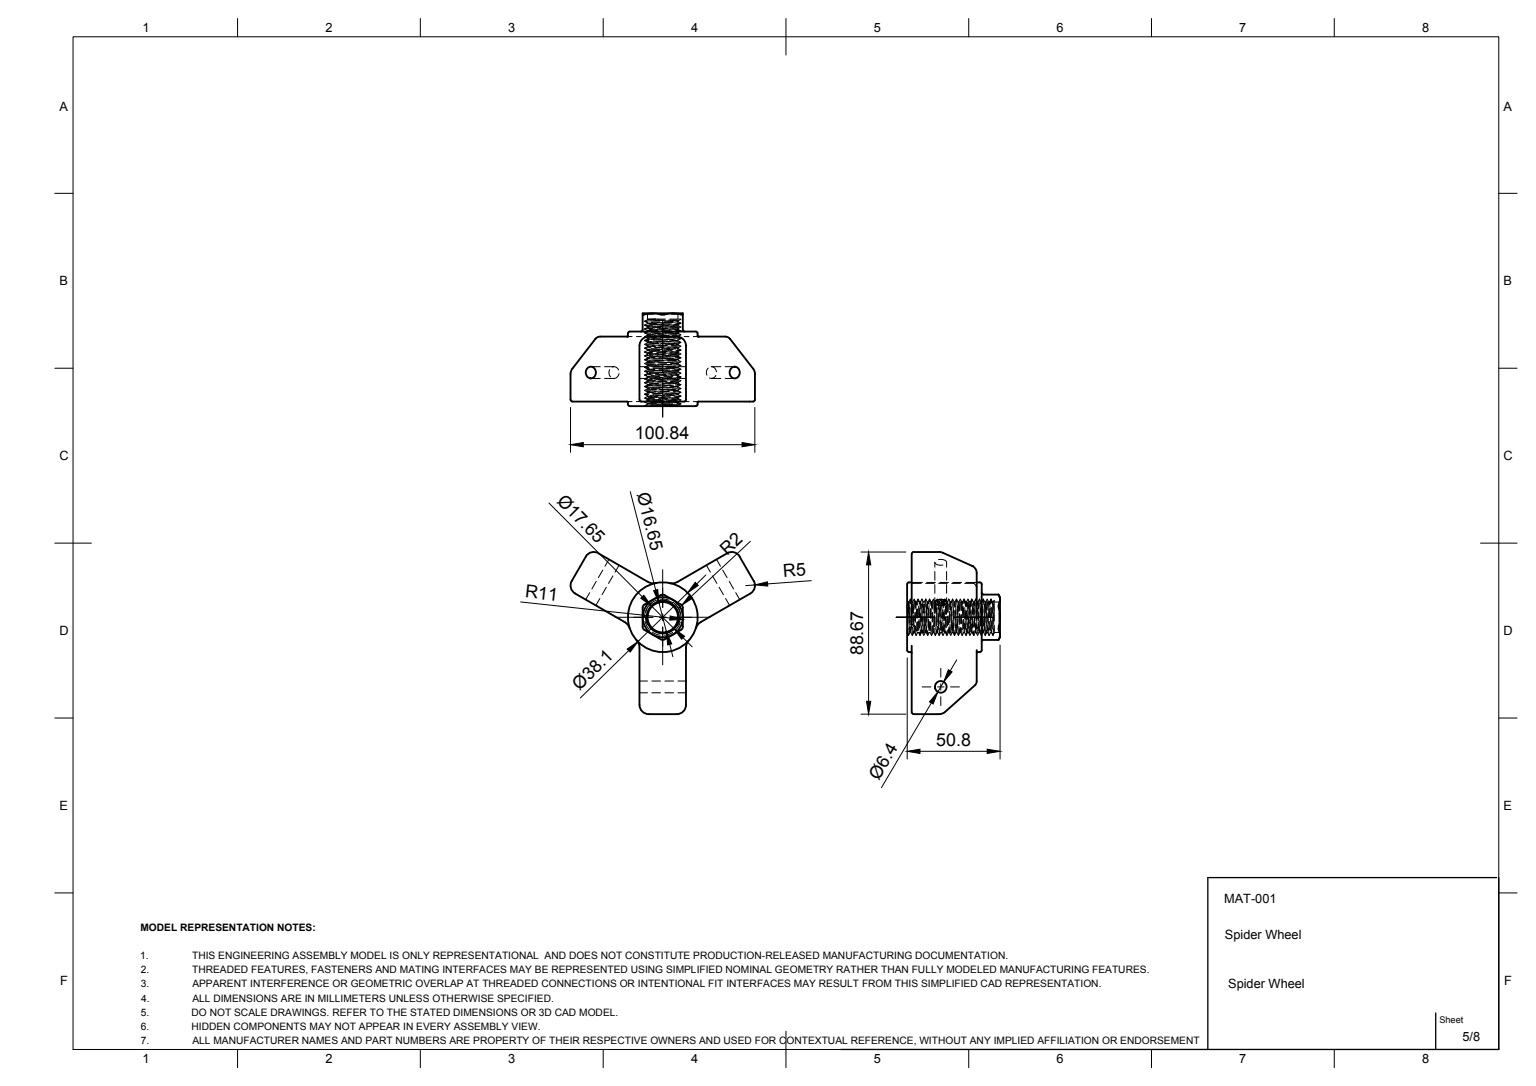
ISO-10303-21;
HEADER;
/* Generated by software containing ST-Developer
 * from STEP Tools, Inc. (www.steptools.com) 
 */

FILE_DESCRIPTION(
/* description */ ('STEP AP214'),
/* implementation_level */ '2;1');

FILE_NAME(
/* name */ 'Spider Wheel.step',
/* time_stamp */ '2026-11-14T04:30:00-08:00',
/* author */ (''),
/* organization */ (''),
/* preprocessor_version */ 'ST-DEVELOPER v20.2',
/* originating_system */ 'Autodesk Translation Framework v15.17.0.0',
/* authorisation */ '');

FILE_SCHEMA (('AUTOMOTIVE_DESIGN { 1 0 10303 214 3 1 1 }'));
ENDSEC;

DATA;
#10=MECHANICAL_DESIGN_GEOMETRIC_PRESENTATION_REPRESENTATION('',(#123),#40809);
#107=SHAPE_REPRESENTATION_RELATIONSHIP('SRR','None',#40857,#115);
#115=ADVANCED_BREP_SHAPE_REPRESENTATION('',(#131),#40801);
#123=STYLED_ITEM('',(#40906),#131);
#131=MANIFOLD_SOLID_BREP('Body1',#6298);
#139=SPHERICAL_SURFACE('',#6615,5.);
#140=SPHERICAL_SURFACE('',#6624,5.);
#141=SPHERICAL_SURFACE('',#6633,5.);
#142=SPHERICAL_SURFACE('',#6642,5.);
#143=SPHERICAL_SURFACE('',#6643,5.);
#144=SPHERICAL_SURFACE('',#6652,5.);
#148=(
BOUNDED_SURFACE()
B_SPLINE_SURFACE(1,2,((#13053,#13054,#13055,#13056,#13057,#13058,#13059,
#13060,#13061,#13062,#13063,#13064,#13065,#13066,#13067,#13068,#13069,#13070,
#13071,#13072,#13073,#13074,#13075,#13076,#13077,#13078,#13079,#13080,#13081,
#13082,#13083,#13084,#13085,#13086,#13087,#13088,#13089,#13090,#13091,#13092,
#13093,#13094,#13095,#13096,#13097,#13098,#13099,#13100,#13101,#13102,#13103,
#13104,#13105,#13106,#13107,#13108,#13109,#13110,#13111,#13112,#13113,#13114,
#13115,#13116,#13117,#13118,#13119,#13120,#13121,#13122,#13123,#13124,#13125,
#13126,#13127,#13128,#13129,#13130,#13131,#13132,#13133,#13134,#13135,#13136,
#13137,#13138,#13139,#13140,#13141,#13142,#13143,#13144,#13145,#13146,#13147,
#13148,#13149,#13150,#13151,#13152,#13153,#13154,#13155,#13156,#13157,#13158,
#13159,#13160,#13161,#13162,#13163,#13164,#13165,#13166,#13167,#13168,#13169,
#13170,#13171,#13172,#13173,#13174,#13175,#13176,#13177,#13178,#13179,#13180,
#13181,#13182,#13183,#13184,#13185,#13186,#13187,#13188,#13189,#13190,#13191,
#13192,#13193,#13194,#13195,#13196,#13197,#13198,#13199,#13200,#13201,#13202,
#13203,#13204,#13205,#13206,#13207,#13208,#13209,#13210,#13211,#13212,#13213,
#13214,#13215,#13216,#13217,#13218,#13219,#13220,#13221,#13222,#13223,#13224,
#13225,#13226,#13227,#13228,#13229,#13230,#13231,#13232,#13233,#13234,#13235,
#13236,#13237,#13238,#13239,#13240,#13241,#13242,#13243,#13244,#13245,#13246,
#13247,#13248,#13249,#13250,#13251,#13252,#13253,#13254,#13255,#13256,#13257,
#13258,#13259,#13260,#13261,#13262,#13263,#13264,#13265,#13266,#13267,#13268,
#13269,#13270,#13271,#13272,#13273,#13274,#13275,#13276,#13277,#13278,#13279,
#13280,#13281,#13282,#13283,#13284,#13285,#13286,#13287,#13288,#13289,#13290,
#13291,#13292,#13293,#13294,#13295,#13296,#13297,#13298,#13299,#13300,#13301,
#13302,#13303,#13304,#13305,#13306,#13307,#13308,#13309,#13310,#13311,#13312,
#13313,#13314,#13315,#13316,#13317,#13318,#13319,#13320,#13321,#13322,#13323,
#13324,#13325,#13326,#13327,#13328,#13329,#13330,#13331,#13332,#13333,#13334,
#13335,#13336,#13337,#13338,#13339,#13340,#13341,#13342,#13343,#13344,#13345,
#13346,#13347,#13348,#13349,#13350,#13351,#13352,#13353,#13354,#13355,#13356,
#13357,#13358,#13359,#13360,#13361,#13362,#13363,#13364,#13365,#13366,#13367,
#13368,#13369,#13370,#13371,#13372,#13373,#13374,#13375,#13376,#13377,#13378,
#13379,#13380,#13381,#13382,#13383,#13384,#13385,#13386,#13387,#13388,#13389,
#13390,#13391,#13392,#13393,#13394,#13395,#13396,#13397,#13398,#13399,#13400,
#13401,#13402,#13403,#13404,#13405,#13406,#13407,#13408,#13409,#13410,#13411,
#13412,#13413,#13414,#13415,#13416,#13417,#13418,#13419,#13420,#13421,#13422,
#13423,#13424,#13425,#13426,#13427,#13428,#13429,#13430,#13431,#13432,#13433,
#13434,#13435,#13436,#13437,#13438,#13439,#13440,#13441,#13442,#13443,#13444,
#13445,#13446,#13447,#13448,#13449,#13450,#13451,#13452,#13453,#13454,#13455,
#13456,#13457,#13458,#13459,#13460,#13461,#13462,#13463,#13464,#13465,#13466,
#13467,#13468,#13469,#13470,#13471,#13472,#13473,#13474,#13475,#13476,#13477,
#13478,#13479,#13480,#13481,#13482,#13483,#13484,#13485,#13486,#13487,#13488,
#13489,#13490,#13491,#13492,#13493,#13494,#13495,#13496,#13497,#13498,#13499,
#13500,#13501,#13502,#13503,#13504,#13505,#13506,#13507,#13508,#13509,#13510,
#13511,#13512,#13513,#13514,#13515,#13516,#13517,#13518,#13519,#13520,#13521,
#13522,#13523,#13524,#13525,#13526,#13527,#13528,#13529,#13530,#13531,#13532,
#13533,#13534,#13535,#13536,#13537,#13538,#13539,#13540,#13541,#13542,#13543,
#13544,#13545,#13546,#13547,#13548,#13549,#13550,#13551,#13552,#13553,#13554,
#13555,#13556,#13557,#13558,#13559,#13560,#13561,#13562,#13563,#13564,#13565,
#13566,#13567,#13568,#13569,#13570,#13571,#13572,#13573,#13574,#13575,#13576,
#13577,#13578,#13579,#13580,#13581,#13582,#13583,#13584,#13585,#13586,#13587,
#13588,#13589,#13590,#13591,#13592,#13593,#13594,#13595,#13596,#13597,#13598,
#13599,#13600,#13601,#13602,#13603,#13604,#13605,#13606,#13607,#13608,#13609,
#13610,#13611,#13612,#13613,#13614,#13615,#13616,#13617,#13618,#13619,#13620,
#13621,#13622,#13623,#13624,#13625,#13626,#13627,#13628,#13629,#13630,#13631,
#13632,#13633,#13634,#13635,#13636,#13637,#13638,#13639,#13640,#13641,#13642,
#13643,#13644,#13645,#13646,#13647,#13648,#13649,#13650,#13651,#13652,#13653,
#13654,#13655,#13656,#13657,#13658,#13659,#13660,#13661,#13662,#13663,#13664,
#13665,#13666,#13667,#13668,#13669,#13670,#13671,#13672,#13673,#13674,#13675,
#13676,#13677,#13678,#13679,#13680,#13681,#13682,#13683,#13684,#13685,#13686,
#13687,#13688,#13689,#13690,#13691,#13692,#13693,#13694,#13695,#13696,#13697,
#13698,#13699,#13700,#13701,#13702,#13703,#13704,#13705,#13706,#13707,#13708,
#13709,#13710,#13711,#13712,#13713,#13714,#13715,#13716,#13717,#13718,#13719,
#13720,#13721,#13722,#13723,#13724,#13725,#13726,#13727,#13728,#13729,#13730,
#13731,#13732,#13733,#13734,#13735,#13736,#13737,#13738,#13739,#13740,#13741,
#13742,#13743,#13744,#13745,#13746,#13747,#13748,#13749,#13750,#13751,#13752,
#13753,#13754,#13755,#13756,#13757,#13758,#13759,#13760,#13761,#13762,#13763,
#13764,#13765,#13766,#13767,#13768,#13769,#13770,#13771,#13772,#13773,#13774,
#13775,#13776,#13777,#13778,#13779,#13780,#13781,#13782,#13783,#13784,#13785,
#13786,#13787,#13788,#13789,#13790,#13791,#13792,#13793,#13794,#13795,#13796,
#13797,#13798,#13799,#13800,#13801,#13802,#13803,#13804,#13805,#13806,#13807,
#13808,#13809,#13810,#13811,#13812,#13813,#13814,#13815,#13816,#13817,#13818,
#13819,#13820,#13821,#13822,#13823,#13824,#13825,#13826,#13827,#13828,#13829,
#13830,#13831,#13832,#13833,#13834,#13835,#13836,#13837,#13838,#13839,#13840,
#13841,#13842,#13843,#13844,#13845,#13846,#13847,#13848,#13849,#13850,#13851,
#13852,#13853,#13854,#13855,#13856,#13857,#13858,#13859,#13860,#13861,#13862,
#13863,#13864,#13865,#13866,#13867,#13868,#13869,#13870,#13871,#13872,#13873,
#13874,#13875,#13876,#13877,#13878,#13879,#13880,#13881,#13882,#13883,#13884,
#13885,#13886,#13887,#13888,#13889,#13890,#13891,#13892,#13893,#13894,#13895,
#13896,#13897,#13898,#13899,#13900,#13901,#13902,#13903,#13904,#13905,#13906,
#13907,#13908,#13909,#13910,#13911,#13912,#13913,#13914,#13915,#13916,#13917,
#13918,#13919,#13920,#13921,#13922,#13923,#13924,#13925,#13926,#13927,#13928,
#13929,#13930,#13931,#13932,#13933,#13934,#13935,#13936,#13937,#13938,#13939,
#13940,#13941,#13942,#13943,#13944,#13945,#13946,#13947,#13948,#13949,#13950,
#13951,#13952,#13953,#13954,#13955,#13956,#13957,#13958,#13959,#13960,#13961,
#13962,#13963,#13964,#13965,#13966,#13967,#13968,#13969,#13970,#13971,#13972,
#13973,#13974,#13975,#13976,#13977,#13978,#13979,#13980,#13981,#13982,#13983,
#13984,#13985,#13986,#13987,#13988,#13989,#13990,#13991,#13992,#13993,#13994,
#13995,#13996,#13997,#13998,#13999,#14000,#14001,#14002,#14003,#14004,#14005,
#14006,#14007,#14008,#14009,#14010,#14011,#14012,#14013,#14014,#14015,#14016,
#14017,#14018,#14019,#14020,#14021,#14022,#14023,#14024,#14025),(#14026,
#14027,#14028,#14029,#14030,#14031,#14032,#14033,#14034,#14035,#14036,#14037,
#14038,#14039,#14040,#14041,#14042,#14043,#14044,#14045,#14046,#14047,#14048,
#14049,#14050,#14051,#14052,#14053,#14054,#14055,#14056,#14057,#14058,#14059,
#14060,#14061,#14062,#14063,#14064,#14065,#14066,#14067,#14068,#14069,#14070,
#14071,#14072,#14073,#14074,#14075,#14076,#14077,#14078,#14079,#14080,#14081,
#14082,#14083,#14084,#14085,#14086,#14087,#14088,#14089,#14090,#14091,#14092,
#14093,#14094,#14095,#14096,#14097,#14098,#14099,#14100,#14101,#14102,#14103,
#14104,#14105,#14106,#14107,#14108,#14109,#14110,#14111,#14112,#14113,#14114,
#14115,#14116,#14117,#14118,#14119,#14120,#14121,#14122,#14123,#14124,#14125,
#14126,#14127,#14128,#14129,#14130,#14131,#14132,#14133,#14134,#14135,#14136,
#14137,#14138,#14139,#14140,#14141,#14142,#14143,#14144,#14145,#14146,#14147,
#14148,#14149,#14150,#14151,#14152,#14153,#14154,#14155,#14156,#14157,#14158,
#14159,#14160,#14161,#14162,#14163,#14164,#14165,#14166,#14167,#14168,#14169,
#14170,#14171,#14172,#14173,#14174,#14175,#14176,#14177,#14178,#14179,#14180,
#14181,#14182,#14183,#14184,#14185,#14186,#14187,#14188,#14189,#14190,#14191,
#14192,#14193,#14194,#14195,#14196,#14197,#14198,#14199,#14200,#14201,#14202,
#14203,#14204,#14205,#14206,#14207,#14208,#14209,#14210,#14211,#14212,#14213,
#14214,#14215,#14216,#14217,#14218,#14219,#14220,#14221,#14222,#14223,#14224,
#14225,#14226,#14227,#14228,#14229,#14230,#14231,#14232,#14233,#14234,#14235,
#14236,#14237,#14238,#14239,#14240,#14241,#14242,#14243,#14244,#14245,#14246,
#14247,#14248,#14249,#14250,#14251,#14252,#14253,#14254,#14255,#14256,#14257,
#14258,#14259,#14260,#14261,#14262,#14263,#14264,#14265,#14266,#14267,#14268,
#14269,#14270,#14271,#14272,#14273,#14274,#14275,#14276,#14277,#14278,#14279,
#14280,#14281,#14282,#14283,#14284,#14285,#14286,#14287,#14288,#14289,#14290,
#14291,#14292,#14293,#14294,#14295,#14296,#14297,#14298,#14299,#14300,#14301,
#14302,#14303,#14304,#14305,#14306,#14307,#14308,#14309,#14310,#14311,#14312,
#14313,#14314,#14315,#14316,#14317,#14318,#14319,#14320,#14321,#14322,#14323,
#14324,#14325,#14326,#14327,#14328,#14329,#14330,#14331,#14332,#14333,#14334,
#14335,#14336,#14337,#14338,#14339,#14340,#14341,#14342,#14343,#14344,#14345,
#14346,#14347,#14348,#14349,#14350,#14351,#14352,#14353,#14354,#14355,#14356,
#14357,#14358,#14359,#14360,#14361,#14362,#14363,#14364,#14365,#14366,#14367,
#14368,#14369,#14370,#14371,#14372,#14373,#14374,#14375,#14376,#14377,#14378,
#14379,#14380,#14381,#14382,#14383,#14384,#14385,#14386,#14387,#14388,#14389,
#14390,#14391,#14392,#14393,#14394,#14395,#14396,#14397,#14398,#14399,#14400,
#14401,#14402,#14403,#14404,#14405,#14406,#14407,#14408,#14409,#14410,#14411,
#14412,#14413,#14414,#14415,#14416,#14417,#14418,#14419,#14420,#14421,#14422,
#14423,#14424,#14425,#14426,#14427,#14428,#14429,#14430,#14431,#14432,#14433,
#14434,#14435,#14436,#14437,#14438,#14439,#14440,#14441,#14442,#14443,#14444,
#14445,#14446,#14447,#14448,#14449,#14450,#14451,#14452,#14453,#14454,#14455,
#14456,#14457,#14458,#14459,#14460,#14461,#14462,#14463,#14464,#14465,#14466,
#14467,#14468,#14469,#14470,#14471,#14472,#14473,#14474,#14475,#14476,#14477,
#14478,#14479,#14480,#14481,#14482,#14483,#14484,#14485,#14486,#14487,#14488,
#14489,#14490,#14491,#14492,#14493,#14494,#14495,#14496,#14497,#14498,#14499,
#14500,#14501,#14502,#14503,#14504,#14505,#14506,#14507,#14508,#14509,#14510,
#14511,#14512,#14513,#14514,#14515,#14516,#14517,#14518,#14519,#14520,#14521,
#14522,#14523,#14524,#14525,#14526,#14527,#14528,#14529,#14530,#14531,#14532,
#14533,#14534,#14535,#14536,#14537,#14538,#14539,#14540,#14541,#14542,#14543,
#14544,#14545,#14546,#14547,#14548,#14549,#14550,#14551,#14552,#14553,#14554,
#14555,#14556,#14557,#14558,#14559,#14560,#14561,#14562,#14563,#14564,#14565,
#14566,#14567,#14568,#14569,#14570,#14571,#14572,#14573,#14574,#14575,#14576,
#14577,#14578,#14579,#14580,#14581,#14582,#14583,#14584,#14585,#14586,#14587,
#14588,#14589,#14590,#14591,#14592,#14593,#14594,#14595,#14596,#14597,#14598,
#14599,#14600,#14601,#14602,#14603,#14604,#14605,#14606,#14607,#14608,#14609,
#14610,#14611,#14612,#14613,#14614,#14615,#14616,#14617,#14618,#14619,#14620,
#14621,#14622,#14623,#14624,#14625,#14626,#14627,#14628,#14629,#14630,#14631,
#14632,#14633,#14634,#14635,#14636,#14637,#14638,#14639,#14640,#14641,#14642,
#14643,#14644,#14645,#14646,#14647,#14648,#14649,#14650,#14651,#14652,#14653,
#14654,#14655,#14656,#14657,#14658,#14659,#14660,#14661,#14662,#14663,#14664,
#14665,#14666,#14667,#14668,#14669,#14670,#14671,#14672,#14673,#14674,#14675,
#14676,#14677,#14678,#14679,#14680,#14681,#14682,#14683,#14684,#14685,#14686,
#14687,#14688,#14689,#14690,#14691,#14692,#14693,#14694,#14695,#14696,#14697,
#14698,#14699,#14700,#14701,#14702,#14703,#14704,#14705,#14706,#14707,#14708,
#14709,#14710,#14711,#14712,#14713,#14714,#14715,#14716,#14717,#14718,#14719,
#14720,#14721,#14722,#14723,#14724,#14725,#14726,#14727,#14728,#14729,#14730,
#14731,#14732,#14733,#14734,#14735,#14736,#14737,#14738,#14739,#14740,#14741,
#14742,#14743,#14744,#14745,#14746,#14747,#14748,#14749,#14750,#14751,#14752,
#14753,#14754,#14755,#14756,#14757,#14758,#14759,#14760,#14761,#14762,#14763,
#14764,#14765,#14766,#14767,#14768,#14769,#14770,#14771,#14772,#14773,#14774,
#14775,#14776,#14777,#14778,#14779,#14780,#14781,#14782,#14783,#14784,#14785,
#14786,#14787,#14788,#14789,#14790,#14791,#14792,#14793,#14794,#14795,#14796,
#14797,#14798,#14799,#14800,#14801,#14802,#14803,#14804,#14805,#14806,#14807,
#14808,#14809,#14810,#14811,#14812,#14813,#14814,#14815,#14816,#14817,#14818,
#14819,#14820,#14821,#14822,#14823,#14824,#14825,#14826,#14827,#14828,#14829,
#14830,#14831,#14832,#14833,#14834,#14835,#14836,#14837,#14838,#14839,#14840,
#14841,#14842,#14843,#14844,#14845,#14846,#14847,#14848,#14849,#14850,#14851,
#14852,#14853,#14854,#14855,#14856,#14857,#14858,#14859,#14860,#14861,#14862,
#14863,#14864,#14865,#14866,#14867,#14868,#14869,#14870,#14871,#14872,#14873,
#14874,#14875,#14876,#14877,#14878,#14879,#14880,#14881,#14882,#14883,#14884,
#14885,#14886,#14887,#14888,#14889,#14890,#14891,#14892,#14893,#14894,#14895,
#14896,#14897,#14898,#14899,#14900,#14901,#14902,#14903,#14904,#14905,#14906,
#14907,#14908,#14909,#14910,#14911,#14912,#14913,#14914,#14915,#14916,#14917,
#14918,#14919,#14920,#14921,#14922,#14923,#14924,#14925,#14926,#14927,#14928,
#14929,#14930,#14931,#14932,#14933,#14934,#14935,#14936,#14937,#14938,#14939,
#14940,#14941,#14942,#14943,#14944,#14945,#14946,#14947,#14948,#14949,#14950,
#14951,#14952,#14953,#14954,#14955,#14956,#14957,#14958,#14959,#14960,#14961,
#14962,#14963,#14964,#14965,#14966,#14967,#14968,#14969,#14970,#14971,#14972,
#14973,#14974,#14975,#14976,#14977,#14978,#14979,#14980,#14981,#14982,#14983,
#14984,#14985,#14986,#14987,#14988,#14989,#14990,#14991,#14992,#14993,#14994,
#14995,#14996,#14997,#14998)),.UNSPECIFIED.,.F.,.F.,.F.)
B_SPLINE_SURFACE_WITH_KNOTS((2,2),(3,2,2,2,2,2,2,2,2,2,2,2,2,2,2,2,2,2,
2,2,2,2,2,2,2,2,2,2,2,2,2,2,2,2,2,2,2,2,2,2,2,2,2,2,2,2,2,2,2,2,2,2,2,2,
2,2,2,2,2,2,2,2,2,2,2,2,2,2,2,2,2,2,2,2,2,2,2,2,2,2,2,2,2,2,2,2,2,2,2,2,
2,2,2,2,2,2,2,2,2,2,2,2,2,2,2,2,2,2,2,2,2,2,2,2,2,2,2,2,2,2,2,2,2,2,2,2,
2,2,2,2,2,2,2,2,2,2,2,2,2,2,2,2,2,2,2,2,2,2,2,2,2,2,2,2,2,2,2,2,2,2,2,2,
2,2,2,2,2,2,2,2,2,2,2,2,2,2,2,2,2,2,2,2,2,2,2,2,2,2,2,2,2,2,2,2,2,2,2,2,
2,2,2,2,2,2,2,2,2,2,2,2,2,2,2,2,2,2,2,2,2,2,2,2,2,2,2,2,2,2,2,2,2,2,2,2,
2,2,2,2,2,2,2,2,2,2,2,2,2,2,2,2,2,2,2,2,2,2,2,2,2,2,2,2,2,2,2,2,2,2,2,2,
2,2,2,2,2,2,2,2,2,2,2,2,2,2,2,2,2,2,2,2,2,2,2,2,2,2,2,2,2,2,2,2,2,2,2,2,
2,2,2,2,2,2,2,2,2,2,2,2,2,2,2,2,2,2,2,2,2,2,2,2,2,2,2,2,2,2,2,2,2,2,2,2,
2,2,2,2,2,2,2,2,2,2,2,2,2,2,2,2,2,2,2,2,2,2,2,2,2,2,2,2,2,2,2,2,2,2,2,2,
2,2,2,2,2,2,2,2,2,2,2,2,2,2,2,2,2,2,2,2,2,2,2,2,2,2,2,2,2,2,2,2,2,2,2,2,
2,2,2,2,2,2,2,2,2,2,2,2,2,2,2,2,2,2,2,2,2,2,2,2,2,2,2,2,2,2,2,2,2,2,2,2,
2,2,2,2,2,2,2,2,2,2,2,2,2,2,2,2,2,2,2,2,2,2,2,2,2,2,2,2,2,2,2,2,2,2,2,2,
3),(0.,1.00000404874212),(0.,0.00205761316872428,0.00411522633744856,0.00617283950617284,
0.00823045267489712,0.0102880658436214,0.0123456790123457,0.01440329218107,
0.0164609053497942,0.0185185185185185,0.0205761316872428,0.0226337448559671,
0.0246913580246914,0.0267489711934156,0.0288065843621399,0.0308641975308642,
0.0329218106995885,0.0349794238683128,0.037037037037037,0.0390946502057613,
0.0411522633744856,0.0432098765432099,0.0452674897119342,0.0473251028806584,
0.0493827160493827,0.051440329218107,0.0534979423868313,0.0555555555555556,
0.0576131687242798,0.0596707818930041,0.0617283950617284,0.0637860082304527,
0.065843621399177,0.0679012345679012,0.0699588477366255,0.0720164609053498,
0.0740740740740741,0.0761316872427984,0.0781893004115226,0.0802469135802469,
0.0823045267489712,0.0843621399176955,0.0864197530864197,0.088477366255144,
0.0905349794238683,0.0925925925925926,0.0946502057613169,0.0967078189300412,
0.0987654320987654,0.10082304526749,0.102880658436214,0.104938271604938,
0.106995884773663,0.109053497942387,0.111111111111111,0.113168724279835,
0.11522633744856,0.117283950617284,0.119341563786008,0.121399176954733,
0.123456790123457,0.125514403292181,0.127572016460905,0.12962962962963,
0.131687242798354,0.133744855967078,0.135802469135802,0.137860082304527,
0.139917695473251,0.141975308641975,0.1440329218107,0.146090534979424,0.148148148148148,
0.150205761316872,0.152263374485597,0.154320987654321,0.156378600823045,
0.15843621399177,0.160493827160494,0.162551440329218,0.164609053497942,
0.166666666666667,0.168724279835391,0.170781893004115,0.172839506172839,
0.174897119341564,0.176954732510288,0.179012345679012,0.181069958847737,
0.183127572016461,0.185185185185185,0.187242798353909,0.189300411522634,
0.191358024691358,0.193415637860082,0.195473251028807,0.197530864197531,
0.199588477366255,0.201646090534979,0.203703703703704,0.205761316872428,
0.207818930041152,0.209876543209877,0.211934156378601,0.213991769547325,
0.216049382716049,0.218106995884774,0.220164609053498,0.222222222222222,
0.224279835390947,0.226337448559671,0.228395061728395,0.230452674897119,
0.232510288065844,0.234567901234568,0.236625514403292,0.238683127572016,
0.240740740740741,0.242798353909465,0.244855967078189,0.246913580246914,
0.248971193415638,0.251028806584362,0.253086419753086,0.255144032921811,
0.257201646090535,0.259259259259259,0.261316872427984,0.263374485596708,
0.265432098765432,0.267489711934156,0.269547325102881,0.271604938271605,
0.273662551440329,0.275720164609054,0.277777777777778,0.279835390946502,
0.281893004115226,0.283950617283951,0.286008230452675,0.288065843621399,
0.290123456790123,0.292181069958848,0.294238683127572,0.296296296296296,
0.298353909465021,0.300411522633745,0.302469135802469,0.304526748971193,
0.306584362139918,0.308641975308642,0.310699588477366,0.312757201646091,
0.314814814814815,0.316872427983539,0.318930041152263,0.320987654320988,
0.323045267489712,0.325102880658436,0.327160493827161,0.329218106995885,
0.331275720164609,0.333333333333333,0.335390946502058,0.337448559670782,
0.339506172839506,0.34156378600823,0.343621399176955,0.345679012345679,
0.347736625514403,0.349794238683128,0.351851851851852,0.353909465020576,
0.3559670781893,0.358024691358025,0.360082304526749,0.362139917695473,0.364197530864198,
0.366255144032922,0.368312757201646,0.37037037037037,0.372427983539095,
0.374485596707819,0.376543209876543,0.378600823045267,0.380658436213992,
0.382716049382716,0.38477366255144,0.386831275720165,0.388888888888889,
0.390946502057613,0.393004115226337,0.395061728395062,0.397119341563786,
0.39917695473251,0.401234567901235,0.403292181069959,0.405349794238683,
0.407407407407407,0.409465020576132,0.411522633744856,0.41358024691358,
0.415637860082305,0.417695473251029,0.419753086419753,0.421810699588477,
0.423868312757202,0.425925925925926,0.42798353909465,0.430041152263374,
0.432098765432099,0.434156378600823,0.436213991769547,0.438271604938272,
0.440329218106996,0.44238683127572,0.444444444444444,0.446502057613169,
0.448559670781893,0.450617283950617,0.452674897119342,0.454732510288066,
0.45679012345679,0.458847736625514,0.460905349794239,0.462962962962963,
0.465020576131687,0.467078189300412,0.469135802469136,0.47119341563786,
0.473251028806584,0.475308641975309,0.477366255144033,0.479423868312757,
0.481481481481481,0.483539094650206,0.48559670781893,0.487654320987654,
0.489711934156379,0.491769547325103,0.493827160493827,0.495884773662551,
0.497942386831276,0.5,0.502057613168724,0.504115226337449,0.506172839506173,
0.508230452674897,0.510288065843621,0.512345679012346,0.51440329218107,
0.516460905349794,0.518518518518518,0.520576131687243,0.522633744855967,
0.524691358024691,0.526748971193416,0.52880658436214,0.530864197530864,
0.532921810699588,0.534979423868313,0.537037037037037,0.539094650205761,
0.541152263374486,0.54320987654321,0.545267489711934,0.547325102880658,
0.549382716049383,0.551440329218107,0.553497942386831,0.555555555555556,
0.55761316872428,0.559670781893004,0.561728395061728,0.563786008230453,
0.565843621399177,0.567901234567901,0.569958847736626,0.57201646090535,
0.574074074074074,0.576131687242798,0.578189300411523,0.580246913580247,
0.582304526748971,0.584362139917695,0.58641975308642,0.588477366255144,
0.590534979423868,0.592592592592593,0.594650205761317,0.596707818930041,
0.598765432098765,0.60082304526749,0.602880658436214,0.604938271604938,
0.606995884773663,0.609053497942387,0.611111111111111,0.613168724279835,
0.61522633744856,0.617283950617284,0.619341563786008,0.621399176954732,
0.623456790123457,0.625514403292181,0.627572016460905,0.62962962962963,
0.631687242798354,0.633744855967078,0.635802469135803,0.637860082304527,
0.639917695473251,0.641975308641975,0.6440329218107,0.646090534979424,0.648148148148148,
0.650205761316872,0.652263374485597,0.654320987654321,0.656378600823045,
0.65843621399177,0.660493827160494,0.662551440329218,0.664609053497942,
0.666666666666667,0.668724279835391,0.670781893004115,0.672839506172839,
0.674897119341564,0.676954732510288,0.679012345679012,0.681069958847737,
0.683127572016461,0.685185185185185,0.687242798353909,0.689300411522634,
0.691358024691358,0.693415637860082,0.695473251028807,0.697530864197531,
0.699588477366255,0.701646090534979,0.703703703703704,0.705761316872428,
0.707818930041152,0.709876543209877,0.711934156378601,0.713991769547325,
0.716049382716049,0.718106995884774,0.720164609053498,0.722222222222222,
0.724279835390947,0.726337448559671,0.728395061728395,0.730452674897119,
0.732510288065844,0.734567901234568,0.736625514403292,0.738683127572016,
0.740740740740741,0.742798353909465,0.744855967078189,0.746913580246914,
0.748971193415638,0.751028806584362,0.753086419753086,0.755144032921811,
0.757201646090535,0.759259259259259,0.761316872427984,0.763374485596708,
0.765432098765432,0.767489711934156,0.769547325102881,0.771604938271605,
0.773662551440329,0.775720164609053,0.777777777777778,0.779835390946502,
0.781893004115226,0.783950617283951,0.786008230452675,0.788065843621399,
0.790123456790123,0.792181069958848,0.794238683127572,0.796296296296296,
0.798353909465021,0.800411522633745,0.802469135802469,0.804526748971193,
0.806584362139918,0.808641975308642,0.810699588477366,0.812757201646091,
0.814814814814815,0.816872427983539,0.818930041152263,0.820987654320988,
0.823045267489712,0.825102880658436,0.827160493827161,0.829218106995885,
0.831275720164609,0.833333333333333,0.835390946502058,0.837448559670782,
0.839506172839506,0.84156378600823,0.843621399176955,0.845679012345679,
0.847736625514403,0.849794238683128,0.851851851851852,0.853909465020576,
0.8559670781893,0.858024691358025,0.860082304526749,0.862139917695473,0.864197530864197,
0.866255144032922,0.868312757201646,0.87037037037037,0.872427983539095,
0.874485596707819,0.876543209876543,0.878600823045268,0.880658436213992,
0.882716049382716,0.88477366255144,0.886831275720165,0.888888888888889,
0.890946502057613,0.893004115226337,0.895061728395062,0.897119341563786,
0.89917695473251,0.901234567901235,0.903292181069959,0.905349794238683,
0.907407407407407,0.909465020576132,0.911522633744856,0.91358024691358,
0.915637860082305,0.917695473251029,0.919753086419753,0.921810699588477,
0.923868312757202,0.925925925925926,0.92798353909465,0.930041152263374,
0.932098765432099,0.934156378600823,0.936213991769547,0.938271604938272,
0.940329218106996,0.94238683127572,0.944444444444444,0.946502057613169,
0.948559670781893,0.950617283950617,0.952674897119342,0.954732510288066,
0.95679012345679,0.958847736625514,0.960905349794239,0.962962962962963,
0.965020576131687,0.967078189300412,0.969135802469136,0.97119341563786,
0.973251028806584,0.975308641975309,0.977366255144033,0.979423868312757,
0.981481481481482,0.983539094650206,0.98559670781893,0.987654320987654,
0.989711934156379,0.991769547325103,0.993827160493827,0.995884773662551,
0.997942386831276,1.),.UNSPECIFIED.)
GEOMETRIC_REPRESENTATION_ITEM()
RATIONAL_B_SPLINE_SURFACE(((1.,0.866025403784439,1.,0.866025403784439,1.,
0.866025403784439,1.,0.866025403784439,1.,0.866025403784439,1.,0.866025403784439,
1.,0.866025403784439,1.,0.866025403784439,1.,0.866025403784439,1.,0.866025403784439,
1.,0.866025403784439,1.,0.866025403784439,1.,0.866025403784439,1.,0.866025403784439,
1.,0.866025403784439,1.,0.866025403784439,1.,0.866025403784439,1.,0.866025403784439,
1.,0.866025403784439,1.,0.866025403784439,1.,0.866025403784439,1.,0.866025403784439,
1.,0.866025403784439,1.,0.866025403784439,1.,0.866025403784439,1.,0.866025403784439,
1.,0.866025403784439,1.,0.866025403784439,1.,0.866025403784439,1.,0.866025403784439,
1.,0.866025403784439,1.,0.866025403784439,1.,0.866025403784439,1.,0.866025403784439,
1.,0.866025403784439,1.,0.866025403784439,1.,0.866025403784439,1.,0.866025403784439,
1.,0.866025403784439,1.,0.866025403784439,1.,0.866025403784439,1.,0.866025403784439,
1.,0.866025403784439,1.,0.866025403784439,1.,0.866025403784439,1.,0.866025403784439,
1.,0.866025403784439,1.,0.866025403784439,1.,0.866025403784439,1.,0.866025403784439,
1.,0.866025403784439,1.,0.866025403784439,1.,0.866025403784439,1.,0.866025403784439,
1.,0.866025403784439,1.,0.866025403784439,1.,0.866025403784439,1.,0.866025403784439,
1.,0.866025403784439,1.,0.866025403784439,1.,0.866025403784439,1.,0.866025403784439,
1.,0.866025403784439,1.,0.866025403784439,1.,0.866025403784439,1.,0.866025403784439,
1.,0.866025403784439,1.,0.866025403784439,1.,0.866025403784439,1.,0.866025403784439,
1.,0.866025403784439,1.,0.866025403784439,1.,0.866025403784439,1.,0.866025403784439,
1.,0.866025403784439,1.,0.866025403784439,1.,0.866025403784439,1.,0.866025403784439,
1.,0.866025403784439,1.,0.866025403784439,1.,0.866025403784439,1.,0.866025403784439,
1.,0.866025403784439,1.,0.866025403784439,1.,0.866025403784439,1.,0.866025403784439,
1.,0.866025403784439,1.,0.866025403784439,1.,0.866025403784439,1.,0.866025403784439,
1.,0.866025403784439,1.,0.866025403784439,1.,0.866025403784439,1.,0.866025403784439,
1.,0.866025403784439,1.,0.866025403784439,1.,0.866025403784439,1.,0.866025403784439,
1.,0.866025403784439,1.,0.866025403784439,1.,0.866025403784439,1.,0.866025403784439,
1.,0.866025403784439,1.,0.866025403784439,1.,0.866025403784439,1.,0.866025403784439,
1.,0.866025403784439,1.,0.866025403784439,1.,0.866025403784439,1.,0.866025403784439,
1.,0.866025403784439,1.,0.866025403784439,1.,0.866025403784439,1.,0.866025403784439,
1.,0.866025403784439,1.,0.866025403784439,1.,0.866025403784439,1.,0.866025403784439,
1.,0.866025403784439,1.,0.866025403784439,1.,0.866025403784439,1.,0.866025403784439,
1.,0.866025403784439,1.,0.866025403784439,1.,0.866025403784439,1.,0.866025403784439,
1.,0.866025403784439,1.,0.866025403784439,1.,0.866025403784439,1.,0.866025403784439,
1.,0.866025403784439,1.,0.866025403784439,1.,0.866025403784439,1.,0.866025403784439,
1.,0.866025403784439,1.,0.866025403784439,1.,0.866025403784439,1.,0.866025403784439,
1.,0.866025403784439,1.,0.866025403784439,1.,0.866025403784439,1.,0.866025403784439,
1.,0.866025403784439,1.,0.866025403784439,1.,0.866025403784439,1.,0.866025403784439,
1.,0.866025403784439,1.,0.866025403784439,1.,0.866025403784439,1.,0.866025403784439,
1.,0.866025403784439,1.,0.866025403784439,1.,0.866025403784439,1.,0.866025403784439,
1.,0.866025403784439,1.,0.866025403784439,1.,0.866025403784439,1.,0.866025403784439,
1.,0.866025403784439,1.,0.866025403784439,1.,0.866025403784439,1.,0.866025403784439,
1.,0.866025403784439,1.,0.866025403784439,1.,0.866025403784439,1.,0.866025403784439,
1.,0.866025403784439,1.,0.866025403784439,1.,0.866025403784439,1.,0.866025403784439,
1.,0.866025403784439,1.,0.866025403784439,1.,0.866025403784439,1.,0.866025403784439,
1.,0.866025403784439,1.,0.866025403784439,1.,0.866025403784439,1.,0.866025403784439,
1.,0.866025403784439,1.,0.866025403784439,1.,0.866025403784439,1.,0.866025403784439,
1.,0.866025403784439,1.,0.866025403784439,1.,0.866025403784439,1.,0.866025403784439,
1.,0.866025403784439,1.,0.866025403784439,1.,0.866025403784439,1.,0.866025403784439,
1.,0.866025403784439,1.,0.866025403784439,1.,0.866025403784439,1.,0.866025403784439,
1.,0.866025403784439,1.,0.866025403784439,1.,0.866025403784439,1.,0.866025403784439,
1.,0.866025403784439,1.,0.866025403784439,1.,0.866025403784439,1.,0.866025403784439,
1.,0.866025403784439,1.,0.866025403784439,1.,0.866025403784439,1.,0.866025403784439,
1.,0.866025403784439,1.,0.866025403784439,1.,0.866025403784439,1.,0.866025403784439,
1.,0.866025403784439,1.,0.866025403784439,1.,0.866025403784439,1.,0.866025403784439,
1.,0.866025403784439,1.,0.866025403784439,1.,0.866025403784439,1.,0.866025403784439,
1.,0.866025403784439,1.,0.866025403784439,1.,0.866025403784439,1.,0.866025403784439,
1.,0.866025403784439,1.,0.866025403784439,1.,0.866025403784439,1.,0.866025403784439,
1.,0.866025403784439,1.,0.866025403784439,1.,0.866025403784439,1.,0.866025403784439,
1.,0.866025403784439,1.,0.866025403784439,1.,0.866025403784439,1.,0.866025403784439,
1.,0.866025403784439,1.,0.866025403784439,1.,0.866025403784439,1.,0.866025403784439,
1.,0.866025403784439,1.,0.866025403784439,1.,0.866025403784439,1.,0.866025403784439,
1.,0.866025403784439,1.,0.866025403784439,1.,0.866025403784439,1.,0.866025403784439,
1.,0.866025403784439,1.,0.866025403784439,1.,0.866025403784439,1.,0.866025403784439,
1.,0.866025403784439,1.,0.866025403784439,1.,0.866025403784439,1.,0.866025403784439,
1.,0.866025403784439,1.,0.866025403784439,1.,0.866025403784439,1.,0.866025403784439,
1.,0.866025403784439,1.,0.866025403784439,1.,0.866025403784439,1.,0.866025403784439,
1.,0.866025403784439,1.,0.866025403784439,1.,0.866025403784439,1.,0.866025403784439,
1.,0.866025403784439,1.,0.866025403784439,1.,0.866025403784439,1.,0.866025403784439,
1.,0.866025403784439,1.,0.866025403784439,1.,0.866025403784439,1.,0.866025403784439,
1.,0.866025403784439,1.,0.866025403784439,1.,0.866025403784439,1.,0.866025403784439,
1.,0.866025403784439,1.,0.866025403784439,1.,0.866025403784439,1.,0.866025403784439,
1.,0.866025403784439,1.,0.866025403784439,1.,0.866025403784439,1.,0.866025403784439,
1.,0.866025403784439,1.,0.866025403784439,1.,0.866025403784439,1.,0.866025403784439,
1.,0.866025403784439,1.,0.866025403784439,1.,0.866025403784439,1.,0.866025403784439,
1.,0.866025403784439,1.,0.866025403784439,1.,0.866025403784439,1.,0.866025403784439,
1.,0.866025403784439,1.,0.866025403784439,1.,0.866025403784439,1.,0.866025403784439,
1.,0.866025403784439,1.,0.866025403784439,1.,0.866025403784439,1.,0.866025403784439,
1.,0.866025403784439,1.,0.866025403784439,1.,0.866025403784439,1.,0.866025403784439,
1.,0.866025403784439,1.,0.866025403784439,1.,0.866025403784439,1.,0.866025403784439,
1.,0.866025403784439,1.,0.866025403784439,1.,0.866025403784439,1.,0.866025403784439,
1.,0.866025403784439,1.,0.866025403784439,1.,0.866025403784439,1.,0.866025403784439,
1.,0.866025403784439,1.,0.866025403784439,1.,0.866025403784439,1.,0.866025403784439,
1.,0.866025403784439,1.,0.866025403784439,1.,0.866025403784439,1.,0.866025403784439,
1.,0.866025403784439,1.,0.866025403784439,1.,0.866025403784439,1.,0.866025403784439,
1.,0.866025403784439,1.,0.866025403784439,1.,0.866025403784439,1.,0.866025403784439,
1.,0.866025403784439,1.,0.866025403784439,1.,0.866025403784439,1.,0.866025403784439,
1.,0.866025403784439,1.,0.866025403784439,1.,0.866025403784439,1.,0.866025403784439,
1.,0.866025403784439,1.,0.866025403784439,1.,0.866025403784439,1.,0.866025403784439,
1.,0.866025403784439,1.,0.866025403784439,1.,0.866025403784439,1.,0.866025403784439,
1.,0.866025403784439,1.,0.866025403784439,1.,0.866025403784439,1.,0.866025403784439,
1.,0.866025403784439,1.,0.866025403784439,1.,0.866025403784439,1.,0.866025403784439,
1.,0.866025403784439,1.,0.866025403784439,1.,0.866025403784439,1.,0.866025403784439,
1.,0.866025403784439,1.,0.866025403784439,1.,0.866025403784439,1.,0.866025403784439,
1.,0.866025403784439,1.,0.866025403784439,1.,0.866025403784439,1.,0.866025403784439,
1.,0.866025403784439,1.,0.866025403784439,1.,0.866025403784439,1.,0.866025403784439,
1.,0.866025403784439,1.,0.866025403784439,1.,0.866025403784439,1.,0.866025403784439,
1.,0.866025403784439,1.,0.866025403784439,1.,0.866025403784439,1.,0.866025403784439,
1.,0.866025403784439,1.,0.866025403784439,1.,0.866025403784439,1.,0.866025403784439,
1.,0.866025403784439,1.,0.866025403784439,1.,0.866025403784439,1.,0.866025403784439,
1.,0.866025403784439,1.,0.866025403784439,1.,0.866025403784439,1.,0.866025403784439,
1.,0.866025403784439,1.,0.866025403784439,1.,0.866025403784439,1.,0.866025403784439,
1.,0.866025403784439,1.,0.866025403784439,1.,0.866025403784439,1.,0.866025403784439,
1.,0.866025403784439,1.,0.866025403784439,1.,0.866025403784439,1.,0.866025403784439,
1.,0.866025403784439,1.,0.866025403784439,1.,0.866025403784439,1.,0.866025403784439,
1.,0.866025403784439,1.,0.866025403784439,1.,0.866025403784439,1.,0.866025403784439,
1.,0.866025403784439,1.,0.866025403784439,1.,0.866025403784439,1.,0.866025403784439,
1.,0.866025403784439,1.,0.866025403784439,1.,0.866025403784439,1.,0.866025403784439,
1.,0.866025403784439,1.,0.866025403784439,1.,0.866025403784439,1.,0.866025403784439,
1.,0.866025403784439,1.,0.866025403784439,1.,0.866025403784439,1.,0.866025403784439,
1.,0.866025403784439,1.,0.866025403784439,1.,0.866025403784439,1.,0.866025403784439,
1.,0.866025403784439,1.,0.866025403784439,1.,0.866025403784439,1.,0.866025403784439,
1.,0.866025403784439,1.,0.866025403784439,1.,0.866025403784439,1.,0.866025403784439,
1.,0.866025403784439,1.,0.866025403784439,1.,0.866025403784439,1.,0.866025403784439,
1.,0.866025403784439,1.,0.866025403784439,1.,0.866025403784439,1.,0.866025403784439,
1.,0.866025403784439,1.,0.866025403784439,1.,0.866025403784439,1.,0.866025403784439,
1.,0.866025403784439,1.,0.866025403784439,1.,0.866025403784439,1.,0.866025403784439,
1.,0.866025403784439,1.,0.866025403784439,1.,0.866025403784439,1.,0.866025403784439,
1.,0.866025403784439,1.,0.866025403784439,1.,0.866025403784439,1.,0.866025403784439,
1.,0.866025403784439,1.,0.866025403784439,1.,0.866025403784439,1.,0.866025403784439,
1.,0.866025403784439,1.,0.866025403784439,1.,0.866025403784439,1.,0.866025403784439,
1.,0.866025403784439,1.,0.866025403784439,1.,0.866025403784439,1.,0.866025403784439,
1.,0.866025403784439,1.,0.866025403784439,1.,0.866025403784439,1.,0.866025403784439,
1.),(1.,0.866025403784439,1.,0.866025403784439,1.,0.866025403784439,1.,
0.866025403784439,1.,0.866025403784439,1.,0.866025403784439,1.,0.866025403784439,
1.,0.866025403784439,1.,0.866025403784439,1.,0.866025403784439,1.,0.866025403784439,
1.,0.866025403784439,1.,0.866025403784439,1.,0.866025403784439,1.,0.866025403784439,
1.,0.866025403784439,1.,0.866025403784439,1.,0.866025403784439,1.,0.866025403784439,
1.,0.866025403784439,1.,0.866025403784439,1.,0.866025403784439,1.,0.866025403784439,
1.,0.866025403784439,1.,0.866025403784439,1.,0.866025403784439,1.,0.866025403784439,
1.,0.866025403784439,1.,0.866025403784439,1.,0.866025403784439,1.,0.866025403784439,
1.,0.866025403784439,1.,0.866025403784439,1.,0.866025403784439,1.,0.866025403784439,
1.,0.866025403784439,1.,0.866025403784439,1.,0.866025403784439,1.,0.866025403784439,
1.,0.866025403784439,1.,0.866025403784439,1.,0.866025403784439,1.,0.866025403784439,
1.,0.866025403784439,1.,0.866025403784439,1.,0.866025403784439,1.,0.866025403784439,
1.,0.866025403784439,1.,0.866025403784439,1.,0.866025403784439,1.,0.866025403784439,
1.,0.866025403784439,1.,0.866025403784439,1.,0.866025403784439,1.,0.866025403784439,
1.,0.866025403784439,1.,0.866025403784439,1.,0.866025403784439,1.,0.866025403784439,
1.,0.866025403784439,1.,0.866025403784439,1.,0.866025403784439,1.,0.866025403784439,
1.,0.866025403784439,1.,0.866025403784439,1.,0.866025403784439,1.,0.866025403784439,
1.,0.866025403784439,1.,0.866025403784439,1.,0.866025403784439,1.,0.866025403784439,
1.,0.866025403784439,1.,0.866025403784439,1.,0.866025403784439,1.,0.866025403784439,
1.,0.866025403784439,1.,0.866025403784439,1.,0.866025403784439,1.,0.866025403784439,
1.,0.866025403784439,1.,0.866025403784439,1.,0.866025403784439,1.,0.866025403784439,
1.,0.866025403784439,1.,0.866025403784439,1.,0.866025403784439,1.,0.866025403784439,
1.,0.866025403784439,1.,0.866025403784439,1.,0.866025403784439,1.,0.866025403784439,
1.,0.866025403784439,1.,0.866025403784439,1.,0.866025403784439,1.,0.866025403784439,
1.,0.866025403784439,1.,0.866025403784439,1.,0.866025403784439,1.,0.866025403784439,
1.,0.866025403784439,1.,0.866025403784439,1.,0.866025403784439,1.,0.866025403784439,
1.,0.866025403784439,1.,0.866025403784439,1.,0.866025403784439,1.,0.866025403784439,
1.,0.866025403784439,1.,0.866025403784439,1.,0.866025403784439,1.,0.866025403784439,
1.,0.866025403784439,1.,0.866025403784439,1.,0.866025403784439,1.,0.866025403784439,
1.,0.866025403784439,1.,0.866025403784439,1.,0.866025403784439,1.,0.866025403784439,
1.,0.866025403784439,1.,0.866025403784439,1.,0.866025403784439,1.,0.866025403784439,
1.,0.866025403784439,1.,0.866025403784439,1.,0.866025403784439,1.,0.866025403784439,
1.,0.866025403784439,1.,0.866025403784439,1.,0.866025403784439,1.,0.866025403784439,
1.,0.866025403784439,1.,0.866025403784439,1.,0.866025403784439,1.,0.866025403784439,
1.,0.866025403784439,1.,0.866025403784439,1.,0.866025403784439,1.,0.866025403784439,
1.,0.866025403784439,1.,0.866025403784439,1.,0.866025403784439,1.,0.866025403784439,
1.,0.866025403784439,1.,0.866025403784439,1.,0.866025403784439,1.,0.866025403784439,
1.,0.866025403784439,1.,0.866025403784439,1.,0.866025403784439,1.,0.866025403784439,
1.,0.866025403784439,1.,0.866025403784439,1.,0.866025403784439,1.,0.866025403784439,
1.,0.866025403784439,1.,0.866025403784439,1.,0.866025403784439,1.,0.866025403784439,
1.,0.866025403784439,1.,0.866025403784439,1.,0.866025403784439,1.,0.866025403784439,
1.,0.866025403784439,1.,0.866025403784439,1.,0.866025403784439,1.,0.866025403784439,
1.,0.866025403784439,1.,0.866025403784439,1.,0.866025403784439,1.,0.866025403784439,
1.,0.866025403784439,1.,0.866025403784439,1.,0.866025403784439,1.,0.866025403784439,
1.,0.866025403784439,1.,0.866025403784439,1.,0.866025403784439,1.,0.866025403784439,
1.,0.866025403784439,1.,0.866025403784439,1.,0.866025403784439,1.,0.866025403784439,
1.,0.866025403784439,1.,0.866025403784439,1.,0.866025403784439,1.,0.866025403784439,
1.,0.866025403784439,1.,0.866025403784439,1.,0.866025403784439,1.,0.866025403784439,
1.,0.866025403784439,1.,0.866025403784439,1.,0.866025403784439,1.,0.866025403784439,
1.,0.866025403784439,1.,0.866025403784439,1.,0.866025403784439,1.,0.866025403784439,
1.,0.866025403784439,1.,0.866025403784439,1.,0.866025403784439,1.,0.866025403784439,
1.,0.866025403784439,1.,0.866025403784439,1.,0.866025403784439,1.,0.866025403784439,
1.,0.866025403784439,1.,0.866025403784439,1.,0.866025403784439,1.,0.866025403784439,
1.,0.866025403784439,1.,0.866025403784439,1.,0.866025403784439,1.,0.866025403784439,
1.,0.866025403784439,1.,0.866025403784439,1.,0.866025403784439,1.,0.866025403784439,
1.,0.866025403784439,1.,0.866025403784439,1.,0.866025403784439,1.,0.866025403784439,
1.,0.866025403784439,1.,0.866025403784439,1.,0.866025403784439,1.,0.866025403784439,
1.,0.866025403784439,1.,0.866025403784439,1.,0.866025403784439,1.,0.866025403784439,
1.,0.866025403784439,1.,0.866025403784439,1.,0.866025403784439,1.,0.866025403784439,
1.,0.866025403784439,1.,0.866025403784439,1.,0.866025403784439,1.,0.866025403784439,
1.,0.866025403784439,1.,0.866025403784439,1.,0.866025403784439,1.,0.866025403784439,
1.,0.866025403784439,1.,0.866025403784439,1.,0.866025403784439,1.,0.866025403784439,
1.,0.866025403784439,1.,0.866025403784439,1.,0.866025403784439,1.,0.866025403784439,
1.,0.866025403784439,1.,0.866025403784439,1.,0.866025403784439,1.,0.866025403784439,
1.,0.866025403784439,1.,0.866025403784439,1.,0.866025403784439,1.,0.866025403784439,
1.,0.866025403784439,1.,0.866025403784439,1.,0.866025403784439,1.,0.866025403784439,
1.,0.866025403784439,1.,0.866025403784439,1.,0.866025403784439,1.,0.866025403784439,
1.,0.866025403784439,1.,0.866025403784439,1.,0.866025403784439,1.,0.866025403784439,
1.,0.866025403784439,1.,0.866025403784439,1.,0.866025403784439,1.,0.866025403784439,
1.,0.866025403784439,1.,0.866025403784439,1.,0.866025403784439,1.,0.866025403784439,
1.,0.866025403784439,1.,0.866025403784439,1.,0.866025403784439,1.,0.866025403784439,
1.,0.866025403784439,1.,0.866025403784439,1.,0.866025403784439,1.,0.866025403784439,
1.,0.866025403784439,1.,0.866025403784439,1.,0.866025403784439,1.,0.866025403784439,
1.,0.866025403784439,1.,0.866025403784439,1.,0.866025403784439,1.,0.866025403784439,
1.,0.866025403784439,1.,0.866025403784439,1.,0.866025403784439,1.,0.866025403784439,
1.,0.866025403784439,1.,0.866025403784439,1.,0.866025403784439,1.,0.866025403784439,
1.,0.866025403784439,1.,0.866025403784439,1.,0.866025403784439,1.,0.866025403784439,
1.,0.866025403784439,1.,0.866025403784439,1.,0.866025403784439,1.,0.866025403784439,
1.,0.866025403784439,1.,0.866025403784439,1.,0.866025403784439,1.,0.866025403784439,
1.,0.866025403784439,1.,0.866025403784439,1.,0.866025403784439,1.,0.866025403784439,
1.,0.866025403784439,1.,0.866025403784439,1.,0.866025403784439,1.,0.866025403784439,
1.,0.866025403784439,1.,0.866025403784439,1.,0.866025403784439,1.,0.866025403784439,
1.,0.866025403784439,1.,0.866025403784439,1.,0.866025403784439,1.,0.866025403784439,
1.,0.866025403784439,1.,0.866025403784439,1.,0.866025403784439,1.,0.866025403784439,
1.,0.866025403784439,1.,0.866025403784439,1.,0.866025403784439,1.,0.866025403784439,
1.,0.866025403784439,1.,0.866025403784439,1.,0.866025403784439,1.,0.866025403784439,
1.,0.866025403784439,1.,0.866025403784439,1.,0.866025403784439,1.,0.866025403784439,
1.,0.866025403784439,1.,0.866025403784439,1.,0.866025403784439,1.,0.866025403784439,
1.,0.866025403784439,1.,0.866025403784439,1.,0.866025403784439,1.,0.866025403784439,
1.,0.866025403784439,1.,0.866025403784439,1.,0.866025403784439,1.,0.866025403784439,
1.,0.866025403784439,1.,0.866025403784439,1.,0.866025403784439,1.,0.866025403784439,
1.,0.866025403784439,1.,0.866025403784439,1.,0.866025403784439,1.,0.866025403784439,
1.,0.866025403784439,1.,0.866025403784439,1.,0.866025403784439,1.,0.866025403784439,
1.,0.866025403784439,1.,0.866025403784439,1.,0.866025403784439,1.,0.866025403784439,
1.,0.866025403784439,1.,0.866025403784439,1.,0.866025403784439,1.,0.866025403784439,
1.,0.866025403784439,1.,0.866025403784439,1.,0.866025403784439,1.,0.866025403784439,
1.,0.866025403784439,1.,0.866025403784439,1.,0.866025403784439,1.,0.866025403784439,
1.,0.866025403784439,1.,0.866025403784439,1.,0.866025403784439,1.,0.866025403784439,
1.,0.866025403784439,1.,0.866025403784439,1.,0.866025403784439,1.,0.866025403784439,
1.,0.866025403784439,1.,0.866025403784439,1.,0.866025403784439,1.,0.866025403784439,
1.,0.866025403784439,1.,0.866025403784439,1.,0.866025403784439,1.,0.866025403784439,
1.,0.866025403784439,1.,0.866025403784439,1.,0.866025403784439,1.,0.866025403784439,
1.,0.866025403784439,1.,0.866025403784439,1.,0.866025403784439,1.,0.866025403784439,
1.,0.866025403784439,1.,0.866025403784439,1.,0.866025403784439,1.,0.866025403784439,
1.,0.866025403784439,1.,0.866025403784439,1.,0.866025403784439,1.,0.866025403784439,
1.,0.866025403784439,1.,0.866025403784439,1.,0.866025403784439,1.,0.866025403784439,
1.,0.866025403784439,1.,0.866025403784439,1.,0.866025403784439,1.,0.866025403784439,
1.,0.866025403784439,1.,0.866025403784439,1.,0.866025403784439,1.,0.866025403784439,
1.,0.866025403784439,1.,0.866025403784439,1.,0.866025403784439,1.,0.866025403784439,
1.,0.866025403784439,1.,0.866025403784439,1.,0.866025403784439,1.,0.866025403784439,
1.,0.866025403784439,1.,0.866025403784439,1.,0.866025403784439,1.,0.866025403784439,
1.,0.866025403784439,1.,0.866025403784439,1.,0.866025403784439,1.,0.866025403784439,
1.,0.866025403784439,1.,0.866025403784439,1.,0.866025403784439,1.,0.866025403784439,
1.,0.866025403784439,1.,0.866025403784439,1.,0.866025403784439,1.,0.866025403784439,
1.,0.866025403784439,1.,0.866025403784439,1.,0.866025403784439,1.,0.866025403784439,
1.,0.866025403784439,1.,0.866025403784439,1.,0.866025403784439,1.,0.866025403784439,
1.,0.866025403784439,1.,0.866025403784439,1.,0.866025403784439,1.,0.866025403784439,
1.,0.866025403784439,1.,0.866025403784439,1.,0.866025403784439,1.,0.866025403784439,
1.,0.866025403784439,1.,0.866025403784439,1.,0.866025403784439,1.,0.866025403784439,
1.,0.866025403784439,1.,0.866025403784439,1.,0.866025403784439,1.,0.866025403784439,
1.,0.866025403784439,1.,0.866025403784439,1.,0.866025403784439,1.,0.866025403784439,
1.,0.866025403784439,1.,0.866025403784439,1.,0.866025403784439,1.)))
REPRESENTATION_ITEM('')
SURFACE()
);
#149=(
BOUNDED_SURFACE()
B_SPLINE_SURFACE(3,2,((#15547,#15548,#15549,#15550,#15551,#15552,#15553,
#15554,#15555,#15556,#15557,#15558,#15559,#15560,#15561,#15562,#15563,#15564,
#15565,#15566,#15567,#15568,#15569,#15570,#15571,#15572,#15573,#15574,#15575,
#15576,#15577,#15578,#15579,#15580,#15581,#15582,#15583,#15584,#15585,#15586,
#15587,#15588,#15589,#15590,#15591,#15592,#15593,#15594,#15595,#15596,#15597,
#15598,#15599,#15600,#15601,#15602,#15603,#15604,#15605,#15606,#15607,#15608,
#15609,#15610,#15611,#15612,#15613,#15614,#15615,#15616,#15617,#15618,#15619,
#15620,#15621,#15622,#15623,#15624,#15625,#15626,#15627,#15628,#15629,#15630,
#15631,#15632,#15633,#15634,#15635,#15636,#15637,#15638,#15639,#15640,#15641,
#15642,#15643,#15644,#15645,#15646,#15647,#15648,#15649,#15650,#15651,#15652,
#15653,#15654,#15655,#15656,#15657,#15658,#15659,#15660,#15661,#15662,#15663,
#15664,#15665,#15666,#15667,#15668,#15669,#15670,#15671,#15672,#15673,#15674,
#15675,#15676,#15677,#15678,#15679,#15680,#15681,#15682,#15683,#15684,#15685,
#15686,#15687,#15688,#15689,#15690,#15691,#15692,#15693,#15694,#15695,#15696,
#15697,#15698,#15699,#15700,#15701,#15702,#15703,#15704,#15705,#15706,#15707,
#15708,#15709,#15710,#15711,#15712,#15713,#15714,#15715,#15716,#15717,#15718,
#15719,#15720,#15721,#15722,#15723,#15724,#15725,#15726,#15727,#15728,#15729,
#15730,#15731,#15732,#15733,#15734,#15735,#15736,#15737,#15738,#15739,#15740,
#15741,#15742,#15743,#15744,#15745,#15746,#15747,#15748,#15749,#15750,#15751,
#15752,#15753,#15754,#15755,#15756,#15757,#15758,#15759,#15760,#15761,#15762,
#15763,#15764,#15765,#15766,#15767,#15768,#15769,#15770,#15771,#15772,#15773,
#15774,#15775,#15776,#15777,#15778,#15779,#15780,#15781,#15782,#15783,#15784,
#15785,#15786,#15787,#15788,#15789,#15790,#15791,#15792,#15793,#15794,#15795,
#15796,#15797,#15798,#15799,#15800,#15801,#15802,#15803,#15804,#15805,#15806,
#15807,#15808,#15809,#15810,#15811,#15812,#15813,#15814,#15815,#15816,#15817,
#15818,#15819,#15820,#15821,#15822,#15823,#15824,#15825,#15826,#15827,#15828,
#15829,#15830,#15831,#15832,#15833,#15834,#15835,#15836,#15837,#15838,#15839,
#15840,#15841,#15842,#15843,#15844,#15845,#15846,#15847,#15848,#15849,#15850,
#15851,#15852,#15853,#15854,#15855,#15856,#15857,#15858,#15859,#15860,#15861,
#15862,#15863,#15864,#15865,#15866,#15867,#15868,#15869,#15870,#15871,#15872,
#15873,#15874,#15875,#15876,#15877,#15878,#15879,#15880,#15881,#15882,#15883,
#15884,#15885,#15886,#15887,#15888,#15889,#15890,#15891,#15892,#15893,#15894,
#15895,#15896,#15897,#15898,#15899,#15900,#15901,#15902,#15903,#15904,#15905,
#15906,#15907,#15908,#15909,#15910,#15911,#15912,#15913,#15914,#15915,#15916,
#15917,#15918,#15919,#15920,#15921,#15922,#15923,#15924,#15925,#15926,#15927,
#15928,#15929,#15930,#15931,#15932,#15933,#15934,#15935,#15936,#15937,#15938,
#15939,#15940,#15941,#15942,#15943,#15944,#15945,#15946,#15947,#15948,#15949,
#15950,#15951,#15952,#15953,#15954,#15955,#15956,#15957,#15958,#15959,#15960,
#15961,#15962,#15963,#15964,#15965,#15966,#15967,#15968,#15969,#15970,#15971,
#15972,#15973,#15974,#15975,#15976,#15977,#15978,#15979,#15980,#15981,#15982,
#15983,#15984,#15985,#15986,#15987,#15988,#15989,#15990,#15991,#15992,#15993,
#15994,#15995,#15996,#15997,#15998,#15999,#16000,#16001,#16002,#16003,#16004,
#16005,#16006,#16007,#16008,#16009,#16010,#16011,#16012,#16013,#16014,#16015,
#16016,#16017,#16018,#16019,#16020,#16021,#16022,#16023,#16024,#16025,#16026,
#16027,#16028,#16029,#16030,#16031,#16032,#16033,#16034,#16035,#16036,#16037,
#16038,#16039,#16040,#16041,#16042,#16043,#16044,#16045,#16046,#16047,#16048,
#16049,#16050,#16051,#16052,#16053,#16054,#16055,#16056,#16057,#16058,#16059,
#16060,#16061,#16062,#16063,#16064,#16065,#16066,#16067,#16068,#16069,#16070,
#16071,#16072,#16073,#16074,#16075,#16076,#16077,#16078,#16079,#16080,#16081,
#16082,#16083,#16084,#16085,#16086,#16087,#16088,#16089,#16090,#16091,#16092,
#16093,#16094,#16095,#16096,#16097,#16098,#16099,#16100,#16101,#16102,#16103,
#16104,#16105,#16106,#16107,#16108,#16109,#16110,#16111,#16112,#16113,#16114,
#16115,#16116,#16117,#16118,#16119,#16120,#16121,#16122,#16123,#16124,#16125,
#16126,#16127,#16128,#16129,#16130,#16131,#16132,#16133,#16134,#16135,#16136,
#16137,#16138,#16139,#16140,#16141,#16142,#16143,#16144,#16145,#16146,#16147,
#16148,#16149,#16150,#16151,#16152,#16153,#16154,#16155,#16156,#16157,#16158,
#16159,#16160,#16161,#16162,#16163,#16164,#16165,#16166,#16167,#16168,#16169,
#16170,#16171,#16172,#16173,#16174,#16175,#16176,#16177,#16178,#16179,#16180,
#16181,#16182,#16183,#16184,#16185,#16186,#16187,#16188,#16189,#16190,#16191,
#16192,#16193,#16194,#16195,#16196,#16197,#16198,#16199,#16200,#16201,#16202,
#16203,#16204,#16205,#16206,#16207,#16208,#16209,#16210,#16211,#16212,#16213,
#16214,#16215,#16216,#16217,#16218,#16219,#16220,#16221,#16222,#16223,#16224,
#16225,#16226,#16227,#16228,#16229,#16230,#16231,#16232,#16233,#16234,#16235,
#16236,#16237,#16238,#16239,#16240,#16241,#16242,#16243,#16244,#16245,#16246,
#16247,#16248,#16249,#16250,#16251,#16252,#16253,#16254,#16255,#16256,#16257,
#16258,#16259,#16260,#16261,#16262,#16263,#16264,#16265,#16266,#16267,#16268,
#16269,#16270,#16271,#16272,#16273,#16274,#16275,#16276,#16277,#16278,#16279,
#16280,#16281,#16282,#16283,#16284,#16285,#16286,#16287,#16288,#16289,#16290,
#16291,#16292,#16293,#16294,#16295,#16296,#16297,#16298,#16299,#16300,#16301,
#16302,#16303,#16304,#16305,#16306,#16307,#16308,#16309,#16310,#16311,#16312,
#16313,#16314,#16315,#16316,#16317,#16318,#16319,#16320,#16321,#16322,#16323,
#16324,#16325,#16326,#16327,#16328,#16329,#16330,#16331,#16332,#16333,#16334,
#16335,#16336,#16337,#16338,#16339,#16340,#16341,#16342,#16343,#16344,#16345,
#16346,#16347,#16348,#16349,#16350,#16351,#16352,#16353,#16354,#16355,#16356,
#16357,#16358,#16359,#16360,#16361,#16362,#16363,#16364,#16365,#16366,#16367,
#16368,#16369,#16370,#16371,#16372,#16373,#16374,#16375,#16376,#16377,#16378,
#16379,#16380,#16381,#16382,#16383,#16384,#16385,#16386,#16387,#16388,#16389,
#16390,#16391,#16392,#16393,#16394,#16395,#16396,#16397,#16398,#16399,#16400,
#16401,#16402,#16403,#16404,#16405,#16406,#16407,#16408,#16409,#16410,#16411,
#16412,#16413,#16414,#16415,#16416,#16417,#16418,#16419,#16420,#16421,#16422,
#16423,#16424,#16425,#16426,#16427,#16428,#16429,#16430,#16431,#16432,#16433,
#16434,#16435,#16436,#16437,#16438,#16439,#16440,#16441,#16442,#16443,#16444,
#16445,#16446,#16447,#16448,#16449,#16450,#16451,#16452,#16453,#16454,#16455,
#16456,#16457,#16458,#16459,#16460,#16461,#16462,#16463,#16464,#16465,#16466,
#16467,#16468,#16469,#16470,#16471,#16472,#16473,#16474,#16475,#16476,#16477,
#16478,#16479,#16480,#16481,#16482,#16483,#16484,#16485,#16486,#16487,#16488,
#16489,#16490,#16491,#16492,#16493,#16494,#16495,#16496,#16497,#16498,#16499,
#16500,#16501,#16502,#16503,#16504,#16505,#16506,#16507,#16508,#16509,#16510,
#16511,#16512,#16513,#16514,#16515,#16516,#16517,#16518,#16519),(#16520,
#16521,#16522,#16523,#16524,#16525,#16526,#16527,#16528,#16529,#16530,#16531,
#16532,#16533,#16534,#16535,#16536,#16537,#16538,#16539,#16540,#16541,#16542,
#16543,#16544,#16545,#16546,#16547,#16548,#16549,#16550,#16551,#16552,#16553,
#16554,#16555,#16556,#16557,#16558,#16559,#16560,#16561,#16562,#16563,#16564,
#16565,#16566,#16567,#16568,#16569,#16570,#16571,#16572,#16573,#16574,#16575,
#16576,#16577,#16578,#16579,#16580,#16581,#16582,#16583,#16584,#16585,#16586,
#16587,#16588,#16589,#16590,#16591,#16592,#16593,#16594,#16595,#16596,#16597,
#16598,#16599,#16600,#16601,#16602,#16603,#16604,#16605,#16606,#16607,#16608,
#16609,#16610,#16611,#16612,#16613,#16614,#16615,#16616,#16617,#16618,#16619,
#16620,#16621,#16622,#16623,#16624,#16625,#16626,#16627,#16628,#16629,#16630,
#16631,#16632,#16633,#16634,#16635,#16636,#16637,#16638,#16639,#16640,#16641,
#16642,#16643,#16644,#16645,#16646,#16647,#16648,#16649,#16650,#16651,#16652,
#16653,#16654,#16655,#16656,#16657,#16658,#16659,#16660,#16661,#16662,#16663,
#16664,#16665,#16666,#16667,#16668,#16669,#16670,#16671,#16672,#16673,#16674,
#16675,#16676,#16677,#16678,#16679,#16680,#16681,#16682,#16683,#16684,#16685,
#16686,#16687,#16688,#16689,#16690,#16691,#16692,#16693,#16694,#16695,#16696,
#16697,#16698,#16699,#16700,#16701,#16702,#16703,#16704,#16705,#16706,#16707,
#16708,#16709,#16710,#16711,#16712,#16713,#16714,#16715,#16716,#16717,#16718,
#16719,#16720,#16721,#16722,#16723,#16724,#16725,#16726,#16727,#16728,#16729,
#16730,#16731,#16732,#16733,#16734,#16735,#16736,#16737,#16738,#16739,#16740,
#16741,#16742,#16743,#16744,#16745,#16746,#16747,#16748,#16749,#16750,#16751,
#16752,#16753,#16754,#16755,#16756,#16757,#16758,#16759,#16760,#16761,#16762,
#16763,#16764,#16765,#16766,#16767,#16768,#16769,#16770,#16771,#16772,#16773,
#16774,#16775,#16776,#16777,#16778,#16779,#16780,#16781,#16782,#16783,#16784,
#16785,#16786,#16787,#16788,#16789,#16790,#16791,#16792,#16793,#16794,#16795,
#16796,#16797,#16798,#16799,#16800,#16801,#16802,#16803,#16804,#16805,#16806,
#16807,#16808,#16809,#16810,#16811,#16812,#16813,#16814,#16815,#16816,#16817,
#16818,#16819,#16820,#16821,#16822,#16823,#16824,#16825,#16826,#16827,#16828,
#16829,#16830,#16831,#16832,#16833,#16834,#16835,#16836,#16837,#16838,#16839,
#16840,#16841,#16842,#16843,#16844,#16845,#16846,#16847,#16848,#16849,#16850,
#16851,#16852,#16853,#16854,#16855,#16856,#16857,#16858,#16859,#16860,#16861,
#16862,#16863,#16864,#16865,#16866,#16867,#16868,#16869,#16870,#16871,#16872,
#16873,#16874,#16875,#16876,#16877,#16878,#16879,#16880,#16881,#16882,#16883,
#16884,#16885,#16886,#16887,#16888,#16889,#16890,#16891,#16892,#16893,#16894,
#16895,#16896,#16897,#16898,#16899,#16900,#16901,#16902,#16903,#16904,#16905,
#16906,#16907,#16908,#16909,#16910,#16911,#16912,#16913,#16914,#16915,#16916,
#16917,#16918,#16919,#16920,#16921,#16922,#16923,#16924,#16925,#16926,#16927,
#16928,#16929,#16930,#16931,#16932,#16933,#16934,#16935,#16936,#16937,#16938,
#16939,#16940,#16941,#16942,#16943,#16944,#16945,#16946,#16947,#16948,#16949,
#16950,#16951,#16952,#16953,#16954,#16955,#16956,#16957,#16958,#16959,#16960,
#16961,#16962,#16963,#16964,#16965,#16966,#16967,#16968,#16969,#16970,#16971,
#16972,#16973,#16974,#16975,#16976,#16977,#16978,#16979,#16980,#16981,#16982,
#16983,#16984,#16985,#16986,#16987,#16988,#16989,#16990,#16991,#16992,#16993,
#16994,#16995,#16996,#16997,#16998,#16999,#17000,#17001,#17002,#17003,#17004,
#17005,#17006,#17007,#17008,#17009,#17010,#17011,#17012,#17013,#17014,#17015,
#17016,#17017,#17018,#17019,#17020,#17021,#17022,#17023,#17024,#17025,#17026,
#17027,#17028,#17029,#17030,#17031,#17032,#17033,#17034,#17035,#17036,#17037,
#17038,#17039,#17040,#17041,#17042,#17043,#17044,#17045,#17046,#17047,#17048,
#17049,#17050,#17051,#17052,#17053,#17054,#17055,#17056,#17057,#17058,#17059,
#17060,#17061,#17062,#17063,#17064,#17065,#17066,#17067,#17068,#17069,#17070,
#17071,#17072,#17073,#17074,#17075,#17076,#17077,#17078,#17079,#17080,#17081,
#17082,#17083,#17084,#17085,#17086,#17087,#17088,#17089,#17090,#17091,#17092,
#17093,#17094,#17095,#17096,#17097,#17098,#17099,#17100,#17101,#17102,#17103,
#17104,#17105,#17106,#17107,#17108,#17109,#17110,#17111,#17112,#17113,#17114,
#17115,#17116,#17117,#17118,#17119,#17120,#17121,#17122,#17123,#17124,#17125,
#17126,#17127,#17128,#17129,#17130,#17131,#17132,#17133,#17134,#17135,#17136,
#17137,#17138,#17139,#17140,#17141,#17142,#17143,#17144,#17145,#17146,#17147,
#17148,#17149,#17150,#17151,#17152,#17153,#17154,#17155,#17156,#17157,#17158,
#17159,#17160,#17161,#17162,#17163,#17164,#17165,#17166,#17167,#17168,#17169,
#17170,#17171,#17172,#17173,#17174,#17175,#17176,#17177,#17178,#17179,#17180,
#17181,#17182,#17183,#17184,#17185,#17186,#17187,#17188,#17189,#17190,#17191,
#17192,#17193,#17194,#17195,#17196,#17197,#17198,#17199,#17200,#17201,#17202,
#17203,#17204,#17205,#17206,#17207,#17208,#17209,#17210,#17211,#17212,#17213,
#17214,#17215,#17216,#17217,#17218,#17219,#17220,#17221,#17222,#17223,#17224,
#17225,#17226,#17227,#17228,#17229,#17230,#17231,#17232,#17233,#17234,#17235,
#17236,#17237,#17238,#17239,#17240,#17241,#17242,#17243,#17244,#17245,#17246,
#17247,#17248,#17249,#17250,#17251,#17252,#17253,#17254,#17255,#17256,#17257,
#17258,#17259,#17260,#17261,#17262,#17263,#17264,#17265,#17266,#17267,#17268,
#17269,#17270,#17271,#17272,#17273,#17274,#17275,#17276,#17277,#17278,#17279,
#17280,#17281,#17282,#17283,#17284,#17285,#17286,#17287,#17288,#17289,#17290,
#17291,#17292,#17293,#17294,#17295,#17296,#17297,#17298,#17299,#17300,#17301,
#17302,#17303,#17304,#17305,#17306,#17307,#17308,#17309,#17310,#17311,#17312,
#17313,#17314,#17315,#17316,#17317,#17318,#17319,#17320,#17321,#17322,#17323,
#17324,#17325,#17326,#17327,#17328,#17329,#17330,#17331,#17332,#17333,#17334,
#17335,#17336,#17337,#17338,#17339,#17340,#17341,#17342,#17343,#17344,#17345,
#17346,#17347,#17348,#17349,#17350,#17351,#17352,#17353,#17354,#17355,#17356,
#17357,#17358,#17359,#17360,#17361,#17362,#17363,#17364,#17365,#17366,#17367,
#17368,#17369,#17370,#17371,#17372,#17373,#17374,#17375,#17376,#17377,#17378,
#17379,#17380,#17381,#17382,#17383,#17384,#17385,#17386,#17387,#17388,#17389,
#17390,#17391,#17392,#17393,#17394,#17395,#17396,#17397,#17398,#17399,#17400,
#17401,#17402,#17403,#17404,#17405,#17406,#17407,#17408,#17409,#17410,#17411,
#17412,#17413,#17414,#17415,#17416,#17417,#17418,#17419,#17420,#17421,#17422,
#17423,#17424,#17425,#17426,#17427,#17428,#17429,#17430,#17431,#17432,#17433,
#17434,#17435,#17436,#17437,#17438,#17439,#17440,#17441,#17442,#17443,#17444,
#17445,#17446,#17447,#17448,#17449,#17450,#17451,#17452,#17453,#17454,#17455,
#17456,#17457,#17458,#17459,#17460,#17461,#17462,#17463,#17464,#17465,#17466,
#17467,#17468,#17469,#17470,#17471,#17472,#17473,#17474,#17475,#17476,#17477,
#17478,#17479,#17480,#17481,#17482,#17483,#17484,#17485,#17486,#17487,#17488,
#17489,#17490,#17491,#17492),(#17493,#17494,#17495,#17496,#17497,#17498,
#17499,#17500,#17501,#17502,#17503,#17504,#17505,#17506,#17507,#17508,#17509,
#17510,#17511,#17512,#17513,#17514,#17515,#17516,#17517,#17518,#17519,#17520,
#17521,#17522,#17523,#17524,#17525,#17526,#17527,#17528,#17529,#17530,#17531,
#17532,#17533,#17534,#17535,#17536,#17537,#17538,#17539,#17540,#17541,#17542,
#17543,#17544,#17545,#17546,#17547,#17548,#17549,#17550,#17551,#17552,#17553,
#17554,#17555,#17556,#17557,#17558,#17559,#17560,#17561,#17562,#17563,#17564,
#17565,#17566,#17567,#17568,#17569,#17570,#17571,#17572,#17573,#17574,#17575,
#17576,#17577,#17578,#17579,#17580,#17581,#17582,#17583,#17584,#17585,#17586,
#17587,#17588,#17589,#17590,#17591,#17592,#17593,#17594,#17595,#17596,#17597,
#17598,#17599,#17600,#17601,#17602,#17603,#17604,#17605,#17606,#17607,#17608,
#17609,#17610,#17611,#17612,#17613,#17614,#17615,#17616,#17617,#17618,#17619,
#17620,#17621,#17622,#17623,#17624,#17625,#17626,#17627,#17628,#17629,#17630,
#17631,#17632,#17633,#17634,#17635,#17636,#17637,#17638,#17639,#17640,#17641,
#17642,#17643,#17644,#17645,#17646,#17647,#17648,#17649,#17650,#17651,#17652,
#17653,#17654,#17655,#17656,#17657,#17658,#17659,#17660,#17661,#17662,#17663,
#17664,#17665,#17666,#17667,#17668,#17669,#17670,#17671,#17672,#17673,#17674,
#17675,#17676,#17677,#17678,#17679,#17680,#17681,#17682,#17683,#17684,#17685,
#17686,#17687,#17688,#17689,#17690,#17691,#17692,#17693,#17694,#17695,#17696,
#17697,#17698,#17699,#17700,#17701,#17702,#17703,#17704,#17705,#17706,#17707,
#17708,#17709,#17710,#17711,#17712,#17713,#17714,#17715,#17716,#17717,#17718,
#17719,#17720,#17721,#17722,#17723,#17724,#17725,#17726,#17727,#17728,#17729,
#17730,#17731,#17732,#17733,#17734,#17735,#17736,#17737,#17738,#17739,#17740,
#17741,#17742,#17743,#17744,#17745,#17746,#17747,#17748,#17749,#17750,#17751,
#17752,#17753,#17754,#17755,#17756,#17757,#17758,#17759,#17760,#17761,#17762,
#17763,#17764,#17765,#17766,#17767,#17768,#17769,#17770,#17771,#17772,#17773,
#17774,#17775,#17776,#17777,#17778,#17779,#17780,#17781,#17782,#17783,#17784,
#17785,#17786,#17787,#17788,#17789,#17790,#17791,#17792,#17793,#17794,#17795,
#17796,#17797,#17798,#17799,#17800,#17801,#17802,#17803,#17804,#17805,#17806,
#17807,#17808,#17809,#17810,#17811,#17812,#17813,#17814,#17815,#17816,#17817,
#17818,#17819,#17820,#17821,#17822,#17823,#17824,#17825,#17826,#17827,#17828,
#17829,#17830,#17831,#17832,#17833,#17834,#17835,#17836,#17837,#17838,#17839,
#17840,#17841,#17842,#17843,#17844,#17845,#17846,#17847,#17848,#17849,#17850,
#17851,#17852,#17853,#17854,#17855,#17856,#17857,#17858,#17859,#17860,#17861,
#17862,#17863,#17864,#17865,#17866,#17867,#17868,#17869,#17870,#17871,#17872,
#17873,#17874,#17875,#17876,#17877,#17878,#17879,#17880,#17881,#17882,#17883,
#17884,#17885,#17886,#17887,#17888,#17889,#17890,#17891,#17892,#17893,#17894,
#17895,#17896,#17897,#17898,#17899,#17900,#17901,#17902,#17903,#17904,#17905,
#17906,#17907,#17908,#17909,#17910,#17911,#17912,#17913,#17914,#17915,#17916,
#17917,#17918,#17919,#17920,#17921,#17922,#17923,#17924,#17925,#17926,#17927,
#17928,#17929,#17930,#17931,#17932,#17933,#17934,#17935,#17936,#17937,#17938,
#17939,#17940,#17941,#17942,#17943,#17944,#17945,#17946,#17947,#17948,#17949,
#17950,#17951,#17952,#17953,#17954,#17955,#17956,#17957,#17958,#17959,#17960,
#17961,#17962,#17963,#17964,#17965,#17966,#17967,#17968,#17969,#17970,#17971,
#17972,#17973,#17974,#17975,#17976,#17977,#17978,#17979,#17980,#17981,#17982,
#17983,#17984,#17985,#17986,#17987,#17988,#17989,#17990,#17991,#17992,#17993,
#17994,#17995,#17996,#17997,#17998,#17999,#18000,#18001,#18002,#18003,#18004,
#18005,#18006,#18007,#18008,#18009,#18010,#18011,#18012,#18013,#18014,#18015,
#18016,#18017,#18018,#18019,#18020,#18021,#18022,#18023,#18024,#18025,#18026,
#18027,#18028,#18029,#18030,#18031,#18032,#18033,#18034,#18035,#18036,#18037,
#18038,#18039,#18040,#18041,#18042,#18043,#18044,#18045,#18046,#18047,#18048,
#18049,#18050,#18051,#18052,#18053,#18054,#18055,#18056,#18057,#18058,#18059,
#18060,#18061,#18062,#18063,#18064,#18065,#18066,#18067,#18068,#18069,#18070,
#18071,#18072,#18073,#18074,#18075,#18076,#18077,#18078,#18079,#18080,#18081,
#18082,#18083,#18084,#18085,#18086,#18087,#18088,#18089,#18090,#18091,#18092,
#18093,#18094,#18095,#18096,#18097,#18098,#18099,#18100,#18101,#18102,#18103,
#18104,#18105,#18106,#18107,#18108,#18109,#18110,#18111,#18112,#18113,#18114,
#18115,#18116,#18117,#18118,#18119,#18120,#18121,#18122,#18123,#18124,#18125,
#18126,#18127,#18128,#18129,#18130,#18131,#18132,#18133,#18134,#18135,#18136,
#18137,#18138,#18139,#18140,#18141,#18142,#18143,#18144,#18145,#18146,#18147,
#18148,#18149,#18150,#18151,#18152,#18153,#18154,#18155,#18156,#18157,#18158,
#18159,#18160,#18161,#18162,#18163,#18164,#18165,#18166,#18167,#18168,#18169,
#18170,#18171,#18172,#18173,#18174,#18175,#18176,#18177,#18178,#18179,#18180,
#18181,#18182,#18183,#18184,#18185,#18186,#18187,#18188,#18189,#18190,#18191,
#18192,#18193,#18194,#18195,#18196,#18197,#18198,#18199,#18200,#18201,#18202,
#18203,#18204,#18205,#18206,#18207,#18208,#18209,#18210,#18211,#18212,#18213,
#18214,#18215,#18216,#18217,#18218,#18219,#18220,#18221,#18222,#18223,#18224,
#18225,#18226,#18227,#18228,#18229,#18230,#18231,#18232,#18233,#18234,#18235,
#18236,#18237,#18238,#18239,#18240,#18241,#18242,#18243,#18244,#18245,#18246,
#18247,#18248,#18249,#18250,#18251,#18252,#18253,#18254,#18255,#18256,#18257,
#18258,#18259,#18260,#18261,#18262,#18263,#18264,#18265,#18266,#18267,#18268,
#18269,#18270,#18271,#18272,#18273,#18274,#18275,#18276,#18277,#18278,#18279,
#18280,#18281,#18282,#18283,#18284,#18285,#18286,#18287,#18288,#18289,#18290,
#18291,#18292,#18293,#18294,#18295,#18296,#18297,#18298,#18299,#18300,#18301,
#18302,#18303,#18304,#18305,#18306,#18307,#18308,#18309,#18310,#18311,#18312,
#18313,#18314,#18315,#18316,#18317,#18318,#18319,#18320,#18321,#18322,#18323,
#18324,#18325,#18326,#18327,#18328,#18329,#18330,#18331,#18332,#18333,#18334,
#18335,#18336,#18337,#18338,#18339,#18340,#18341,#18342,#18343,#18344,#18345,
#18346,#18347,#18348,#18349,#18350,#18351,#18352,#18353,#18354,#18355,#18356,
#18357,#18358,#18359,#18360,#18361,#18362,#18363,#18364,#18365,#18366,#18367,
#18368,#18369,#18370,#18371,#18372,#18373,#18374,#18375,#18376,#18377,#18378,
#18379,#18380,#18381,#18382,#18383,#18384,#18385,#18386,#18387,#18388,#18389,
#18390,#18391,#18392,#18393,#18394,#18395,#18396,#18397,#18398,#18399,#18400,
#18401,#18402,#18403,#18404,#18405,#18406,#18407,#18408,#18409,#18410,#18411,
#18412,#18413,#18414,#18415,#18416,#18417,#18418,#18419,#18420,#18421,#18422,
#18423,#18424,#18425,#18426,#18427,#18428,#18429,#18430,#18431,#18432,#18433,
#18434,#18435,#18436,#18437,#18438,#18439,#18440,#18441,#18442,#18443,#18444,
#18445,#18446,#18447,#18448,#18449,#18450,#18451,#18452,#18453,#18454,#18455,
#18456,#18457,#18458,#18459,#18460,#18461,#18462,#18463,#18464,#18465),
(#18466,#18467,#18468,#18469,#18470,#18471,#18472,#18473,#18474,#18475,
#18476,#18477,#18478,#18479,#18480,#18481,#18482,#18483,#18484,#18485,#18486,
#18487,#18488,#18489,#18490,#18491,#18492,#18493,#18494,#18495,#18496,#18497,
#18498,#18499,#18500,#18501,#18502,#18503,#18504,#18505,#18506,#18507,#18508,
#18509,#18510,#18511,#18512,#18513,#18514,#18515,#18516,#18517,#18518,#18519,
#18520,#18521,#18522,#18523,#18524,#18525,#18526,#18527,#18528,#18529,#18530,
#18531,#18532,#18533,#18534,#18535,#18536,#18537,#18538,#18539,#18540,#18541,
#18542,#18543,#18544,#18545,#18546,#18547,#18548,#18549,#18550,#18551,#18552,
#18553,#18554,#18555,#18556,#18557,#18558,#18559,#18560,#18561,#18562,#18563,
#18564,#18565,#18566,#18567,#18568,#18569,#18570,#18571,#18572,#18573,#18574,
#18575,#18576,#18577,#18578,#18579,#18580,#18581,#18582,#18583,#18584,#18585,
#18586,#18587,#18588,#18589,#18590,#18591,#18592,#18593,#18594,#18595,#18596,
#18597,#18598,#18599,#18600,#18601,#18602,#18603,#18604,#18605,#18606,#18607,
#18608,#18609,#18610,#18611,#18612,#18613,#18614,#18615,#18616,#18617,#18618,
#18619,#18620,#18621,#18622,#18623,#18624,#18625,#18626,#18627,#18628,#18629,
#18630,#18631,#18632,#18633,#18634,#18635,#18636,#18637,#18638,#18639,#18640,
#18641,#18642,#18643,#18644,#18645,#18646,#18647,#18648,#18649,#18650,#18651,
#18652,#18653,#18654,#18655,#18656,#18657,#18658,#18659,#18660,#18661,#18662,
#18663,#18664,#18665,#18666,#18667,#18668,#18669,#18670,#18671,#18672,#18673,
#18674,#18675,#18676,#18677,#18678,#18679,#18680,#18681,#18682,#18683,#18684,
#18685,#18686,#18687,#18688,#18689,#18690,#18691,#18692,#18693,#18694,#18695,
#18696,#18697,#18698,#18699,#18700,#18701,#18702,#18703,#18704,#18705,#18706,
#18707,#18708,#18709,#18710,#18711,#18712,#18713,#18714,#18715,#18716,#18717,
#18718,#18719,#18720,#18721,#18722,#18723,#18724,#18725,#18726,#18727,#18728,
#18729,#18730,#18731,#18732,#18733,#18734,#18735,#18736,#18737,#18738,#18739,
#18740,#18741,#18742,#18743,#18744,#18745,#18746,#18747,#18748,#18749,#18750,
#18751,#18752,#18753,#18754,#18755,#18756,#18757,#18758,#18759,#18760,#18761,
#18762,#18763,#18764,#18765,#18766,#18767,#18768,#18769,#18770,#18771,#18772,
#18773,#18774,#18775,#18776,#18777,#18778,#18779,#18780,#18781,#18782,#18783,
#18784,#18785,#18786,#18787,#18788,#18789,#18790,#18791,#18792,#18793,#18794,
#18795,#18796,#18797,#18798,#18799,#18800,#18801,#18802,#18803,#18804,#18805,
#18806,#18807,#18808,#18809,#18810,#18811,#18812,#18813,#18814,#18815,#18816,
#18817,#18818,#18819,#18820,#18821,#18822,#18823,#18824,#18825,#18826,#18827,
#18828,#18829,#18830,#18831,#18832,#18833,#18834,#18835,#18836,#18837,#18838,
#18839,#18840,#18841,#18842,#18843,#18844,#18845,#18846,#18847,#18848,#18849,
#18850,#18851,#18852,#18853,#18854,#18855,#18856,#18857,#18858,#18859,#18860,
#18861,#18862,#18863,#18864,#18865,#18866,#18867,#18868,#18869,#18870,#18871,
#18872,#18873,#18874,#18875,#18876,#18877,#18878,#18879,#18880,#18881,#18882,
#18883,#18884,#18885,#18886,#18887,#18888,#18889,#18890,#18891,#18892,#18893,
#18894,#18895,#18896,#18897,#18898,#18899,#18900,#18901,#18902,#18903,#18904,
#18905,#18906,#18907,#18908,#18909,#18910,#18911,#18912,#18913,#18914,#18915,
#18916,#18917,#18918,#18919,#18920,#18921,#18922,#18923,#18924,#18925,#18926,
#18927,#18928,#18929,#18930,#18931,#18932,#18933,#18934,#18935,#18936,#18937,
#18938,#18939,#18940,#18941,#18942,#18943,#18944,#18945,#18946,#18947,#18948,
#18949,#18950,#18951,#18952,#18953,#18954,#18955,#18956,#18957,#18958,#18959,
#18960,#18961,#18962,#18963,#18964,#18965,#18966,#18967,#18968,#18969,#18970,
#18971,#18972,#18973,#18974,#18975,#18976,#18977,#18978,#18979,#18980,#18981,
#18982,#18983,#18984,#18985,#18986,#18987,#18988,#18989,#18990,#18991,#18992,
#18993,#18994,#18995,#18996,#18997,#18998,#18999,#19000,#19001,#19002,#19003,
#19004,#19005,#19006,#19007,#19008,#19009,#19010,#19011,#19012,#19013,#19014,
#19015,#19016,#19017,#19018,#19019,#19020,#19021,#19022,#19023,#19024,#19025,
#19026,#19027,#19028,#19029,#19030,#19031,#19032,#19033,#19034,#19035,#19036,
#19037,#19038,#19039,#19040,#19041,#19042,#19043,#19044,#19045,#19046,#19047,
#19048,#19049,#19050,#19051,#19052,#19053,#19054,#19055,#19056,#19057,#19058,
#19059,#19060,#19061,#19062,#19063,#19064,#19065,#19066,#19067,#19068,#19069,
#19070,#19071,#19072,#19073,#19074,#19075,#19076,#19077,#19078,#19079,#19080,
#19081,#19082,#19083,#19084,#19085,#19086,#19087,#19088,#19089,#19090,#19091,
#19092,#19093,#19094,#19095,#19096,#19097,#19098,#19099,#19100,#19101,#19102,
#19103,#19104,#19105,#19106,#19107,#19108,#19109,#19110,#19111,#19112,#19113,
#19114,#19115,#19116,#19117,#19118,#19119,#19120,#19121,#19122,#19123,#19124,
#19125,#19126,#19127,#19128,#19129,#19130,#19131,#19132,#19133,#19134,#19135,
#19136,#19137,#19138,#19139,#19140,#19141,#19142,#19143,#19144,#19145,#19146,
#19147,#19148,#19149,#19150,#19151,#19152,#19153,#19154,#19155,#19156,#19157,
#19158,#19159,#19160,#19161,#19162,#19163,#19164,#19165,#19166,#19167,#19168,
#19169,#19170,#19171,#19172,#19173,#19174,#19175,#19176,#19177,#19178,#19179,
#19180,#19181,#19182,#19183,#19184,#19185,#19186,#19187,#19188,#19189,#19190,
#19191,#19192,#19193,#19194,#19195,#19196,#19197,#19198,#19199,#19200,#19201,
#19202,#19203,#19204,#19205,#19206,#19207,#19208,#19209,#19210,#19211,#19212,
#19213,#19214,#19215,#19216,#19217,#19218,#19219,#19220,#19221,#19222,#19223,
#19224,#19225,#19226,#19227,#19228,#19229,#19230,#19231,#19232,#19233,#19234,
#19235,#19236,#19237,#19238,#19239,#19240,#19241,#19242,#19243,#19244,#19245,
#19246,#19247,#19248,#19249,#19250,#19251,#19252,#19253,#19254,#19255,#19256,
#19257,#19258,#19259,#19260,#19261,#19262,#19263,#19264,#19265,#19266,#19267,
#19268,#19269,#19270,#19271,#19272,#19273,#19274,#19275,#19276,#19277,#19278,
#19279,#19280,#19281,#19282,#19283,#19284,#19285,#19286,#19287,#19288,#19289,
#19290,#19291,#19292,#19293,#19294,#19295,#19296,#19297,#19298,#19299,#19300,
#19301,#19302,#19303,#19304,#19305,#19306,#19307,#19308,#19309,#19310,#19311,
#19312,#19313,#19314,#19315,#19316,#19317,#19318,#19319,#19320,#19321,#19322,
#19323,#19324,#19325,#19326,#19327,#19328,#19329,#19330,#19331,#19332,#19333,
#19334,#19335,#19336,#19337,#19338,#19339,#19340,#19341,#19342,#19343,#19344,
#19345,#19346,#19347,#19348,#19349,#19350,#19351,#19352,#19353,#19354,#19355,
#19356,#19357,#19358,#19359,#19360,#19361,#19362,#19363,#19364,#19365,#19366,
#19367,#19368,#19369,#19370,#19371,#19372,#19373,#19374,#19375,#19376,#19377,
#19378,#19379,#19380,#19381,#19382,#19383,#19384,#19385,#19386,#19387,#19388,
#19389,#19390,#19391,#19392,#19393,#19394,#19395,#19396,#19397,#19398,#19399,
#19400,#19401,#19402,#19403,#19404,#19405,#19406,#19407,#19408,#19409,#19410,
#19411,#19412,#19413,#19414,#19415,#19416,#19417,#19418,#19419,#19420,#19421,
#19422,#19423,#19424,#19425,#19426,#19427,#19428,#19429,#19430,#19431,#19432,
#19433,#19434,#19435,#19436,#19437,#19438)),.UNSPECIFIED.,.F.,.F.,.F.)
B_SPLINE_SURFACE_WITH_KNOTS((4,4),(3,2,2,2,2,2,2,2,2,2,2,2,2,2,2,2,2,2,
2,2,2,2,2,2,2,2,2,2,2,2,2,2,2,2,2,2,2,2,2,2,2,2,2,2,2,2,2,2,2,2,2,2,2,2,
2,2,2,2,2,2,2,2,2,2,2,2,2,2,2,2,2,2,2,2,2,2,2,2,2,2,2,2,2,2,2,2,2,2,2,2,
2,2,2,2,2,2,2,2,2,2,2,2,2,2,2,2,2,2,2,2,2,2,2,2,2,2,2,2,2,2,2,2,2,2,2,2,
2,2,2,2,2,2,2,2,2,2,2,2,2,2,2,2,2,2,2,2,2,2,2,2,2,2,2,2,2,2,2,2,2,2,2,2,
2,2,2,2,2,2,2,2,2,2,2,2,2,2,2,2,2,2,2,2,2,2,2,2,2,2,2,2,2,2,2,2,2,2,2,2,
2,2,2,2,2,2,2,2,2,2,2,2,2,2,2,2,2,2,2,2,2,2,2,2,2,2,2,2,2,2,2,2,2,2,2,2,
2,2,2,2,2,2,2,2,2,2,2,2,2,2,2,2,2,2,2,2,2,2,2,2,2,2,2,2,2,2,2,2,2,2,2,2,
2,2,2,2,2,2,2,2,2,2,2,2,2,2,2,2,2,2,2,2,2,2,2,2,2,2,2,2,2,2,2,2,2,2,2,2,
2,2,2,2,2,2,2,2,2,2,2,2,2,2,2,2,2,2,2,2,2,2,2,2,2,2,2,2,2,2,2,2,2,2,2,2,
2,2,2,2,2,2,2,2,2,2,2,2,2,2,2,2,2,2,2,2,2,2,2,2,2,2,2,2,2,2,2,2,2,2,2,2,
2,2,2,2,2,2,2,2,2,2,2,2,2,2,2,2,2,2,2,2,2,2,2,2,2,2,2,2,2,2,2,2,2,2,2,2,
2,2,2,2,2,2,2,2,2,2,2,2,2,2,2,2,2,2,2,2,2,2,2,2,2,2,2,2,2,2,2,2,2,2,2,2,
2,2,2,2,2,2,2,2,2,2,2,2,2,2,2,2,2,2,2,2,2,2,2,2,2,2,2,2,2,2,2,2,2,2,2,2,
3),(0.,1.),(0.,0.00205761316872428,0.00411522633744856,0.00617283950617284,
0.00823045267489712,0.0102880658436214,0.0123456790123457,0.01440329218107,
0.0164609053497942,0.0185185185185185,0.0205761316872428,0.0226337448559671,
0.0246913580246914,0.0267489711934156,0.0288065843621399,0.0308641975308642,
0.0329218106995885,0.0349794238683128,0.037037037037037,0.0390946502057613,
0.0411522633744856,0.0432098765432099,0.0452674897119342,0.0473251028806584,
0.0493827160493827,0.051440329218107,0.0534979423868313,0.0555555555555556,
0.0576131687242798,0.0596707818930041,0.0617283950617284,0.0637860082304527,
0.065843621399177,0.0679012345679012,0.0699588477366255,0.0720164609053498,
0.0740740740740741,0.0761316872427984,0.0781893004115226,0.0802469135802469,
0.0823045267489712,0.0843621399176955,0.0864197530864197,0.088477366255144,
0.0905349794238683,0.0925925925925926,0.0946502057613169,0.0967078189300412,
0.0987654320987654,0.10082304526749,0.102880658436214,0.104938271604938,
0.106995884773663,0.109053497942387,0.111111111111111,0.113168724279835,
0.11522633744856,0.117283950617284,0.119341563786008,0.121399176954733,
0.123456790123457,0.125514403292181,0.127572016460905,0.12962962962963,
0.131687242798354,0.133744855967078,0.135802469135802,0.137860082304527,
0.139917695473251,0.141975308641975,0.1440329218107,0.146090534979424,0.148148148148148,
0.150205761316872,0.152263374485597,0.154320987654321,0.156378600823045,
0.15843621399177,0.160493827160494,0.162551440329218,0.164609053497942,
0.166666666666667,0.168724279835391,0.170781893004115,0.172839506172839,
0.174897119341564,0.176954732510288,0.179012345679012,0.181069958847737,
0.183127572016461,0.185185185185185,0.187242798353909,0.189300411522634,
0.191358024691358,0.193415637860082,0.195473251028807,0.197530864197531,
0.199588477366255,0.201646090534979,0.203703703703704,0.205761316872428,
0.207818930041152,0.209876543209877,0.211934156378601,0.213991769547325,
0.216049382716049,0.218106995884774,0.220164609053498,0.222222222222222,
0.224279835390947,0.226337448559671,0.228395061728395,0.230452674897119,
0.232510288065844,0.234567901234568,0.236625514403292,0.238683127572016,
0.240740740740741,0.242798353909465,0.244855967078189,0.246913580246914,
0.248971193415638,0.251028806584362,0.253086419753086,0.255144032921811,
0.257201646090535,0.259259259259259,0.261316872427984,0.263374485596708,
0.265432098765432,0.267489711934156,0.269547325102881,0.271604938271605,
0.273662551440329,0.275720164609054,0.277777777777778,0.279835390946502,
0.281893004115226,0.283950617283951,0.286008230452675,0.288065843621399,
0.290123456790123,0.292181069958848,0.294238683127572,0.296296296296296,
0.298353909465021,0.300411522633745,0.302469135802469,0.304526748971193,
0.306584362139918,0.308641975308642,0.310699588477366,0.312757201646091,
0.314814814814815,0.316872427983539,0.318930041152263,0.320987654320988,
0.323045267489712,0.325102880658436,0.327160493827161,0.329218106995885,
0.331275720164609,0.333333333333333,0.335390946502058,0.337448559670782,
0.339506172839506,0.34156378600823,0.343621399176955,0.345679012345679,
0.347736625514403,0.349794238683128,0.351851851851852,0.353909465020576,
0.3559670781893,0.358024691358025,0.360082304526749,0.362139917695473,0.364197530864198,
0.366255144032922,0.368312757201646,0.37037037037037,0.372427983539095,
0.374485596707819,0.376543209876543,0.378600823045267,0.380658436213992,
0.382716049382716,0.38477366255144,0.386831275720165,0.388888888888889,
0.390946502057613,0.393004115226337,0.395061728395062,0.397119341563786,
0.39917695473251,0.401234567901235,0.403292181069959,0.405349794238683,
0.407407407407407,0.409465020576132,0.411522633744856,0.41358024691358,
0.415637860082305,0.417695473251029,0.419753086419753,0.421810699588477,
0.423868312757202,0.425925925925926,0.42798353909465,0.430041152263374,
0.432098765432099,0.434156378600823,0.436213991769547,0.438271604938272,
0.440329218106996,0.44238683127572,0.444444444444444,0.446502057613169,
0.448559670781893,0.450617283950617,0.452674897119342,0.454732510288066,
0.45679012345679,0.458847736625514,0.460905349794239,0.462962962962963,
0.465020576131687,0.467078189300412,0.469135802469136,0.47119341563786,
0.473251028806584,0.475308641975309,0.477366255144033,0.479423868312757,
0.481481481481481,0.483539094650206,0.48559670781893,0.487654320987654,
0.489711934156379,0.491769547325103,0.493827160493827,0.495884773662551,
0.497942386831276,0.5,0.502057613168724,0.504115226337449,0.506172839506173,
0.508230452674897,0.510288065843621,0.512345679012346,0.51440329218107,
0.516460905349794,0.518518518518518,0.520576131687243,0.522633744855967,
0.524691358024691,0.526748971193416,0.52880658436214,0.530864197530864,
0.532921810699588,0.534979423868313,0.537037037037037,0.539094650205761,
0.541152263374486,0.54320987654321,0.545267489711934,0.547325102880658,
0.549382716049383,0.551440329218107,0.553497942386831,0.555555555555556,
0.55761316872428,0.559670781893004,0.561728395061728,0.563786008230453,
0.565843621399177,0.567901234567901,0.569958847736626,0.57201646090535,
0.574074074074074,0.576131687242798,0.578189300411523,0.580246913580247,
0.582304526748971,0.584362139917695,0.58641975308642,0.588477366255144,
0.590534979423868,0.592592592592593,0.594650205761317,0.596707818930041,
0.598765432098765,0.60082304526749,0.602880658436214,0.604938271604938,
0.606995884773663,0.609053497942387,0.611111111111111,0.613168724279835,
0.61522633744856,0.617283950617284,0.619341563786008,0.621399176954732,
0.623456790123457,0.625514403292181,0.627572016460905,0.62962962962963,
0.631687242798354,0.633744855967078,0.635802469135803,0.637860082304527,
0.639917695473251,0.641975308641975,0.6440329218107,0.646090534979424,0.648148148148148,
0.650205761316872,0.652263374485597,0.654320987654321,0.656378600823045,
0.65843621399177,0.660493827160494,0.662551440329218,0.664609053497942,
0.666666666666667,0.668724279835391,0.670781893004115,0.672839506172839,
0.674897119341564,0.676954732510288,0.679012345679012,0.681069958847737,
0.683127572016461,0.685185185185185,0.687242798353909,0.689300411522634,
0.691358024691358,0.693415637860082,0.695473251028807,0.697530864197531,
0.699588477366255,0.701646090534979,0.703703703703704,0.705761316872428,
0.707818930041152,0.709876543209877,0.711934156378601,0.713991769547325,
0.716049382716049,0.718106995884774,0.720164609053498,0.722222222222222,
0.724279835390947,0.726337448559671,0.728395061728395,0.730452674897119,
0.732510288065844,0.734567901234568,0.736625514403292,0.738683127572016,
0.740740740740741,0.742798353909465,0.744855967078189,0.746913580246914,
0.748971193415638,0.751028806584362,0.753086419753086,0.755144032921811,
0.757201646090535,0.759259259259259,0.761316872427984,0.763374485596708,
0.765432098765432,0.767489711934156,0.769547325102881,0.771604938271605,
0.773662551440329,0.775720164609053,0.777777777777778,0.779835390946502,
0.781893004115226,0.783950617283951,0.786008230452675,0.788065843621399,
0.790123456790123,0.792181069958848,0.794238683127572,0.796296296296296,
0.798353909465021,0.800411522633745,0.802469135802469,0.804526748971193,
0.806584362139918,0.808641975308642,0.810699588477366,0.812757201646091,
0.814814814814815,0.816872427983539,0.818930041152263,0.820987654320988,
0.823045267489712,0.825102880658436,0.827160493827161,0.829218106995885,
0.831275720164609,0.833333333333333,0.835390946502058,0.837448559670782,
0.839506172839506,0.84156378600823,0.843621399176955,0.845679012345679,
0.847736625514403,0.849794238683128,0.851851851851852,0.853909465020576,
0.8559670781893,0.858024691358025,0.860082304526749,0.862139917695473,0.864197530864197,
0.866255144032922,0.868312757201646,0.87037037037037,0.872427983539095,
0.874485596707819,0.876543209876543,0.878600823045268,0.880658436213992,
0.882716049382716,0.88477366255144,0.886831275720165,0.888888888888889,
0.890946502057613,0.893004115226337,0.895061728395062,0.897119341563786,
0.89917695473251,0.901234567901235,0.903292181069959,0.905349794238683,
0.907407407407407,0.909465020576132,0.911522633744856,0.91358024691358,
0.915637860082305,0.917695473251029,0.919753086419753,0.921810699588477,
0.923868312757202,0.925925925925926,0.92798353909465,0.930041152263374,
0.932098765432099,0.934156378600823,0.936213991769547,0.938271604938272,
0.940329218106996,0.94238683127572,0.944444444444444,0.946502057613169,
0.948559670781893,0.950617283950617,0.952674897119342,0.954732510288066,
0.95679012345679,0.958847736625514,0.960905349794239,0.962962962962963,
0.965020576131687,0.967078189300412,0.969135802469136,0.97119341563786,
0.973251028806584,0.975308641975309,0.977366255144033,0.979423868312757,
0.981481481481482,0.983539094650206,0.98559670781893,0.987654320987654,
0.989711934156379,0.991769547325103,0.993827160493827,0.995884773662551,
0.997942386831276,1.),.UNSPECIFIED.)
GEOMETRIC_REPRESENTATION_ITEM()
RATIONAL_B_SPLINE_SURFACE(((1.,0.866025403784439,1.,0.866025403784439,1.,
0.866025403784439,1.,0.866025403784439,1.,0.866025403784439,1.,0.866025403784439,
1.,0.866025403784439,1.,0.866025403784439,1.,0.866025403784439,1.,0.866025403784439,
1.,0.866025403784439,1.,0.866025403784439,1.,0.866025403784439,1.,0.866025403784439,
1.,0.866025403784439,1.,0.866025403784439,1.,0.866025403784439,1.,0.866025403784439,
1.,0.866025403784439,1.,0.866025403784439,1.,0.866025403784439,1.,0.866025403784439,
1.,0.866025403784439,1.,0.866025403784439,1.,0.866025403784439,1.,0.866025403784439,
1.,0.866025403784439,1.,0.866025403784439,1.,0.866025403784439,1.,0.866025403784439,
1.,0.866025403784439,1.,0.866025403784439,1.,0.866025403784439,1.,0.866025403784439,
1.,0.866025403784439,1.,0.866025403784439,1.,0.866025403784439,1.,0.866025403784439,
1.,0.866025403784439,1.,0.866025403784439,1.,0.866025403784439,1.,0.866025403784439,
1.,0.866025403784439,1.,0.866025403784439,1.,0.866025403784439,1.,0.866025403784439,
1.,0.866025403784439,1.,0.866025403784439,1.,0.866025403784439,1.,0.866025403784439,
1.,0.866025403784439,1.,0.866025403784439,1.,0.866025403784439,1.,0.866025403784439,
1.,0.866025403784439,1.,0.866025403784439,1.,0.866025403784439,1.,0.866025403784439,
1.,0.866025403784439,1.,0.866025403784439,1.,0.866025403784439,1.,0.866025403784439,
1.,0.866025403784439,1.,0.866025403784439,1.,0.866025403784439,1.,0.866025403784439,
1.,0.866025403784439,1.,0.866025403784439,1.,0.866025403784439,1.,0.866025403784439,
1.,0.866025403784439,1.,0.866025403784439,1.,0.866025403784439,1.,0.866025403784439,
1.,0.866025403784439,1.,0.866025403784439,1.,0.866025403784439,1.,0.866025403784439,
1.,0.866025403784439,1.,0.866025403784439,1.,0.866025403784439,1.,0.866025403784439,
1.,0.866025403784439,1.,0.866025403784439,1.,0.866025403784439,1.,0.866025403784439,
1.,0.866025403784439,1.,0.866025403784439,1.,0.866025403784439,1.,0.866025403784439,
1.,0.866025403784439,1.,0.866025403784439,1.,0.866025403784439,1.,0.866025403784439,
1.,0.866025403784439,1.,0.866025403784439,1.,0.866025403784439,1.,0.866025403784439,
1.,0.866025403784439,1.,0.866025403784439,1.,0.866025403784439,1.,0.866025403784439,
1.,0.866025403784439,1.,0.866025403784439,1.,0.866025403784439,1.,0.866025403784439,
1.,0.866025403784439,1.,0.866025403784439,1.,0.866025403784439,1.,0.866025403784439,
1.,0.866025403784439,1.,0.866025403784439,1.,0.866025403784439,1.,0.866025403784439,
1.,0.866025403784439,1.,0.866025403784439,1.,0.866025403784439,1.,0.866025403784439,
1.,0.866025403784439,1.,0.866025403784439,1.,0.866025403784439,1.,0.866025403784439,
1.,0.866025403784439,1.,0.866025403784439,1.,0.866025403784439,1.,0.866025403784439,
1.,0.866025403784439,1.,0.866025403784439,1.,0.866025403784439,1.,0.866025403784439,
1.,0.866025403784439,1.,0.866025403784439,1.,0.866025403784439,1.,0.866025403784439,
1.,0.866025403784439,1.,0.866025403784439,1.,0.866025403784439,1.,0.866025403784439,
1.,0.866025403784439,1.,0.866025403784439,1.,0.866025403784439,1.,0.866025403784439,
1.,0.866025403784439,1.,0.866025403784439,1.,0.866025403784439,1.,0.866025403784439,
1.,0.866025403784439,1.,0.866025403784439,1.,0.866025403784439,1.,0.866025403784439,
1.,0.866025403784439,1.,0.866025403784439,1.,0.866025403784439,1.,0.866025403784439,
1.,0.866025403784439,1.,0.866025403784439,1.,0.866025403784439,1.,0.866025403784439,
1.,0.866025403784439,1.,0.866025403784439,1.,0.866025403784439,1.,0.866025403784439,
1.,0.866025403784439,1.,0.866025403784439,1.,0.866025403784439,1.,0.866025403784439,
1.,0.866025403784439,1.,0.866025403784439,1.,0.866025403784439,1.,0.866025403784439,
1.,0.866025403784439,1.,0.866025403784439,1.,0.866025403784439,1.,0.866025403784439,
1.,0.866025403784439,1.,0.866025403784439,1.,0.866025403784439,1.,0.866025403784439,
1.,0.866025403784439,1.,0.866025403784439,1.,0.866025403784439,1.,0.866025403784439,
1.,0.866025403784439,1.,0.866025403784439,1.,0.866025403784439,1.,0.866025403784439,
1.,0.866025403784439,1.,0.866025403784439,1.,0.866025403784439,1.,0.866025403784439,
1.,0.866025403784439,1.,0.866025403784439,1.,0.866025403784439,1.,0.866025403784439,
1.,0.866025403784439,1.,0.866025403784439,1.,0.866025403784439,1.,0.866025403784439,
1.,0.866025403784439,1.,0.866025403784439,1.,0.866025403784439,1.,0.866025403784439,
1.,0.866025403784439,1.,0.866025403784439,1.,0.866025403784439,1.,0.866025403784439,
1.,0.866025403784439,1.,0.866025403784439,1.,0.866025403784439,1.,0.866025403784439,
1.,0.866025403784439,1.,0.866025403784439,1.,0.866025403784439,1.,0.866025403784439,
1.,0.866025403784439,1.,0.866025403784439,1.,0.866025403784439,1.,0.866025403784439,
1.,0.866025403784439,1.,0.866025403784439,1.,0.866025403784439,1.,0.866025403784439,
1.,0.866025403784439,1.,0.866025403784439,1.,0.866025403784439,1.,0.866025403784439,
1.,0.866025403784439,1.,0.866025403784439,1.,0.866025403784439,1.,0.866025403784439,
1.,0.866025403784439,1.,0.866025403784439,1.,0.866025403784439,1.,0.866025403784439,
1.,0.866025403784439,1.,0.866025403784439,1.,0.866025403784439,1.,0.866025403784439,
1.,0.866025403784439,1.,0.866025403784439,1.,0.866025403784439,1.,0.866025403784439,
1.,0.866025403784439,1.,0.866025403784439,1.,0.866025403784439,1.,0.866025403784439,
1.,0.866025403784439,1.,0.866025403784439,1.,0.866025403784439,1.,0.866025403784439,
1.,0.866025403784439,1.,0.866025403784439,1.,0.866025403784439,1.,0.866025403784439,
1.,0.866025403784439,1.,0.866025403784439,1.,0.866025403784439,1.,0.866025403784439,
1.,0.866025403784439,1.,0.866025403784439,1.,0.866025403784439,1.,0.866025403784439,
1.,0.866025403784439,1.,0.866025403784439,1.,0.866025403784439,1.,0.866025403784439,
1.,0.866025403784439,1.,0.866025403784439,1.,0.866025403784439,1.,0.866025403784439,
1.,0.866025403784439,1.,0.866025403784439,1.,0.866025403784439,1.,0.866025403784439,
1.,0.866025403784439,1.,0.866025403784439,1.,0.866025403784439,1.,0.866025403784439,
1.,0.866025403784439,1.,0.866025403784439,1.,0.866025403784439,1.,0.866025403784439,
1.,0.866025403784439,1.,0.866025403784439,1.,0.866025403784439,1.,0.866025403784439,
1.,0.866025403784439,1.,0.866025403784439,1.,0.866025403784439,1.,0.866025403784439,
1.,0.866025403784439,1.,0.866025403784439,1.,0.866025403784439,1.,0.866025403784439,
1.,0.866025403784439,1.,0.866025403784439,1.,0.866025403784439,1.,0.866025403784439,
1.,0.866025403784439,1.,0.866025403784439,1.,0.866025403784439,1.,0.866025403784439,
1.,0.866025403784439,1.,0.866025403784439,1.,0.866025403784439,1.,0.866025403784439,
1.,0.866025403784439,1.,0.866025403784439,1.,0.866025403784439,1.,0.866025403784439,
1.,0.866025403784439,1.,0.866025403784439,1.,0.866025403784439,1.,0.866025403784439,
1.,0.866025403784439,1.,0.866025403784439,1.,0.866025403784439,1.,0.866025403784439,
1.,0.866025403784439,1.,0.866025403784439,1.,0.866025403784439,1.,0.866025403784439,
1.,0.866025403784439,1.,0.866025403784439,1.,0.866025403784439,1.,0.866025403784439,
1.,0.866025403784439,1.,0.866025403784439,1.,0.866025403784439,1.,0.866025403784439,
1.,0.866025403784439,1.,0.866025403784439,1.,0.866025403784439,1.,0.866025403784439,
1.,0.866025403784439,1.,0.866025403784439,1.,0.866025403784439,1.,0.866025403784439,
1.,0.866025403784439,1.,0.866025403784439,1.,0.866025403784439,1.,0.866025403784439,
1.,0.866025403784439,1.,0.866025403784439,1.,0.866025403784439,1.,0.866025403784439,
1.,0.866025403784439,1.,0.866025403784439,1.,0.866025403784439,1.,0.866025403784439,
1.,0.866025403784439,1.,0.866025403784439,1.,0.866025403784439,1.,0.866025403784439,
1.,0.866025403784439,1.,0.866025403784439,1.,0.866025403784439,1.,0.866025403784439,
1.,0.866025403784439,1.,0.866025403784439,1.,0.866025403784439,1.,0.866025403784439,
1.,0.866025403784439,1.,0.866025403784439,1.,0.866025403784439,1.,0.866025403784439,
1.,0.866025403784439,1.,0.866025403784439,1.,0.866025403784439,1.,0.866025403784439,
1.,0.866025403784439,1.,0.866025403784439,1.,0.866025403784439,1.,0.866025403784439,
1.,0.866025403784439,1.,0.866025403784439,1.,0.866025403784439,1.,0.866025403784439,
1.,0.866025403784439,1.,0.866025403784439,1.,0.866025403784439,1.,0.866025403784439,
1.,0.866025403784439,1.,0.866025403784439,1.,0.866025403784439,1.,0.866025403784439,
1.,0.866025403784439,1.,0.866025403784439,1.,0.866025403784439,1.,0.866025403784439,
1.,0.866025403784439,1.,0.866025403784439,1.,0.866025403784439,1.,0.866025403784439,
1.,0.866025403784439,1.,0.866025403784439,1.,0.866025403784439,1.,0.866025403784439,
1.,0.866025403784439,1.,0.866025403784439,1.,0.866025403784439,1.,0.866025403784439,
1.,0.866025403784439,1.,0.866025403784439,1.,0.866025403784439,1.,0.866025403784439,
1.,0.866025403784439,1.,0.866025403784439,1.,0.866025403784439,1.,0.866025403784439,
1.,0.866025403784439,1.,0.866025403784439,1.,0.866025403784439,1.,0.866025403784439,
1.,0.866025403784439,1.,0.866025403784439,1.,0.866025403784439,1.,0.866025403784439,
1.,0.866025403784439,1.,0.866025403784439,1.,0.866025403784439,1.,0.866025403784439,
1.,0.866025403784439,1.,0.866025403784439,1.,0.866025403784439,1.,0.866025403784439,
1.,0.866025403784439,1.,0.866025403784439,1.,0.866025403784439,1.,0.866025403784439,
1.,0.866025403784439,1.,0.866025403784439,1.,0.866025403784439,1.,0.866025403784439,
1.,0.866025403784439,1.,0.866025403784439,1.,0.866025403784439,1.,0.866025403784439,
1.,0.866025403784439,1.,0.866025403784439,1.,0.866025403784439,1.,0.866025403784439,
1.,0.866025403784439,1.,0.866025403784439,1.,0.866025403784439,1.,0.866025403784439,
1.,0.866025403784439,1.,0.866025403784439,1.,0.866025403784439,1.,0.866025403784439,
1.,0.866025403784439,1.,0.866025403784439,1.,0.866025403784439,1.,0.866025403784439,
1.,0.866025403784439,1.,0.866025403784439,1.,0.866025403784439,1.,0.866025403784439,
1.,0.866025403784439,1.,0.866025403784439,1.,0.866025403784439,1.,0.866025403784439,
1.,0.866025403784439,1.,0.866025403784439,1.,0.866025403784439,1.,0.866025403784439,
1.,0.866025403784439,1.,0.866025403784439,1.,0.866025403784439,1.,0.866025403784439,
1.,0.866025403784439,1.,0.866025403784439,1.,0.866025403784439,1.,0.866025403784439,
1.,0.866025403784439,1.,0.866025403784439,1.,0.866025403784439,1.,0.866025403784439,
1.,0.866025403784439,1.,0.866025403784439,1.,0.866025403784439,1.,0.866025403784439,
1.,0.866025403784439,1.,0.866025403784439,1.,0.866025403784439,1.,0.866025403784439,
1.),(0.641165742156689,0.555265820743996,0.641165742156689,0.555265820743996,
0.641165742156689,0.555265820743996,0.641165742156689,0.555265820743996,
0.641165742156689,0.555265820743996,0.641165742156689,0.555265820743996,
0.641165742156689,0.555265820743996,0.641165742156689,0.555265820743996,
0.641165742156689,0.555265820743996,0.641165742156689,0.555265820743996,
0.641165742156689,0.555265820743996,0.641165742156689,0.555265820743996,
0.641165742156689,0.555265820743996,0.641165742156689,0.555265820743996,
0.641165742156689,0.555265820743996,0.641165742156689,0.555265820743996,
0.641165742156689,0.555265820743996,0.641165742156689,0.555265820743996,
0.641165742156689,0.555265820743996,0.641165742156689,0.555265820743996,
0.641165742156689,0.555265820743996,0.641165742156689,0.555265820743996,
0.641165742156689,0.555265820743996,0.641165742156689,0.555265820743996,
0.641165742156689,0.555265820743996,0.641165742156689,0.555265820743996,
0.641165742156689,0.555265820743996,0.641165742156689,0.555265820743996,
0.641165742156689,0.555265820743996,0.641165742156689,0.555265820743996,
0.641165742156689,0.555265820743996,0.641165742156689,0.555265820743996,
0.641165742156689,0.555265820743996,0.641165742156689,0.555265820743996,
0.641165742156689,0.555265820743996,0.641165742156689,0.555265820743996,
0.641165742156689,0.555265820743996,0.641165742156689,0.555265820743996,
0.641165742156689,0.555265820743996,0.641165742156689,0.555265820743996,
0.641165742156689,0.555265820743996,0.641165742156689,0.555265820743996,
0.641165742156689,0.555265820743996,0.641165742156689,0.555265820743996,
0.641165742156689,0.555265820743996,0.641165742156689,0.555265820743996,
0.641165742156689,0.555265820743996,0.641165742156689,0.555265820743996,
0.641165742156689,0.555265820743996,0.641165742156689,0.555265820743996,
0.641165742156689,0.555265820743996,0.641165742156689,0.555265820743996,
0.641165742156689,0.555265820743996,0.641165742156689,0.555265820743996,
0.641165742156689,0.555265820743996,0.641165742156689,0.555265820743996,
0.641165742156689,0.555265820743996,0.641165742156689,0.555265820743996,
0.641165742156689,0.555265820743996,0.641165742156689,0.555265820743996,
0.641165742156689,0.555265820743996,0.641165742156689,0.555265820743996,
0.641165742156689,0.555265820743996,0.641165742156689,0.555265820743996,
0.641165742156689,0.555265820743996,0.641165742156689,0.555265820743996,
0.641165742156689,0.555265820743996,0.641165742156689,0.555265820743996,
0.641165742156689,0.555265820743996,0.641165742156689,0.555265820743996,
0.641165742156689,0.555265820743996,0.641165742156689,0.555265820743996,
0.641165742156689,0.555265820743996,0.641165742156689,0.555265820743996,
0.641165742156689,0.555265820743996,0.641165742156689,0.555265820743996,
0.641165742156689,0.555265820743996,0.641165742156689,0.555265820743996,
0.641165742156689,0.555265820743996,0.641165742156689,0.555265820743996,
0.641165742156689,0.555265820743996,0.641165742156689,0.555265820743996,
0.641165742156689,0.555265820743996,0.641165742156689,0.555265820743996,
0.641165742156689,0.555265820743996,0.641165742156689,0.555265820743996,
0.641165742156689,0.555265820743996,0.641165742156689,0.555265820743996,
0.641165742156689,0.555265820743996,0.641165742156689,0.555265820743996,
0.641165742156689,0.555265820743996,0.641165742156689,0.555265820743996,
0.641165742156689,0.555265820743996,0.641165742156689,0.555265820743996,
0.641165742156689,0.555265820743996,0.641165742156689,0.555265820743996,
0.641165742156689,0.555265820743996,0.641165742156689,0.555265820743996,
0.641165742156689,0.555265820743996,0.641165742156689,0.555265820743996,
0.641165742156689,0.555265820743996,0.641165742156689,0.555265820743996,
0.641165742156689,0.555265820743996,0.641165742156689,0.555265820743996,
0.641165742156689,0.555265820743996,0.641165742156689,0.555265820743996,
0.641165742156689,0.555265820743996,0.641165742156689,0.555265820743996,
0.641165742156689,0.555265820743996,0.641165742156689,0.555265820743996,
0.641165742156689,0.555265820743996,0.641165742156689,0.555265820743996,
0.641165742156689,0.555265820743996,0.641165742156689,0.555265820743996,
0.641165742156689,0.555265820743996,0.641165742156689,0.555265820743996,
0.641165742156689,0.555265820743996,0.641165742156689,0.555265820743996,
0.641165742156689,0.555265820743996,0.641165742156689,0.555265820743996,
0.641165742156689,0.555265820743996,0.641165742156689,0.555265820743996,
0.641165742156689,0.555265820743996,0.641165742156689,0.555265820743996,
0.641165742156689,0.555265820743996,0.641165742156689,0.555265820743996,
0.641165742156689,0.555265820743996,0.641165742156689,0.555265820743996,
0.641165742156689,0.555265820743996,0.641165742156689,0.555265820743996,
0.641165742156689,0.555265820743996,0.641165742156689,0.555265820743996,
0.641165742156689,0.555265820743996,0.641165742156689,0.555265820743996,
0.641165742156689,0.555265820743996,0.641165742156689,0.555265820743996,
0.641165742156689,0.555265820743996,0.641165742156689,0.555265820743996,
0.641165742156689,0.555265820743996,0.641165742156689,0.555265820743996,
0.641165742156689,0.555265820743996,0.641165742156689,0.555265820743996,
0.641165742156689,0.555265820743996,0.641165742156689,0.555265820743996,
0.641165742156689,0.555265820743996,0.641165742156689,0.555265820743996,
0.641165742156689,0.555265820743996,0.641165742156689,0.555265820743996,
0.641165742156689,0.555265820743996,0.641165742156689,0.555265820743996,
0.641165742156689,0.555265820743996,0.641165742156689,0.555265820743996,
0.641165742156689,0.555265820743996,0.641165742156689,0.555265820743996,
0.641165742156689,0.555265820743996,0.641165742156689,0.555265820743996,
0.641165742156689,0.555265820743996,0.641165742156689,0.555265820743996,
0.641165742156689,0.555265820743996,0.641165742156689,0.555265820743996,
0.641165742156689,0.555265820743996,0.641165742156689,0.555265820743996,
0.641165742156689,0.555265820743996,0.641165742156689,0.555265820743996,
0.641165742156689,0.555265820743996,0.641165742156689,0.555265820743996,
0.641165742156689,0.555265820743996,0.641165742156689,0.555265820743996,
0.641165742156689,0.555265820743996,0.641165742156689,0.555265820743996,
0.641165742156689,0.555265820743996,0.641165742156689,0.555265820743996,
0.641165742156689,0.555265820743996,0.641165742156689,0.555265820743996,
0.641165742156689,0.555265820743996,0.641165742156689,0.555265820743996,
0.641165742156689,0.555265820743996,0.641165742156689,0.555265820743996,
0.641165742156689,0.555265820743996,0.641165742156689,0.555265820743996,
0.641165742156689,0.555265820743996,0.641165742156689,0.555265820743996,
0.641165742156689,0.555265820743996,0.641165742156689,0.555265820743996,
0.641165742156689,0.555265820743996,0.641165742156689,0.555265820743996,
0.641165742156689,0.555265820743996,0.641165742156689,0.555265820743996,
0.641165742156689,0.555265820743996,0.641165742156689,0.555265820743996,
0.641165742156689,0.555265820743996,0.641165742156689,0.555265820743996,
0.641165742156689,0.555265820743996,0.641165742156689,0.555265820743996,
0.641165742156689,0.555265820743996,0.641165742156689,0.555265820743996,
0.641165742156689,0.555265820743996,0.641165742156689,0.555265820743996,
0.641165742156689,0.555265820743996,0.641165742156689,0.555265820743996,
0.641165742156689,0.555265820743996,0.641165742156689,0.555265820743996,
0.641165742156689,0.555265820743996,0.641165742156689,0.555265820743996,
0.641165742156689,0.555265820743996,0.641165742156689,0.555265820743996,
0.641165742156689,0.555265820743996,0.641165742156689,0.555265820743996,
0.641165742156689,0.555265820743996,0.641165742156689,0.555265820743996,
0.641165742156689,0.555265820743996,0.641165742156689,0.555265820743996,
0.641165742156689,0.555265820743996,0.641165742156689,0.555265820743996,
0.641165742156689,0.555265820743996,0.641165742156689,0.555265820743996,
0.641165742156689,0.555265820743996,0.641165742156689,0.555265820743996,
0.641165742156689,0.555265820743996,0.641165742156689,0.555265820743996,
0.641165742156689,0.555265820743996,0.641165742156689,0.555265820743996,
0.641165742156689,0.555265820743996,0.641165742156689,0.555265820743996,
0.641165742156689,0.555265820743996,0.641165742156689,0.555265820743996,
0.641165742156689,0.555265820743996,0.641165742156689,0.555265820743996,
0.641165742156689,0.555265820743996,0.641165742156689,0.555265820743996,
0.641165742156689,0.555265820743996,0.641165742156689,0.555265820743996,
0.641165742156689,0.555265820743996,0.641165742156689,0.555265820743996,
0.641165742156689,0.555265820743996,0.641165742156689,0.555265820743996,
0.641165742156689,0.555265820743996,0.641165742156689,0.555265820743996,
0.641165742156689,0.555265820743996,0.641165742156689,0.555265820743996,
0.641165742156689,0.555265820743996,0.641165742156689,0.555265820743996,
0.641165742156689,0.555265820743996,0.641165742156689,0.555265820743996,
0.641165742156689,0.555265820743996,0.641165742156689,0.555265820743996,
0.641165742156689,0.555265820743996,0.641165742156689,0.555265820743996,
0.641165742156689,0.555265820743996,0.641165742156689,0.555265820743996,
0.641165742156689,0.555265820743996,0.641165742156689,0.555265820743996,
0.641165742156689,0.555265820743996,0.641165742156689,0.555265820743996,
0.641165742156689,0.555265820743996,0.641165742156689,0.555265820743996,
0.641165742156689,0.555265820743996,0.641165742156689,0.555265820743996,
0.641165742156689,0.555265820743996,0.641165742156689,0.555265820743996,
0.641165742156689,0.555265820743996,0.641165742156689,0.555265820743996,
0.641165742156689,0.555265820743996,0.641165742156689,0.555265820743996,
0.641165742156689,0.555265820743996,0.641165742156689,0.555265820743996,
0.641165742156689,0.555265820743996,0.641165742156689,0.555265820743996,
0.641165742156689,0.555265820743996,0.641165742156689,0.555265820743996,
0.641165742156689,0.555265820743996,0.641165742156689,0.555265820743996,
0.641165742156689,0.555265820743996,0.641165742156689,0.555265820743996,
0.641165742156689,0.555265820743996,0.641165742156689,0.555265820743996,
0.641165742156689,0.555265820743996,0.641165742156689,0.555265820743996,
0.641165742156689,0.555265820743996,0.641165742156689,0.555265820743996,
0.641165742156689,0.555265820743996,0.641165742156689,0.555265820743996,
0.641165742156689,0.555265820743996,0.641165742156689,0.555265820743996,
0.641165742156689,0.555265820743996,0.641165742156689,0.555265820743996,
0.641165742156689,0.555265820743996,0.641165742156689,0.555265820743996,
0.641165742156689,0.555265820743996,0.641165742156689,0.555265820743996,
0.641165742156689,0.555265820743996,0.641165742156689,0.555265820743996,
0.641165742156689,0.555265820743996,0.641165742156689,0.555265820743996,
0.641165742156689,0.555265820743996,0.641165742156689,0.555265820743996,
0.641165742156689,0.555265820743996,0.641165742156689,0.555265820743996,
0.641165742156689,0.555265820743996,0.641165742156689,0.555265820743996,
0.641165742156689,0.555265820743996,0.641165742156689,0.555265820743996,
0.641165742156689,0.555265820743996,0.641165742156689,0.555265820743996,
0.641165742156689,0.555265820743996,0.641165742156689,0.555265820743996,
0.641165742156689,0.555265820743996,0.641165742156689,0.555265820743996,
0.641165742156689,0.555265820743996,0.641165742156689,0.555265820743996,
0.641165742156689,0.555265820743996,0.641165742156689,0.555265820743996,
0.641165742156689,0.555265820743996,0.641165742156689,0.555265820743996,
0.641165742156689,0.555265820743996,0.641165742156689,0.555265820743996,
0.641165742156689,0.555265820743996,0.641165742156689,0.555265820743996,
0.641165742156689,0.555265820743996,0.641165742156689,0.555265820743996,
0.641165742156689,0.555265820743996,0.641165742156689,0.555265820743996,
0.641165742156689,0.555265820743996,0.641165742156689,0.555265820743996,
0.641165742156689,0.555265820743996,0.641165742156689,0.555265820743996,
0.641165742156689,0.555265820743996,0.641165742156689,0.555265820743996,
0.641165742156689,0.555265820743996,0.641165742156689,0.555265820743996,
0.641165742156689,0.555265820743996,0.641165742156689,0.555265820743996,
0.641165742156689,0.555265820743996,0.641165742156689,0.555265820743996,
0.641165742156689,0.555265820743996,0.641165742156689,0.555265820743996,
0.641165742156689,0.555265820743996,0.641165742156689,0.555265820743996,
0.641165742156689,0.555265820743996,0.641165742156689,0.555265820743996,
0.641165742156689,0.555265820743996,0.641165742156689,0.555265820743996,
0.641165742156689,0.555265820743996,0.641165742156689,0.555265820743996,
0.641165742156689,0.555265820743996,0.641165742156689,0.555265820743996,
0.641165742156689,0.555265820743996,0.641165742156689,0.555265820743996,
0.641165742156689,0.555265820743996,0.641165742156689,0.555265820743996,
0.641165742156689,0.555265820743996,0.641165742156689,0.555265820743996,
0.641165742156689,0.555265820743996,0.641165742156689,0.555265820743996,
0.641165742156689,0.555265820743996,0.641165742156689,0.555265820743996,
0.641165742156689,0.555265820743996,0.641165742156689,0.555265820743996,
0.641165742156689,0.555265820743996,0.641165742156689,0.555265820743996,
0.641165742156689,0.555265820743996,0.641165742156689,0.555265820743996,
0.641165742156689,0.555265820743996,0.641165742156689,0.555265820743996,
0.641165742156689,0.555265820743996,0.641165742156689,0.555265820743996,
0.641165742156689,0.555265820743996,0.641165742156689,0.555265820743996,
0.641165742156689,0.555265820743996,0.641165742156689,0.555265820743996,
0.641165742156689,0.555265820743996,0.641165742156689,0.555265820743996,
0.641165742156689,0.555265820743996,0.641165742156689,0.555265820743996,
0.641165742156689,0.555265820743996,0.641165742156689,0.555265820743996,
0.641165742156689,0.555265820743996,0.641165742156689,0.555265820743996,
0.641165742156689,0.555265820743996,0.641165742156689,0.555265820743996,
0.641165742156689,0.555265820743996,0.641165742156689,0.555265820743996,
0.641165742156689,0.555265820743996,0.641165742156689,0.555265820743996,
0.641165742156689,0.555265820743996,0.641165742156689,0.555265820743996,
0.641165742156689,0.555265820743996,0.641165742156689,0.555265820743996,
0.641165742156689,0.555265820743996,0.641165742156689,0.555265820743996,
0.641165742156689,0.555265820743996,0.641165742156689,0.555265820743996,
0.641165742156689,0.555265820743996,0.641165742156689,0.555265820743996,
0.641165742156689,0.555265820743996,0.641165742156689,0.555265820743996,
0.641165742156689,0.555265820743996,0.641165742156689,0.555265820743996,
0.641165742156689,0.555265820743996,0.641165742156689,0.555265820743996,
0.641165742156689,0.555265820743996,0.641165742156689,0.555265820743996,
0.641165742156689,0.555265820743996,0.641165742156689,0.555265820743996,
0.641165742156689,0.555265820743996,0.641165742156689,0.555265820743996,
0.641165742156689,0.555265820743996,0.641165742156689,0.555265820743996,
0.641165742156689,0.555265820743996,0.641165742156689,0.555265820743996,
0.641165742156689,0.555265820743996,0.641165742156689,0.555265820743996,
0.641165742156689,0.555265820743996,0.641165742156689,0.555265820743996,
0.641165742156689,0.555265820743996,0.641165742156689,0.555265820743996,
0.641165742156689,0.555265820743996,0.641165742156689,0.555265820743996,
0.641165742156689,0.555265820743996,0.641165742156689,0.555265820743996,
0.641165742156689,0.555265820743996,0.641165742156689,0.555265820743996,
0.641165742156689,0.555265820743996,0.641165742156689,0.555265820743996,
0.641165742156689,0.555265820743996,0.641165742156689,0.555265820743996,
0.641165742156689,0.555265820743996,0.641165742156689,0.555265820743996,
0.641165742156689,0.555265820743996,0.641165742156689,0.555265820743996,
0.641165742156689,0.555265820743996,0.641165742156689,0.555265820743996,
0.641165742156689,0.555265820743996,0.641165742156689,0.555265820743996,
0.641165742156689,0.555265820743996,0.641165742156689,0.555265820743996,
0.641165742156689,0.555265820743996,0.641165742156689,0.555265820743996,
0.641165742156689,0.555265820743996,0.641165742156689,0.555265820743996,
0.641165742156689,0.555265820743996,0.641165742156689,0.555265820743996,
0.641165742156689,0.555265820743996,0.641165742156689,0.555265820743996,
0.641165742156689,0.555265820743996,0.641165742156689,0.555265820743996,
0.641165742156689,0.555265820743996,0.641165742156689,0.555265820743996,
0.641165742156689,0.555265820743996,0.641165742156689,0.555265820743996,
0.641165742156689,0.555265820743996,0.641165742156689,0.555265820743996,
0.641165742156689,0.555265820743996,0.641165742156689,0.555265820743996,
0.641165742156689,0.555265820743996,0.641165742156689,0.555265820743996,
0.641165742156689,0.555265820743996,0.641165742156689,0.555265820743996,
0.641165742156689,0.555265820743996,0.641165742156689,0.555265820743996,
0.641165742156689,0.555265820743996,0.641165742156689,0.555265820743996,
0.641165742156689,0.555265820743996,0.641165742156689,0.555265820743996,
0.641165742156689,0.555265820743996,0.641165742156689,0.555265820743996,
0.641165742156689,0.555265820743996,0.641165742156689,0.555265820743996,
0.641165742156689,0.555265820743996,0.641165742156689,0.555265820743996,
0.641165742156689,0.555265820743996,0.641165742156689,0.555265820743996,
0.641165742156689,0.555265820743996,0.641165742156689,0.555265820743996,
0.641165742156689,0.555265820743996,0.641165742156689,0.555265820743996,
0.641165742156689,0.555265820743996,0.641165742156689,0.555265820743996,
0.641165742156689,0.555265820743996,0.641165742156689,0.555265820743996,
0.641165742156689,0.555265820743996,0.641165742156689,0.555265820743996,
0.641165742156689,0.555265820743996,0.641165742156689,0.555265820743996,
0.641165742156689,0.555265820743996,0.641165742156689,0.555265820743996,
0.641165742156689),(0.641165742156689,0.555265820743996,0.641165742156689,
0.555265820743996,0.641165742156689,0.555265820743996,0.641165742156689,
0.555265820743996,0.641165742156689,0.555265820743996,0.641165742156689,
0.555265820743996,0.641165742156689,0.555265820743996,0.641165742156689,
0.555265820743996,0.641165742156689,0.555265820743996,0.641165742156689,
0.555265820743996,0.641165742156689,0.555265820743996,0.641165742156689,
0.555265820743996,0.641165742156689,0.555265820743996,0.641165742156689,
0.555265820743996,0.641165742156689,0.555265820743996,0.641165742156689,
0.555265820743996,0.641165742156689,0.555265820743996,0.641165742156689,
0.555265820743996,0.641165742156689,0.555265820743996,0.641165742156689,
0.555265820743996,0.641165742156689,0.555265820743996,0.641165742156689,
0.555265820743996,0.641165742156689,0.555265820743996,0.641165742156689,
0.555265820743996,0.641165742156689,0.555265820743996,0.641165742156689,
0.555265820743996,0.641165742156689,0.555265820743996,0.641165742156689,
0.555265820743996,0.641165742156689,0.555265820743996,0.641165742156689,
0.555265820743996,0.641165742156689,0.555265820743996,0.641165742156689,
0.555265820743996,0.641165742156689,0.555265820743996,0.641165742156689,
0.555265820743996,0.641165742156689,0.555265820743996,0.641165742156689,
0.555265820743996,0.641165742156689,0.555265820743996,0.641165742156689,
0.555265820743996,0.641165742156689,0.555265820743996,0.641165742156689,
0.555265820743996,0.641165742156689,0.555265820743996,0.641165742156689,
0.555265820743996,0.641165742156689,0.555265820743996,0.641165742156689,
0.555265820743996,0.641165742156689,0.555265820743996,0.641165742156689,
0.555265820743996,0.641165742156689,0.555265820743996,0.641165742156689,
0.555265820743996,0.641165742156689,0.555265820743996,0.641165742156689,
0.555265820743996,0.641165742156689,0.555265820743996,0.641165742156689,
0.555265820743996,0.641165742156689,0.555265820743996,0.641165742156689,
0.555265820743996,0.641165742156689,0.555265820743996,0.641165742156689,
0.555265820743996,0.641165742156689,0.555265820743996,0.641165742156689,
0.555265820743996,0.641165742156689,0.555265820743996,0.641165742156689,
0.555265820743996,0.641165742156689,0.555265820743996,0.641165742156689,
0.555265820743996,0.641165742156689,0.555265820743996,0.641165742156689,
0.555265820743996,0.641165742156689,0.555265820743996,0.641165742156689,
0.555265820743996,0.641165742156689,0.555265820743996,0.641165742156689,
0.555265820743996,0.641165742156689,0.555265820743996,0.641165742156689,
0.555265820743996,0.641165742156689,0.555265820743996,0.641165742156689,
0.555265820743996,0.641165742156689,0.555265820743996,0.641165742156689,
0.555265820743996,0.641165742156689,0.555265820743996,0.641165742156689,
0.555265820743996,0.641165742156689,0.555265820743996,0.641165742156689,
0.555265820743996,0.641165742156689,0.555265820743996,0.641165742156689,
0.555265820743996,0.641165742156689,0.555265820743996,0.641165742156689,
0.555265820743996,0.641165742156689,0.555265820743996,0.641165742156689,
0.555265820743996,0.641165742156689,0.555265820743996,0.641165742156689,
0.555265820743996,0.641165742156689,0.555265820743996,0.641165742156689,
0.555265820743996,0.641165742156689,0.555265820743996,0.641165742156689,
0.555265820743996,0.641165742156689,0.555265820743996,0.641165742156689,
0.555265820743996,0.641165742156689,0.555265820743996,0.641165742156689,
0.555265820743996,0.641165742156689,0.555265820743996,0.641165742156689,
0.555265820743996,0.641165742156689,0.555265820743996,0.641165742156689,
0.555265820743996,0.641165742156689,0.555265820743996,0.641165742156689,
0.555265820743996,0.641165742156689,0.555265820743996,0.641165742156689,
0.555265820743996,0.641165742156689,0.555265820743996,0.641165742156689,
0.555265820743996,0.641165742156689,0.555265820743996,0.641165742156689,
0.555265820743996,0.641165742156689,0.555265820743996,0.641165742156689,
0.555265820743996,0.641165742156689,0.555265820743996,0.641165742156689,
0.555265820743996,0.641165742156689,0.555265820743996,0.641165742156689,
0.555265820743996,0.641165742156689,0.555265820743996,0.641165742156689,
0.555265820743996,0.641165742156689,0.555265820743996,0.641165742156689,
0.555265820743996,0.641165742156689,0.555265820743996,0.641165742156689,
0.555265820743996,0.641165742156689,0.555265820743996,0.641165742156689,
0.555265820743996,0.641165742156689,0.555265820743996,0.641165742156689,
0.555265820743996,0.641165742156689,0.555265820743996,0.641165742156689,
0.555265820743996,0.641165742156689,0.555265820743996,0.641165742156689,
0.555265820743996,0.641165742156689,0.555265820743996,0.641165742156689,
0.555265820743996,0.641165742156689,0.555265820743996,0.641165742156689,
0.555265820743996,0.641165742156689,0.555265820743996,0.641165742156689,
0.555265820743996,0.641165742156689,0.555265820743996,0.641165742156689,
0.555265820743996,0.641165742156689,0.555265820743996,0.641165742156689,
0.555265820743996,0.641165742156689,0.555265820743996,0.641165742156689,
0.555265820743996,0.641165742156689,0.555265820743996,0.641165742156689,
0.555265820743996,0.641165742156689,0.555265820743996,0.641165742156689,
0.555265820743996,0.641165742156689,0.555265820743996,0.641165742156689,
0.555265820743996,0.641165742156689,0.555265820743996,0.641165742156689,
0.555265820743996,0.641165742156689,0.555265820743996,0.641165742156689,
0.555265820743996,0.641165742156689,0.555265820743996,0.641165742156689,
0.555265820743996,0.641165742156689,0.555265820743996,0.641165742156689,
0.555265820743996,0.641165742156689,0.555265820743996,0.641165742156689,
0.555265820743996,0.641165742156689,0.555265820743996,0.641165742156689,
0.555265820743996,0.641165742156689,0.555265820743996,0.641165742156689,
0.555265820743996,0.641165742156689,0.555265820743996,0.641165742156689,
0.555265820743996,0.641165742156689,0.555265820743996,0.641165742156689,
0.555265820743996,0.641165742156689,0.555265820743996,0.641165742156689,
0.555265820743996,0.641165742156689,0.555265820743996,0.641165742156689,
0.555265820743996,0.641165742156689,0.555265820743996,0.641165742156689,
0.555265820743996,0.641165742156689,0.555265820743996,0.641165742156689,
0.555265820743996,0.641165742156689,0.555265820743996,0.641165742156689,
0.555265820743996,0.641165742156689,0.555265820743996,0.641165742156689,
0.555265820743996,0.641165742156689,0.555265820743996,0.641165742156689,
0.555265820743996,0.641165742156689,0.555265820743996,0.641165742156689,
0.555265820743996,0.641165742156689,0.555265820743996,0.641165742156689,
0.555265820743996,0.641165742156689,0.555265820743996,0.641165742156689,
0.555265820743996,0.641165742156689,0.555265820743996,0.641165742156689,
0.555265820743996,0.641165742156689,0.555265820743996,0.641165742156689,
0.555265820743996,0.641165742156689,0.555265820743996,0.641165742156689,
0.555265820743996,0.641165742156689,0.555265820743996,0.641165742156689,
0.555265820743996,0.641165742156689,0.555265820743996,0.641165742156689,
0.555265820743996,0.641165742156689,0.555265820743996,0.641165742156689,
0.555265820743996,0.641165742156689,0.555265820743996,0.641165742156689,
0.555265820743996,0.641165742156689,0.555265820743996,0.641165742156689,
0.555265820743996,0.641165742156689,0.555265820743996,0.641165742156689,
0.555265820743996,0.641165742156689,0.555265820743996,0.641165742156689,
0.555265820743996,0.641165742156689,0.555265820743996,0.641165742156689,
0.555265820743996,0.641165742156689,0.555265820743996,0.641165742156689,
0.555265820743996,0.641165742156689,0.555265820743996,0.641165742156689,
0.555265820743996,0.641165742156689,0.555265820743996,0.641165742156689,
0.555265820743996,0.641165742156689,0.555265820743996,0.641165742156689,
0.555265820743996,0.641165742156689,0.555265820743996,0.641165742156689,
0.555265820743996,0.641165742156689,0.555265820743996,0.641165742156689,
0.555265820743996,0.641165742156689,0.555265820743996,0.641165742156689,
0.555265820743996,0.641165742156689,0.555265820743996,0.641165742156689,
0.555265820743996,0.641165742156689,0.555265820743996,0.641165742156689,
0.555265820743996,0.641165742156689,0.555265820743996,0.641165742156689,
0.555265820743996,0.641165742156689,0.555265820743996,0.641165742156689,
0.555265820743996,0.641165742156689,0.555265820743996,0.641165742156689,
0.555265820743996,0.641165742156689,0.555265820743996,0.641165742156689,
0.555265820743996,0.641165742156689,0.555265820743996,0.641165742156689,
0.555265820743996,0.641165742156689,0.555265820743996,0.641165742156689,
0.555265820743996,0.641165742156689,0.555265820743996,0.641165742156689,
0.555265820743996,0.641165742156689,0.555265820743996,0.641165742156689,
0.555265820743996,0.641165742156689,0.555265820743996,0.641165742156689,
0.555265820743996,0.641165742156689,0.555265820743996,0.641165742156689,
0.555265820743996,0.641165742156689,0.555265820743996,0.641165742156689,
0.555265820743996,0.641165742156689,0.555265820743996,0.641165742156689,
0.555265820743996,0.641165742156689,0.555265820743996,0.641165742156689,
0.555265820743996,0.641165742156689,0.555265820743996,0.641165742156689,
0.555265820743996,0.641165742156689,0.555265820743996,0.641165742156689,
0.555265820743996,0.641165742156689,0.555265820743996,0.641165742156689,
0.555265820743996,0.641165742156689,0.555265820743996,0.641165742156689,
0.555265820743996,0.641165742156689,0.555265820743996,0.641165742156689,
0.555265820743996,0.641165742156689,0.555265820743996,0.641165742156689,
0.555265820743996,0.641165742156689,0.555265820743996,0.641165742156689,
0.555265820743996,0.641165742156689,0.555265820743996,0.641165742156689,
0.555265820743996,0.641165742156689,0.555265820743996,0.641165742156689,
0.555265820743996,0.641165742156689,0.555265820743996,0.641165742156689,
0.555265820743996,0.641165742156689,0.555265820743996,0.641165742156689,
0.555265820743996,0.641165742156689,0.555265820743996,0.641165742156689,
0.555265820743996,0.641165742156689,0.555265820743996,0.641165742156689,
0.555265820743996,0.641165742156689,0.555265820743996,0.641165742156689,
0.555265820743996,0.641165742156689,0.555265820743996,0.641165742156689,
0.555265820743996,0.641165742156689,0.555265820743996,0.641165742156689,
0.555265820743996,0.641165742156689,0.555265820743996,0.641165742156689,
0.555265820743996,0.641165742156689,0.555265820743996,0.641165742156689,
0.555265820743996,0.641165742156689,0.555265820743996,0.641165742156689,
0.555265820743996,0.641165742156689,0.555265820743996,0.641165742156689,
0.555265820743996,0.641165742156689,0.555265820743996,0.641165742156689,
0.555265820743996,0.641165742156689,0.555265820743996,0.641165742156689,
0.555265820743996,0.641165742156689,0.555265820743996,0.641165742156689,
0.555265820743996,0.641165742156689,0.555265820743996,0.641165742156689,
0.555265820743996,0.641165742156689,0.555265820743996,0.641165742156689,
0.555265820743996,0.641165742156689,0.555265820743996,0.641165742156689,
0.555265820743996,0.641165742156689,0.555265820743996,0.641165742156689,
0.555265820743996,0.641165742156689,0.555265820743996,0.641165742156689,
0.555265820743996,0.641165742156689,0.555265820743996,0.641165742156689,
0.555265820743996,0.641165742156689,0.555265820743996,0.641165742156689,
0.555265820743996,0.641165742156689,0.555265820743996,0.641165742156689,
0.555265820743996,0.641165742156689,0.555265820743996,0.641165742156689,
0.555265820743996,0.641165742156689,0.555265820743996,0.641165742156689,
0.555265820743996,0.641165742156689,0.555265820743996,0.641165742156689,
0.555265820743996,0.641165742156689,0.555265820743996,0.641165742156689,
0.555265820743996,0.641165742156689,0.555265820743996,0.641165742156689,
0.555265820743996,0.641165742156689,0.555265820743996,0.641165742156689,
0.555265820743996,0.641165742156689,0.555265820743996,0.641165742156689,
0.555265820743996,0.641165742156689,0.555265820743996,0.641165742156689,
0.555265820743996,0.641165742156689,0.555265820743996,0.641165742156689,
0.555265820743996,0.641165742156689,0.555265820743996,0.641165742156689,
0.555265820743996,0.641165742156689,0.555265820743996,0.641165742156689,
0.555265820743996,0.641165742156689,0.555265820743996,0.641165742156689,
0.555265820743996,0.641165742156689,0.555265820743996,0.641165742156689,
0.555265820743996,0.641165742156689,0.555265820743996,0.641165742156689,
0.555265820743996,0.641165742156689,0.555265820743996,0.641165742156689,
0.555265820743996,0.641165742156689,0.555265820743996,0.641165742156689,
0.555265820743996,0.641165742156689,0.555265820743996,0.641165742156689,
0.555265820743996,0.641165742156689,0.555265820743996,0.641165742156689,
0.555265820743996,0.641165742156689,0.555265820743996,0.641165742156689,
0.555265820743996,0.641165742156689,0.555265820743996,0.641165742156689,
0.555265820743996,0.641165742156689,0.555265820743996,0.641165742156689,
0.555265820743996,0.641165742156689,0.555265820743996,0.641165742156689,
0.555265820743996,0.641165742156689,0.555265820743996,0.641165742156689,
0.555265820743996,0.641165742156689,0.555265820743996,0.641165742156689,
0.555265820743996,0.641165742156689,0.555265820743996,0.641165742156689,
0.555265820743996,0.641165742156689,0.555265820743996,0.641165742156689,
0.555265820743996,0.641165742156689,0.555265820743996,0.641165742156689,
0.555265820743996,0.641165742156689,0.555265820743996,0.641165742156689,
0.555265820743996,0.641165742156689,0.555265820743996,0.641165742156689,
0.555265820743996,0.641165742156689,0.555265820743996,0.641165742156689,
0.555265820743996,0.641165742156689,0.555265820743996,0.641165742156689,
0.555265820743996,0.641165742156689,0.555265820743996,0.641165742156689,
0.555265820743996,0.641165742156689,0.555265820743996,0.641165742156689,
0.555265820743996,0.641165742156689,0.555265820743996,0.641165742156689,
0.555265820743996,0.641165742156689,0.555265820743996,0.641165742156689,
0.555265820743996,0.641165742156689,0.555265820743996,0.641165742156689,
0.555265820743996,0.641165742156689,0.555265820743996,0.641165742156689,
0.555265820743996,0.641165742156689,0.555265820743996,0.641165742156689,
0.555265820743996,0.641165742156689,0.555265820743996,0.641165742156689,
0.555265820743996,0.641165742156689,0.555265820743996,0.641165742156689,
0.555265820743996,0.641165742156689,0.555265820743996,0.641165742156689,
0.555265820743996,0.641165742156689,0.555265820743996,0.641165742156689,
0.555265820743996,0.641165742156689,0.555265820743996,0.641165742156689,
0.555265820743996,0.641165742156689,0.555265820743996,0.641165742156689,
0.555265820743996,0.641165742156689,0.555265820743996,0.641165742156689,
0.555265820743996,0.641165742156689,0.555265820743996,0.641165742156689,
0.555265820743996,0.641165742156689,0.555265820743996,0.641165742156689,
0.555265820743996,0.641165742156689,0.555265820743996,0.641165742156689,
0.555265820743996,0.641165742156689,0.555265820743996,0.641165742156689,
0.555265820743996,0.641165742156689,0.555265820743996,0.641165742156689,
0.555265820743996,0.641165742156689,0.555265820743996,0.641165742156689,
0.555265820743996,0.641165742156689,0.555265820743996,0.641165742156689,
0.555265820743996,0.641165742156689,0.555265820743996,0.641165742156689,
0.555265820743996,0.641165742156689,0.555265820743996,0.641165742156689,
0.555265820743996,0.641165742156689,0.555265820743996,0.641165742156689,
0.555265820743996,0.641165742156689,0.555265820743996,0.641165742156689,
0.555265820743996,0.641165742156689,0.555265820743996,0.641165742156689,
0.555265820743996,0.641165742156689,0.555265820743996,0.641165742156689,
0.555265820743996,0.641165742156689,0.555265820743996,0.641165742156689,
0.555265820743996,0.641165742156689,0.555265820743996,0.641165742156689,
0.555265820743996,0.641165742156689,0.555265820743996,0.641165742156689,
0.555265820743996,0.641165742156689,0.555265820743996,0.641165742156689,
0.555265820743996,0.641165742156689,0.555265820743996,0.641165742156689,
0.555265820743996,0.641165742156689,0.555265820743996,0.641165742156689,
0.555265820743996,0.641165742156689,0.555265820743996,0.641165742156689,
0.555265820743996,0.641165742156689,0.555265820743996,0.641165742156689,
0.555265820743996,0.641165742156689,0.555265820743996,0.641165742156689,
0.555265820743996,0.641165742156689,0.555265820743996,0.641165742156689,
0.555265820743996,0.641165742156689,0.555265820743996,0.641165742156689,
0.555265820743996,0.641165742156689,0.555265820743996,0.641165742156689,
0.555265820743996,0.641165742156689,0.555265820743996,0.641165742156689,
0.555265820743996,0.641165742156689,0.555265820743996,0.641165742156689,
0.555265820743996,0.641165742156689,0.555265820743996,0.641165742156689,
0.555265820743996,0.641165742156689,0.555265820743996,0.641165742156689,
0.555265820743996,0.641165742156689,0.555265820743996,0.641165742156689,
0.555265820743996,0.641165742156689,0.555265820743996,0.641165742156689,
0.555265820743996,0.641165742156689,0.555265820743996,0.641165742156689,
0.555265820743996,0.641165742156689,0.555265820743996,0.641165742156689,
0.555265820743996,0.641165742156689,0.555265820743996,0.641165742156689,
0.555265820743996,0.641165742156689,0.555265820743996,0.641165742156689,
0.555265820743996,0.641165742156689,0.555265820743996,0.641165742156689,
0.555265820743996,0.641165742156689,0.555265820743996,0.641165742156689,
0.555265820743996,0.641165742156689,0.555265820743996,0.641165742156689,
0.555265820743996,0.641165742156689,0.555265820743996,0.641165742156689,
0.555265820743996,0.641165742156689,0.555265820743996,0.641165742156689,
0.555265820743996,0.641165742156689,0.555265820743996,0.641165742156689,
0.555265820743996,0.641165742156689,0.555265820743996,0.641165742156689,
0.555265820743996,0.641165742156689,0.555265820743996,0.641165742156689,
0.555265820743996,0.641165742156689),(1.,0.866025403784439,1.,0.866025403784439,
1.,0.866025403784439,1.,0.866025403784439,1.,0.866025403784439,1.,0.866025403784439,
1.,0.866025403784439,1.,0.866025403784439,1.,0.866025403784439,1.,0.866025403784439,
1.,0.866025403784439,1.,0.866025403784439,1.,0.866025403784439,1.,0.866025403784439,
1.,0.866025403784439,1.,0.866025403784439,1.,0.866025403784439,1.,0.866025403784439,
1.,0.866025403784439,1.,0.866025403784439,1.,0.866025403784439,1.,0.866025403784439,
1.,0.866025403784439,1.,0.866025403784439,1.,0.866025403784439,1.,0.866025403784439,
1.,0.866025403784439,1.,0.866025403784439,1.,0.866025403784439,1.,0.866025403784439,
1.,0.866025403784439,1.,0.866025403784439,1.,0.866025403784439,1.,0.866025403784439,
1.,0.866025403784439,1.,0.866025403784439,1.,0.866025403784439,1.,0.866025403784439,
1.,0.866025403784439,1.,0.866025403784439,1.,0.866025403784439,1.,0.866025403784439,
1.,0.866025403784439,1.,0.866025403784439,1.,0.866025403784439,1.,0.866025403784439,
1.,0.866025403784439,1.,0.866025403784439,1.,0.866025403784439,1.,0.866025403784439,
1.,0.866025403784439,1.,0.866025403784439,1.,0.866025403784439,1.,0.866025403784439,
1.,0.866025403784439,1.,0.866025403784439,1.,0.866025403784439,1.,0.866025403784439,
1.,0.866025403784439,1.,0.866025403784439,1.,0.866025403784439,1.,0.866025403784439,
1.,0.866025403784439,1.,0.866025403784439,1.,0.866025403784439,1.,0.866025403784439,
1.,0.866025403784439,1.,0.866025403784439,1.,0.866025403784439,1.,0.866025403784439,
1.,0.866025403784439,1.,0.866025403784439,1.,0.866025403784439,1.,0.866025403784439,
1.,0.866025403784439,1.,0.866025403784439,1.,0.866025403784439,1.,0.866025403784439,
1.,0.866025403784439,1.,0.866025403784439,1.,0.866025403784439,1.,0.866025403784439,
1.,0.866025403784439,1.,0.866025403784439,1.,0.866025403784439,1.,0.866025403784439,
1.,0.866025403784439,1.,0.866025403784439,1.,0.866025403784439,1.,0.866025403784439,
1.,0.866025403784439,1.,0.866025403784439,1.,0.866025403784439,1.,0.866025403784439,
1.,0.866025403784439,1.,0.866025403784439,1.,0.866025403784439,1.,0.866025403784439,
1.,0.866025403784439,1.,0.866025403784439,1.,0.866025403784439,1.,0.866025403784439,
1.,0.866025403784439,1.,0.866025403784439,1.,0.866025403784439,1.,0.866025403784439,
1.,0.866025403784439,1.,0.866025403784439,1.,0.866025403784439,1.,0.866025403784439,
1.,0.866025403784439,1.,0.866025403784439,1.,0.866025403784439,1.,0.866025403784439,
1.,0.866025403784439,1.,0.866025403784439,1.,0.866025403784439,1.,0.866025403784439,
1.,0.866025403784439,1.,0.866025403784439,1.,0.866025403784439,1.,0.866025403784439,
1.,0.866025403784439,1.,0.866025403784439,1.,0.866025403784439,1.,0.866025403784439,
1.,0.866025403784439,1.,0.866025403784439,1.,0.866025403784439,1.,0.866025403784439,
1.,0.866025403784439,1.,0.866025403784439,1.,0.866025403784439,1.,0.866025403784439,
1.,0.866025403784439,1.,0.866025403784439,1.,0.866025403784439,1.,0.866025403784439,
1.,0.866025403784439,1.,0.866025403784439,1.,0.866025403784439,1.,0.866025403784439,
1.,0.866025403784439,1.,0.866025403784439,1.,0.866025403784439,1.,0.866025403784439,
1.,0.866025403784439,1.,0.866025403784439,1.,0.866025403784439,1.,0.866025403784439,
1.,0.866025403784439,1.,0.866025403784439,1.,0.866025403784439,1.,0.866025403784439,
1.,0.866025403784439,1.,0.866025403784439,1.,0.866025403784439,1.,0.866025403784439,
1.,0.866025403784439,1.,0.866025403784439,1.,0.866025403784439,1.,0.866025403784439,
1.,0.866025403784439,1.,0.866025403784439,1.,0.866025403784439,1.,0.866025403784439,
1.,0.866025403784439,1.,0.866025403784439,1.,0.866025403784439,1.,0.866025403784439,
1.,0.866025403784439,1.,0.866025403784439,1.,0.866025403784439,1.,0.866025403784439,
1.,0.866025403784439,1.,0.866025403784439,1.,0.866025403784439,1.,0.866025403784439,
1.,0.866025403784439,1.,0.866025403784439,1.,0.866025403784439,1.,0.866025403784439,
1.,0.866025403784439,1.,0.866025403784439,1.,0.866025403784439,1.,0.866025403784439,
1.,0.866025403784439,1.,0.866025403784439,1.,0.866025403784439,1.,0.866025403784439,
1.,0.866025403784439,1.,0.866025403784439,1.,0.866025403784439,1.,0.866025403784439,
1.,0.866025403784439,1.,0.866025403784439,1.,0.866025403784439,1.,0.866025403784439,
1.,0.866025403784439,1.,0.866025403784439,1.,0.866025403784439,1.,0.866025403784439,
1.,0.866025403784439,1.,0.866025403784439,1.,0.866025403784439,1.,0.866025403784439,
1.,0.866025403784439,1.,0.866025403784439,1.,0.866025403784439,1.,0.866025403784439,
1.,0.866025403784439,1.,0.866025403784439,1.,0.866025403784439,1.,0.866025403784439,
1.,0.866025403784439,1.,0.866025403784439,1.,0.866025403784439,1.,0.866025403784439,
1.,0.866025403784439,1.,0.866025403784439,1.,0.866025403784439,1.,0.866025403784439,
1.,0.866025403784439,1.,0.866025403784439,1.,0.866025403784439,1.,0.866025403784439,
1.,0.866025403784439,1.,0.866025403784439,1.,0.866025403784439,1.,0.866025403784439,
1.,0.866025403784439,1.,0.866025403784439,1.,0.866025403784439,1.,0.866025403784439,
1.,0.866025403784439,1.,0.866025403784439,1.,0.866025403784439,1.,0.866025403784439,
1.,0.866025403784439,1.,0.866025403784439,1.,0.866025403784439,1.,0.866025403784439,
1.,0.866025403784439,1.,0.866025403784439,1.,0.866025403784439,1.,0.866025403784439,
1.,0.866025403784439,1.,0.866025403784439,1.,0.866025403784439,1.,0.866025403784439,
1.,0.866025403784439,1.,0.866025403784439,1.,0.866025403784439,1.,0.866025403784439,
1.,0.866025403784439,1.,0.866025403784439,1.,0.866025403784439,1.,0.866025403784439,
1.,0.866025403784439,1.,0.866025403784439,1.,0.866025403784439,1.,0.866025403784439,
1.,0.866025403784439,1.,0.866025403784439,1.,0.866025403784439,1.,0.866025403784439,
1.,0.866025403784439,1.,0.866025403784439,1.,0.866025403784439,1.,0.866025403784439,
1.,0.866025403784439,1.,0.866025403784439,1.,0.866025403784439,1.,0.866025403784439,
1.,0.866025403784439,1.,0.866025403784439,1.,0.866025403784439,1.,0.866025403784439,
1.,0.866025403784439,1.,0.866025403784439,1.,0.866025403784439,1.,0.866025403784439,
1.,0.866025403784439,1.,0.866025403784439,1.,0.866025403784439,1.,0.866025403784439,
1.,0.866025403784439,1.,0.866025403784439,1.,0.866025403784439,1.,0.866025403784439,
1.,0.866025403784439,1.,0.866025403784439,1.,0.866025403784439,1.,0.866025403784439,
1.,0.866025403784439,1.,0.866025403784439,1.,0.866025403784439,1.,0.866025403784439,
1.,0.866025403784439,1.,0.866025403784439,1.,0.866025403784439,1.,0.866025403784439,
1.,0.866025403784439,1.,0.866025403784439,1.,0.866025403784439,1.,0.866025403784439,
1.,0.866025403784439,1.,0.866025403784439,1.,0.866025403784439,1.,0.866025403784439,
1.,0.866025403784439,1.,0.866025403784439,1.,0.866025403784439,1.,0.866025403784439,
1.,0.866025403784439,1.,0.866025403784439,1.,0.866025403784439,1.,0.866025403784439,
1.,0.866025403784439,1.,0.866025403784439,1.,0.866025403784439,1.,0.866025403784439,
1.,0.866025403784439,1.,0.866025403784439,1.,0.866025403784439,1.,0.866025403784439,
1.,0.866025403784439,1.,0.866025403784439,1.,0.866025403784439,1.,0.866025403784439,
1.,0.866025403784439,1.,0.866025403784439,1.,0.866025403784439,1.,0.866025403784439,
1.,0.866025403784439,1.,0.866025403784439,1.,0.866025403784439,1.,0.866025403784439,
1.,0.866025403784439,1.,0.866025403784439,1.,0.866025403784439,1.,0.866025403784439,
1.,0.866025403784439,1.,0.866025403784439,1.,0.866025403784439,1.,0.866025403784439,
1.,0.866025403784439,1.,0.866025403784439,1.,0.866025403784439,1.,0.866025403784439,
1.,0.866025403784439,1.,0.866025403784439,1.,0.866025403784439,1.,0.866025403784439,
1.,0.866025403784439,1.,0.866025403784439,1.,0.866025403784439,1.,0.866025403784439,
1.,0.866025403784439,1.,0.866025403784439,1.,0.866025403784439,1.,0.866025403784439,
1.,0.866025403784439,1.,0.866025403784439,1.,0.866025403784439,1.,0.866025403784439,
1.,0.866025403784439,1.,0.866025403784439,1.,0.866025403784439,1.,0.866025403784439,
1.,0.866025403784439,1.,0.866025403784439,1.,0.866025403784439,1.,0.866025403784439,
1.,0.866025403784439,1.,0.866025403784439,1.,0.866025403784439,1.,0.866025403784439,
1.,0.866025403784439,1.,0.866025403784439,1.,0.866025403784439,1.,0.866025403784439,
1.,0.866025403784439,1.,0.866025403784439,1.,0.866025403784439,1.,0.866025403784439,
1.,0.866025403784439,1.,0.866025403784439,1.,0.866025403784439,1.,0.866025403784439,
1.,0.866025403784439,1.,0.866025403784439,1.,0.866025403784439,1.,0.866025403784439,
1.,0.866025403784439,1.,0.866025403784439,1.,0.866025403784439,1.,0.866025403784439,
1.,0.866025403784439,1.,0.866025403784439,1.,0.866025403784439,1.,0.866025403784439,
1.,0.866025403784439,1.,0.866025403784439,1.,0.866025403784439,1.,0.866025403784439,
1.,0.866025403784439,1.,0.866025403784439,1.,0.866025403784439,1.,0.866025403784439,
1.,0.866025403784439,1.,0.866025403784439,1.,0.866025403784439,1.,0.866025403784439,
1.,0.866025403784439,1.,0.866025403784439,1.,0.866025403784439,1.,0.866025403784439,
1.,0.866025403784439,1.,0.866025403784439,1.,0.866025403784439,1.,0.866025403784439,
1.,0.866025403784439,1.,0.866025403784439,1.,0.866025403784439,1.,0.866025403784439,
1.,0.866025403784439,1.,0.866025403784439,1.,0.866025403784439,1.,0.866025403784439,
1.,0.866025403784439,1.,0.866025403784439,1.,0.866025403784439,1.,0.866025403784439,
1.,0.866025403784439,1.,0.866025403784439,1.,0.866025403784439,1.,0.866025403784439,
1.,0.866025403784439,1.,0.866025403784439,1.,0.866025403784439,1.,0.866025403784439,
1.,0.866025403784439,1.,0.866025403784439,1.,0.866025403784439,1.,0.866025403784439,
1.,0.866025403784439,1.,0.866025403784439,1.,0.866025403784439,1.,0.866025403784439,
1.,0.866025403784439,1.,0.866025403784439,1.,0.866025403784439,1.,0.866025403784439,
1.,0.866025403784439,1.,0.866025403784439,1.,0.866025403784439,1.,0.866025403784439,
1.,0.866025403784439,1.,0.866025403784439,1.,0.866025403784439,1.,0.866025403784439,
1.,0.866025403784439,1.,0.866025403784439,1.,0.866025403784439,1.,0.866025403784439,
1.,0.866025403784439,1.,0.866025403784439,1.,0.866025403784439,1.,0.866025403784439,
1.,0.866025403784439,1.,0.866025403784439,1.,0.866025403784439,1.,0.866025403784439,
1.,0.866025403784439,1.,0.866025403784439,1.,0.866025403784439,1.,0.866025403784439,
1.,0.866025403784439,1.,0.866025403784439,1.,0.866025403784439,1.,0.866025403784439,
1.,0.866025403784439,1.,0.866025403784439,1.,0.866025403784439,1.,0.866025403784439,
1.)))
REPRESENTATION_ITEM('')
SURFACE()
);
#150=(
BOUNDED_SURFACE()
B_SPLINE_SURFACE(1,2,((#19439,#19440,#19441,#19442,#19443,#19444,#19445,
#19446,#19447,#19448,#19449,#19450,#19451,#19452,#19453,#19454,#19455,#19456,
#19457,#19458,#19459,#19460,#19461,#19462,#19463,#19464,#19465,#19466,#19467,
#19468,#19469,#19470,#19471,#19472,#19473,#19474,#19475,#19476,#19477,#19478,
#19479,#19480,#19481,#19482,#19483,#19484,#19485,#19486,#19487,#19488,#19489,
#19490,#19491,#19492,#19493,#19494,#19495,#19496,#19497,#19498,#19499,#19500,
#19501,#19502,#19503,#19504,#19505,#19506,#19507,#19508,#19509,#19510,#19511,
#19512,#19513,#19514,#19515,#19516,#19517,#19518,#19519,#19520,#19521,#19522,
#19523,#19524,#19525,#19526,#19527,#19528,#19529,#19530,#19531,#19532,#19533,
#19534,#19535,#19536,#19537,#19538,#19539,#19540,#19541,#19542,#19543,#19544,
#19545,#19546,#19547,#19548,#19549,#19550,#19551,#19552,#19553,#19554,#19555,
#19556,#19557,#19558,#19559,#19560,#19561,#19562,#19563,#19564,#19565,#19566,
#19567,#19568,#19569,#19570,#19571,#19572,#19573,#19574,#19575,#19576,#19577,
#19578,#19579,#19580,#19581,#19582,#19583,#19584,#19585,#19586,#19587,#19588,
#19589,#19590,#19591,#19592,#19593,#19594,#19595,#19596,#19597,#19598,#19599,
#19600,#19601,#19602,#19603,#19604,#19605,#19606,#19607,#19608,#19609,#19610,
#19611,#19612,#19613,#19614,#19615,#19616,#19617,#19618,#19619,#19620,#19621,
#19622,#19623,#19624,#19625,#19626,#19627,#19628,#19629,#19630,#19631,#19632,
#19633,#19634,#19635,#19636,#19637,#19638,#19639,#19640,#19641,#19642,#19643,
#19644,#19645,#19646,#19647,#19648,#19649,#19650,#19651,#19652,#19653,#19654,
#19655,#19656,#19657,#19658,#19659,#19660,#19661,#19662,#19663,#19664,#19665,
#19666,#19667,#19668,#19669,#19670,#19671,#19672,#19673,#19674,#19675,#19676,
#19677,#19678,#19679,#19680,#19681,#19682,#19683,#19684,#19685,#19686,#19687,
#19688,#19689,#19690,#19691,#19692,#19693,#19694,#19695,#19696,#19697,#19698,
#19699,#19700,#19701,#19702,#19703,#19704,#19705,#19706,#19707,#19708,#19709,
#19710,#19711,#19712,#19713,#19714,#19715,#19716,#19717,#19718,#19719,#19720,
#19721,#19722,#19723,#19724,#19725,#19726,#19727,#19728,#19729,#19730,#19731,
#19732,#19733,#19734,#19735,#19736,#19737,#19738,#19739,#19740,#19741,#19742,
#19743,#19744,#19745,#19746,#19747,#19748,#19749,#19750,#19751,#19752,#19753,
#19754,#19755,#19756,#19757,#19758,#19759,#19760,#19761,#19762,#19763,#19764,
#19765,#19766,#19767,#19768,#19769,#19770,#19771,#19772,#19773,#19774,#19775,
#19776,#19777,#19778,#19779,#19780,#19781,#19782,#19783,#19784,#19785,#19786,
#19787,#19788,#19789,#19790,#19791,#19792,#19793,#19794,#19795,#19796,#19797,
#19798,#19799,#19800,#19801,#19802,#19803,#19804,#19805,#19806,#19807,#19808,
#19809,#19810,#19811,#19812,#19813,#19814,#19815,#19816,#19817,#19818,#19819,
#19820,#19821,#19822,#19823,#19824,#19825,#19826,#19827,#19828,#19829,#19830,
#19831,#19832,#19833,#19834,#19835,#19836,#19837,#19838,#19839,#19840,#19841,
#19842,#19843,#19844,#19845,#19846,#19847,#19848,#19849,#19850,#19851,#19852,
#19853,#19854,#19855,#19856,#19857,#19858,#19859,#19860,#19861,#19862,#19863,
#19864,#19865,#19866,#19867,#19868,#19869,#19870,#19871,#19872,#19873,#19874,
#19875,#19876,#19877,#19878,#19879,#19880,#19881,#19882,#19883,#19884,#19885,
#19886,#19887,#19888,#19889,#19890,#19891,#19892,#19893,#19894,#19895,#19896,
#19897,#19898,#19899,#19900,#19901,#19902,#19903,#19904,#19905,#19906,#19907,
#19908,#19909,#19910,#19911,#19912,#19913,#19914,#19915,#19916,#19917,#19918,
#19919,#19920,#19921,#19922,#19923,#19924,#19925,#19926,#19927,#19928,#19929,
#19930,#19931,#19932,#19933,#19934,#19935,#19936,#19937,#19938,#19939,#19940,
#19941,#19942,#19943,#19944,#19945,#19946,#19947,#19948,#19949,#19950,#19951,
#19952,#19953,#19954,#19955,#19956,#19957,#19958,#19959,#19960,#19961,#19962,
#19963,#19964,#19965,#19966,#19967,#19968,#19969,#19970,#19971,#19972,#19973,
#19974,#19975,#19976,#19977,#19978,#19979,#19980,#19981,#19982,#19983,#19984,
#19985,#19986,#19987,#19988,#19989,#19990,#19991,#19992,#19993,#19994,#19995,
#19996,#19997,#19998,#19999,#20000,#20001,#20002,#20003,#20004,#20005,#20006,
#20007,#20008,#20009,#20010,#20011,#20012,#20013,#20014,#20015,#20016,#20017,
#20018,#20019,#20020,#20021,#20022,#20023,#20024,#20025,#20026,#20027,#20028,
#20029,#20030,#20031,#20032,#20033,#20034,#20035,#20036,#20037,#20038,#20039,
#20040,#20041,#20042,#20043,#20044,#20045,#20046,#20047,#20048,#20049,#20050,
#20051,#20052,#20053,#20054,#20055,#20056,#20057,#20058,#20059,#20060,#20061,
#20062,#20063,#20064,#20065,#20066,#20067,#20068,#20069,#20070,#20071,#20072,
#20073,#20074,#20075,#20076,#20077,#20078,#20079,#20080,#20081,#20082,#20083,
#20084,#20085,#20086,#20087,#20088,#20089,#20090,#20091,#20092,#20093,#20094,
#20095,#20096,#20097,#20098,#20099,#20100,#20101,#20102,#20103,#20104,#20105,
#20106,#20107,#20108,#20109,#20110,#20111,#20112,#20113,#20114,#20115,#20116,
#20117,#20118,#20119,#20120,#20121,#20122,#20123,#20124,#20125,#20126,#20127,
#20128,#20129,#20130,#20131,#20132,#20133,#20134,#20135,#20136,#20137,#20138,
#20139,#20140,#20141,#20142,#20143,#20144,#20145,#20146,#20147,#20148,#20149,
#20150,#20151,#20152,#20153,#20154,#20155,#20156,#20157,#20158,#20159,#20160,
#20161,#20162,#20163,#20164,#20165,#20166,#20167,#20168,#20169,#20170,#20171,
#20172,#20173,#20174,#20175,#20176,#20177,#20178,#20179,#20180,#20181,#20182,
#20183,#20184,#20185,#20186,#20187,#20188,#20189,#20190,#20191,#20192,#20193,
#20194,#20195,#20196,#20197,#20198,#20199,#20200,#20201,#20202,#20203,#20204,
#20205,#20206,#20207,#20208,#20209,#20210,#20211,#20212,#20213,#20214,#20215,
#20216,#20217,#20218,#20219,#20220,#20221,#20222,#20223,#20224,#20225,#20226,
#20227,#20228,#20229,#20230,#20231,#20232,#20233,#20234,#20235,#20236,#20237,
#20238,#20239,#20240,#20241,#20242,#20243,#20244,#20245,#20246,#20247,#20248,
#20249,#20250,#20251,#20252,#20253,#20254,#20255,#20256,#20257,#20258,#20259,
#20260,#20261,#20262,#20263,#20264,#20265,#20266,#20267,#20268,#20269,#20270,
#20271,#20272,#20273,#20274,#20275,#20276,#20277,#20278,#20279,#20280,#20281,
#20282,#20283,#20284,#20285,#20286,#20287,#20288,#20289,#20290,#20291,#20292,
#20293,#20294,#20295,#20296,#20297,#20298,#20299,#20300,#20301,#20302,#20303,
#20304,#20305,#20306,#20307,#20308,#20309,#20310,#20311,#20312,#20313,#20314,
#20315,#20316,#20317,#20318,#20319,#20320,#20321,#20322,#20323,#20324,#20325,
#20326,#20327,#20328,#20329,#20330,#20331,#20332,#20333,#20334,#20335,#20336,
#20337,#20338,#20339,#20340,#20341,#20342,#20343,#20344,#20345,#20346,#20347,
#20348,#20349,#20350,#20351,#20352,#20353,#20354,#20355,#20356,#20357,#20358,
#20359,#20360,#20361,#20362,#20363,#20364,#20365,#20366,#20367,#20368,#20369,
#20370,#20371,#20372,#20373,#20374,#20375,#20376,#20377,#20378,#20379,#20380,
#20381,#20382,#20383,#20384,#20385,#20386,#20387,#20388,#20389,#20390,#20391,
#20392,#20393,#20394,#20395,#20396,#20397,#20398,#20399,#20400,#20401,#20402,
#20403,#20404,#20405,#20406,#20407,#20408,#20409,#20410,#20411),(#20412,
#20413,#20414,#20415,#20416,#20417,#20418,#20419,#20420,#20421,#20422,#20423,
#20424,#20425,#20426,#20427,#20428,#20429,#20430,#20431,#20432,#20433,#20434,
#20435,#20436,#20437,#20438,#20439,#20440,#20441,#20442,#20443,#20444,#20445,
#20446,#20447,#20448,#20449,#20450,#20451,#20452,#20453,#20454,#20455,#20456,
#20457,#20458,#20459,#20460,#20461,#20462,#20463,#20464,#20465,#20466,#20467,
#20468,#20469,#20470,#20471,#20472,#20473,#20474,#20475,#20476,#20477,#20478,
#20479,#20480,#20481,#20482,#20483,#20484,#20485,#20486,#20487,#20488,#20489,
#20490,#20491,#20492,#20493,#20494,#20495,#20496,#20497,#20498,#20499,#20500,
#20501,#20502,#20503,#20504,#20505,#20506,#20507,#20508,#20509,#20510,#20511,
#20512,#20513,#20514,#20515,#20516,#20517,#20518,#20519,#20520,#20521,#20522,
#20523,#20524,#20525,#20526,#20527,#20528,#20529,#20530,#20531,#20532,#20533,
#20534,#20535,#20536,#20537,#20538,#20539,#20540,#20541,#20542,#20543,#20544,
#20545,#20546,#20547,#20548,#20549,#20550,#20551,#20552,#20553,#20554,#20555,
#20556,#20557,#20558,#20559,#20560,#20561,#20562,#20563,#20564,#20565,#20566,
#20567,#20568,#20569,#20570,#20571,#20572,#20573,#20574,#20575,#20576,#20577,
#20578,#20579,#20580,#20581,#20582,#20583,#20584,#20585,#20586,#20587,#20588,
#20589,#20590,#20591,#20592,#20593,#20594,#20595,#20596,#20597,#20598,#20599,
#20600,#20601,#20602,#20603,#20604,#20605,#20606,#20607,#20608,#20609,#20610,
#20611,#20612,#20613,#20614,#20615,#20616,#20617,#20618,#20619,#20620,#20621,
#20622,#20623,#20624,#20625,#20626,#20627,#20628,#20629,#20630,#20631,#20632,
#20633,#20634,#20635,#20636,#20637,#20638,#20639,#20640,#20641,#20642,#20643,
#20644,#20645,#20646,#20647,#20648,#20649,#20650,#20651,#20652,#20653,#20654,
#20655,#20656,#20657,#20658,#20659,#20660,#20661,#20662,#20663,#20664,#20665,
#20666,#20667,#20668,#20669,#20670,#20671,#20672,#20673,#20674,#20675,#20676,
#20677,#20678,#20679,#20680,#20681,#20682,#20683,#20684,#20685,#20686,#20687,
#20688,#20689,#20690,#20691,#20692,#20693,#20694,#20695,#20696,#20697,#20698,
#20699,#20700,#20701,#20702,#20703,#20704,#20705,#20706,#20707,#20708,#20709,
#20710,#20711,#20712,#20713,#20714,#20715,#20716,#20717,#20718,#20719,#20720,
#20721,#20722,#20723,#20724,#20725,#20726,#20727,#20728,#20729,#20730,#20731,
#20732,#20733,#20734,#20735,#20736,#20737,#20738,#20739,#20740,#20741,#20742,
#20743,#20744,#20745,#20746,#20747,#20748,#20749,#20750,#20751,#20752,#20753,
#20754,#20755,#20756,#20757,#20758,#20759,#20760,#20761,#20762,#20763,#20764,
#20765,#20766,#20767,#20768,#20769,#20770,#20771,#20772,#20773,#20774,#20775,
#20776,#20777,#20778,#20779,#20780,#20781,#20782,#20783,#20784,#20785,#20786,
#20787,#20788,#20789,#20790,#20791,#20792,#20793,#20794,#20795,#20796,#20797,
#20798,#20799,#20800,#20801,#20802,#20803,#20804,#20805,#20806,#20807,#20808,
#20809,#20810,#20811,#20812,#20813,#20814,#20815,#20816,#20817,#20818,#20819,
#20820,#20821,#20822,#20823,#20824,#20825,#20826,#20827,#20828,#20829,#20830,
#20831,#20832,#20833,#20834,#20835,#20836,#20837,#20838,#20839,#20840,#20841,
#20842,#20843,#20844,#20845,#20846,#20847,#20848,#20849,#20850,#20851,#20852,
#20853,#20854,#20855,#20856,#20857,#20858,#20859,#20860,#20861,#20862,#20863,
#20864,#20865,#20866,#20867,#20868,#20869,#20870,#20871,#20872,#20873,#20874,
#20875,#20876,#20877,#20878,#20879,#20880,#20881,#20882,#20883,#20884,#20885,
#20886,#20887,#20888,#20889,#20890,#20891,#20892,#20893,#20894,#20895,#20896,
#20897,#20898,#20899,#20900,#20901,#20902,#20903,#20904,#20905,#20906,#20907,
#20908,#20909,#20910,#20911,#20912,#20913,#20914,#20915,#20916,#20917,#20918,
#20919,#20920,#20921,#20922,#20923,#20924,#20925,#20926,#20927,#20928,#20929,
#20930,#20931,#20932,#20933,#20934,#20935,#20936,#20937,#20938,#20939,#20940,
#20941,#20942,#20943,#20944,#20945,#20946,#20947,#20948,#20949,#20950,#20951,
#20952,#20953,#20954,#20955,#20956,#20957,#20958,#20959,#20960,#20961,#20962,
#20963,#20964,#20965,#20966,#20967,#20968,#20969,#20970,#20971,#20972,#20973,
#20974,#20975,#20976,#20977,#20978,#20979,#20980,#20981,#20982,#20983,#20984,
#20985,#20986,#20987,#20988,#20989,#20990,#20991,#20992,#20993,#20994,#20995,
#20996,#20997,#20998,#20999,#21000,#21001,#21002,#21003,#21004,#21005,#21006,
#21007,#21008,#21009,#21010,#21011,#21012,#21013,#21014,#21015,#21016,#21017,
#21018,#21019,#21020,#21021,#21022,#21023,#21024,#21025,#21026,#21027,#21028,
#21029,#21030,#21031,#21032,#21033,#21034,#21035,#21036,#21037,#21038,#21039,
#21040,#21041,#21042,#21043,#21044,#21045,#21046,#21047,#21048,#21049,#21050,
#21051,#21052,#21053,#21054,#21055,#21056,#21057,#21058,#21059,#21060,#21061,
#21062,#21063,#21064,#21065,#21066,#21067,#21068,#21069,#21070,#21071,#21072,
#21073,#21074,#21075,#21076,#21077,#21078,#21079,#21080,#21081,#21082,#21083,
#21084,#21085,#21086,#21087,#21088,#21089,#21090,#21091,#21092,#21093,#21094,
#21095,#21096,#21097,#21098,#21099,#21100,#21101,#21102,#21103,#21104,#21105,
#21106,#21107,#21108,#21109,#21110,#21111,#21112,#21113,#21114,#21115,#21116,
#21117,#21118,#21119,#21120,#21121,#21122,#21123,#21124,#21125,#21126,#21127,
#21128,#21129,#21130,#21131,#21132,#21133,#21134,#21135,#21136,#21137,#21138,
#21139,#21140,#21141,#21142,#21143,#21144,#21145,#21146,#21147,#21148,#21149,
#21150,#21151,#21152,#21153,#21154,#21155,#21156,#21157,#21158,#21159,#21160,
#21161,#21162,#21163,#21164,#21165,#21166,#21167,#21168,#21169,#21170,#21171,
#21172,#21173,#21174,#21175,#21176,#21177,#21178,#21179,#21180,#21181,#21182,
#21183,#21184,#21185,#21186,#21187,#21188,#21189,#21190,#21191,#21192,#21193,
#21194,#21195,#21196,#21197,#21198,#21199,#21200,#21201,#21202,#21203,#21204,
#21205,#21206,#21207,#21208,#21209,#21210,#21211,#21212,#21213,#21214,#21215,
#21216,#21217,#21218,#21219,#21220,#21221,#21222,#21223,#21224,#21225,#21226,
#21227,#21228,#21229,#21230,#21231,#21232,#21233,#21234,#21235,#21236,#21237,
#21238,#21239,#21240,#21241,#21242,#21243,#21244,#21245,#21246,#21247,#21248,
#21249,#21250,#21251,#21252,#21253,#21254,#21255,#21256,#21257,#21258,#21259,
#21260,#21261,#21262,#21263,#21264,#21265,#21266,#21267,#21268,#21269,#21270,
#21271,#21272,#21273,#21274,#21275,#21276,#21277,#21278,#21279,#21280,#21281,
#21282,#21283,#21284,#21285,#21286,#21287,#21288,#21289,#21290,#21291,#21292,
#21293,#21294,#21295,#21296,#21297,#21298,#21299,#21300,#21301,#21302,#21303,
#21304,#21305,#21306,#21307,#21308,#21309,#21310,#21311,#21312,#21313,#21314,
#21315,#21316,#21317,#21318,#21319,#21320,#21321,#21322,#21323,#21324,#21325,
#21326,#21327,#21328,#21329,#21330,#21331,#21332,#21333,#21334,#21335,#21336,
#21337,#21338,#21339,#21340,#21341,#21342,#21343,#21344,#21345,#21346,#21347,
#21348,#21349,#21350,#21351,#21352,#21353,#21354,#21355,#21356,#21357,#21358,
#21359,#21360,#21361,#21362,#21363,#21364,#21365,#21366,#21367,#21368,#21369,
#21370,#21371,#21372,#21373,#21374,#21375,#21376,#21377,#21378,#21379,#21380,
#21381,#21382,#21383,#21384)),.UNSPECIFIED.,.F.,.F.,.F.)
B_SPLINE_SURFACE_WITH_KNOTS((2,2),(3,2,2,2,2,2,2,2,2,2,2,2,2,2,2,2,2,2,
2,2,2,2,2,2,2,2,2,2,2,2,2,2,2,2,2,2,2,2,2,2,2,2,2,2,2,2,2,2,2,2,2,2,2,2,
2,2,2,2,2,2,2,2,2,2,2,2,2,2,2,2,2,2,2,2,2,2,2,2,2,2,2,2,2,2,2,2,2,2,2,2,
2,2,2,2,2,2,2,2,2,2,2,2,2,2,2,2,2,2,2,2,2,2,2,2,2,2,2,2,2,2,2,2,2,2,2,2,
2,2,2,2,2,2,2,2,2,2,2,2,2,2,2,2,2,2,2,2,2,2,2,2,2,2,2,2,2,2,2,2,2,2,2,2,
2,2,2,2,2,2,2,2,2,2,2,2,2,2,2,2,2,2,2,2,2,2,2,2,2,2,2,2,2,2,2,2,2,2,2,2,
2,2,2,2,2,2,2,2,2,2,2,2,2,2,2,2,2,2,2,2,2,2,2,2,2,2,2,2,2,2,2,2,2,2,2,2,
2,2,2,2,2,2,2,2,2,2,2,2,2,2,2,2,2,2,2,2,2,2,2,2,2,2,2,2,2,2,2,2,2,2,2,2,
2,2,2,2,2,2,2,2,2,2,2,2,2,2,2,2,2,2,2,2,2,2,2,2,2,2,2,2,2,2,2,2,2,2,2,2,
2,2,2,2,2,2,2,2,2,2,2,2,2,2,2,2,2,2,2,2,2,2,2,2,2,2,2,2,2,2,2,2,2,2,2,2,
2,2,2,2,2,2,2,2,2,2,2,2,2,2,2,2,2,2,2,2,2,2,2,2,2,2,2,2,2,2,2,2,2,2,2,2,
2,2,2,2,2,2,2,2,2,2,2,2,2,2,2,2,2,2,2,2,2,2,2,2,2,2,2,2,2,2,2,2,2,2,2,2,
2,2,2,2,2,2,2,2,2,2,2,2,2,2,2,2,2,2,2,2,2,2,2,2,2,2,2,2,2,2,2,2,2,2,2,2,
2,2,2,2,2,2,2,2,2,2,2,2,2,2,2,2,2,2,2,2,2,2,2,2,2,2,2,2,2,2,2,2,2,2,2,2,
3),(-1.70634721592824E-6,1.),(0.,0.00205761316872428,0.00411522633744856,
0.00617283950617284,0.00823045267489712,0.0102880658436214,0.0123456790123457,
0.01440329218107,0.0164609053497942,0.0185185185185185,0.0205761316872428,
0.0226337448559671,0.0246913580246914,0.0267489711934156,0.0288065843621399,
0.0308641975308642,0.0329218106995885,0.0349794238683128,0.037037037037037,
0.0390946502057613,0.0411522633744856,0.0432098765432099,0.0452674897119342,
0.0473251028806584,0.0493827160493827,0.051440329218107,0.0534979423868313,
0.0555555555555556,0.0576131687242798,0.0596707818930041,0.0617283950617284,
0.0637860082304527,0.065843621399177,0.0679012345679012,0.0699588477366255,
0.0720164609053498,0.0740740740740741,0.0761316872427984,0.0781893004115226,
0.0802469135802469,0.0823045267489712,0.0843621399176955,0.0864197530864197,
0.088477366255144,0.0905349794238683,0.0925925925925926,0.0946502057613169,
0.0967078189300412,0.0987654320987654,0.10082304526749,0.102880658436214,
0.104938271604938,0.106995884773663,0.109053497942387,0.111111111111111,
0.113168724279835,0.11522633744856,0.117283950617284,0.119341563786008,
0.121399176954733,0.123456790123457,0.125514403292181,0.127572016460905,
0.12962962962963,0.131687242798354,0.133744855967078,0.135802469135802,
0.137860082304527,0.139917695473251,0.141975308641975,0.1440329218107,0.146090534979424,
0.148148148148148,0.150205761316872,0.152263374485597,0.154320987654321,
0.156378600823045,0.15843621399177,0.160493827160494,0.162551440329218,
0.164609053497942,0.166666666666667,0.168724279835391,0.170781893004115,
0.172839506172839,0.174897119341564,0.176954732510288,0.179012345679012,
0.181069958847737,0.183127572016461,0.185185185185185,0.187242798353909,
0.189300411522634,0.191358024691358,0.193415637860082,0.195473251028807,
0.197530864197531,0.199588477366255,0.201646090534979,0.203703703703704,
0.205761316872428,0.207818930041152,0.209876543209877,0.211934156378601,
0.213991769547325,0.216049382716049,0.218106995884774,0.220164609053498,
0.222222222222222,0.224279835390947,0.226337448559671,0.228395061728395,
0.230452674897119,0.232510288065844,0.234567901234568,0.236625514403292,
0.238683127572016,0.240740740740741,0.242798353909465,0.244855967078189,
0.246913580246914,0.248971193415638,0.251028806584362,0.253086419753086,
0.255144032921811,0.257201646090535,0.259259259259259,0.261316872427984,
0.263374485596708,0.265432098765432,0.267489711934156,0.269547325102881,
0.271604938271605,0.273662551440329,0.275720164609054,0.277777777777778,
0.279835390946502,0.281893004115226,0.283950617283951,0.286008230452675,
0.288065843621399,0.290123456790123,0.292181069958848,0.294238683127572,
0.296296296296296,0.298353909465021,0.300411522633745,0.302469135802469,
0.304526748971193,0.306584362139918,0.308641975308642,0.310699588477366,
0.312757201646091,0.314814814814815,0.316872427983539,0.318930041152263,
0.320987654320988,0.323045267489712,0.325102880658436,0.327160493827161,
0.329218106995885,0.331275720164609,0.333333333333333,0.335390946502058,
0.337448559670782,0.339506172839506,0.34156378600823,0.343621399176955,
0.345679012345679,0.347736625514403,0.349794238683128,0.351851851851852,
0.353909465020576,0.3559670781893,0.358024691358025,0.360082304526749,0.362139917695473,
0.364197530864198,0.366255144032922,0.368312757201646,0.37037037037037,
0.372427983539095,0.374485596707819,0.376543209876543,0.378600823045267,
0.380658436213992,0.382716049382716,0.38477366255144,0.386831275720165,
0.388888888888889,0.390946502057613,0.393004115226337,0.395061728395062,
0.397119341563786,0.39917695473251,0.401234567901235,0.403292181069959,
0.405349794238683,0.407407407407407,0.409465020576132,0.411522633744856,
0.41358024691358,0.415637860082305,0.417695473251029,0.419753086419753,
0.421810699588477,0.423868312757202,0.425925925925926,0.42798353909465,
0.430041152263374,0.432098765432099,0.434156378600823,0.436213991769547,
0.438271604938272,0.440329218106996,0.44238683127572,0.444444444444444,
0.446502057613169,0.448559670781893,0.450617283950617,0.452674897119342,
0.454732510288066,0.45679012345679,0.458847736625514,0.460905349794239,
0.462962962962963,0.465020576131687,0.467078189300412,0.469135802469136,
0.47119341563786,0.473251028806584,0.475308641975309,0.477366255144033,
0.479423868312757,0.481481481481481,0.483539094650206,0.48559670781893,
0.487654320987654,0.489711934156379,0.491769547325103,0.493827160493827,
0.495884773662551,0.497942386831276,0.5,0.502057613168724,0.504115226337449,
0.506172839506173,0.508230452674897,0.510288065843621,0.512345679012346,
0.51440329218107,0.516460905349794,0.518518518518518,0.520576131687243,
0.522633744855967,0.524691358024691,0.526748971193416,0.52880658436214,
0.530864197530864,0.532921810699588,0.534979423868313,0.537037037037037,
0.539094650205761,0.541152263374486,0.54320987654321,0.545267489711934,
0.547325102880658,0.549382716049383,0.551440329218107,0.553497942386831,
0.555555555555556,0.55761316872428,0.559670781893004,0.561728395061728,
0.563786008230453,0.565843621399177,0.567901234567901,0.569958847736626,
0.57201646090535,0.574074074074074,0.576131687242798,0.578189300411523,
0.580246913580247,0.582304526748971,0.584362139917695,0.58641975308642,
0.588477366255144,0.590534979423868,0.592592592592593,0.594650205761317,
0.596707818930041,0.598765432098765,0.60082304526749,0.602880658436214,
0.604938271604938,0.606995884773663,0.609053497942387,0.611111111111111,
0.613168724279835,0.61522633744856,0.617283950617284,0.619341563786008,
0.621399176954732,0.623456790123457,0.625514403292181,0.627572016460905,
0.62962962962963,0.631687242798354,0.633744855967078,0.635802469135803,
0.637860082304527,0.639917695473251,0.641975308641975,0.6440329218107,0.646090534979424,
0.648148148148148,0.650205761316872,0.652263374485597,0.654320987654321,
0.656378600823045,0.65843621399177,0.660493827160494,0.662551440329218,
0.664609053497942,0.666666666666667,0.668724279835391,0.670781893004115,
0.672839506172839,0.674897119341564,0.676954732510288,0.679012345679012,
0.681069958847737,0.683127572016461,0.685185185185185,0.687242798353909,
0.689300411522634,0.691358024691358,0.693415637860082,0.695473251028807,
0.697530864197531,0.699588477366255,0.701646090534979,0.703703703703704,
0.705761316872428,0.707818930041152,0.709876543209877,0.711934156378601,
0.713991769547325,0.716049382716049,0.718106995884774,0.720164609053498,
0.722222222222222,0.724279835390947,0.726337448559671,0.728395061728395,
0.730452674897119,0.732510288065844,0.734567901234568,0.736625514403292,
0.738683127572016,0.740740740740741,0.742798353909465,0.744855967078189,
0.746913580246914,0.748971193415638,0.751028806584362,0.753086419753086,
0.755144032921811,0.757201646090535,0.759259259259259,0.761316872427984,
0.763374485596708,0.765432098765432,0.767489711934156,0.769547325102881,
0.771604938271605,0.773662551440329,0.775720164609053,0.777777777777778,
0.779835390946502,0.781893004115226,0.783950617283951,0.786008230452675,
0.788065843621399,0.790123456790123,0.792181069958848,0.794238683127572,
0.796296296296296,0.798353909465021,0.800411522633745,0.802469135802469,
0.804526748971193,0.806584362139918,0.808641975308642,0.810699588477366,
0.812757201646091,0.814814814814815,0.816872427983539,0.818930041152263,
0.820987654320988,0.823045267489712,0.825102880658436,0.827160493827161,
0.829218106995885,0.831275720164609,0.833333333333333,0.835390946502058,
0.837448559670782,0.839506172839506,0.84156378600823,0.843621399176955,
0.845679012345679,0.847736625514403,0.849794238683128,0.851851851851852,
0.853909465020576,0.8559670781893,0.858024691358025,0.860082304526749,0.862139917695473,
0.864197530864197,0.866255144032922,0.868312757201646,0.87037037037037,
0.872427983539095,0.874485596707819,0.876543209876543,0.878600823045268,
0.880658436213992,0.882716049382716,0.88477366255144,0.886831275720165,
0.888888888888889,0.890946502057613,0.893004115226337,0.895061728395062,
0.897119341563786,0.89917695473251,0.901234567901235,0.903292181069959,
0.905349794238683,0.907407407407407,0.909465020576132,0.911522633744856,
0.91358024691358,0.915637860082305,0.917695473251029,0.919753086419753,
0.921810699588477,0.923868312757202,0.925925925925926,0.92798353909465,
0.930041152263374,0.932098765432099,0.934156378600823,0.936213991769547,
0.938271604938272,0.940329218106996,0.94238683127572,0.944444444444444,
0.946502057613169,0.948559670781893,0.950617283950617,0.952674897119342,
0.954732510288066,0.95679012345679,0.958847736625514,0.960905349794239,
0.962962962962963,0.965020576131687,0.967078189300412,0.969135802469136,
0.97119341563786,0.973251028806584,0.975308641975309,0.977366255144033,
0.979423868312757,0.981481481481482,0.983539094650206,0.98559670781893,
0.987654320987654,0.989711934156379,0.991769547325103,0.993827160493827,
0.995884773662551,0.997942386831276,1.),.UNSPECIFIED.)
GEOMETRIC_REPRESENTATION_ITEM()
RATIONAL_B_SPLINE_SURFACE(((1.,0.866025403784439,1.,0.866025403784439,1.,
0.866025403784439,1.,0.866025403784439,1.,0.866025403784439,1.,0.866025403784439,
1.,0.866025403784439,1.,0.866025403784439,1.,0.866025403784439,1.,0.866025403784439,
1.,0.866025403784439,1.,0.866025403784439,1.,0.866025403784439,1.,0.866025403784439,
1.,0.866025403784439,1.,0.866025403784439,1.,0.866025403784439,1.,0.866025403784439,
1.,0.866025403784439,1.,0.866025403784439,1.,0.866025403784439,1.,0.866025403784439,
1.,0.866025403784439,1.,0.866025403784439,1.,0.866025403784439,1.,0.866025403784439,
1.,0.866025403784439,1.,0.866025403784439,1.,0.866025403784439,1.,0.866025403784439,
1.,0.866025403784439,1.,0.866025403784439,1.,0.866025403784439,1.,0.866025403784439,
1.,0.866025403784439,1.,0.866025403784439,1.,0.866025403784439,1.,0.866025403784439,
1.,0.866025403784439,1.,0.866025403784439,1.,0.866025403784439,1.,0.866025403784439,
1.,0.866025403784439,1.,0.866025403784439,1.,0.866025403784439,1.,0.866025403784439,
1.,0.866025403784439,1.,0.866025403784439,1.,0.866025403784439,1.,0.866025403784439,
1.,0.866025403784439,1.,0.866025403784439,1.,0.866025403784439,1.,0.866025403784439,
1.,0.866025403784439,1.,0.866025403784439,1.,0.866025403784439,1.,0.866025403784439,
1.,0.866025403784439,1.,0.866025403784439,1.,0.866025403784439,1.,0.866025403784439,
1.,0.866025403784439,1.,0.866025403784439,1.,0.866025403784439,1.,0.866025403784439,
1.,0.866025403784439,1.,0.866025403784439,1.,0.866025403784439,1.,0.866025403784439,
1.,0.866025403784439,1.,0.866025403784439,1.,0.866025403784439,1.,0.866025403784439,
1.,0.866025403784439,1.,0.866025403784439,1.,0.866025403784439,1.,0.866025403784439,
1.,0.866025403784439,1.,0.866025403784439,1.,0.866025403784439,1.,0.866025403784439,
1.,0.866025403784439,1.,0.866025403784439,1.,0.866025403784439,1.,0.866025403784439,
1.,0.866025403784439,1.,0.866025403784439,1.,0.866025403784439,1.,0.866025403784439,
1.,0.866025403784439,1.,0.866025403784439,1.,0.866025403784439,1.,0.866025403784439,
1.,0.866025403784439,1.,0.866025403784439,1.,0.866025403784439,1.,0.866025403784439,
1.,0.866025403784439,1.,0.866025403784439,1.,0.866025403784439,1.,0.866025403784439,
1.,0.866025403784439,1.,0.866025403784439,1.,0.866025403784439,1.,0.866025403784439,
1.,0.866025403784439,1.,0.866025403784439,1.,0.866025403784439,1.,0.866025403784439,
1.,0.866025403784439,1.,0.866025403784439,1.,0.866025403784439,1.,0.866025403784439,
1.,0.866025403784439,1.,0.866025403784439,1.,0.866025403784439,1.,0.866025403784439,
1.,0.866025403784439,1.,0.866025403784439,1.,0.866025403784439,1.,0.866025403784439,
1.,0.866025403784439,1.,0.866025403784439,1.,0.866025403784439,1.,0.866025403784439,
1.,0.866025403784439,1.,0.866025403784439,1.,0.866025403784439,1.,0.866025403784439,
1.,0.866025403784439,1.,0.866025403784439,1.,0.866025403784439,1.,0.866025403784439,
1.,0.866025403784439,1.,0.866025403784439,1.,0.866025403784439,1.,0.866025403784439,
1.,0.866025403784439,1.,0.866025403784439,1.,0.866025403784439,1.,0.866025403784439,
1.,0.866025403784439,1.,0.866025403784439,1.,0.866025403784439,1.,0.866025403784439,
1.,0.866025403784439,1.,0.866025403784439,1.,0.866025403784439,1.,0.866025403784439,
1.,0.866025403784439,1.,0.866025403784439,1.,0.866025403784439,1.,0.866025403784439,
1.,0.866025403784439,1.,0.866025403784439,1.,0.866025403784439,1.,0.866025403784439,
1.,0.866025403784439,1.,0.866025403784439,1.,0.866025403784439,1.,0.866025403784439,
1.,0.866025403784439,1.,0.866025403784439,1.,0.866025403784439,1.,0.866025403784439,
1.,0.866025403784439,1.,0.866025403784439,1.,0.866025403784439,1.,0.866025403784439,
1.,0.866025403784439,1.,0.866025403784439,1.,0.866025403784439,1.,0.866025403784439,
1.,0.866025403784439,1.,0.866025403784439,1.,0.866025403784439,1.,0.866025403784439,
1.,0.866025403784439,1.,0.866025403784439,1.,0.866025403784439,1.,0.866025403784439,
1.,0.866025403784439,1.,0.866025403784439,1.,0.866025403784439,1.,0.866025403784439,
1.,0.866025403784439,1.,0.866025403784439,1.,0.866025403784439,1.,0.866025403784439,
1.,0.866025403784439,1.,0.866025403784439,1.,0.866025403784439,1.,0.866025403784439,
1.,0.866025403784439,1.,0.866025403784439,1.,0.866025403784439,1.,0.866025403784439,
1.,0.866025403784439,1.,0.866025403784439,1.,0.866025403784439,1.,0.866025403784439,
1.,0.866025403784439,1.,0.866025403784439,1.,0.866025403784439,1.,0.866025403784439,
1.,0.866025403784439,1.,0.866025403784439,1.,0.866025403784439,1.,0.866025403784439,
1.,0.866025403784439,1.,0.866025403784439,1.,0.866025403784439,1.,0.866025403784439,
1.,0.866025403784439,1.,0.866025403784439,1.,0.866025403784439,1.,0.866025403784439,
1.,0.866025403784439,1.,0.866025403784439,1.,0.866025403784439,1.,0.866025403784439,
1.,0.866025403784439,1.,0.866025403784439,1.,0.866025403784439,1.,0.866025403784439,
1.,0.866025403784439,1.,0.866025403784439,1.,0.866025403784439,1.,0.866025403784439,
1.,0.866025403784439,1.,0.866025403784439,1.,0.866025403784439,1.,0.866025403784439,
1.,0.866025403784439,1.,0.866025403784439,1.,0.866025403784439,1.,0.866025403784439,
1.,0.866025403784439,1.,0.866025403784439,1.,0.866025403784439,1.,0.866025403784439,
1.,0.866025403784439,1.,0.866025403784439,1.,0.866025403784439,1.,0.866025403784439,
1.,0.866025403784439,1.,0.866025403784439,1.,0.866025403784439,1.,0.866025403784439,
1.,0.866025403784439,1.,0.866025403784439,1.,0.866025403784439,1.,0.866025403784439,
1.,0.866025403784439,1.,0.866025403784439,1.,0.866025403784439,1.,0.866025403784439,
1.,0.866025403784439,1.,0.866025403784439,1.,0.866025403784439,1.,0.866025403784439,
1.,0.866025403784439,1.,0.866025403784439,1.,0.866025403784439,1.,0.866025403784439,
1.,0.866025403784439,1.,0.866025403784439,1.,0.866025403784439,1.,0.866025403784439,
1.,0.866025403784439,1.,0.866025403784439,1.,0.866025403784439,1.,0.866025403784439,
1.,0.866025403784439,1.,0.866025403784439,1.,0.866025403784439,1.,0.866025403784439,
1.,0.866025403784439,1.,0.866025403784439,1.,0.866025403784439,1.,0.866025403784439,
1.,0.866025403784439,1.,0.866025403784439,1.,0.866025403784439,1.,0.866025403784439,
1.,0.866025403784439,1.,0.866025403784439,1.,0.866025403784439,1.,0.866025403784439,
1.,0.866025403784439,1.,0.866025403784439,1.,0.866025403784439,1.,0.866025403784439,
1.,0.866025403784439,1.,0.866025403784439,1.,0.866025403784439,1.,0.866025403784439,
1.,0.866025403784439,1.,0.866025403784439,1.,0.866025403784439,1.,0.866025403784439,
1.,0.866025403784439,1.,0.866025403784439,1.,0.866025403784439,1.,0.866025403784439,
1.,0.866025403784439,1.,0.866025403784439,1.,0.866025403784439,1.,0.866025403784439,
1.,0.866025403784439,1.,0.866025403784439,1.,0.866025403784439,1.,0.866025403784439,
1.,0.866025403784439,1.,0.866025403784439,1.,0.866025403784439,1.,0.866025403784439,
1.,0.866025403784439,1.,0.866025403784439,1.,0.866025403784439,1.,0.866025403784439,
1.,0.866025403784439,1.,0.866025403784439,1.,0.866025403784439,1.,0.866025403784439,
1.,0.866025403784439,1.,0.866025403784439,1.,0.866025403784439,1.,0.866025403784439,
1.,0.866025403784439,1.,0.866025403784439,1.,0.866025403784439,1.,0.866025403784439,
1.,0.866025403784439,1.,0.866025403784439,1.,0.866025403784439,1.,0.866025403784439,
1.,0.866025403784439,1.,0.866025403784439,1.,0.866025403784439,1.,0.866025403784439,
1.,0.866025403784439,1.,0.866025403784439,1.,0.866025403784439,1.,0.866025403784439,
1.,0.866025403784439,1.,0.866025403784439,1.,0.866025403784439,1.,0.866025403784439,
1.,0.866025403784439,1.,0.866025403784439,1.,0.866025403784439,1.,0.866025403784439,
1.,0.866025403784439,1.,0.866025403784439,1.,0.866025403784439,1.,0.866025403784439,
1.,0.866025403784439,1.,0.866025403784439,1.,0.866025403784439,1.,0.866025403784439,
1.,0.866025403784439,1.,0.866025403784439,1.,0.866025403784439,1.,0.866025403784439,
1.,0.866025403784439,1.,0.866025403784439,1.,0.866025403784439,1.,0.866025403784439,
1.,0.866025403784439,1.,0.866025403784439,1.,0.866025403784439,1.,0.866025403784439,
1.,0.866025403784439,1.,0.866025403784439,1.,0.866025403784439,1.,0.866025403784439,
1.,0.866025403784439,1.,0.866025403784439,1.,0.866025403784439,1.,0.866025403784439,
1.,0.866025403784439,1.,0.866025403784439,1.,0.866025403784439,1.,0.866025403784439,
1.,0.866025403784439,1.,0.866025403784439,1.,0.866025403784439,1.,0.866025403784439,
1.,0.866025403784439,1.,0.866025403784439,1.,0.866025403784439,1.,0.866025403784439,
1.,0.866025403784439,1.,0.866025403784439,1.,0.866025403784439,1.,0.866025403784439,
1.,0.866025403784439,1.,0.866025403784439,1.,0.866025403784439,1.,0.866025403784439,
1.,0.866025403784439,1.,0.866025403784439,1.,0.866025403784439,1.,0.866025403784439,
1.,0.866025403784439,1.,0.866025403784439,1.,0.866025403784439,1.,0.866025403784439,
1.,0.866025403784439,1.,0.866025403784439,1.,0.866025403784439,1.,0.866025403784439,
1.,0.866025403784439,1.,0.866025403784439,1.,0.866025403784439,1.,0.866025403784439,
1.,0.866025403784439,1.,0.866025403784439,1.,0.866025403784439,1.,0.866025403784439,
1.,0.866025403784439,1.,0.866025403784439,1.,0.866025403784439,1.,0.866025403784439,
1.,0.866025403784439,1.,0.866025403784439,1.,0.866025403784439,1.,0.866025403784439,
1.,0.866025403784439,1.,0.866025403784439,1.,0.866025403784439,1.,0.866025403784439,
1.,0.866025403784439,1.,0.866025403784439,1.,0.866025403784439,1.,0.866025403784439,
1.,0.866025403784439,1.,0.866025403784439,1.,0.866025403784439,1.,0.866025403784439,
1.,0.866025403784439,1.,0.866025403784439,1.,0.866025403784439,1.,0.866025403784439,
1.,0.866025403784439,1.,0.866025403784439,1.,0.866025403784439,1.,0.866025403784439,
1.,0.866025403784439,1.,0.866025403784439,1.,0.866025403784439,1.,0.866025403784439,
1.,0.866025403784439,1.,0.866025403784439,1.,0.866025403784439,1.,0.866025403784439,
1.,0.866025403784439,1.,0.866025403784439,1.,0.866025403784439,1.,0.866025403784439,
1.,0.866025403784439,1.,0.866025403784439,1.,0.866025403784439,1.,0.866025403784439,
1.,0.866025403784439,1.,0.866025403784439,1.,0.866025403784439,1.,0.866025403784439,
1.,0.866025403784439,1.,0.866025403784439,1.,0.866025403784439,1.,0.866025403784439,
1.,0.866025403784439,1.,0.866025403784439,1.,0.866025403784439,1.,0.866025403784439,
1.,0.866025403784439,1.,0.866025403784439,1.,0.866025403784439,1.,0.866025403784439,
1.,0.866025403784439,1.,0.866025403784439,1.,0.866025403784439,1.,0.866025403784439,
1.),(1.,0.866025403784439,1.,0.866025403784439,1.,0.866025403784439,1.,
0.866025403784439,1.,0.866025403784439,1.,0.866025403784439,1.,0.866025403784439,
1.,0.866025403784439,1.,0.866025403784439,1.,0.866025403784439,1.,0.866025403784439,
1.,0.866025403784439,1.,0.866025403784439,1.,0.866025403784439,1.,0.866025403784439,
1.,0.866025403784439,1.,0.866025403784439,1.,0.866025403784439,1.,0.866025403784439,
1.,0.866025403784439,1.,0.866025403784439,1.,0.866025403784439,1.,0.866025403784439,
1.,0.866025403784439,1.,0.866025403784439,1.,0.866025403784439,1.,0.866025403784439,
1.,0.866025403784439,1.,0.866025403784439,1.,0.866025403784439,1.,0.866025403784439,
1.,0.866025403784439,1.,0.866025403784439,1.,0.866025403784439,1.,0.866025403784439,
1.,0.866025403784439,1.,0.866025403784439,1.,0.866025403784439,1.,0.866025403784439,
1.,0.866025403784439,1.,0.866025403784439,1.,0.866025403784439,1.,0.866025403784439,
1.,0.866025403784439,1.,0.866025403784439,1.,0.866025403784439,1.,0.866025403784439,
1.,0.866025403784439,1.,0.866025403784439,1.,0.866025403784439,1.,0.866025403784439,
1.,0.866025403784439,1.,0.866025403784439,1.,0.866025403784439,1.,0.866025403784439,
1.,0.866025403784439,1.,0.866025403784439,1.,0.866025403784439,1.,0.866025403784439,
1.,0.866025403784439,1.,0.866025403784439,1.,0.866025403784439,1.,0.866025403784439,
1.,0.866025403784439,1.,0.866025403784439,1.,0.866025403784439,1.,0.866025403784439,
1.,0.866025403784439,1.,0.866025403784439,1.,0.866025403784439,1.,0.866025403784439,
1.,0.866025403784439,1.,0.866025403784439,1.,0.866025403784439,1.,0.866025403784439,
1.,0.866025403784439,1.,0.866025403784439,1.,0.866025403784439,1.,0.866025403784439,
1.,0.866025403784439,1.,0.866025403784439,1.,0.866025403784439,1.,0.866025403784439,
1.,0.866025403784439,1.,0.866025403784439,1.,0.866025403784439,1.,0.866025403784439,
1.,0.866025403784439,1.,0.866025403784439,1.,0.866025403784439,1.,0.866025403784439,
1.,0.866025403784439,1.,0.866025403784439,1.,0.866025403784439,1.,0.866025403784439,
1.,0.866025403784439,1.,0.866025403784439,1.,0.866025403784439,1.,0.866025403784439,
1.,0.866025403784439,1.,0.866025403784439,1.,0.866025403784439,1.,0.866025403784439,
1.,0.866025403784439,1.,0.866025403784439,1.,0.866025403784439,1.,0.866025403784439,
1.,0.866025403784439,1.,0.866025403784439,1.,0.866025403784439,1.,0.866025403784439,
1.,0.866025403784439,1.,0.866025403784439,1.,0.866025403784439,1.,0.866025403784439,
1.,0.866025403784439,1.,0.866025403784439,1.,0.866025403784439,1.,0.866025403784439,
1.,0.866025403784439,1.,0.866025403784439,1.,0.866025403784439,1.,0.866025403784439,
1.,0.866025403784439,1.,0.866025403784439,1.,0.866025403784439,1.,0.866025403784439,
1.,0.866025403784439,1.,0.866025403784439,1.,0.866025403784439,1.,0.866025403784439,
1.,0.866025403784439,1.,0.866025403784439,1.,0.866025403784439,1.,0.866025403784439,
1.,0.866025403784439,1.,0.866025403784439,1.,0.866025403784439,1.,0.866025403784439,
1.,0.866025403784439,1.,0.866025403784439,1.,0.866025403784439,1.,0.866025403784439,
1.,0.866025403784439,1.,0.866025403784439,1.,0.866025403784439,1.,0.866025403784439,
1.,0.866025403784439,1.,0.866025403784439,1.,0.866025403784439,1.,0.866025403784439,
1.,0.866025403784439,1.,0.866025403784439,1.,0.866025403784439,1.,0.866025403784439,
1.,0.866025403784439,1.,0.866025403784439,1.,0.866025403784439,1.,0.866025403784439,
1.,0.866025403784439,1.,0.866025403784439,1.,0.866025403784439,1.,0.866025403784439,
1.,0.866025403784439,1.,0.866025403784439,1.,0.866025403784439,1.,0.866025403784439,
1.,0.866025403784439,1.,0.866025403784439,1.,0.866025403784439,1.,0.866025403784439,
1.,0.866025403784439,1.,0.866025403784439,1.,0.866025403784439,1.,0.866025403784439,
1.,0.866025403784439,1.,0.866025403784439,1.,0.866025403784439,1.,0.866025403784439,
1.,0.866025403784439,1.,0.866025403784439,1.,0.866025403784439,1.,0.866025403784439,
1.,0.866025403784439,1.,0.866025403784439,1.,0.866025403784439,1.,0.866025403784439,
1.,0.866025403784439,1.,0.866025403784439,1.,0.866025403784439,1.,0.866025403784439,
1.,0.866025403784439,1.,0.866025403784439,1.,0.866025403784439,1.,0.866025403784439,
1.,0.866025403784439,1.,0.866025403784439,1.,0.866025403784439,1.,0.866025403784439,
1.,0.866025403784439,1.,0.866025403784439,1.,0.866025403784439,1.,0.866025403784439,
1.,0.866025403784439,1.,0.866025403784439,1.,0.866025403784439,1.,0.866025403784439,
1.,0.866025403784439,1.,0.866025403784439,1.,0.866025403784439,1.,0.866025403784439,
1.,0.866025403784439,1.,0.866025403784439,1.,0.866025403784439,1.,0.866025403784439,
1.,0.866025403784439,1.,0.866025403784439,1.,0.866025403784439,1.,0.866025403784439,
1.,0.866025403784439,1.,0.866025403784439,1.,0.866025403784439,1.,0.866025403784439,
1.,0.866025403784439,1.,0.866025403784439,1.,0.866025403784439,1.,0.866025403784439,
1.,0.866025403784439,1.,0.866025403784439,1.,0.866025403784439,1.,0.866025403784439,
1.,0.866025403784439,1.,0.866025403784439,1.,0.866025403784439,1.,0.866025403784439,
1.,0.866025403784439,1.,0.866025403784439,1.,0.866025403784439,1.,0.866025403784439,
1.,0.866025403784439,1.,0.866025403784439,1.,0.866025403784439,1.,0.866025403784439,
1.,0.866025403784439,1.,0.866025403784439,1.,0.866025403784439,1.,0.866025403784439,
1.,0.866025403784439,1.,0.866025403784439,1.,0.866025403784439,1.,0.866025403784439,
1.,0.866025403784439,1.,0.866025403784439,1.,0.866025403784439,1.,0.866025403784439,
1.,0.866025403784439,1.,0.866025403784439,1.,0.866025403784439,1.,0.866025403784439,
1.,0.866025403784439,1.,0.866025403784439,1.,0.866025403784439,1.,0.866025403784439,
1.,0.866025403784439,1.,0.866025403784439,1.,0.866025403784439,1.,0.866025403784439,
1.,0.866025403784439,1.,0.866025403784439,1.,0.866025403784439,1.,0.866025403784439,
1.,0.866025403784439,1.,0.866025403784439,1.,0.866025403784439,1.,0.866025403784439,
1.,0.866025403784439,1.,0.866025403784439,1.,0.866025403784439,1.,0.866025403784439,
1.,0.866025403784439,1.,0.866025403784439,1.,0.866025403784439,1.,0.866025403784439,
1.,0.866025403784439,1.,0.866025403784439,1.,0.866025403784439,1.,0.866025403784439,
1.,0.866025403784439,1.,0.866025403784439,1.,0.866025403784439,1.,0.866025403784439,
1.,0.866025403784439,1.,0.866025403784439,1.,0.866025403784439,1.,0.866025403784439,
1.,0.866025403784439,1.,0.866025403784439,1.,0.866025403784439,1.,0.866025403784439,
1.,0.866025403784439,1.,0.866025403784439,1.,0.866025403784439,1.,0.866025403784439,
1.,0.866025403784439,1.,0.866025403784439,1.,0.866025403784439,1.,0.866025403784439,
1.,0.866025403784439,1.,0.866025403784439,1.,0.866025403784439,1.,0.866025403784439,
1.,0.866025403784439,1.,0.866025403784439,1.,0.866025403784439,1.,0.866025403784439,
1.,0.866025403784439,1.,0.866025403784439,1.,0.866025403784439,1.,0.866025403784439,
1.,0.866025403784439,1.,0.866025403784439,1.,0.866025403784439,1.,0.866025403784439,
1.,0.866025403784439,1.,0.866025403784439,1.,0.866025403784439,1.,0.866025403784439,
1.,0.866025403784439,1.,0.866025403784439,1.,0.866025403784439,1.,0.866025403784439,
1.,0.866025403784439,1.,0.866025403784439,1.,0.866025403784439,1.,0.866025403784439,
1.,0.866025403784439,1.,0.866025403784439,1.,0.866025403784439,1.,0.866025403784439,
1.,0.866025403784439,1.,0.866025403784439,1.,0.866025403784439,1.,0.866025403784439,
1.,0.866025403784439,1.,0.866025403784439,1.,0.866025403784439,1.,0.866025403784439,
1.,0.866025403784439,1.,0.866025403784439,1.,0.866025403784439,1.,0.866025403784439,
1.,0.866025403784439,1.,0.866025403784439,1.,0.866025403784439,1.,0.866025403784439,
1.,0.866025403784439,1.,0.866025403784439,1.,0.866025403784439,1.,0.866025403784439,
1.,0.866025403784439,1.,0.866025403784439,1.,0.866025403784439,1.,0.866025403784439,
1.,0.866025403784439,1.,0.866025403784439,1.,0.866025403784439,1.,0.866025403784439,
1.,0.866025403784439,1.,0.866025403784439,1.,0.866025403784439,1.,0.866025403784439,
1.,0.866025403784439,1.,0.866025403784439,1.,0.866025403784439,1.,0.866025403784439,
1.,0.866025403784439,1.,0.866025403784439,1.,0.866025403784439,1.,0.866025403784439,
1.,0.866025403784439,1.,0.866025403784439,1.,0.866025403784439,1.,0.866025403784439,
1.,0.866025403784439,1.,0.866025403784439,1.,0.866025403784439,1.,0.866025403784439,
1.,0.866025403784439,1.,0.866025403784439,1.,0.866025403784439,1.,0.866025403784439,
1.,0.866025403784439,1.,0.866025403784439,1.,0.866025403784439,1.,0.866025403784439,
1.,0.866025403784439,1.,0.866025403784439,1.,0.866025403784439,1.,0.866025403784439,
1.,0.866025403784439,1.,0.866025403784439,1.,0.866025403784439,1.,0.866025403784439,
1.,0.866025403784439,1.,0.866025403784439,1.,0.866025403784439,1.,0.866025403784439,
1.,0.866025403784439,1.,0.866025403784439,1.,0.866025403784439,1.,0.866025403784439,
1.,0.866025403784439,1.,0.866025403784439,1.,0.866025403784439,1.,0.866025403784439,
1.,0.866025403784439,1.,0.866025403784439,1.,0.866025403784439,1.,0.866025403784439,
1.,0.866025403784439,1.,0.866025403784439,1.,0.866025403784439,1.,0.866025403784439,
1.,0.866025403784439,1.,0.866025403784439,1.,0.866025403784439,1.,0.866025403784439,
1.,0.866025403784439,1.,0.866025403784439,1.,0.866025403784439,1.,0.866025403784439,
1.,0.866025403784439,1.,0.866025403784439,1.,0.866025403784439,1.,0.866025403784439,
1.,0.866025403784439,1.,0.866025403784439,1.,0.866025403784439,1.,0.866025403784439,
1.,0.866025403784439,1.,0.866025403784439,1.,0.866025403784439,1.,0.866025403784439,
1.,0.866025403784439,1.,0.866025403784439,1.,0.866025403784439,1.,0.866025403784439,
1.,0.866025403784439,1.,0.866025403784439,1.,0.866025403784439,1.,0.866025403784439,
1.,0.866025403784439,1.,0.866025403784439,1.,0.866025403784439,1.,0.866025403784439,
1.,0.866025403784439,1.,0.866025403784439,1.,0.866025403784439,1.,0.866025403784439,
1.,0.866025403784439,1.,0.866025403784439,1.,0.866025403784439,1.,0.866025403784439,
1.,0.866025403784439,1.,0.866025403784439,1.,0.866025403784439,1.,0.866025403784439,
1.,0.866025403784439,1.,0.866025403784439,1.,0.866025403784439,1.,0.866025403784439,
1.,0.866025403784439,1.,0.866025403784439,1.,0.866025403784439,1.,0.866025403784439,
1.,0.866025403784439,1.,0.866025403784439,1.,0.866025403784439,1.,0.866025403784439,
1.,0.866025403784439,1.,0.866025403784439,1.,0.866025403784439,1.,0.866025403784439,
1.,0.866025403784439,1.,0.866025403784439,1.,0.866025403784439,1.)))
REPRESENTATION_ITEM('')
SURFACE()
);
#151=(
BOUNDED_SURFACE()
B_SPLINE_SURFACE(3,2,((#21658,#21659,#21660,#21661,#21662,#21663,#21664,
#21665,#21666,#21667,#21668,#21669,#21670,#21671,#21672,#21673,#21674,#21675,
#21676,#21677,#21678,#21679,#21680,#21681,#21682,#21683,#21684,#21685,#21686,
#21687,#21688,#21689,#21690,#21691,#21692,#21693,#21694,#21695,#21696,#21697,
#21698,#21699,#21700,#21701,#21702,#21703,#21704,#21705,#21706,#21707,#21708,
#21709,#21710,#21711,#21712,#21713,#21714,#21715,#21716,#21717,#21718,#21719,
#21720,#21721,#21722,#21723,#21724,#21725,#21726,#21727,#21728,#21729,#21730,
#21731,#21732,#21733,#21734,#21735,#21736,#21737,#21738,#21739,#21740,#21741,
#21742,#21743,#21744,#21745,#21746,#21747,#21748,#21749,#21750,#21751,#21752,
#21753,#21754,#21755,#21756,#21757,#21758,#21759,#21760,#21761,#21762,#21763,
#21764,#21765,#21766,#21767,#21768,#21769,#21770,#21771,#21772,#21773,#21774,
#21775,#21776,#21777,#21778,#21779,#21780,#21781,#21782,#21783,#21784,#21785,
#21786,#21787,#21788,#21789,#21790,#21791,#21792,#21793,#21794,#21795,#21796,
#21797,#21798,#21799,#21800,#21801,#21802,#21803,#21804,#21805,#21806,#21807,
#21808,#21809,#21810,#21811,#21812,#21813,#21814,#21815,#21816,#21817,#21818,
#21819,#21820,#21821,#21822,#21823,#21824,#21825,#21826,#21827,#21828,#21829,
#21830,#21831,#21832,#21833,#21834,#21835,#21836,#21837,#21838,#21839,#21840,
#21841,#21842,#21843,#21844,#21845,#21846,#21847,#21848,#21849,#21850,#21851,
#21852,#21853,#21854,#21855,#21856,#21857,#21858,#21859,#21860,#21861,#21862,
#21863,#21864,#21865,#21866,#21867,#21868,#21869,#21870,#21871,#21872,#21873,
#21874,#21875,#21876,#21877,#21878,#21879,#21880,#21881,#21882,#21883,#21884,
#21885,#21886,#21887,#21888,#21889,#21890,#21891,#21892,#21893,#21894,#21895,
#21896,#21897,#21898,#21899,#21900,#21901,#21902,#21903,#21904,#21905,#21906,
#21907,#21908,#21909,#21910,#21911,#21912,#21913,#21914,#21915,#21916,#21917,
#21918,#21919,#21920,#21921,#21922,#21923,#21924,#21925,#21926,#21927,#21928,
#21929,#21930,#21931,#21932,#21933,#21934,#21935,#21936,#21937,#21938,#21939,
#21940,#21941,#21942,#21943,#21944,#21945,#21946,#21947,#21948,#21949,#21950,
#21951,#21952,#21953,#21954,#21955,#21956,#21957,#21958,#21959,#21960,#21961,
#21962,#21963,#21964,#21965,#21966,#21967,#21968,#21969,#21970,#21971,#21972,
#21973,#21974,#21975,#21976,#21977,#21978,#21979,#21980,#21981,#21982,#21983,
#21984,#21985,#21986,#21987,#21988,#21989,#21990,#21991,#21992,#21993,#21994,
#21995,#21996,#21997,#21998,#21999,#22000,#22001,#22002,#22003,#22004,#22005,
#22006,#22007,#22008,#22009,#22010,#22011,#22012,#22013,#22014,#22015,#22016,
#22017,#22018,#22019,#22020,#22021,#22022,#22023,#22024,#22025,#22026,#22027,
#22028,#22029,#22030,#22031,#22032,#22033,#22034,#22035,#22036,#22037,#22038,
#22039,#22040,#22041,#22042,#22043,#22044,#22045,#22046,#22047,#22048,#22049,
#22050,#22051,#22052,#22053,#22054,#22055,#22056,#22057,#22058,#22059,#22060,
#22061,#22062,#22063,#22064,#22065,#22066,#22067,#22068,#22069,#22070,#22071,
#22072,#22073,#22074,#22075,#22076,#22077,#22078,#22079,#22080,#22081,#22082,
#22083,#22084,#22085,#22086,#22087,#22088,#22089,#22090,#22091,#22092,#22093,
#22094,#22095,#22096,#22097,#22098,#22099,#22100,#22101,#22102,#22103,#22104,
#22105,#22106,#22107,#22108,#22109,#22110,#22111,#22112,#22113,#22114,#22115,
#22116,#22117,#22118,#22119,#22120,#22121,#22122,#22123,#22124,#22125,#22126,
#22127,#22128,#22129,#22130,#22131,#22132,#22133,#22134,#22135,#22136,#22137,
#22138,#22139,#22140,#22141,#22142,#22143,#22144,#22145,#22146,#22147,#22148,
#22149,#22150,#22151,#22152,#22153,#22154,#22155,#22156,#22157,#22158,#22159,
#22160,#22161,#22162,#22163,#22164,#22165,#22166,#22167,#22168,#22169,#22170,
#22171,#22172,#22173,#22174,#22175,#22176,#22177,#22178,#22179,#22180,#22181,
#22182,#22183,#22184,#22185,#22186,#22187,#22188,#22189,#22190,#22191,#22192,
#22193,#22194,#22195,#22196,#22197,#22198,#22199,#22200,#22201,#22202,#22203,
#22204,#22205,#22206,#22207,#22208,#22209,#22210,#22211,#22212,#22213,#22214,
#22215,#22216,#22217,#22218,#22219,#22220,#22221,#22222,#22223,#22224,#22225,
#22226,#22227,#22228,#22229,#22230,#22231,#22232,#22233,#22234,#22235,#22236,
#22237,#22238,#22239,#22240,#22241,#22242,#22243,#22244,#22245,#22246,#22247,
#22248,#22249,#22250,#22251,#22252,#22253,#22254,#22255,#22256,#22257,#22258,
#22259,#22260,#22261,#22262,#22263,#22264,#22265,#22266,#22267,#22268,#22269,
#22270,#22271,#22272,#22273,#22274,#22275,#22276,#22277,#22278,#22279,#22280,
#22281,#22282,#22283,#22284,#22285,#22286,#22287,#22288,#22289,#22290,#22291,
#22292,#22293,#22294,#22295,#22296,#22297,#22298,#22299,#22300,#22301,#22302,
#22303,#22304,#22305,#22306,#22307,#22308,#22309,#22310,#22311,#22312,#22313,
#22314,#22315,#22316,#22317,#22318,#22319,#22320,#22321,#22322,#22323,#22324,
#22325,#22326,#22327,#22328,#22329,#22330,#22331,#22332,#22333,#22334,#22335,
#22336,#22337,#22338,#22339,#22340,#22341,#22342,#22343,#22344,#22345,#22346,
#22347,#22348,#22349,#22350,#22351,#22352,#22353,#22354,#22355,#22356,#22357,
#22358,#22359,#22360,#22361,#22362,#22363,#22364,#22365,#22366,#22367,#22368,
#22369,#22370,#22371,#22372,#22373,#22374,#22375,#22376,#22377,#22378,#22379,
#22380,#22381,#22382,#22383,#22384,#22385,#22386,#22387,#22388,#22389,#22390,
#22391,#22392,#22393,#22394,#22395,#22396,#22397,#22398,#22399,#22400,#22401,
#22402,#22403,#22404,#22405,#22406,#22407,#22408,#22409,#22410,#22411,#22412,
#22413,#22414,#22415,#22416,#22417,#22418,#22419,#22420,#22421,#22422,#22423,
#22424,#22425,#22426,#22427,#22428,#22429,#22430,#22431,#22432,#22433,#22434,
#22435,#22436,#22437,#22438,#22439,#22440,#22441,#22442,#22443,#22444,#22445,
#22446,#22447,#22448,#22449,#22450,#22451,#22452,#22453,#22454,#22455,#22456,
#22457,#22458,#22459,#22460,#22461,#22462,#22463,#22464,#22465,#22466,#22467,
#22468,#22469,#22470,#22471,#22472,#22473,#22474,#22475,#22476,#22477,#22478,
#22479,#22480,#22481,#22482,#22483,#22484,#22485,#22486,#22487,#22488,#22489,
#22490,#22491,#22492,#22493,#22494,#22495,#22496,#22497,#22498,#22499,#22500,
#22501,#22502,#22503,#22504,#22505,#22506,#22507,#22508,#22509,#22510,#22511,
#22512,#22513,#22514,#22515,#22516,#22517,#22518,#22519,#22520,#22521,#22522,
#22523,#22524,#22525,#22526,#22527,#22528,#22529,#22530,#22531,#22532,#22533,
#22534,#22535,#22536,#22537,#22538,#22539,#22540,#22541,#22542,#22543,#22544,
#22545,#22546,#22547,#22548,#22549,#22550,#22551,#22552,#22553,#22554,#22555,
#22556,#22557,#22558,#22559,#22560,#22561,#22562,#22563,#22564,#22565,#22566,
#22567,#22568,#22569,#22570,#22571,#22572,#22573,#22574,#22575,#22576,#22577,
#22578,#22579,#22580,#22581,#22582,#22583,#22584,#22585,#22586,#22587,#22588,
#22589,#22590,#22591,#22592,#22593,#22594,#22595,#22596,#22597,#22598,#22599,
#22600,#22601,#22602,#22603,#22604,#22605,#22606,#22607,#22608,#22609,#22610,
#22611,#22612,#22613,#22614,#22615,#22616,#22617,#22618,#22619,#22620,#22621,
#22622,#22623,#22624,#22625,#22626,#22627,#22628,#22629,#22630),(#22631,
#22632,#22633,#22634,#22635,#22636,#22637,#22638,#22639,#22640,#22641,#22642,
#22643,#22644,#22645,#22646,#22647,#22648,#22649,#22650,#22651,#22652,#22653,
#22654,#22655,#22656,#22657,#22658,#22659,#22660,#22661,#22662,#22663,#22664,
#22665,#22666,#22667,#22668,#22669,#22670,#22671,#22672,#22673,#22674,#22675,
#22676,#22677,#22678,#22679,#22680,#22681,#22682,#22683,#22684,#22685,#22686,
#22687,#22688,#22689,#22690,#22691,#22692,#22693,#22694,#22695,#22696,#22697,
#22698,#22699,#22700,#22701,#22702,#22703,#22704,#22705,#22706,#22707,#22708,
#22709,#22710,#22711,#22712,#22713,#22714,#22715,#22716,#22717,#22718,#22719,
#22720,#22721,#22722,#22723,#22724,#22725,#22726,#22727,#22728,#22729,#22730,
#22731,#22732,#22733,#22734,#22735,#22736,#22737,#22738,#22739,#22740,#22741,
#22742,#22743,#22744,#22745,#22746,#22747,#22748,#22749,#22750,#22751,#22752,
#22753,#22754,#22755,#22756,#22757,#22758,#22759,#22760,#22761,#22762,#22763,
#22764,#22765,#22766,#22767,#22768,#22769,#22770,#22771,#22772,#22773,#22774,
#22775,#22776,#22777,#22778,#22779,#22780,#22781,#22782,#22783,#22784,#22785,
#22786,#22787,#22788,#22789,#22790,#22791,#22792,#22793,#22794,#22795,#22796,
#22797,#22798,#22799,#22800,#22801,#22802,#22803,#22804,#22805,#22806,#22807,
#22808,#22809,#22810,#22811,#22812,#22813,#22814,#22815,#22816,#22817,#22818,
#22819,#22820,#22821,#22822,#22823,#22824,#22825,#22826,#22827,#22828,#22829,
#22830,#22831,#22832,#22833,#22834,#22835,#22836,#22837,#22838,#22839,#22840,
#22841,#22842,#22843,#22844,#22845,#22846,#22847,#22848,#22849,#22850,#22851,
#22852,#22853,#22854,#22855,#22856,#22857,#22858,#22859,#22860,#22861,#22862,
#22863,#22864,#22865,#22866,#22867,#22868,#22869,#22870,#22871,#22872,#22873,
#22874,#22875,#22876,#22877,#22878,#22879,#22880,#22881,#22882,#22883,#22884,
#22885,#22886,#22887,#22888,#22889,#22890,#22891,#22892,#22893,#22894,#22895,
#22896,#22897,#22898,#22899,#22900,#22901,#22902,#22903,#22904,#22905,#22906,
#22907,#22908,#22909,#22910,#22911,#22912,#22913,#22914,#22915,#22916,#22917,
#22918,#22919,#22920,#22921,#22922,#22923,#22924,#22925,#22926,#22927,#22928,
#22929,#22930,#22931,#22932,#22933,#22934,#22935,#22936,#22937,#22938,#22939,
#22940,#22941,#22942,#22943,#22944,#22945,#22946,#22947,#22948,#22949,#22950,
#22951,#22952,#22953,#22954,#22955,#22956,#22957,#22958,#22959,#22960,#22961,
#22962,#22963,#22964,#22965,#22966,#22967,#22968,#22969,#22970,#22971,#22972,
#22973,#22974,#22975,#22976,#22977,#22978,#22979,#22980,#22981,#22982,#22983,
#22984,#22985,#22986,#22987,#22988,#22989,#22990,#22991,#22992,#22993,#22994,
#22995,#22996,#22997,#22998,#22999,#23000,#23001,#23002,#23003,#23004,#23005,
#23006,#23007,#23008,#23009,#23010,#23011,#23012,#23013,#23014,#23015,#23016,
#23017,#23018,#23019,#23020,#23021,#23022,#23023,#23024,#23025,#23026,#23027,
#23028,#23029,#23030,#23031,#23032,#23033,#23034,#23035,#23036,#23037,#23038,
#23039,#23040,#23041,#23042,#23043,#23044,#23045,#23046,#23047,#23048,#23049,
#23050,#23051,#23052,#23053,#23054,#23055,#23056,#23057,#23058,#23059,#23060,
#23061,#23062,#23063,#23064,#23065,#23066,#23067,#23068,#23069,#23070,#23071,
#23072,#23073,#23074,#23075,#23076,#23077,#23078,#23079,#23080,#23081,#23082,
#23083,#23084,#23085,#23086,#23087,#23088,#23089,#23090,#23091,#23092,#23093,
#23094,#23095,#23096,#23097,#23098,#23099,#23100,#23101,#23102,#23103,#23104,
#23105,#23106,#23107,#23108,#23109,#23110,#23111,#23112,#23113,#23114,#23115,
#23116,#23117,#23118,#23119,#23120,#23121,#23122,#23123,#23124,#23125,#23126,
#23127,#23128,#23129,#23130,#23131,#23132,#23133,#23134,#23135,#23136,#23137,
#23138,#23139,#23140,#23141,#23142,#23143,#23144,#23145,#23146,#23147,#23148,
#23149,#23150,#23151,#23152,#23153,#23154,#23155,#23156,#23157,#23158,#23159,
#23160,#23161,#23162,#23163,#23164,#23165,#23166,#23167,#23168,#23169,#23170,
#23171,#23172,#23173,#23174,#23175,#23176,#23177,#23178,#23179,#23180,#23181,
#23182,#23183,#23184,#23185,#23186,#23187,#23188,#23189,#23190,#23191,#23192,
#23193,#23194,#23195,#23196,#23197,#23198,#23199,#23200,#23201,#23202,#23203,
#23204,#23205,#23206,#23207,#23208,#23209,#23210,#23211,#23212,#23213,#23214,
#23215,#23216,#23217,#23218,#23219,#23220,#23221,#23222,#23223,#23224,#23225,
#23226,#23227,#23228,#23229,#23230,#23231,#23232,#23233,#23234,#23235,#23236,
#23237,#23238,#23239,#23240,#23241,#23242,#23243,#23244,#23245,#23246,#23247,
#23248,#23249,#23250,#23251,#23252,#23253,#23254,#23255,#23256,#23257,#23258,
#23259,#23260,#23261,#23262,#23263,#23264,#23265,#23266,#23267,#23268,#23269,
#23270,#23271,#23272,#23273,#23274,#23275,#23276,#23277,#23278,#23279,#23280,
#23281,#23282,#23283,#23284,#23285,#23286,#23287,#23288,#23289,#23290,#23291,
#23292,#23293,#23294,#23295,#23296,#23297,#23298,#23299,#23300,#23301,#23302,
#23303,#23304,#23305,#23306,#23307,#23308,#23309,#23310,#23311,#23312,#23313,
#23314,#23315,#23316,#23317,#23318,#23319,#23320,#23321,#23322,#23323,#23324,
#23325,#23326,#23327,#23328,#23329,#23330,#23331,#23332,#23333,#23334,#23335,
#23336,#23337,#23338,#23339,#23340,#23341,#23342,#23343,#23344,#23345,#23346,
#23347,#23348,#23349,#23350,#23351,#23352,#23353,#23354,#23355,#23356,#23357,
#23358,#23359,#23360,#23361,#23362,#23363,#23364,#23365,#23366,#23367,#23368,
#23369,#23370,#23371,#23372,#23373,#23374,#23375,#23376,#23377,#23378,#23379,
#23380,#23381,#23382,#23383,#23384,#23385,#23386,#23387,#23388,#23389,#23390,
#23391,#23392,#23393,#23394,#23395,#23396,#23397,#23398,#23399,#23400,#23401,
#23402,#23403,#23404,#23405,#23406,#23407,#23408,#23409,#23410,#23411,#23412,
#23413,#23414,#23415,#23416,#23417,#23418,#23419,#23420,#23421,#23422,#23423,
#23424,#23425,#23426,#23427,#23428,#23429,#23430,#23431,#23432,#23433,#23434,
#23435,#23436,#23437,#23438,#23439,#23440,#23441,#23442,#23443,#23444,#23445,
#23446,#23447,#23448,#23449,#23450,#23451,#23452,#23453,#23454,#23455,#23456,
#23457,#23458,#23459,#23460,#23461,#23462,#23463,#23464,#23465,#23466,#23467,
#23468,#23469,#23470,#23471,#23472,#23473,#23474,#23475,#23476,#23477,#23478,
#23479,#23480,#23481,#23482,#23483,#23484,#23485,#23486,#23487,#23488,#23489,
#23490,#23491,#23492,#23493,#23494,#23495,#23496,#23497,#23498,#23499,#23500,
#23501,#23502,#23503,#23504,#23505,#23506,#23507,#23508,#23509,#23510,#23511,
#23512,#23513,#23514,#23515,#23516,#23517,#23518,#23519,#23520,#23521,#23522,
#23523,#23524,#23525,#23526,#23527,#23528,#23529,#23530,#23531,#23532,#23533,
#23534,#23535,#23536,#23537,#23538,#23539,#23540,#23541,#23542,#23543,#23544,
#23545,#23546,#23547,#23548,#23549,#23550,#23551,#23552,#23553,#23554,#23555,
#23556,#23557,#23558,#23559,#23560,#23561,#23562,#23563,#23564,#23565,#23566,
#23567,#23568,#23569,#23570,#23571,#23572,#23573,#23574,#23575,#23576,#23577,
#23578,#23579,#23580,#23581,#23582,#23583,#23584,#23585,#23586,#23587,#23588,
#23589,#23590,#23591,#23592,#23593,#23594,#23595,#23596,#23597,#23598,#23599,
#23600,#23601,#23602,#23603),(#23604,#23605,#23606,#23607,#23608,#23609,
#23610,#23611,#23612,#23613,#23614,#23615,#23616,#23617,#23618,#23619,#23620,
#23621,#23622,#23623,#23624,#23625,#23626,#23627,#23628,#23629,#23630,#23631,
#23632,#23633,#23634,#23635,#23636,#23637,#23638,#23639,#23640,#23641,#23642,
#23643,#23644,#23645,#23646,#23647,#23648,#23649,#23650,#23651,#23652,#23653,
#23654,#23655,#23656,#23657,#23658,#23659,#23660,#23661,#23662,#23663,#23664,
#23665,#23666,#23667,#23668,#23669,#23670,#23671,#23672,#23673,#23674,#23675,
#23676,#23677,#23678,#23679,#23680,#23681,#23682,#23683,#23684,#23685,#23686,
#23687,#23688,#23689,#23690,#23691,#23692,#23693,#23694,#23695,#23696,#23697,
#23698,#23699,#23700,#23701,#23702,#23703,#23704,#23705,#23706,#23707,#23708,
#23709,#23710,#23711,#23712,#23713,#23714,#23715,#23716,#23717,#23718,#23719,
#23720,#23721,#23722,#23723,#23724,#23725,#23726,#23727,#23728,#23729,#23730,
#23731,#23732,#23733,#23734,#23735,#23736,#23737,#23738,#23739,#23740,#23741,
#23742,#23743,#23744,#23745,#23746,#23747,#23748,#23749,#23750,#23751,#23752,
#23753,#23754,#23755,#23756,#23757,#23758,#23759,#23760,#23761,#23762,#23763,
#23764,#23765,#23766,#23767,#23768,#23769,#23770,#23771,#23772,#23773,#23774,
#23775,#23776,#23777,#23778,#23779,#23780,#23781,#23782,#23783,#23784,#23785,
#23786,#23787,#23788,#23789,#23790,#23791,#23792,#23793,#23794,#23795,#23796,
#23797,#23798,#23799,#23800,#23801,#23802,#23803,#23804,#23805,#23806,#23807,
#23808,#23809,#23810,#23811,#23812,#23813,#23814,#23815,#23816,#23817,#23818,
#23819,#23820,#23821,#23822,#23823,#23824,#23825,#23826,#23827,#23828,#23829,
#23830,#23831,#23832,#23833,#23834,#23835,#23836,#23837,#23838,#23839,#23840,
#23841,#23842,#23843,#23844,#23845,#23846,#23847,#23848,#23849,#23850,#23851,
#23852,#23853,#23854,#23855,#23856,#23857,#23858,#23859,#23860,#23861,#23862,
#23863,#23864,#23865,#23866,#23867,#23868,#23869,#23870,#23871,#23872,#23873,
#23874,#23875,#23876,#23877,#23878,#23879,#23880,#23881,#23882,#23883,#23884,
#23885,#23886,#23887,#23888,#23889,#23890,#23891,#23892,#23893,#23894,#23895,
#23896,#23897,#23898,#23899,#23900,#23901,#23902,#23903,#23904,#23905,#23906,
#23907,#23908,#23909,#23910,#23911,#23912,#23913,#23914,#23915,#23916,#23917,
#23918,#23919,#23920,#23921,#23922,#23923,#23924,#23925,#23926,#23927,#23928,
#23929,#23930,#23931,#23932,#23933,#23934,#23935,#23936,#23937,#23938,#23939,
#23940,#23941,#23942,#23943,#23944,#23945,#23946,#23947,#23948,#23949,#23950,
#23951,#23952,#23953,#23954,#23955,#23956,#23957,#23958,#23959,#23960,#23961,
#23962,#23963,#23964,#23965,#23966,#23967,#23968,#23969,#23970,#23971,#23972,
#23973,#23974,#23975,#23976,#23977,#23978,#23979,#23980,#23981,#23982,#23983,
#23984,#23985,#23986,#23987,#23988,#23989,#23990,#23991,#23992,#23993,#23994,
#23995,#23996,#23997,#23998,#23999,#24000,#24001,#24002,#24003,#24004,#24005,
#24006,#24007,#24008,#24009,#24010,#24011,#24012,#24013,#24014,#24015,#24016,
#24017,#24018,#24019,#24020,#24021,#24022,#24023,#24024,#24025,#24026,#24027,
#24028,#24029,#24030,#24031,#24032,#24033,#24034,#24035,#24036,#24037,#24038,
#24039,#24040,#24041,#24042,#24043,#24044,#24045,#24046,#24047,#24048,#24049,
#24050,#24051,#24052,#24053,#24054,#24055,#24056,#24057,#24058,#24059,#24060,
#24061,#24062,#24063,#24064,#24065,#24066,#24067,#24068,#24069,#24070,#24071,
#24072,#24073,#24074,#24075,#24076,#24077,#24078,#24079,#24080,#24081,#24082,
#24083,#24084,#24085,#24086,#24087,#24088,#24089,#24090,#24091,#24092,#24093,
#24094,#24095,#24096,#24097,#24098,#24099,#24100,#24101,#24102,#24103,#24104,
#24105,#24106,#24107,#24108,#24109,#24110,#24111,#24112,#24113,#24114,#24115,
#24116,#24117,#24118,#24119,#24120,#24121,#24122,#24123,#24124,#24125,#24126,
#24127,#24128,#24129,#24130,#24131,#24132,#24133,#24134,#24135,#24136,#24137,
#24138,#24139,#24140,#24141,#24142,#24143,#24144,#24145,#24146,#24147,#24148,
#24149,#24150,#24151,#24152,#24153,#24154,#24155,#24156,#24157,#24158,#24159,
#24160,#24161,#24162,#24163,#24164,#24165,#24166,#24167,#24168,#24169,#24170,
#24171,#24172,#24173,#24174,#24175,#24176,#24177,#24178,#24179,#24180,#24181,
#24182,#24183,#24184,#24185,#24186,#24187,#24188,#24189,#24190,#24191,#24192,
#24193,#24194,#24195,#24196,#24197,#24198,#24199,#24200,#24201,#24202,#24203,
#24204,#24205,#24206,#24207,#24208,#24209,#24210,#24211,#24212,#24213,#24214,
#24215,#24216,#24217,#24218,#24219,#24220,#24221,#24222,#24223,#24224,#24225,
#24226,#24227,#24228,#24229,#24230,#24231,#24232,#24233,#24234,#24235,#24236,
#24237,#24238,#24239,#24240,#24241,#24242,#24243,#24244,#24245,#24246,#24247,
#24248,#24249,#24250,#24251,#24252,#24253,#24254,#24255,#24256,#24257,#24258,
#24259,#24260,#24261,#24262,#24263,#24264,#24265,#24266,#24267,#24268,#24269,
#24270,#24271,#24272,#24273,#24274,#24275,#24276,#24277,#24278,#24279,#24280,
#24281,#24282,#24283,#24284,#24285,#24286,#24287,#24288,#24289,#24290,#24291,
#24292,#24293,#24294,#24295,#24296,#24297,#24298,#24299,#24300,#24301,#24302,
#24303,#24304,#24305,#24306,#24307,#24308,#24309,#24310,#24311,#24312,#24313,
#24314,#24315,#24316,#24317,#24318,#24319,#24320,#24321,#24322,#24323,#24324,
#24325,#24326,#24327,#24328,#24329,#24330,#24331,#24332,#24333,#24334,#24335,
#24336,#24337,#24338,#24339,#24340,#24341,#24342,#24343,#24344,#24345,#24346,
#24347,#24348,#24349,#24350,#24351,#24352,#24353,#24354,#24355,#24356,#24357,
#24358,#24359,#24360,#24361,#24362,#24363,#24364,#24365,#24366,#24367,#24368,
#24369,#24370,#24371,#24372,#24373,#24374,#24375,#24376,#24377,#24378,#24379,
#24380,#24381,#24382,#24383,#24384,#24385,#24386,#24387,#24388,#24389,#24390,
#24391,#24392,#24393,#24394,#24395,#24396,#24397,#24398,#24399,#24400,#24401,
#24402,#24403,#24404,#24405,#24406,#24407,#24408,#24409,#24410,#24411,#24412,
#24413,#24414,#24415,#24416,#24417,#24418,#24419,#24420,#24421,#24422,#24423,
#24424,#24425,#24426,#24427,#24428,#24429,#24430,#24431,#24432,#24433,#24434,
#24435,#24436,#24437,#24438,#24439,#24440,#24441,#24442,#24443,#24444,#24445,
#24446,#24447,#24448,#24449,#24450,#24451,#24452,#24453,#24454,#24455,#24456,
#24457,#24458,#24459,#24460,#24461,#24462,#24463,#24464,#24465,#24466,#24467,
#24468,#24469,#24470,#24471,#24472,#24473,#24474,#24475,#24476,#24477,#24478,
#24479,#24480,#24481,#24482,#24483,#24484,#24485,#24486,#24487,#24488,#24489,
#24490,#24491,#24492,#24493,#24494,#24495,#24496,#24497,#24498,#24499,#24500,
#24501,#24502,#24503,#24504,#24505,#24506,#24507,#24508,#24509,#24510,#24511,
#24512,#24513,#24514,#24515,#24516,#24517,#24518,#24519,#24520,#24521,#24522,
#24523,#24524,#24525,#24526,#24527,#24528,#24529,#24530,#24531,#24532,#24533,
#24534,#24535,#24536,#24537,#24538,#24539,#24540,#24541,#24542,#24543,#24544,
#24545,#24546,#24547,#24548,#24549,#24550,#24551,#24552,#24553,#24554,#24555,
#24556,#24557,#24558,#24559,#24560,#24561,#24562,#24563,#24564,#24565,#24566,
#24567,#24568,#24569,#24570,#24571,#24572,#24573,#24574,#24575,#24576),
(#24577,#24578,#24579,#24580,#24581,#24582,#24583,#24584,#24585,#24586,
#24587,#24588,#24589,#24590,#24591,#24592,#24593,#24594,#24595,#24596,#24597,
#24598,#24599,#24600,#24601,#24602,#24603,#24604,#24605,#24606,#24607,#24608,
#24609,#24610,#24611,#24612,#24613,#24614,#24615,#24616,#24617,#24618,#24619,
#24620,#24621,#24622,#24623,#24624,#24625,#24626,#24627,#24628,#24629,#24630,
#24631,#24632,#24633,#24634,#24635,#24636,#24637,#24638,#24639,#24640,#24641,
#24642,#24643,#24644,#24645,#24646,#24647,#24648,#24649,#24650,#24651,#24652,
#24653,#24654,#24655,#24656,#24657,#24658,#24659,#24660,#24661,#24662,#24663,
#24664,#24665,#24666,#24667,#24668,#24669,#24670,#24671,#24672,#24673,#24674,
#24675,#24676,#24677,#24678,#24679,#24680,#24681,#24682,#24683,#24684,#24685,
#24686,#24687,#24688,#24689,#24690,#24691,#24692,#24693,#24694,#24695,#24696,
#24697,#24698,#24699,#24700,#24701,#24702,#24703,#24704,#24705,#24706,#24707,
#24708,#24709,#24710,#24711,#24712,#24713,#24714,#24715,#24716,#24717,#24718,
#24719,#24720,#24721,#24722,#24723,#24724,#24725,#24726,#24727,#24728,#24729,
#24730,#24731,#24732,#24733,#24734,#24735,#24736,#24737,#24738,#24739,#24740,
#24741,#24742,#24743,#24744,#24745,#24746,#24747,#24748,#24749,#24750,#24751,
#24752,#24753,#24754,#24755,#24756,#24757,#24758,#24759,#24760,#24761,#24762,
#24763,#24764,#24765,#24766,#24767,#24768,#24769,#24770,#24771,#24772,#24773,
#24774,#24775,#24776,#24777,#24778,#24779,#24780,#24781,#24782,#24783,#24784,
#24785,#24786,#24787,#24788,#24789,#24790,#24791,#24792,#24793,#24794,#24795,
#24796,#24797,#24798,#24799,#24800,#24801,#24802,#24803,#24804,#24805,#24806,
#24807,#24808,#24809,#24810,#24811,#24812,#24813,#24814,#24815,#24816,#24817,
#24818,#24819,#24820,#24821,#24822,#24823,#24824,#24825,#24826,#24827,#24828,
#24829,#24830,#24831,#24832,#24833,#24834,#24835,#24836,#24837,#24838,#24839,
#24840,#24841,#24842,#24843,#24844,#24845,#24846,#24847,#24848,#24849,#24850,
#24851,#24852,#24853,#24854,#24855,#24856,#24857,#24858,#24859,#24860,#24861,
#24862,#24863,#24864,#24865,#24866,#24867,#24868,#24869,#24870,#24871,#24872,
#24873,#24874,#24875,#24876,#24877,#24878,#24879,#24880,#24881,#24882,#24883,
#24884,#24885,#24886,#24887,#24888,#24889,#24890,#24891,#24892,#24893,#24894,
#24895,#24896,#24897,#24898,#24899,#24900,#24901,#24902,#24903,#24904,#24905,
#24906,#24907,#24908,#24909,#24910,#24911,#24912,#24913,#24914,#24915,#24916,
#24917,#24918,#24919,#24920,#24921,#24922,#24923,#24924,#24925,#24926,#24927,
#24928,#24929,#24930,#24931,#24932,#24933,#24934,#24935,#24936,#24937,#24938,
#24939,#24940,#24941,#24942,#24943,#24944,#24945,#24946,#24947,#24948,#24949,
#24950,#24951,#24952,#24953,#24954,#24955,#24956,#24957,#24958,#24959,#24960,
#24961,#24962,#24963,#24964,#24965,#24966,#24967,#24968,#24969,#24970,#24971,
#24972,#24973,#24974,#24975,#24976,#24977,#24978,#24979,#24980,#24981,#24982,
#24983,#24984,#24985,#24986,#24987,#24988,#24989,#24990,#24991,#24992,#24993,
#24994,#24995,#24996,#24997,#24998,#24999,#25000,#25001,#25002,#25003,#25004,
#25005,#25006,#25007,#25008,#25009,#25010,#25011,#25012,#25013,#25014,#25015,
#25016,#25017,#25018,#25019,#25020,#25021,#25022,#25023,#25024,#25025,#25026,
#25027,#25028,#25029,#25030,#25031,#25032,#25033,#25034,#25035,#25036,#25037,
#25038,#25039,#25040,#25041,#25042,#25043,#25044,#25045,#25046,#25047,#25048,
#25049,#25050,#25051,#25052,#25053,#25054,#25055,#25056,#25057,#25058,#25059,
#25060,#25061,#25062,#25063,#25064,#25065,#25066,#25067,#25068,#25069,#25070,
#25071,#25072,#25073,#25074,#25075,#25076,#25077,#25078,#25079,#25080,#25081,
#25082,#25083,#25084,#25085,#25086,#25087,#25088,#25089,#25090,#25091,#25092,
#25093,#25094,#25095,#25096,#25097,#25098,#25099,#25100,#25101,#25102,#25103,
#25104,#25105,#25106,#25107,#25108,#25109,#25110,#25111,#25112,#25113,#25114,
#25115,#25116,#25117,#25118,#25119,#25120,#25121,#25122,#25123,#25124,#25125,
#25126,#25127,#25128,#25129,#25130,#25131,#25132,#25133,#25134,#25135,#25136,
#25137,#25138,#25139,#25140,#25141,#25142,#25143,#25144,#25145,#25146,#25147,
#25148,#25149,#25150,#25151,#25152,#25153,#25154,#25155,#25156,#25157,#25158,
#25159,#25160,#25161,#25162,#25163,#25164,#25165,#25166,#25167,#25168,#25169,
#25170,#25171,#25172,#25173,#25174,#25175,#25176,#25177,#25178,#25179,#25180,
#25181,#25182,#25183,#25184,#25185,#25186,#25187,#25188,#25189,#25190,#25191,
#25192,#25193,#25194,#25195,#25196,#25197,#25198,#25199,#25200,#25201,#25202,
#25203,#25204,#25205,#25206,#25207,#25208,#25209,#25210,#25211,#25212,#25213,
#25214,#25215,#25216,#25217,#25218,#25219,#25220,#25221,#25222,#25223,#25224,
#25225,#25226,#25227,#25228,#25229,#25230,#25231,#25232,#25233,#25234,#25235,
#25236,#25237,#25238,#25239,#25240,#25241,#25242,#25243,#25244,#25245,#25246,
#25247,#25248,#25249,#25250,#25251,#25252,#25253,#25254,#25255,#25256,#25257,
#25258,#25259,#25260,#25261,#25262,#25263,#25264,#25265,#25266,#25267,#25268,
#25269,#25270,#25271,#25272,#25273,#25274,#25275,#25276,#25277,#25278,#25279,
#25280,#25281,#25282,#25283,#25284,#25285,#25286,#25287,#25288,#25289,#25290,
#25291,#25292,#25293,#25294,#25295,#25296,#25297,#25298,#25299,#25300,#25301,
#25302,#25303,#25304,#25305,#25306,#25307,#25308,#25309,#25310,#25311,#25312,
#25313,#25314,#25315,#25316,#25317,#25318,#25319,#25320,#25321,#25322,#25323,
#25324,#25325,#25326,#25327,#25328,#25329,#25330,#25331,#25332,#25333,#25334,
#25335,#25336,#25337,#25338,#25339,#25340,#25341,#25342,#25343,#25344,#25345,
#25346,#25347,#25348,#25349,#25350,#25351,#25352,#25353,#25354,#25355,#25356,
#25357,#25358,#25359,#25360,#25361,#25362,#25363,#25364,#25365,#25366,#25367,
#25368,#25369,#25370,#25371,#25372,#25373,#25374,#25375,#25376,#25377,#25378,
#25379,#25380,#25381,#25382,#25383,#25384,#25385,#25386,#25387,#25388,#25389,
#25390,#25391,#25392,#25393,#25394,#25395,#25396,#25397,#25398,#25399,#25400,
#25401,#25402,#25403,#25404,#25405,#25406,#25407,#25408,#25409,#25410,#25411,
#25412,#25413,#25414,#25415,#25416,#25417,#25418,#25419,#25420,#25421,#25422,
#25423,#25424,#25425,#25426,#25427,#25428,#25429,#25430,#25431,#25432,#25433,
#25434,#25435,#25436,#25437,#25438,#25439,#25440,#25441,#25442,#25443,#25444,
#25445,#25446,#25447,#25448,#25449,#25450,#25451,#25452,#25453,#25454,#25455,
#25456,#25457,#25458,#25459,#25460,#25461,#25462,#25463,#25464,#25465,#25466,
#25467,#25468,#25469,#25470,#25471,#25472,#25473,#25474,#25475,#25476,#25477,
#25478,#25479,#25480,#25481,#25482,#25483,#25484,#25485,#25486,#25487,#25488,
#25489,#25490,#25491,#25492,#25493,#25494,#25495,#25496,#25497,#25498,#25499,
#25500,#25501,#25502,#25503,#25504,#25505,#25506,#25507,#25508,#25509,#25510,
#25511,#25512,#25513,#25514,#25515,#25516,#25517,#25518,#25519,#25520,#25521,
#25522,#25523,#25524,#25525,#25526,#25527,#25528,#25529,#25530,#25531,#25532,
#25533,#25534,#25535,#25536,#25537,#25538,#25539,#25540,#25541,#25542,#25543,
#25544,#25545,#25546,#25547,#25548,#25549)),.UNSPECIFIED.,.F.,.F.,.F.)
B_SPLINE_SURFACE_WITH_KNOTS((4,4),(3,2,2,2,2,2,2,2,2,2,2,2,2,2,2,2,2,2,
2,2,2,2,2,2,2,2,2,2,2,2,2,2,2,2,2,2,2,2,2,2,2,2,2,2,2,2,2,2,2,2,2,2,2,2,
2,2,2,2,2,2,2,2,2,2,2,2,2,2,2,2,2,2,2,2,2,2,2,2,2,2,2,2,2,2,2,2,2,2,2,2,
2,2,2,2,2,2,2,2,2,2,2,2,2,2,2,2,2,2,2,2,2,2,2,2,2,2,2,2,2,2,2,2,2,2,2,2,
2,2,2,2,2,2,2,2,2,2,2,2,2,2,2,2,2,2,2,2,2,2,2,2,2,2,2,2,2,2,2,2,2,2,2,2,
2,2,2,2,2,2,2,2,2,2,2,2,2,2,2,2,2,2,2,2,2,2,2,2,2,2,2,2,2,2,2,2,2,2,2,2,
2,2,2,2,2,2,2,2,2,2,2,2,2,2,2,2,2,2,2,2,2,2,2,2,2,2,2,2,2,2,2,2,2,2,2,2,
2,2,2,2,2,2,2,2,2,2,2,2,2,2,2,2,2,2,2,2,2,2,2,2,2,2,2,2,2,2,2,2,2,2,2,2,
2,2,2,2,2,2,2,2,2,2,2,2,2,2,2,2,2,2,2,2,2,2,2,2,2,2,2,2,2,2,2,2,2,2,2,2,
2,2,2,2,2,2,2,2,2,2,2,2,2,2,2,2,2,2,2,2,2,2,2,2,2,2,2,2,2,2,2,2,2,2,2,2,
2,2,2,2,2,2,2,2,2,2,2,2,2,2,2,2,2,2,2,2,2,2,2,2,2,2,2,2,2,2,2,2,2,2,2,2,
2,2,2,2,2,2,2,2,2,2,2,2,2,2,2,2,2,2,2,2,2,2,2,2,2,2,2,2,2,2,2,2,2,2,2,2,
2,2,2,2,2,2,2,2,2,2,2,2,2,2,2,2,2,2,2,2,2,2,2,2,2,2,2,2,2,2,2,2,2,2,2,2,
2,2,2,2,2,2,2,2,2,2,2,2,2,2,2,2,2,2,2,2,2,2,2,2,2,2,2,2,2,2,2,2,2,2,2,2,
3),(0.,1.),(0.,0.00205761316872428,0.00411522633744856,0.00617283950617284,
0.00823045267489712,0.0102880658436214,0.0123456790123457,0.01440329218107,
0.0164609053497942,0.0185185185185185,0.0205761316872428,0.0226337448559671,
0.0246913580246914,0.0267489711934156,0.0288065843621399,0.0308641975308642,
0.0329218106995885,0.0349794238683128,0.037037037037037,0.0390946502057613,
0.0411522633744856,0.0432098765432099,0.0452674897119342,0.0473251028806584,
0.0493827160493827,0.051440329218107,0.0534979423868313,0.0555555555555556,
0.0576131687242798,0.0596707818930041,0.0617283950617284,0.0637860082304527,
0.065843621399177,0.0679012345679012,0.0699588477366255,0.0720164609053498,
0.0740740740740741,0.0761316872427984,0.0781893004115226,0.0802469135802469,
0.0823045267489712,0.0843621399176955,0.0864197530864197,0.088477366255144,
0.0905349794238683,0.0925925925925926,0.0946502057613169,0.0967078189300412,
0.0987654320987654,0.10082304526749,0.102880658436214,0.104938271604938,
0.106995884773663,0.109053497942387,0.111111111111111,0.113168724279835,
0.11522633744856,0.117283950617284,0.119341563786008,0.121399176954733,
0.123456790123457,0.125514403292181,0.127572016460905,0.12962962962963,
0.131687242798354,0.133744855967078,0.135802469135802,0.137860082304527,
0.139917695473251,0.141975308641975,0.1440329218107,0.146090534979424,0.148148148148148,
0.150205761316872,0.152263374485597,0.154320987654321,0.156378600823045,
0.15843621399177,0.160493827160494,0.162551440329218,0.164609053497942,
0.166666666666667,0.168724279835391,0.170781893004115,0.172839506172839,
0.174897119341564,0.176954732510288,0.179012345679012,0.181069958847737,
0.183127572016461,0.185185185185185,0.187242798353909,0.189300411522634,
0.191358024691358,0.193415637860082,0.195473251028807,0.197530864197531,
0.199588477366255,0.201646090534979,0.203703703703704,0.205761316872428,
0.207818930041152,0.209876543209877,0.211934156378601,0.213991769547325,
0.216049382716049,0.218106995884774,0.220164609053498,0.222222222222222,
0.224279835390947,0.226337448559671,0.228395061728395,0.230452674897119,
0.232510288065844,0.234567901234568,0.236625514403292,0.238683127572016,
0.240740740740741,0.242798353909465,0.244855967078189,0.246913580246914,
0.248971193415638,0.251028806584362,0.253086419753086,0.255144032921811,
0.257201646090535,0.259259259259259,0.261316872427984,0.263374485596708,
0.265432098765432,0.267489711934156,0.269547325102881,0.271604938271605,
0.273662551440329,0.275720164609054,0.277777777777778,0.279835390946502,
0.281893004115226,0.283950617283951,0.286008230452675,0.288065843621399,
0.290123456790123,0.292181069958848,0.294238683127572,0.296296296296296,
0.298353909465021,0.300411522633745,0.302469135802469,0.304526748971193,
0.306584362139918,0.308641975308642,0.310699588477366,0.312757201646091,
0.314814814814815,0.316872427983539,0.318930041152263,0.320987654320988,
0.323045267489712,0.325102880658436,0.327160493827161,0.329218106995885,
0.331275720164609,0.333333333333333,0.335390946502058,0.337448559670782,
0.339506172839506,0.34156378600823,0.343621399176955,0.345679012345679,
0.347736625514403,0.349794238683128,0.351851851851852,0.353909465020576,
0.3559670781893,0.358024691358025,0.360082304526749,0.362139917695473,0.364197530864198,
0.366255144032922,0.368312757201646,0.37037037037037,0.372427983539095,
0.374485596707819,0.376543209876543,0.378600823045267,0.380658436213992,
0.382716049382716,0.38477366255144,0.386831275720165,0.388888888888889,
0.390946502057613,0.393004115226337,0.395061728395062,0.397119341563786,
0.39917695473251,0.401234567901235,0.403292181069959,0.405349794238683,
0.407407407407407,0.409465020576132,0.411522633744856,0.41358024691358,
0.415637860082305,0.417695473251029,0.419753086419753,0.421810699588477,
0.423868312757202,0.425925925925926,0.42798353909465,0.430041152263374,
0.432098765432099,0.434156378600823,0.436213991769547,0.438271604938272,
0.440329218106996,0.44238683127572,0.444444444444444,0.446502057613169,
0.448559670781893,0.450617283950617,0.452674897119342,0.454732510288066,
0.45679012345679,0.458847736625514,0.460905349794239,0.462962962962963,
0.465020576131687,0.467078189300412,0.469135802469136,0.47119341563786,
0.473251028806584,0.475308641975309,0.477366255144033,0.479423868312757,
0.481481481481481,0.483539094650206,0.48559670781893,0.487654320987654,
0.489711934156379,0.491769547325103,0.493827160493827,0.495884773662551,
0.497942386831276,0.5,0.502057613168724,0.504115226337449,0.506172839506173,
0.508230452674897,0.510288065843621,0.512345679012346,0.51440329218107,
0.516460905349794,0.518518518518518,0.520576131687243,0.522633744855967,
0.524691358024691,0.526748971193416,0.52880658436214,0.530864197530864,
0.532921810699588,0.534979423868313,0.537037037037037,0.539094650205761,
0.541152263374486,0.54320987654321,0.545267489711934,0.547325102880658,
0.549382716049383,0.551440329218107,0.553497942386831,0.555555555555556,
0.55761316872428,0.559670781893004,0.561728395061728,0.563786008230453,
0.565843621399177,0.567901234567901,0.569958847736626,0.57201646090535,
0.574074074074074,0.576131687242798,0.578189300411523,0.580246913580247,
0.582304526748971,0.584362139917695,0.58641975308642,0.588477366255144,
0.590534979423868,0.592592592592593,0.594650205761317,0.596707818930041,
0.598765432098765,0.60082304526749,0.602880658436214,0.604938271604938,
0.606995884773663,0.609053497942387,0.611111111111111,0.613168724279835,
0.61522633744856,0.617283950617284,0.619341563786008,0.621399176954732,
0.623456790123457,0.625514403292181,0.627572016460905,0.62962962962963,
0.631687242798354,0.633744855967078,0.635802469135803,0.637860082304527,
0.639917695473251,0.641975308641975,0.6440329218107,0.646090534979424,0.648148148148148,
0.650205761316872,0.652263374485597,0.654320987654321,0.656378600823045,
0.65843621399177,0.660493827160494,0.662551440329218,0.664609053497942,
0.666666666666667,0.668724279835391,0.670781893004115,0.672839506172839,
0.674897119341564,0.676954732510288,0.679012345679012,0.681069958847737,
0.683127572016461,0.685185185185185,0.687242798353909,0.689300411522634,
0.691358024691358,0.693415637860082,0.695473251028807,0.697530864197531,
0.699588477366255,0.701646090534979,0.703703703703704,0.705761316872428,
0.707818930041152,0.709876543209877,0.711934156378601,0.713991769547325,
0.716049382716049,0.718106995884774,0.720164609053498,0.722222222222222,
0.724279835390947,0.726337448559671,0.728395061728395,0.730452674897119,
0.732510288065844,0.734567901234568,0.736625514403292,0.738683127572016,
0.740740740740741,0.742798353909465,0.744855967078189,0.746913580246914,
0.748971193415638,0.751028806584362,0.753086419753086,0.755144032921811,
0.757201646090535,0.759259259259259,0.761316872427984,0.763374485596708,
0.765432098765432,0.767489711934156,0.769547325102881,0.771604938271605,
0.773662551440329,0.775720164609053,0.777777777777778,0.779835390946502,
0.781893004115226,0.783950617283951,0.786008230452675,0.788065843621399,
0.790123456790123,0.792181069958848,0.794238683127572,0.796296296296296,
0.798353909465021,0.800411522633745,0.802469135802469,0.804526748971193,
0.806584362139918,0.808641975308642,0.810699588477366,0.812757201646091,
0.814814814814815,0.816872427983539,0.818930041152263,0.820987654320988,
0.823045267489712,0.825102880658436,0.827160493827161,0.829218106995885,
0.831275720164609,0.833333333333333,0.835390946502058,0.837448559670782,
0.839506172839506,0.84156378600823,0.843621399176955,0.845679012345679,
0.847736625514403,0.849794238683128,0.851851851851852,0.853909465020576,
0.8559670781893,0.858024691358025,0.860082304526749,0.862139917695473,0.864197530864197,
0.866255144032922,0.868312757201646,0.87037037037037,0.872427983539095,
0.874485596707819,0.876543209876543,0.878600823045268,0.880658436213992,
0.882716049382716,0.88477366255144,0.886831275720165,0.888888888888889,
0.890946502057613,0.893004115226337,0.895061728395062,0.897119341563786,
0.89917695473251,0.901234567901235,0.903292181069959,0.905349794238683,
0.907407407407407,0.909465020576132,0.911522633744856,0.91358024691358,
0.915637860082305,0.917695473251029,0.919753086419753,0.921810699588477,
0.923868312757202,0.925925925925926,0.92798353909465,0.930041152263374,
0.932098765432099,0.934156378600823,0.936213991769547,0.938271604938272,
0.940329218106996,0.94238683127572,0.944444444444444,0.946502057613169,
0.948559670781893,0.950617283950617,0.952674897119342,0.954732510288066,
0.95679012345679,0.958847736625514,0.960905349794239,0.962962962962963,
0.965020576131687,0.967078189300412,0.969135802469136,0.97119341563786,
0.973251028806584,0.975308641975309,0.977366255144033,0.979423868312757,
0.981481481481482,0.983539094650206,0.98559670781893,0.987654320987654,
0.989711934156379,0.991769547325103,0.993827160493827,0.995884773662551,
0.997942386831276,1.),.UNSPECIFIED.)
GEOMETRIC_REPRESENTATION_ITEM()
RATIONAL_B_SPLINE_SURFACE(((1.,0.866025403784439,1.,0.866025403784439,1.,
0.866025403784439,1.,0.866025403784439,1.,0.866025403784439,1.,0.866025403784439,
1.,0.866025403784439,1.,0.866025403784439,1.,0.866025403784439,1.,0.866025403784439,
1.,0.866025403784439,1.,0.866025403784439,1.,0.866025403784439,1.,0.866025403784439,
1.,0.866025403784439,1.,0.866025403784439,1.,0.866025403784439,1.,0.866025403784439,
1.,0.866025403784439,1.,0.866025403784439,1.,0.866025403784439,1.,0.866025403784439,
1.,0.866025403784439,1.,0.866025403784439,1.,0.866025403784439,1.,0.866025403784439,
1.,0.866025403784439,1.,0.866025403784439,1.,0.866025403784439,1.,0.866025403784439,
1.,0.866025403784439,1.,0.866025403784439,1.,0.866025403784439,1.,0.866025403784439,
1.,0.866025403784439,1.,0.866025403784439,1.,0.866025403784439,1.,0.866025403784439,
1.,0.866025403784439,1.,0.866025403784439,1.,0.866025403784439,1.,0.866025403784439,
1.,0.866025403784439,1.,0.866025403784439,1.,0.866025403784439,1.,0.866025403784439,
1.,0.866025403784439,1.,0.866025403784439,1.,0.866025403784439,1.,0.866025403784439,
1.,0.866025403784439,1.,0.866025403784439,1.,0.866025403784439,1.,0.866025403784439,
1.,0.866025403784439,1.,0.866025403784439,1.,0.866025403784439,1.,0.866025403784439,
1.,0.866025403784439,1.,0.866025403784439,1.,0.866025403784439,1.,0.866025403784439,
1.,0.866025403784439,1.,0.866025403784439,1.,0.866025403784439,1.,0.866025403784439,
1.,0.866025403784439,1.,0.866025403784439,1.,0.866025403784439,1.,0.866025403784439,
1.,0.866025403784439,1.,0.866025403784439,1.,0.866025403784439,1.,0.866025403784439,
1.,0.866025403784439,1.,0.866025403784439,1.,0.866025403784439,1.,0.866025403784439,
1.,0.866025403784439,1.,0.866025403784439,1.,0.866025403784439,1.,0.866025403784439,
1.,0.866025403784439,1.,0.866025403784439,1.,0.866025403784439,1.,0.866025403784439,
1.,0.866025403784439,1.,0.866025403784439,1.,0.866025403784439,1.,0.866025403784439,
1.,0.866025403784439,1.,0.866025403784439,1.,0.866025403784439,1.,0.866025403784439,
1.,0.866025403784439,1.,0.866025403784439,1.,0.866025403784439,1.,0.866025403784439,
1.,0.866025403784439,1.,0.866025403784439,1.,0.866025403784439,1.,0.866025403784439,
1.,0.866025403784439,1.,0.866025403784439,1.,0.866025403784439,1.,0.866025403784439,
1.,0.866025403784439,1.,0.866025403784439,1.,0.866025403784439,1.,0.866025403784439,
1.,0.866025403784439,1.,0.866025403784439,1.,0.866025403784439,1.,0.866025403784439,
1.,0.866025403784439,1.,0.866025403784439,1.,0.866025403784439,1.,0.866025403784439,
1.,0.866025403784439,1.,0.866025403784439,1.,0.866025403784439,1.,0.866025403784439,
1.,0.866025403784439,1.,0.866025403784439,1.,0.866025403784439,1.,0.866025403784439,
1.,0.866025403784439,1.,0.866025403784439,1.,0.866025403784439,1.,0.866025403784439,
1.,0.866025403784439,1.,0.866025403784439,1.,0.866025403784439,1.,0.866025403784439,
1.,0.866025403784439,1.,0.866025403784439,1.,0.866025403784439,1.,0.866025403784439,
1.,0.866025403784439,1.,0.866025403784439,1.,0.866025403784439,1.,0.866025403784439,
1.,0.866025403784439,1.,0.866025403784439,1.,0.866025403784439,1.,0.866025403784439,
1.,0.866025403784439,1.,0.866025403784439,1.,0.866025403784439,1.,0.866025403784439,
1.,0.866025403784439,1.,0.866025403784439,1.,0.866025403784439,1.,0.866025403784439,
1.,0.866025403784439,1.,0.866025403784439,1.,0.866025403784439,1.,0.866025403784439,
1.,0.866025403784439,1.,0.866025403784439,1.,0.866025403784439,1.,0.866025403784439,
1.,0.866025403784439,1.,0.866025403784439,1.,0.866025403784439,1.,0.866025403784439,
1.,0.866025403784439,1.,0.866025403784439,1.,0.866025403784439,1.,0.866025403784439,
1.,0.866025403784439,1.,0.866025403784439,1.,0.866025403784439,1.,0.866025403784439,
1.,0.866025403784439,1.,0.866025403784439,1.,0.866025403784439,1.,0.866025403784439,
1.,0.866025403784439,1.,0.866025403784439,1.,0.866025403784439,1.,0.866025403784439,
1.,0.866025403784439,1.,0.866025403784439,1.,0.866025403784439,1.,0.866025403784439,
1.,0.866025403784439,1.,0.866025403784439,1.,0.866025403784439,1.,0.866025403784439,
1.,0.866025403784439,1.,0.866025403784439,1.,0.866025403784439,1.,0.866025403784439,
1.,0.866025403784439,1.,0.866025403784439,1.,0.866025403784439,1.,0.866025403784439,
1.,0.866025403784439,1.,0.866025403784439,1.,0.866025403784439,1.,0.866025403784439,
1.,0.866025403784439,1.,0.866025403784439,1.,0.866025403784439,1.,0.866025403784439,
1.,0.866025403784439,1.,0.866025403784439,1.,0.866025403784439,1.,0.866025403784439,
1.,0.866025403784439,1.,0.866025403784439,1.,0.866025403784439,1.,0.866025403784439,
1.,0.866025403784439,1.,0.866025403784439,1.,0.866025403784439,1.,0.866025403784439,
1.,0.866025403784439,1.,0.866025403784439,1.,0.866025403784439,1.,0.866025403784439,
1.,0.866025403784439,1.,0.866025403784439,1.,0.866025403784439,1.,0.866025403784439,
1.,0.866025403784439,1.,0.866025403784439,1.,0.866025403784439,1.,0.866025403784439,
1.,0.866025403784439,1.,0.866025403784439,1.,0.866025403784439,1.,0.866025403784439,
1.,0.866025403784439,1.,0.866025403784439,1.,0.866025403784439,1.,0.866025403784439,
1.,0.866025403784439,1.,0.866025403784439,1.,0.866025403784439,1.,0.866025403784439,
1.,0.866025403784439,1.,0.866025403784439,1.,0.866025403784439,1.,0.866025403784439,
1.,0.866025403784439,1.,0.866025403784439,1.,0.866025403784439,1.,0.866025403784439,
1.,0.866025403784439,1.,0.866025403784439,1.,0.866025403784439,1.,0.866025403784439,
1.,0.866025403784439,1.,0.866025403784439,1.,0.866025403784439,1.,0.866025403784439,
1.,0.866025403784439,1.,0.866025403784439,1.,0.866025403784439,1.,0.866025403784439,
1.,0.866025403784439,1.,0.866025403784439,1.,0.866025403784439,1.,0.866025403784439,
1.,0.866025403784439,1.,0.866025403784439,1.,0.866025403784439,1.,0.866025403784439,
1.,0.866025403784439,1.,0.866025403784439,1.,0.866025403784439,1.,0.866025403784439,
1.,0.866025403784439,1.,0.866025403784439,1.,0.866025403784439,1.,0.866025403784439,
1.,0.866025403784439,1.,0.866025403784439,1.,0.866025403784439,1.,0.866025403784439,
1.,0.866025403784439,1.,0.866025403784439,1.,0.866025403784439,1.,0.866025403784439,
1.,0.866025403784439,1.,0.866025403784439,1.,0.866025403784439,1.,0.866025403784439,
1.,0.866025403784439,1.,0.866025403784439,1.,0.866025403784439,1.,0.866025403784439,
1.,0.866025403784439,1.,0.866025403784439,1.,0.866025403784439,1.,0.866025403784439,
1.,0.866025403784439,1.,0.866025403784439,1.,0.866025403784439,1.,0.866025403784439,
1.,0.866025403784439,1.,0.866025403784439,1.,0.866025403784439,1.,0.866025403784439,
1.,0.866025403784439,1.,0.866025403784439,1.,0.866025403784439,1.,0.866025403784439,
1.,0.866025403784439,1.,0.866025403784439,1.,0.866025403784439,1.,0.866025403784439,
1.,0.866025403784439,1.,0.866025403784439,1.,0.866025403784439,1.,0.866025403784439,
1.,0.866025403784439,1.,0.866025403784439,1.,0.866025403784439,1.,0.866025403784439,
1.,0.866025403784439,1.,0.866025403784439,1.,0.866025403784439,1.,0.866025403784439,
1.,0.866025403784439,1.,0.866025403784439,1.,0.866025403784439,1.,0.866025403784439,
1.,0.866025403784439,1.,0.866025403784439,1.,0.866025403784439,1.,0.866025403784439,
1.,0.866025403784439,1.,0.866025403784439,1.,0.866025403784439,1.,0.866025403784439,
1.,0.866025403784439,1.,0.866025403784439,1.,0.866025403784439,1.,0.866025403784439,
1.,0.866025403784439,1.,0.866025403784439,1.,0.866025403784439,1.,0.866025403784439,
1.,0.866025403784439,1.,0.866025403784439,1.,0.866025403784439,1.,0.866025403784439,
1.,0.866025403784439,1.,0.866025403784439,1.,0.866025403784439,1.,0.866025403784439,
1.,0.866025403784439,1.,0.866025403784439,1.,0.866025403784439,1.,0.866025403784439,
1.,0.866025403784439,1.,0.866025403784439,1.,0.866025403784439,1.,0.866025403784439,
1.,0.866025403784439,1.,0.866025403784439,1.,0.866025403784439,1.,0.866025403784439,
1.,0.866025403784439,1.,0.866025403784439,1.,0.866025403784439,1.,0.866025403784439,
1.,0.866025403784439,1.,0.866025403784439,1.,0.866025403784439,1.,0.866025403784439,
1.,0.866025403784439,1.,0.866025403784439,1.,0.866025403784439,1.,0.866025403784439,
1.,0.866025403784439,1.,0.866025403784439,1.,0.866025403784439,1.,0.866025403784439,
1.,0.866025403784439,1.,0.866025403784439,1.,0.866025403784439,1.,0.866025403784439,
1.,0.866025403784439,1.,0.866025403784439,1.,0.866025403784439,1.,0.866025403784439,
1.,0.866025403784439,1.,0.866025403784439,1.,0.866025403784439,1.,0.866025403784439,
1.,0.866025403784439,1.,0.866025403784439,1.,0.866025403784439,1.,0.866025403784439,
1.,0.866025403784439,1.,0.866025403784439,1.,0.866025403784439,1.,0.866025403784439,
1.,0.866025403784439,1.,0.866025403784439,1.,0.866025403784439,1.,0.866025403784439,
1.,0.866025403784439,1.,0.866025403784439,1.,0.866025403784439,1.,0.866025403784439,
1.,0.866025403784439,1.,0.866025403784439,1.,0.866025403784439,1.,0.866025403784439,
1.,0.866025403784439,1.,0.866025403784439,1.,0.866025403784439,1.,0.866025403784439,
1.,0.866025403784439,1.,0.866025403784439,1.,0.866025403784439,1.,0.866025403784439,
1.,0.866025403784439,1.,0.866025403784439,1.,0.866025403784439,1.,0.866025403784439,
1.,0.866025403784439,1.,0.866025403784439,1.,0.866025403784439,1.,0.866025403784439,
1.,0.866025403784439,1.,0.866025403784439,1.,0.866025403784439,1.,0.866025403784439,
1.,0.866025403784439,1.,0.866025403784439,1.,0.866025403784439,1.,0.866025403784439,
1.,0.866025403784439,1.,0.866025403784439,1.,0.866025403784439,1.,0.866025403784439,
1.,0.866025403784439,1.,0.866025403784439,1.,0.866025403784439,1.,0.866025403784439,
1.,0.866025403784439,1.,0.866025403784439,1.,0.866025403784439,1.,0.866025403784439,
1.,0.866025403784439,1.,0.866025403784439,1.,0.866025403784439,1.,0.866025403784439,
1.,0.866025403784439,1.,0.866025403784439,1.,0.866025403784439,1.,0.866025403784439,
1.,0.866025403784439,1.,0.866025403784439,1.,0.866025403784439,1.,0.866025403784439,
1.,0.866025403784439,1.,0.866025403784439,1.,0.866025403784439,1.,0.866025403784439,
1.,0.866025403784439,1.,0.866025403784439,1.,0.866025403784439,1.,0.866025403784439,
1.,0.866025403784439,1.,0.866025403784439,1.,0.866025403784439,1.,0.866025403784439,
1.,0.866025403784439,1.,0.866025403784439,1.,0.866025403784439,1.,0.866025403784439,
1.,0.866025403784439,1.,0.866025403784439,1.,0.866025403784439,1.,0.866025403784439,
1.,0.866025403784439,1.,0.866025403784439,1.,0.866025403784439,1.,0.866025403784439,
1.),(0.641165742156689,0.555265820743996,0.641165742156689,0.555265820743996,
0.641165742156689,0.555265820743996,0.641165742156689,0.555265820743996,
0.641165742156689,0.555265820743996,0.641165742156689,0.555265820743996,
0.641165742156689,0.555265820743996,0.641165742156689,0.555265820743996,
0.641165742156689,0.555265820743996,0.641165742156689,0.555265820743996,
0.641165742156689,0.555265820743996,0.641165742156689,0.555265820743996,
0.641165742156689,0.555265820743996,0.641165742156689,0.555265820743996,
0.641165742156689,0.555265820743996,0.641165742156689,0.555265820743996,
0.641165742156689,0.555265820743996,0.641165742156689,0.555265820743996,
0.641165742156689,0.555265820743996,0.641165742156689,0.555265820743996,
0.641165742156689,0.555265820743996,0.641165742156689,0.555265820743996,
0.641165742156689,0.555265820743996,0.641165742156689,0.555265820743996,
0.641165742156689,0.555265820743996,0.641165742156689,0.555265820743996,
0.641165742156689,0.555265820743996,0.641165742156689,0.555265820743996,
0.641165742156689,0.555265820743996,0.641165742156689,0.555265820743996,
0.641165742156689,0.555265820743996,0.641165742156689,0.555265820743996,
0.641165742156689,0.555265820743996,0.641165742156689,0.555265820743996,
0.641165742156689,0.555265820743996,0.641165742156689,0.555265820743996,
0.641165742156689,0.555265820743996,0.641165742156689,0.555265820743996,
0.641165742156689,0.555265820743996,0.641165742156689,0.555265820743996,
0.641165742156689,0.555265820743996,0.641165742156689,0.555265820743996,
0.641165742156689,0.555265820743996,0.641165742156689,0.555265820743996,
0.641165742156689,0.555265820743996,0.641165742156689,0.555265820743996,
0.641165742156689,0.555265820743996,0.641165742156689,0.555265820743996,
0.641165742156689,0.555265820743996,0.641165742156689,0.555265820743996,
0.641165742156689,0.555265820743996,0.641165742156689,0.555265820743996,
0.641165742156689,0.555265820743996,0.641165742156689,0.555265820743996,
0.641165742156689,0.555265820743996,0.641165742156689,0.555265820743996,
0.641165742156689,0.555265820743996,0.641165742156689,0.555265820743996,
0.641165742156689,0.555265820743996,0.641165742156689,0.555265820743996,
0.641165742156689,0.555265820743996,0.641165742156689,0.555265820743996,
0.641165742156689,0.555265820743996,0.641165742156689,0.555265820743996,
0.641165742156689,0.555265820743996,0.641165742156689,0.555265820743996,
0.641165742156689,0.555265820743996,0.641165742156689,0.555265820743996,
0.641165742156689,0.555265820743996,0.641165742156689,0.555265820743996,
0.641165742156689,0.555265820743996,0.641165742156689,0.555265820743996,
0.641165742156689,0.555265820743996,0.641165742156689,0.555265820743996,
0.641165742156689,0.555265820743996,0.641165742156689,0.555265820743996,
0.641165742156689,0.555265820743996,0.641165742156689,0.555265820743996,
0.641165742156689,0.555265820743996,0.641165742156689,0.555265820743996,
0.641165742156689,0.555265820743996,0.641165742156689,0.555265820743996,
0.641165742156689,0.555265820743996,0.641165742156689,0.555265820743996,
0.641165742156689,0.555265820743996,0.641165742156689,0.555265820743996,
0.641165742156689,0.555265820743996,0.641165742156689,0.555265820743996,
0.641165742156689,0.555265820743996,0.641165742156689,0.555265820743996,
0.641165742156689,0.555265820743996,0.641165742156689,0.555265820743996,
0.641165742156689,0.555265820743996,0.641165742156689,0.555265820743996,
0.641165742156689,0.555265820743996,0.641165742156689,0.555265820743996,
0.641165742156689,0.555265820743996,0.641165742156689,0.555265820743996,
0.641165742156689,0.555265820743996,0.641165742156689,0.555265820743996,
0.641165742156689,0.555265820743996,0.641165742156689,0.555265820743996,
0.641165742156689,0.555265820743996,0.641165742156689,0.555265820743996,
0.641165742156689,0.555265820743996,0.641165742156689,0.555265820743996,
0.641165742156689,0.555265820743996,0.641165742156689,0.555265820743996,
0.641165742156689,0.555265820743996,0.641165742156689,0.555265820743996,
0.641165742156689,0.555265820743996,0.641165742156689,0.555265820743996,
0.641165742156689,0.555265820743996,0.641165742156689,0.555265820743996,
0.641165742156689,0.555265820743996,0.641165742156689,0.555265820743996,
0.641165742156689,0.555265820743996,0.641165742156689,0.555265820743996,
0.641165742156689,0.555265820743996,0.641165742156689,0.555265820743996,
0.641165742156689,0.555265820743996,0.641165742156689,0.555265820743996,
0.641165742156689,0.555265820743996,0.641165742156689,0.555265820743996,
0.641165742156689,0.555265820743996,0.641165742156689,0.555265820743996,
0.641165742156689,0.555265820743996,0.641165742156689,0.555265820743996,
0.641165742156689,0.555265820743996,0.641165742156689,0.555265820743996,
0.641165742156689,0.555265820743996,0.641165742156689,0.555265820743996,
0.641165742156689,0.555265820743996,0.641165742156689,0.555265820743996,
0.641165742156689,0.555265820743996,0.641165742156689,0.555265820743996,
0.641165742156689,0.555265820743996,0.641165742156689,0.555265820743996,
0.641165742156689,0.555265820743996,0.641165742156689,0.555265820743996,
0.641165742156689,0.555265820743996,0.641165742156689,0.555265820743996,
0.641165742156689,0.555265820743996,0.641165742156689,0.555265820743996,
0.641165742156689,0.555265820743996,0.641165742156689,0.555265820743996,
0.641165742156689,0.555265820743996,0.641165742156689,0.555265820743996,
0.641165742156689,0.555265820743996,0.641165742156689,0.555265820743996,
0.641165742156689,0.555265820743996,0.641165742156689,0.555265820743996,
0.641165742156689,0.555265820743996,0.641165742156689,0.555265820743996,
0.641165742156689,0.555265820743996,0.641165742156689,0.555265820743996,
0.641165742156689,0.555265820743996,0.641165742156689,0.555265820743996,
0.641165742156689,0.555265820743996,0.641165742156689,0.555265820743996,
0.641165742156689,0.555265820743996,0.641165742156689,0.555265820743996,
0.641165742156689,0.555265820743996,0.641165742156689,0.555265820743996,
0.641165742156689,0.555265820743996,0.641165742156689,0.555265820743996,
0.641165742156689,0.555265820743996,0.641165742156689,0.555265820743996,
0.641165742156689,0.555265820743996,0.641165742156689,0.555265820743996,
0.641165742156689,0.555265820743996,0.641165742156689,0.555265820743996,
0.641165742156689,0.555265820743996,0.641165742156689,0.555265820743996,
0.641165742156689,0.555265820743996,0.641165742156689,0.555265820743996,
0.641165742156689,0.555265820743996,0.641165742156689,0.555265820743996,
0.641165742156689,0.555265820743996,0.641165742156689,0.555265820743996,
0.641165742156689,0.555265820743996,0.641165742156689,0.555265820743996,
0.641165742156689,0.555265820743996,0.641165742156689,0.555265820743996,
0.641165742156689,0.555265820743996,0.641165742156689,0.555265820743996,
0.641165742156689,0.555265820743996,0.641165742156689,0.555265820743996,
0.641165742156689,0.555265820743996,0.641165742156689,0.555265820743996,
0.641165742156689,0.555265820743996,0.641165742156689,0.555265820743996,
0.641165742156689,0.555265820743996,0.641165742156689,0.555265820743996,
0.641165742156689,0.555265820743996,0.641165742156689,0.555265820743996,
0.641165742156689,0.555265820743996,0.641165742156689,0.555265820743996,
0.641165742156689,0.555265820743996,0.641165742156689,0.555265820743996,
0.641165742156689,0.555265820743996,0.641165742156689,0.555265820743996,
0.641165742156689,0.555265820743996,0.641165742156689,0.555265820743996,
0.641165742156689,0.555265820743996,0.641165742156689,0.555265820743996,
0.641165742156689,0.555265820743996,0.641165742156689,0.555265820743996,
0.641165742156689,0.555265820743996,0.641165742156689,0.555265820743996,
0.641165742156689,0.555265820743996,0.641165742156689,0.555265820743996,
0.641165742156689,0.555265820743996,0.641165742156689,0.555265820743996,
0.641165742156689,0.555265820743996,0.641165742156689,0.555265820743996,
0.641165742156689,0.555265820743996,0.641165742156689,0.555265820743996,
0.641165742156689,0.555265820743996,0.641165742156689,0.555265820743996,
0.641165742156689,0.555265820743996,0.641165742156689,0.555265820743996,
0.641165742156689,0.555265820743996,0.641165742156689,0.555265820743996,
0.641165742156689,0.555265820743996,0.641165742156689,0.555265820743996,
0.641165742156689,0.555265820743996,0.641165742156689,0.555265820743996,
0.641165742156689,0.555265820743996,0.641165742156689,0.555265820743996,
0.641165742156689,0.555265820743996,0.641165742156689,0.555265820743996,
0.641165742156689,0.555265820743996,0.641165742156689,0.555265820743996,
0.641165742156689,0.555265820743996,0.641165742156689,0.555265820743996,
0.641165742156689,0.555265820743996,0.641165742156689,0.555265820743996,
0.641165742156689,0.555265820743996,0.641165742156689,0.555265820743996,
0.641165742156689,0.555265820743996,0.641165742156689,0.555265820743996,
0.641165742156689,0.555265820743996,0.641165742156689,0.555265820743996,
0.641165742156689,0.555265820743996,0.641165742156689,0.555265820743996,
0.641165742156689,0.555265820743996,0.641165742156689,0.555265820743996,
0.641165742156689,0.555265820743996,0.641165742156689,0.555265820743996,
0.641165742156689,0.555265820743996,0.641165742156689,0.555265820743996,
0.641165742156689,0.555265820743996,0.641165742156689,0.555265820743996,
0.641165742156689,0.555265820743996,0.641165742156689,0.555265820743996,
0.641165742156689,0.555265820743996,0.641165742156689,0.555265820743996,
0.641165742156689,0.555265820743996,0.641165742156689,0.555265820743996,
0.641165742156689,0.555265820743996,0.641165742156689,0.555265820743996,
0.641165742156689,0.555265820743996,0.641165742156689,0.555265820743996,
0.641165742156689,0.555265820743996,0.641165742156689,0.555265820743996,
0.641165742156689,0.555265820743996,0.641165742156689,0.555265820743996,
0.641165742156689,0.555265820743996,0.641165742156689,0.555265820743996,
0.641165742156689,0.555265820743996,0.641165742156689,0.555265820743996,
0.641165742156689,0.555265820743996,0.641165742156689,0.555265820743996,
0.641165742156689,0.555265820743996,0.641165742156689,0.555265820743996,
0.641165742156689,0.555265820743996,0.641165742156689,0.555265820743996,
0.641165742156689,0.555265820743996,0.641165742156689,0.555265820743996,
0.641165742156689,0.555265820743996,0.641165742156689,0.555265820743996,
0.641165742156689,0.555265820743996,0.641165742156689,0.555265820743996,
0.641165742156689,0.555265820743996,0.641165742156689,0.555265820743996,
0.641165742156689,0.555265820743996,0.641165742156689,0.555265820743996,
0.641165742156689,0.555265820743996,0.641165742156689,0.555265820743996,
0.641165742156689,0.555265820743996,0.641165742156689,0.555265820743996,
0.641165742156689,0.555265820743996,0.641165742156689,0.555265820743996,
0.641165742156689,0.555265820743996,0.641165742156689,0.555265820743996,
0.641165742156689,0.555265820743996,0.641165742156689,0.555265820743996,
0.641165742156689,0.555265820743996,0.641165742156689,0.555265820743996,
0.641165742156689,0.555265820743996,0.641165742156689,0.555265820743996,
0.641165742156689,0.555265820743996,0.641165742156689,0.555265820743996,
0.641165742156689,0.555265820743996,0.641165742156689,0.555265820743996,
0.641165742156689,0.555265820743996,0.641165742156689,0.555265820743996,
0.641165742156689,0.555265820743996,0.641165742156689,0.555265820743996,
0.641165742156689,0.555265820743996,0.641165742156689,0.555265820743996,
0.641165742156689,0.555265820743996,0.641165742156689,0.555265820743996,
0.641165742156689,0.555265820743996,0.641165742156689,0.555265820743996,
0.641165742156689,0.555265820743996,0.641165742156689,0.555265820743996,
0.641165742156689,0.555265820743996,0.641165742156689,0.555265820743996,
0.641165742156689,0.555265820743996,0.641165742156689,0.555265820743996,
0.641165742156689,0.555265820743996,0.641165742156689,0.555265820743996,
0.641165742156689,0.555265820743996,0.641165742156689,0.555265820743996,
0.641165742156689,0.555265820743996,0.641165742156689,0.555265820743996,
0.641165742156689,0.555265820743996,0.641165742156689,0.555265820743996,
0.641165742156689,0.555265820743996,0.641165742156689,0.555265820743996,
0.641165742156689,0.555265820743996,0.641165742156689,0.555265820743996,
0.641165742156689,0.555265820743996,0.641165742156689,0.555265820743996,
0.641165742156689,0.555265820743996,0.641165742156689,0.555265820743996,
0.641165742156689,0.555265820743996,0.641165742156689,0.555265820743996,
0.641165742156689,0.555265820743996,0.641165742156689,0.555265820743996,
0.641165742156689,0.555265820743996,0.641165742156689,0.555265820743996,
0.641165742156689,0.555265820743996,0.641165742156689,0.555265820743996,
0.641165742156689,0.555265820743996,0.641165742156689,0.555265820743996,
0.641165742156689,0.555265820743996,0.641165742156689,0.555265820743996,
0.641165742156689,0.555265820743996,0.641165742156689,0.555265820743996,
0.641165742156689,0.555265820743996,0.641165742156689,0.555265820743996,
0.641165742156689,0.555265820743996,0.641165742156689,0.555265820743996,
0.641165742156689,0.555265820743996,0.641165742156689,0.555265820743996,
0.641165742156689,0.555265820743996,0.641165742156689,0.555265820743996,
0.641165742156689,0.555265820743996,0.641165742156689,0.555265820743996,
0.641165742156689,0.555265820743996,0.641165742156689,0.555265820743996,
0.641165742156689,0.555265820743996,0.641165742156689,0.555265820743996,
0.641165742156689,0.555265820743996,0.641165742156689,0.555265820743996,
0.641165742156689,0.555265820743996,0.641165742156689,0.555265820743996,
0.641165742156689,0.555265820743996,0.641165742156689,0.555265820743996,
0.641165742156689,0.555265820743996,0.641165742156689,0.555265820743996,
0.641165742156689,0.555265820743996,0.641165742156689,0.555265820743996,
0.641165742156689,0.555265820743996,0.641165742156689,0.555265820743996,
0.641165742156689,0.555265820743996,0.641165742156689,0.555265820743996,
0.641165742156689,0.555265820743996,0.641165742156689,0.555265820743996,
0.641165742156689,0.555265820743996,0.641165742156689,0.555265820743996,
0.641165742156689,0.555265820743996,0.641165742156689,0.555265820743996,
0.641165742156689,0.555265820743996,0.641165742156689,0.555265820743996,
0.641165742156689,0.555265820743996,0.641165742156689,0.555265820743996,
0.641165742156689,0.555265820743996,0.641165742156689,0.555265820743996,
0.641165742156689,0.555265820743996,0.641165742156689,0.555265820743996,
0.641165742156689,0.555265820743996,0.641165742156689,0.555265820743996,
0.641165742156689,0.555265820743996,0.641165742156689,0.555265820743996,
0.641165742156689,0.555265820743996,0.641165742156689,0.555265820743996,
0.641165742156689,0.555265820743996,0.641165742156689,0.555265820743996,
0.641165742156689,0.555265820743996,0.641165742156689,0.555265820743996,
0.641165742156689,0.555265820743996,0.641165742156689,0.555265820743996,
0.641165742156689,0.555265820743996,0.641165742156689,0.555265820743996,
0.641165742156689,0.555265820743996,0.641165742156689,0.555265820743996,
0.641165742156689,0.555265820743996,0.641165742156689,0.555265820743996,
0.641165742156689,0.555265820743996,0.641165742156689,0.555265820743996,
0.641165742156689,0.555265820743996,0.641165742156689,0.555265820743996,
0.641165742156689,0.555265820743996,0.641165742156689,0.555265820743996,
0.641165742156689,0.555265820743996,0.641165742156689,0.555265820743996,
0.641165742156689,0.555265820743996,0.641165742156689,0.555265820743996,
0.641165742156689,0.555265820743996,0.641165742156689,0.555265820743996,
0.641165742156689,0.555265820743996,0.641165742156689,0.555265820743996,
0.641165742156689,0.555265820743996,0.641165742156689,0.555265820743996,
0.641165742156689,0.555265820743996,0.641165742156689,0.555265820743996,
0.641165742156689,0.555265820743996,0.641165742156689,0.555265820743996,
0.641165742156689,0.555265820743996,0.641165742156689,0.555265820743996,
0.641165742156689,0.555265820743996,0.641165742156689,0.555265820743996,
0.641165742156689,0.555265820743996,0.641165742156689,0.555265820743996,
0.641165742156689,0.555265820743996,0.641165742156689,0.555265820743996,
0.641165742156689,0.555265820743996,0.641165742156689,0.555265820743996,
0.641165742156689,0.555265820743996,0.641165742156689,0.555265820743996,
0.641165742156689,0.555265820743996,0.641165742156689,0.555265820743996,
0.641165742156689,0.555265820743996,0.641165742156689,0.555265820743996,
0.641165742156689,0.555265820743996,0.641165742156689,0.555265820743996,
0.641165742156689,0.555265820743996,0.641165742156689,0.555265820743996,
0.641165742156689,0.555265820743996,0.641165742156689,0.555265820743996,
0.641165742156689,0.555265820743996,0.641165742156689,0.555265820743996,
0.641165742156689,0.555265820743996,0.641165742156689,0.555265820743996,
0.641165742156689,0.555265820743996,0.641165742156689,0.555265820743996,
0.641165742156689,0.555265820743996,0.641165742156689,0.555265820743996,
0.641165742156689,0.555265820743996,0.641165742156689,0.555265820743996,
0.641165742156689,0.555265820743996,0.641165742156689,0.555265820743996,
0.641165742156689,0.555265820743996,0.641165742156689,0.555265820743996,
0.641165742156689,0.555265820743996,0.641165742156689,0.555265820743996,
0.641165742156689,0.555265820743996,0.641165742156689,0.555265820743996,
0.641165742156689,0.555265820743996,0.641165742156689,0.555265820743996,
0.641165742156689,0.555265820743996,0.641165742156689,0.555265820743996,
0.641165742156689,0.555265820743996,0.641165742156689,0.555265820743996,
0.641165742156689,0.555265820743996,0.641165742156689,0.555265820743996,
0.641165742156689,0.555265820743996,0.641165742156689,0.555265820743996,
0.641165742156689,0.555265820743996,0.641165742156689,0.555265820743996,
0.641165742156689,0.555265820743996,0.641165742156689,0.555265820743996,
0.641165742156689),(0.641165742156689,0.555265820743996,0.641165742156689,
0.555265820743996,0.641165742156689,0.555265820743996,0.641165742156689,
0.555265820743996,0.641165742156689,0.555265820743996,0.641165742156689,
0.555265820743996,0.641165742156689,0.555265820743996,0.641165742156689,
0.555265820743996,0.641165742156689,0.555265820743996,0.641165742156689,
0.555265820743996,0.641165742156689,0.555265820743996,0.641165742156689,
0.555265820743996,0.641165742156689,0.555265820743996,0.641165742156689,
0.555265820743996,0.641165742156689,0.555265820743996,0.641165742156689,
0.555265820743996,0.641165742156689,0.555265820743996,0.641165742156689,
0.555265820743996,0.641165742156689,0.555265820743996,0.641165742156689,
0.555265820743996,0.641165742156689,0.555265820743996,0.641165742156689,
0.555265820743996,0.641165742156689,0.555265820743996,0.641165742156689,
0.555265820743996,0.641165742156689,0.555265820743996,0.641165742156689,
0.555265820743996,0.641165742156689,0.555265820743996,0.641165742156689,
0.555265820743996,0.641165742156689,0.555265820743996,0.641165742156689,
0.555265820743996,0.641165742156689,0.555265820743996,0.641165742156689,
0.555265820743996,0.641165742156689,0.555265820743996,0.641165742156689,
0.555265820743996,0.641165742156689,0.555265820743996,0.641165742156689,
0.555265820743996,0.641165742156689,0.555265820743996,0.641165742156689,
0.555265820743996,0.641165742156689,0.555265820743996,0.641165742156689,
0.555265820743996,0.641165742156689,0.555265820743996,0.641165742156689,
0.555265820743996,0.641165742156689,0.555265820743996,0.641165742156689,
0.555265820743996,0.641165742156689,0.555265820743996,0.641165742156689,
0.555265820743996,0.641165742156689,0.555265820743996,0.641165742156689,
0.555265820743996,0.641165742156689,0.555265820743996,0.641165742156689,
0.555265820743996,0.641165742156689,0.555265820743996,0.641165742156689,
0.555265820743996,0.641165742156689,0.555265820743996,0.641165742156689,
0.555265820743996,0.641165742156689,0.555265820743996,0.641165742156689,
0.555265820743996,0.641165742156689,0.555265820743996,0.641165742156689,
0.555265820743996,0.641165742156689,0.555265820743996,0.641165742156689,
0.555265820743996,0.641165742156689,0.555265820743996,0.641165742156689,
0.555265820743996,0.641165742156689,0.555265820743996,0.641165742156689,
0.555265820743996,0.641165742156689,0.555265820743996,0.641165742156689,
0.555265820743996,0.641165742156689,0.555265820743996,0.641165742156689,
0.555265820743996,0.641165742156689,0.555265820743996,0.641165742156689,
0.555265820743996,0.641165742156689,0.555265820743996,0.641165742156689,
0.555265820743996,0.641165742156689,0.555265820743996,0.641165742156689,
0.555265820743996,0.641165742156689,0.555265820743996,0.641165742156689,
0.555265820743996,0.641165742156689,0.555265820743996,0.641165742156689,
0.555265820743996,0.641165742156689,0.555265820743996,0.641165742156689,
0.555265820743996,0.641165742156689,0.555265820743996,0.641165742156689,
0.555265820743996,0.641165742156689,0.555265820743996,0.641165742156689,
0.555265820743996,0.641165742156689,0.555265820743996,0.641165742156689,
0.555265820743996,0.641165742156689,0.555265820743996,0.641165742156689,
0.555265820743996,0.641165742156689,0.555265820743996,0.641165742156689,
0.555265820743996,0.641165742156689,0.555265820743996,0.641165742156689,
0.555265820743996,0.641165742156689,0.555265820743996,0.641165742156689,
0.555265820743996,0.641165742156689,0.555265820743996,0.641165742156689,
0.555265820743996,0.641165742156689,0.555265820743996,0.641165742156689,
0.555265820743996,0.641165742156689,0.555265820743996,0.641165742156689,
0.555265820743996,0.641165742156689,0.555265820743996,0.641165742156689,
0.555265820743996,0.641165742156689,0.555265820743996,0.641165742156689,
0.555265820743996,0.641165742156689,0.555265820743996,0.641165742156689,
0.555265820743996,0.641165742156689,0.555265820743996,0.641165742156689,
0.555265820743996,0.641165742156689,0.555265820743996,0.641165742156689,
0.555265820743996,0.641165742156689,0.555265820743996,0.641165742156689,
0.555265820743996,0.641165742156689,0.555265820743996,0.641165742156689,
0.555265820743996,0.641165742156689,0.555265820743996,0.641165742156689,
0.555265820743996,0.641165742156689,0.555265820743996,0.641165742156689,
0.555265820743996,0.641165742156689,0.555265820743996,0.641165742156689,
0.555265820743996,0.641165742156689,0.555265820743996,0.641165742156689,
0.555265820743996,0.641165742156689,0.555265820743996,0.641165742156689,
0.555265820743996,0.641165742156689,0.555265820743996,0.641165742156689,
0.555265820743996,0.641165742156689,0.555265820743996,0.641165742156689,
0.555265820743996,0.641165742156689,0.555265820743996,0.641165742156689,
0.555265820743996,0.641165742156689,0.555265820743996,0.641165742156689,
0.555265820743996,0.641165742156689,0.555265820743996,0.641165742156689,
0.555265820743996,0.641165742156689,0.555265820743996,0.641165742156689,
0.555265820743996,0.641165742156689,0.555265820743996,0.641165742156689,
0.555265820743996,0.641165742156689,0.555265820743996,0.641165742156689,
0.555265820743996,0.641165742156689,0.555265820743996,0.641165742156689,
0.555265820743996,0.641165742156689,0.555265820743996,0.641165742156689,
0.555265820743996,0.641165742156689,0.555265820743996,0.641165742156689,
0.555265820743996,0.641165742156689,0.555265820743996,0.641165742156689,
0.555265820743996,0.641165742156689,0.555265820743996,0.641165742156689,
0.555265820743996,0.641165742156689,0.555265820743996,0.641165742156689,
0.555265820743996,0.641165742156689,0.555265820743996,0.641165742156689,
0.555265820743996,0.641165742156689,0.555265820743996,0.641165742156689,
0.555265820743996,0.641165742156689,0.555265820743996,0.641165742156689,
0.555265820743996,0.641165742156689,0.555265820743996,0.641165742156689,
0.555265820743996,0.641165742156689,0.555265820743996,0.641165742156689,
0.555265820743996,0.641165742156689,0.555265820743996,0.641165742156689,
0.555265820743996,0.641165742156689,0.555265820743996,0.641165742156689,
0.555265820743996,0.641165742156689,0.555265820743996,0.641165742156689,
0.555265820743996,0.641165742156689,0.555265820743996,0.641165742156689,
0.555265820743996,0.641165742156689,0.555265820743996,0.641165742156689,
0.555265820743996,0.641165742156689,0.555265820743996,0.641165742156689,
0.555265820743996,0.641165742156689,0.555265820743996,0.641165742156689,
0.555265820743996,0.641165742156689,0.555265820743996,0.641165742156689,
0.555265820743996,0.641165742156689,0.555265820743996,0.641165742156689,
0.555265820743996,0.641165742156689,0.555265820743996,0.641165742156689,
0.555265820743996,0.641165742156689,0.555265820743996,0.641165742156689,
0.555265820743996,0.641165742156689,0.555265820743996,0.641165742156689,
0.555265820743996,0.641165742156689,0.555265820743996,0.641165742156689,
0.555265820743996,0.641165742156689,0.555265820743996,0.641165742156689,
0.555265820743996,0.641165742156689,0.555265820743996,0.641165742156689,
0.555265820743996,0.641165742156689,0.555265820743996,0.641165742156689,
0.555265820743996,0.641165742156689,0.555265820743996,0.641165742156689,
0.555265820743996,0.641165742156689,0.555265820743996,0.641165742156689,
0.555265820743996,0.641165742156689,0.555265820743996,0.641165742156689,
0.555265820743996,0.641165742156689,0.555265820743996,0.641165742156689,
0.555265820743996,0.641165742156689,0.555265820743996,0.641165742156689,
0.555265820743996,0.641165742156689,0.555265820743996,0.641165742156689,
0.555265820743996,0.641165742156689,0.555265820743996,0.641165742156689,
0.555265820743996,0.641165742156689,0.555265820743996,0.641165742156689,
0.555265820743996,0.641165742156689,0.555265820743996,0.641165742156689,
0.555265820743996,0.641165742156689,0.555265820743996,0.641165742156689,
0.555265820743996,0.641165742156689,0.555265820743996,0.641165742156689,
0.555265820743996,0.641165742156689,0.555265820743996,0.641165742156689,
0.555265820743996,0.641165742156689,0.555265820743996,0.641165742156689,
0.555265820743996,0.641165742156689,0.555265820743996,0.641165742156689,
0.555265820743996,0.641165742156689,0.555265820743996,0.641165742156689,
0.555265820743996,0.641165742156689,0.555265820743996,0.641165742156689,
0.555265820743996,0.641165742156689,0.555265820743996,0.641165742156689,
0.555265820743996,0.641165742156689,0.555265820743996,0.641165742156689,
0.555265820743996,0.641165742156689,0.555265820743996,0.641165742156689,
0.555265820743996,0.641165742156689,0.555265820743996,0.641165742156689,
0.555265820743996,0.641165742156689,0.555265820743996,0.641165742156689,
0.555265820743996,0.641165742156689,0.555265820743996,0.641165742156689,
0.555265820743996,0.641165742156689,0.555265820743996,0.641165742156689,
0.555265820743996,0.641165742156689,0.555265820743996,0.641165742156689,
0.555265820743996,0.641165742156689,0.555265820743996,0.641165742156689,
0.555265820743996,0.641165742156689,0.555265820743996,0.641165742156689,
0.555265820743996,0.641165742156689,0.555265820743996,0.641165742156689,
0.555265820743996,0.641165742156689,0.555265820743996,0.641165742156689,
0.555265820743996,0.641165742156689,0.555265820743996,0.641165742156689,
0.555265820743996,0.641165742156689,0.555265820743996,0.641165742156689,
0.555265820743996,0.641165742156689,0.555265820743996,0.641165742156689,
0.555265820743996,0.641165742156689,0.555265820743996,0.641165742156689,
0.555265820743996,0.641165742156689,0.555265820743996,0.641165742156689,
0.555265820743996,0.641165742156689,0.555265820743996,0.641165742156689,
0.555265820743996,0.641165742156689,0.555265820743996,0.641165742156689,
0.555265820743996,0.641165742156689,0.555265820743996,0.641165742156689,
0.555265820743996,0.641165742156689,0.555265820743996,0.641165742156689,
0.555265820743996,0.641165742156689,0.555265820743996,0.641165742156689,
0.555265820743996,0.641165742156689,0.555265820743996,0.641165742156689,
0.555265820743996,0.641165742156689,0.555265820743996,0.641165742156689,
0.555265820743996,0.641165742156689,0.555265820743996,0.641165742156689,
0.555265820743996,0.641165742156689,0.555265820743996,0.641165742156689,
0.555265820743996,0.641165742156689,0.555265820743996,0.641165742156689,
0.555265820743996,0.641165742156689,0.555265820743996,0.641165742156689,
0.555265820743996,0.641165742156689,0.555265820743996,0.641165742156689,
0.555265820743996,0.641165742156689,0.555265820743996,0.641165742156689,
0.555265820743996,0.641165742156689,0.555265820743996,0.641165742156689,
0.555265820743996,0.641165742156689,0.555265820743996,0.641165742156689,
0.555265820743996,0.641165742156689,0.555265820743996,0.641165742156689,
0.555265820743996,0.641165742156689,0.555265820743996,0.641165742156689,
0.555265820743996,0.641165742156689,0.555265820743996,0.641165742156689,
0.555265820743996,0.641165742156689,0.555265820743996,0.641165742156689,
0.555265820743996,0.641165742156689,0.555265820743996,0.641165742156689,
0.555265820743996,0.641165742156689,0.555265820743996,0.641165742156689,
0.555265820743996,0.641165742156689,0.555265820743996,0.641165742156689,
0.555265820743996,0.641165742156689,0.555265820743996,0.641165742156689,
0.555265820743996,0.641165742156689,0.555265820743996,0.641165742156689,
0.555265820743996,0.641165742156689,0.555265820743996,0.641165742156689,
0.555265820743996,0.641165742156689,0.555265820743996,0.641165742156689,
0.555265820743996,0.641165742156689,0.555265820743996,0.641165742156689,
0.555265820743996,0.641165742156689,0.555265820743996,0.641165742156689,
0.555265820743996,0.641165742156689,0.555265820743996,0.641165742156689,
0.555265820743996,0.641165742156689,0.555265820743996,0.641165742156689,
0.555265820743996,0.641165742156689,0.555265820743996,0.641165742156689,
0.555265820743996,0.641165742156689,0.555265820743996,0.641165742156689,
0.555265820743996,0.641165742156689,0.555265820743996,0.641165742156689,
0.555265820743996,0.641165742156689,0.555265820743996,0.641165742156689,
0.555265820743996,0.641165742156689,0.555265820743996,0.641165742156689,
0.555265820743996,0.641165742156689,0.555265820743996,0.641165742156689,
0.555265820743996,0.641165742156689,0.555265820743996,0.641165742156689,
0.555265820743996,0.641165742156689,0.555265820743996,0.641165742156689,
0.555265820743996,0.641165742156689,0.555265820743996,0.641165742156689,
0.555265820743996,0.641165742156689,0.555265820743996,0.641165742156689,
0.555265820743996,0.641165742156689,0.555265820743996,0.641165742156689,
0.555265820743996,0.641165742156689,0.555265820743996,0.641165742156689,
0.555265820743996,0.641165742156689,0.555265820743996,0.641165742156689,
0.555265820743996,0.641165742156689,0.555265820743996,0.641165742156689,
0.555265820743996,0.641165742156689,0.555265820743996,0.641165742156689,
0.555265820743996,0.641165742156689,0.555265820743996,0.641165742156689,
0.555265820743996,0.641165742156689,0.555265820743996,0.641165742156689,
0.555265820743996,0.641165742156689,0.555265820743996,0.641165742156689,
0.555265820743996,0.641165742156689,0.555265820743996,0.641165742156689,
0.555265820743996,0.641165742156689,0.555265820743996,0.641165742156689,
0.555265820743996,0.641165742156689,0.555265820743996,0.641165742156689,
0.555265820743996,0.641165742156689,0.555265820743996,0.641165742156689,
0.555265820743996,0.641165742156689,0.555265820743996,0.641165742156689,
0.555265820743996,0.641165742156689,0.555265820743996,0.641165742156689,
0.555265820743996,0.641165742156689,0.555265820743996,0.641165742156689,
0.555265820743996,0.641165742156689,0.555265820743996,0.641165742156689,
0.555265820743996,0.641165742156689,0.555265820743996,0.641165742156689,
0.555265820743996,0.641165742156689,0.555265820743996,0.641165742156689,
0.555265820743996,0.641165742156689,0.555265820743996,0.641165742156689,
0.555265820743996,0.641165742156689,0.555265820743996,0.641165742156689,
0.555265820743996,0.641165742156689,0.555265820743996,0.641165742156689,
0.555265820743996,0.641165742156689,0.555265820743996,0.641165742156689,
0.555265820743996,0.641165742156689,0.555265820743996,0.641165742156689,
0.555265820743996,0.641165742156689,0.555265820743996,0.641165742156689,
0.555265820743996,0.641165742156689,0.555265820743996,0.641165742156689,
0.555265820743996,0.641165742156689,0.555265820743996,0.641165742156689,
0.555265820743996,0.641165742156689,0.555265820743996,0.641165742156689,
0.555265820743996,0.641165742156689,0.555265820743996,0.641165742156689,
0.555265820743996,0.641165742156689,0.555265820743996,0.641165742156689,
0.555265820743996,0.641165742156689,0.555265820743996,0.641165742156689,
0.555265820743996,0.641165742156689,0.555265820743996,0.641165742156689,
0.555265820743996,0.641165742156689,0.555265820743996,0.641165742156689,
0.555265820743996,0.641165742156689,0.555265820743996,0.641165742156689,
0.555265820743996,0.641165742156689,0.555265820743996,0.641165742156689,
0.555265820743996,0.641165742156689,0.555265820743996,0.641165742156689,
0.555265820743996,0.641165742156689,0.555265820743996,0.641165742156689,
0.555265820743996,0.641165742156689,0.555265820743996,0.641165742156689,
0.555265820743996,0.641165742156689,0.555265820743996,0.641165742156689,
0.555265820743996,0.641165742156689,0.555265820743996,0.641165742156689,
0.555265820743996,0.641165742156689,0.555265820743996,0.641165742156689,
0.555265820743996,0.641165742156689,0.555265820743996,0.641165742156689,
0.555265820743996,0.641165742156689,0.555265820743996,0.641165742156689,
0.555265820743996,0.641165742156689,0.555265820743996,0.641165742156689,
0.555265820743996,0.641165742156689,0.555265820743996,0.641165742156689,
0.555265820743996,0.641165742156689,0.555265820743996,0.641165742156689,
0.555265820743996,0.641165742156689,0.555265820743996,0.641165742156689,
0.555265820743996,0.641165742156689,0.555265820743996,0.641165742156689,
0.555265820743996,0.641165742156689,0.555265820743996,0.641165742156689,
0.555265820743996,0.641165742156689,0.555265820743996,0.641165742156689,
0.555265820743996,0.641165742156689,0.555265820743996,0.641165742156689,
0.555265820743996,0.641165742156689,0.555265820743996,0.641165742156689,
0.555265820743996,0.641165742156689,0.555265820743996,0.641165742156689,
0.555265820743996,0.641165742156689,0.555265820743996,0.641165742156689,
0.555265820743996,0.641165742156689,0.555265820743996,0.641165742156689,
0.555265820743996,0.641165742156689,0.555265820743996,0.641165742156689,
0.555265820743996,0.641165742156689,0.555265820743996,0.641165742156689,
0.555265820743996,0.641165742156689,0.555265820743996,0.641165742156689,
0.555265820743996,0.641165742156689,0.555265820743996,0.641165742156689,
0.555265820743996,0.641165742156689,0.555265820743996,0.641165742156689,
0.555265820743996,0.641165742156689,0.555265820743996,0.641165742156689,
0.555265820743996,0.641165742156689,0.555265820743996,0.641165742156689,
0.555265820743996,0.641165742156689,0.555265820743996,0.641165742156689,
0.555265820743996,0.641165742156689,0.555265820743996,0.641165742156689,
0.555265820743996,0.641165742156689,0.555265820743996,0.641165742156689,
0.555265820743996,0.641165742156689,0.555265820743996,0.641165742156689,
0.555265820743996,0.641165742156689,0.555265820743996,0.641165742156689,
0.555265820743996,0.641165742156689,0.555265820743996,0.641165742156689,
0.555265820743996,0.641165742156689,0.555265820743996,0.641165742156689,
0.555265820743996,0.641165742156689,0.555265820743996,0.641165742156689,
0.555265820743996,0.641165742156689,0.555265820743996,0.641165742156689,
0.555265820743996,0.641165742156689,0.555265820743996,0.641165742156689,
0.555265820743996,0.641165742156689,0.555265820743996,0.641165742156689,
0.555265820743996,0.641165742156689,0.555265820743996,0.641165742156689,
0.555265820743996,0.641165742156689),(1.,0.866025403784439,1.,0.866025403784439,
1.,0.866025403784439,1.,0.866025403784439,1.,0.866025403784439,1.,0.866025403784439,
1.,0.866025403784439,1.,0.866025403784439,1.,0.866025403784439,1.,0.866025403784439,
1.,0.866025403784439,1.,0.866025403784439,1.,0.866025403784439,1.,0.866025403784439,
1.,0.866025403784439,1.,0.866025403784439,1.,0.866025403784439,1.,0.866025403784439,
1.,0.866025403784439,1.,0.866025403784439,1.,0.866025403784439,1.,0.866025403784439,
1.,0.866025403784439,1.,0.866025403784439,1.,0.866025403784439,1.,0.866025403784439,
1.,0.866025403784439,1.,0.866025403784439,1.,0.866025403784439,1.,0.866025403784439,
1.,0.866025403784439,1.,0.866025403784439,1.,0.866025403784439,1.,0.866025403784439,
1.,0.866025403784439,1.,0.866025403784439,1.,0.866025403784439,1.,0.866025403784439,
1.,0.866025403784439,1.,0.866025403784439,1.,0.866025403784439,1.,0.866025403784439,
1.,0.866025403784439,1.,0.866025403784439,1.,0.866025403784439,1.,0.866025403784439,
1.,0.866025403784439,1.,0.866025403784439,1.,0.866025403784439,1.,0.866025403784439,
1.,0.866025403784439,1.,0.866025403784439,1.,0.866025403784439,1.,0.866025403784439,
1.,0.866025403784439,1.,0.866025403784439,1.,0.866025403784439,1.,0.866025403784439,
1.,0.866025403784439,1.,0.866025403784439,1.,0.866025403784439,1.,0.866025403784439,
1.,0.866025403784439,1.,0.866025403784439,1.,0.866025403784439,1.,0.866025403784439,
1.,0.866025403784439,1.,0.866025403784439,1.,0.866025403784439,1.,0.866025403784439,
1.,0.866025403784439,1.,0.866025403784439,1.,0.866025403784439,1.,0.866025403784439,
1.,0.866025403784439,1.,0.866025403784439,1.,0.866025403784439,1.,0.866025403784439,
1.,0.866025403784439,1.,0.866025403784439,1.,0.866025403784439,1.,0.866025403784439,
1.,0.866025403784439,1.,0.866025403784439,1.,0.866025403784439,1.,0.866025403784439,
1.,0.866025403784439,1.,0.866025403784439,1.,0.866025403784439,1.,0.866025403784439,
1.,0.866025403784439,1.,0.866025403784439,1.,0.866025403784439,1.,0.866025403784439,
1.,0.866025403784439,1.,0.866025403784439,1.,0.866025403784439,1.,0.866025403784439,
1.,0.866025403784439,1.,0.866025403784439,1.,0.866025403784439,1.,0.866025403784439,
1.,0.866025403784439,1.,0.866025403784439,1.,0.866025403784439,1.,0.866025403784439,
1.,0.866025403784439,1.,0.866025403784439,1.,0.866025403784439,1.,0.866025403784439,
1.,0.866025403784439,1.,0.866025403784439,1.,0.866025403784439,1.,0.866025403784439,
1.,0.866025403784439,1.,0.866025403784439,1.,0.866025403784439,1.,0.866025403784439,
1.,0.866025403784439,1.,0.866025403784439,1.,0.866025403784439,1.,0.866025403784439,
1.,0.866025403784439,1.,0.866025403784439,1.,0.866025403784439,1.,0.866025403784439,
1.,0.866025403784439,1.,0.866025403784439,1.,0.866025403784439,1.,0.866025403784439,
1.,0.866025403784439,1.,0.866025403784439,1.,0.866025403784439,1.,0.866025403784439,
1.,0.866025403784439,1.,0.866025403784439,1.,0.866025403784439,1.,0.866025403784439,
1.,0.866025403784439,1.,0.866025403784439,1.,0.866025403784439,1.,0.866025403784439,
1.,0.866025403784439,1.,0.866025403784439,1.,0.866025403784439,1.,0.866025403784439,
1.,0.866025403784439,1.,0.866025403784439,1.,0.866025403784439,1.,0.866025403784439,
1.,0.866025403784439,1.,0.866025403784439,1.,0.866025403784439,1.,0.866025403784439,
1.,0.866025403784439,1.,0.866025403784439,1.,0.866025403784439,1.,0.866025403784439,
1.,0.866025403784439,1.,0.866025403784439,1.,0.866025403784439,1.,0.866025403784439,
1.,0.866025403784439,1.,0.866025403784439,1.,0.866025403784439,1.,0.866025403784439,
1.,0.866025403784439,1.,0.866025403784439,1.,0.866025403784439,1.,0.866025403784439,
1.,0.866025403784439,1.,0.866025403784439,1.,0.866025403784439,1.,0.866025403784439,
1.,0.866025403784439,1.,0.866025403784439,1.,0.866025403784439,1.,0.866025403784439,
1.,0.866025403784439,1.,0.866025403784439,1.,0.866025403784439,1.,0.866025403784439,
1.,0.866025403784439,1.,0.866025403784439,1.,0.866025403784439,1.,0.866025403784439,
1.,0.866025403784439,1.,0.866025403784439,1.,0.866025403784439,1.,0.866025403784439,
1.,0.866025403784439,1.,0.866025403784439,1.,0.866025403784439,1.,0.866025403784439,
1.,0.866025403784439,1.,0.866025403784439,1.,0.866025403784439,1.,0.866025403784439,
1.,0.866025403784439,1.,0.866025403784439,1.,0.866025403784439,1.,0.866025403784439,
1.,0.866025403784439,1.,0.866025403784439,1.,0.866025403784439,1.,0.866025403784439,
1.,0.866025403784439,1.,0.866025403784439,1.,0.866025403784439,1.,0.866025403784439,
1.,0.866025403784439,1.,0.866025403784439,1.,0.866025403784439,1.,0.866025403784439,
1.,0.866025403784439,1.,0.866025403784439,1.,0.866025403784439,1.,0.866025403784439,
1.,0.866025403784439,1.,0.866025403784439,1.,0.866025403784439,1.,0.866025403784439,
1.,0.866025403784439,1.,0.866025403784439,1.,0.866025403784439,1.,0.866025403784439,
1.,0.866025403784439,1.,0.866025403784439,1.,0.866025403784439,1.,0.866025403784439,
1.,0.866025403784439,1.,0.866025403784439,1.,0.866025403784439,1.,0.866025403784439,
1.,0.866025403784439,1.,0.866025403784439,1.,0.866025403784439,1.,0.866025403784439,
1.,0.866025403784439,1.,0.866025403784439,1.,0.866025403784439,1.,0.866025403784439,
1.,0.866025403784439,1.,0.866025403784439,1.,0.866025403784439,1.,0.866025403784439,
1.,0.866025403784439,1.,0.866025403784439,1.,0.866025403784439,1.,0.866025403784439,
1.,0.866025403784439,1.,0.866025403784439,1.,0.866025403784439,1.,0.866025403784439,
1.,0.866025403784439,1.,0.866025403784439,1.,0.866025403784439,1.,0.866025403784439,
1.,0.866025403784439,1.,0.866025403784439,1.,0.866025403784439,1.,0.866025403784439,
1.,0.866025403784439,1.,0.866025403784439,1.,0.866025403784439,1.,0.866025403784439,
1.,0.866025403784439,1.,0.866025403784439,1.,0.866025403784439,1.,0.866025403784439,
1.,0.866025403784439,1.,0.866025403784439,1.,0.866025403784439,1.,0.866025403784439,
1.,0.866025403784439,1.,0.866025403784439,1.,0.866025403784439,1.,0.866025403784439,
1.,0.866025403784439,1.,0.866025403784439,1.,0.866025403784439,1.,0.866025403784439,
1.,0.866025403784439,1.,0.866025403784439,1.,0.866025403784439,1.,0.866025403784439,
1.,0.866025403784439,1.,0.866025403784439,1.,0.866025403784439,1.,0.866025403784439,
1.,0.866025403784439,1.,0.866025403784439,1.,0.866025403784439,1.,0.866025403784439,
1.,0.866025403784439,1.,0.866025403784439,1.,0.866025403784439,1.,0.866025403784439,
1.,0.866025403784439,1.,0.866025403784439,1.,0.866025403784439,1.,0.866025403784439,
1.,0.866025403784439,1.,0.866025403784439,1.,0.866025403784439,1.,0.866025403784439,
1.,0.866025403784439,1.,0.866025403784439,1.,0.866025403784439,1.,0.866025403784439,
1.,0.866025403784439,1.,0.866025403784439,1.,0.866025403784439,1.,0.866025403784439,
1.,0.866025403784439,1.,0.866025403784439,1.,0.866025403784439,1.,0.866025403784439,
1.,0.866025403784439,1.,0.866025403784439,1.,0.866025403784439,1.,0.866025403784439,
1.,0.866025403784439,1.,0.866025403784439,1.,0.866025403784439,1.,0.866025403784439,
1.,0.866025403784439,1.,0.866025403784439,1.,0.866025403784439,1.,0.866025403784439,
1.,0.866025403784439,1.,0.866025403784439,1.,0.866025403784439,1.,0.866025403784439,
1.,0.866025403784439,1.,0.866025403784439,1.,0.866025403784439,1.,0.866025403784439,
1.,0.866025403784439,1.,0.866025403784439,1.,0.866025403784439,1.,0.866025403784439,
1.,0.866025403784439,1.,0.866025403784439,1.,0.866025403784439,1.,0.866025403784439,
1.,0.866025403784439,1.,0.866025403784439,1.,0.866025403784439,1.,0.866025403784439,
1.,0.866025403784439,1.,0.866025403784439,1.,0.866025403784439,1.,0.866025403784439,
1.,0.866025403784439,1.,0.866025403784439,1.,0.866025403784439,1.,0.866025403784439,
1.,0.866025403784439,1.,0.866025403784439,1.,0.866025403784439,1.,0.866025403784439,
1.,0.866025403784439,1.,0.866025403784439,1.,0.866025403784439,1.,0.866025403784439,
1.,0.866025403784439,1.,0.866025403784439,1.,0.866025403784439,1.,0.866025403784439,
1.,0.866025403784439,1.,0.866025403784439,1.,0.866025403784439,1.,0.866025403784439,
1.,0.866025403784439,1.,0.866025403784439,1.,0.866025403784439,1.,0.866025403784439,
1.,0.866025403784439,1.,0.866025403784439,1.,0.866025403784439,1.,0.866025403784439,
1.,0.866025403784439,1.,0.866025403784439,1.,0.866025403784439,1.,0.866025403784439,
1.,0.866025403784439,1.,0.866025403784439,1.,0.866025403784439,1.,0.866025403784439,
1.,0.866025403784439,1.,0.866025403784439,1.,0.866025403784439,1.,0.866025403784439,
1.,0.866025403784439,1.,0.866025403784439,1.,0.866025403784439,1.,0.866025403784439,
1.,0.866025403784439,1.,0.866025403784439,1.,0.866025403784439,1.,0.866025403784439,
1.,0.866025403784439,1.,0.866025403784439,1.,0.866025403784439,1.,0.866025403784439,
1.,0.866025403784439,1.,0.866025403784439,1.,0.866025403784439,1.,0.866025403784439,
1.,0.866025403784439,1.,0.866025403784439,1.,0.866025403784439,1.,0.866025403784439,
1.,0.866025403784439,1.,0.866025403784439,1.,0.866025403784439,1.,0.866025403784439,
1.,0.866025403784439,1.,0.866025403784439,1.,0.866025403784439,1.,0.866025403784439,
1.,0.866025403784439,1.,0.866025403784439,1.,0.866025403784439,1.,0.866025403784439,
1.,0.866025403784439,1.,0.866025403784439,1.,0.866025403784439,1.,0.866025403784439,
1.,0.866025403784439,1.,0.866025403784439,1.,0.866025403784439,1.,0.866025403784439,
1.,0.866025403784439,1.,0.866025403784439,1.,0.866025403784439,1.,0.866025403784439,
1.,0.866025403784439,1.,0.866025403784439,1.,0.866025403784439,1.,0.866025403784439,
1.,0.866025403784439,1.,0.866025403784439,1.,0.866025403784439,1.,0.866025403784439,
1.,0.866025403784439,1.,0.866025403784439,1.,0.866025403784439,1.,0.866025403784439,
1.,0.866025403784439,1.,0.866025403784439,1.,0.866025403784439,1.,0.866025403784439,
1.,0.866025403784439,1.,0.866025403784439,1.,0.866025403784439,1.,0.866025403784439,
1.,0.866025403784439,1.,0.866025403784439,1.,0.866025403784439,1.,0.866025403784439,
1.,0.866025403784439,1.,0.866025403784439,1.,0.866025403784439,1.,0.866025403784439,
1.,0.866025403784439,1.,0.866025403784439,1.,0.866025403784439,1.,0.866025403784439,
1.,0.866025403784439,1.,0.866025403784439,1.,0.866025403784439,1.,0.866025403784439,
1.,0.866025403784439,1.,0.866025403784439,1.,0.866025403784439,1.,0.866025403784439,
1.,0.866025403784439,1.,0.866025403784439,1.,0.866025403784439,1.,0.866025403784439,
1.,0.866025403784439,1.,0.866025403784439,1.,0.866025403784439,1.,0.866025403784439,
1.)))
REPRESENTATION_ITEM('')
SURFACE()
);
#152=(
BOUNDED_SURFACE()
B_SPLINE_SURFACE(3,2,((#25753,#25754,#25755),(#25756,#25757,#25758),(#25759,
#25760,#25761),(#25762,#25763,#25764),(#25765,#25766,#25767),(#25768,#25769,
#25770),(#25771,#25772,#25773),(#25774,#25775,#25776),(#25777,#25778,#25779),
(#25780,#25781,#25782),(#25783,#25784,#25785),(#25786,#25787,#25788)),
 .UNSPECIFIED.,.F.,.F.,.F.)
B_SPLINE_SURFACE_WITH_KNOTS((4,2,2,2,2,4),(3,3),(1.5707963267949,1.96349540849362,
2.35619449019234,2.74889357189107,2.94524311274043,3.14159265358979),(0.,
1.),.UNSPECIFIED.)
GEOMETRIC_REPRESENTATION_ITEM()
RATIONAL_B_SPLINE_SURFACE(((1.,1.,1.),(1.,1.00006916239765,1.),(1.,0.995525209532845,
1.),(1.,0.979889883266457,1.),(1.,0.96878674661341,1.),(1.,0.945974626665763,
1.),(1.,0.934399279488173,1.),(1.,0.921892172356123,1.),(1.,0.918525872087786,
1.),(1.,0.913964997467621,1.),(1.,0.912767252466787,1.),(1.,0.912773552586276,
1.)))
REPRESENTATION_ITEM('')
SURFACE()
);
#153=(
BOUNDED_SURFACE()
B_SPLINE_SURFACE(3,2,((#25861,#25862,#25863),(#25864,#25865,#25866),(#25867,
#25868,#25869),(#25870,#25871,#25872)),.UNSPECIFIED.,.F.,.F.,.F.)
B_SPLINE_SURFACE_WITH_KNOTS((4,4),(3,3),(0.,0.00117394043814937),(0.,1.),
 .UNSPECIFIED.)
GEOMETRIC_REPRESENTATION_ITEM()
RATIONAL_B_SPLINE_SURFACE(((1.,0.707106781186547,1.),(1.,0.716249811896345,
1.),(1.,0.725602237863733,1.),(1.,0.73518030613814,1.)))
REPRESENTATION_ITEM('')
SURFACE()
);
#154=(
BOUNDED_SURFACE()
B_SPLINE_SURFACE(3,2,((#25874,#25875,#25876),(#25877,#25878,#25879),(#25880,
#25881,#25882),(#25883,#25884,#25885),(#25886,#25887,#25888),(#25889,#25890,
#25891),(#25892,#25893,#25894),(#25895,#25896,#25897),(#25898,#25899,#25900),
(#25901,#25902,#25903),(#25904,#25905,#25906),(#25907,#25908,#25909),(#25910,
#25911,#25912),(#25913,#25914,#25915)),.UNSPECIFIED.,.F.,.F.,.F.)
B_SPLINE_SURFACE_WITH_KNOTS((4,2,2,2,2,2,4),(3,3),(0.00114691688133867,
0.00238785904737931,0.00362880121341995,0.00486974337946059,0.00611068554550123,
0.0085925698775825,0.0110744542096638),(0.,1.),.UNSPECIFIED.)
GEOMETRIC_REPRESENTATION_ITEM()
RATIONAL_B_SPLINE_SURFACE(((1.,0.73518030613814,1.),(1.,0.747335275388272,
1.),(1.,0.761871430108272,1.),(1.,0.792538055362494,1.),(1.,0.808614330671284,
1.),(1.,0.840725708343004,1.),(1.,0.856795297690254,1.),(1.,0.887571556502581,
1.),(1.,0.902056904395603,1.),(1.,0.941769515107707,1.),(1.,0.963202620969872,
1.),(1.,0.992355658691941,1.),(1.,1.00006184400175,1.),(1.,1.,1.)))
REPRESENTATION_ITEM('')
SURFACE()
);
#155=(
BOUNDED_SURFACE()
B_SPLINE_SURFACE(3,2,((#25992,#25993,#25994),(#25995,#25996,#25997),(#25998,
#25999,#26000),(#26001,#26002,#26003),(#26004,#26005,#26006),(#26007,#26008,
#26009),(#26010,#26011,#26012),(#26013,#26014,#26015),(#26016,#26017,#26018),
(#26019,#26020,#26021),(#26022,#26023,#26024),(#26025,#26026,#26027)),
 .UNSPECIFIED.,.F.,.F.,.F.)
B_SPLINE_SURFACE_WITH_KNOTS((4,2,2,2,2,4),(3,3),(1.5707963267949,1.96349540849362,
2.35619449019234,2.74889357189107,2.94524311274043,3.14159265358979),(0.,
1.),.UNSPECIFIED.)
GEOMETRIC_REPRESENTATION_ITEM()
RATIONAL_B_SPLINE_SURFACE(((1.,1.,1.),(1.,1.00006916239765,1.),(1.,0.995525209532845,
1.),(1.,0.979889883266457,1.),(1.,0.968786746613379,1.),(1.,0.945974626665793,
1.),(1.,0.934399279488203,1.),(1.,0.921892172356108,1.),(1.,0.918525872087757,
1.),(1.,0.91396499746765,1.),(1.,0.912767252466765,1.),(1.,0.912773552586276,
1.)))
REPRESENTATION_ITEM('')
SURFACE()
);
#156=(
BOUNDED_SURFACE()
B_SPLINE_SURFACE(3,2,((#26100,#26101,#26102),(#26103,#26104,#26105),(#26106,
#26107,#26108),(#26109,#26110,#26111)),.UNSPECIFIED.,.F.,.F.,.F.)
B_SPLINE_SURFACE_WITH_KNOTS((4,4),(3,3),(-3.46944695195361E-18,0.00117394043814936),
(0.,1.),.UNSPECIFIED.)
GEOMETRIC_REPRESENTATION_ITEM()
RATIONAL_B_SPLINE_SURFACE(((1.,0.707106781186547,1.),(1.,0.716249811896345,
1.),(1.,0.725602237863732,1.),(1.,0.73518030613814,1.)))
REPRESENTATION_ITEM('')
SURFACE()
);
#157=(
BOUNDED_SURFACE()
B_SPLINE_SURFACE(3,2,((#26113,#26114,#26115),(#26116,#26117,#26118),(#26119,
#26120,#26121),(#26122,#26123,#26124),(#26125,#26126,#26127),(#26128,#26129,
#26130),(#26131,#26132,#26133),(#26134,#26135,#26136),(#26137,#26138,#26139),
(#26140,#26141,#26142),(#26143,#26144,#26145),(#26146,#26147,#26148),(#26149,
#26150,#26151),(#26152,#26153,#26154),(#26155,#26156,#26157),(#26158,#26159,
#26160)),.UNSPECIFIED.,.F.,.F.,.F.)
B_SPLINE_SURFACE_WITH_KNOTS((4,2,2,2,2,2,2,4),(3,3),(0.,0.00123568368061385,
0.00247136736122769,0.00370705104184154,0.00494273472245539,0.00617841840306923,
0.00741410208368308,0.00988546944491077),(0.,1.),.UNSPECIFIED.)
GEOMETRIC_REPRESENTATION_ITEM()
RATIONAL_B_SPLINE_SURFACE(((1.,0.73518030613814,1.),(1.,0.74764045440481,
1.),(1.,0.76189463212101,1.),(1.,0.792176992862199,1.),(1.,0.808203903859881,
1.),(1.,0.840503928826669,1.),(1.,0.856707888838066,1.),(1.,0.887226799422037,
1.),(1.,0.901676438639821,1.),(1.,0.928191888592131,1.),(1.,0.940260041314769,
1.),(1.,0.961420720965591,1.),(1.,0.970500238972907,1.),(1.,0.992409706176274,
1.),(1.,1.00002397099295,1.),(1.,1.,1.)))
REPRESENTATION_ITEM('')
SURFACE()
);
#158=(
BOUNDED_SURFACE()
B_SPLINE_SURFACE(3,2,((#26237,#26238,#26239),(#26240,#26241,#26242),(#26243,
#26244,#26245),(#26246,#26247,#26248),(#26249,#26250,#26251),(#26252,#26253,
#26254),(#26255,#26256,#26257),(#26258,#26259,#26260),(#26261,#26262,#26263),
(#26264,#26265,#26266),(#26267,#26268,#26269),(#26270,#26271,#26272)),
 .UNSPECIFIED.,.F.,.F.,.F.)
B_SPLINE_SURFACE_WITH_KNOTS((4,2,2,2,2,4),(3,3),(1.5707963267949,1.96349540849362,
2.35619449019234,2.74889357189107,2.94524311274043,3.14159265358979),(0.,
1.),.UNSPECIFIED.)
GEOMETRIC_REPRESENTATION_ITEM()
RATIONAL_B_SPLINE_SURFACE(((1.,1.,1.),(1.,1.00006916239765,1.),(1.,0.995525209532845,
1.),(1.,0.979889883266457,1.),(1.,0.968786746613379,1.),(1.,0.945974626665793,
1.),(1.,0.934399279488143,1.),(1.,0.921892172356137,1.),(1.,0.918525872087757,
1.),(1.,0.91396499746765,1.),(1.,0.912767252466764,1.),(1.,0.912773552586276,
1.)))
REPRESENTATION_ITEM('')
SURFACE()
);
#159=(
BOUNDED_SURFACE()
B_SPLINE_SURFACE(3,2,((#26345,#26346,#26347),(#26348,#26349,#26350),(#26351,
#26352,#26353),(#26354,#26355,#26356)),.UNSPECIFIED.,.F.,.F.,.F.)
B_SPLINE_SURFACE_WITH_KNOTS((4,4),(3,3),(0.,0.00117394043814937),(0.,1.),
 .UNSPECIFIED.)
GEOMETRIC_REPRESENTATION_ITEM()
RATIONAL_B_SPLINE_SURFACE(((1.,0.707106781186548,1.),(1.,0.716249811896345,
1.),(1.,0.725602237863732,1.),(1.,0.73518030613814,1.)))
REPRESENTATION_ITEM('')
SURFACE()
);
#160=(
BOUNDED_SURFACE()
B_SPLINE_SURFACE(3,2,((#26358,#26359,#26360),(#26361,#26362,#26363),(#26364,
#26365,#26366),(#26367,#26368,#26369),(#26370,#26371,#26372),(#26373,#26374,
#26375),(#26376,#26377,#26378),(#26379,#26380,#26381),(#26382,#26383,#26384),
(#26385,#26386,#26387),(#26388,#26389,#26390),(#26391,#26392,#26393),(#26394,
#26395,#26396),(#26397,#26398,#26399),(#26400,#26401,#26402),(#26403,#26404,
#26405)),.UNSPECIFIED.,.F.,.F.,.F.)
B_SPLINE_SURFACE_WITH_KNOTS((4,2,2,2,2,2,2,4),(3,3),(0.,0.00123568368061384,
0.00247136736122769,0.00370705104184153,0.00494273472245538,0.00617841840306922,
0.00741410208368307,0.00988546944491076),(0.,1.),.UNSPECIFIED.)
GEOMETRIC_REPRESENTATION_ITEM()
RATIONAL_B_SPLINE_SURFACE(((1.,0.73518030613814,1.),(1.,0.74764045440481,
1.),(1.,0.76189463212101,1.),(1.,0.792176992862198,1.),(1.,0.808203903859835,
1.),(1.,0.840503928826715,1.),(1.,0.856707888838066,1.),(1.,0.887226799422036,
1.),(1.,0.901676438639843,1.),(1.,0.928191888592107,1.),(1.,0.940260041314815,
1.),(1.,0.961420720965544,1.),(1.,0.970500238972907,1.),(1.,0.992409706176273,
1.),(1.,1.00002397099295,1.),(1.,1.,1.)))
REPRESENTATION_ITEM('')
SURFACE()
);
#161=(
BOUNDED_SURFACE()
B_SPLINE_SURFACE(3,2,((#26406,#26407,#26408),(#26409,#26410,#26411),(#26412,
#26413,#26414),(#26415,#26416,#26417),(#26418,#26419,#26420),(#26421,#26422,
#26423),(#26424,#26425,#26426),(#26427,#26428,#26429),(#26430,#26431,#26432),
(#26433,#26434,#26435),(#26436,#26437,#26438),(#26439,#26440,#26441),(#26442,
#26443,#26444),(#26445,#26446,#26447)),.UNSPECIFIED.,.F.,.F.,.F.)
B_SPLINE_SURFACE_WITH_KNOTS((4,2,2,2,2,2,4),(3,3),(0.00114691688133867,
0.00238785904737931,0.00362880121341995,0.00486974337946058,0.00611068554550122,
0.0085925698775825,0.0110744542096638),(0.,1.),.UNSPECIFIED.)
GEOMETRIC_REPRESENTATION_ITEM()
RATIONAL_B_SPLINE_SURFACE(((1.,0.73518030613814,1.),(1.,0.747335275388254,
1.),(1.,0.761871430108295,1.),(1.,0.79253805536247,1.),(1.,0.808614330671284,
1.),(1.,0.840725708343004,1.),(1.,0.856795297690208,1.),(1.,0.887571556502627,
1.),(1.,0.902056904395603,1.),(1.,0.941769515107708,1.),(1.,0.963202620969872,
1.),(1.,0.992355658691941,1.),(1.,1.00006184400175,1.),(1.,1.,1.)))
REPRESENTATION_ITEM('')
SURFACE()
);
#162=(
BOUNDED_SURFACE()
B_SPLINE_SURFACE(3,2,((#26449,#26450,#26451),(#26452,#26453,#26454),(#26455,
#26456,#26457),(#26458,#26459,#26460)),.UNSPECIFIED.,.F.,.F.,.F.)
B_SPLINE_SURFACE_WITH_KNOTS((4,4),(3,3),(0.,0.00117394043814936),(0.,1.),
 .UNSPECIFIED.)
GEOMETRIC_REPRESENTATION_ITEM()
RATIONAL_B_SPLINE_SURFACE(((1.,0.707106781186548,1.),(1.,0.716249811896344,
1.),(1.,0.725602237863733,1.),(1.,0.73518030613814,1.)))
REPRESENTATION_ITEM('')
SURFACE()
);
#163=(
BOUNDED_SURFACE()
B_SPLINE_SURFACE(3,2,((#26533,#26534,#26535),(#26536,#26537,#26538),(#26539,
#26540,#26541),(#26542,#26543,#26544),(#26545,#26546,#26547),(#26548,#26549,
#26550),(#26551,#26552,#26553),(#26554,#26555,#26556),(#26557,#26558,#26559),
(#26560,#26561,#26562),(#26563,#26564,#26565),(#26566,#26567,#26568)),
 .UNSPECIFIED.,.F.,.F.,.F.)
B_SPLINE_SURFACE_WITH_KNOTS((4,2,2,2,2,4),(3,3),(1.5707963267949,1.96349540849362,
2.35619449019234,2.74889357189107,2.94524311274043,3.14159265358979),(0.,
1.),.UNSPECIFIED.)
GEOMETRIC_REPRESENTATION_ITEM()
RATIONAL_B_SPLINE_SURFACE(((1.,1.,1.),(1.,1.00006916239762,1.),(1.,0.995525209532876,
1.),(1.,0.979889883266425,1.),(1.,0.968786746613409,1.),(1.,0.945974626665762,
1.),(1.,0.934399279488143,1.),(1.,0.921892172356137,1.),(1.,0.918525872087764,
1.),(1.,0.913964997467643,1.),(1.,0.912767252466769,1.),(1.,0.912773552586275,
1.)))
REPRESENTATION_ITEM('')
SURFACE()
);
#164=(
BOUNDED_SURFACE()
B_SPLINE_SURFACE(3,2,((#26571,#26572,#26573),(#26574,#26575,#26576),(#26577,
#26578,#26579),(#26580,#26581,#26582),(#26583,#26584,#26585),(#26586,#26587,
#26588),(#26589,#26590,#26591),(#26592,#26593,#26594),(#26595,#26596,#26597),
(#26598,#26599,#26600),(#26601,#26602,#26603),(#26604,#26605,#26606)),
 .UNSPECIFIED.,.F.,.F.,.F.)
B_SPLINE_SURFACE_WITH_KNOTS((4,2,2,2,2,4),(3,3),(1.5707963267949,1.96349540849362,
2.35619449019234,2.74889357189107,2.94524311274043,3.14159265358979),(0.,
1.),.UNSPECIFIED.)
GEOMETRIC_REPRESENTATION_ITEM()
RATIONAL_B_SPLINE_SURFACE(((1.,1.,1.),(1.,1.00006916239762,1.),(1.,0.995525209532877,
1.),(1.,0.979889883266426,1.),(1.,0.968786746613333,1.),(1.,0.945974626665839,
1.),(1.,0.934399279488187,1.),(1.,0.921892172356115,1.),(1.,0.918525872087757,
1.),(1.,0.91396499746765,1.),(1.,0.912767252466765,1.),(1.,0.912773552586276,
1.)))
REPRESENTATION_ITEM('')
SURFACE()
);
#165=(
BOUNDED_SURFACE()
B_SPLINE_SURFACE(3,2,((#26679,#26680,#26681),(#26682,#26683,#26684),(#26685,
#26686,#26687),(#26688,#26689,#26690)),.UNSPECIFIED.,.F.,.F.,.F.)
B_SPLINE_SURFACE_WITH_KNOTS((4,4),(3,3),(0.,0.00117394043814935),(0.,1.),
 .UNSPECIFIED.)
GEOMETRIC_REPRESENTATION_ITEM()
RATIONAL_B_SPLINE_SURFACE(((1.,0.707106781186548,1.),(1.,0.716249811896346,
1.),(1.,0.725602237863731,1.),(1.,0.73518030613814,1.)))
REPRESENTATION_ITEM('')
SURFACE()
);
#166=(
BOUNDED_SURFACE()
B_SPLINE_SURFACE(3,2,((#26692,#26693,#26694),(#26695,#26696,#26697),(#26698,
#26699,#26700),(#26701,#26702,#26703),(#26704,#26705,#26706),(#26707,#26708,
#26709),(#26710,#26711,#26712),(#26713,#26714,#26715),(#26716,#26717,#26718),
(#26719,#26720,#26721),(#26722,#26723,#26724),(#26725,#26726,#26727),(#26728,
#26729,#26730),(#26731,#26732,#26733),(#26734,#26735,#26736),(#26737,#26738,
#26739)),.UNSPECIFIED.,.F.,.F.,.F.)
B_SPLINE_SURFACE_WITH_KNOTS((4,2,2,2,2,2,2,4),(3,3),(0.,0.00123568368061385,
0.00247136736122769,0.00370705104184154,0.00494273472245539,0.00617841840306923,
0.00741410208368308,0.00988546944491077),(0.,1.),.UNSPECIFIED.)
GEOMETRIC_REPRESENTATION_ITEM()
RATIONAL_B_SPLINE_SURFACE(((1.,0.73518030613814,1.),(1.,0.747640454404809,
1.),(1.,0.76189463212101,1.),(1.,0.792176992862198,1.),(1.,0.808203903859881,
1.),(1.,0.840503928826668,1.),(1.,0.856707888838043,1.),(1.,0.887226799422059,
1.),(1.,0.901676438639843,1.),(1.,0.928191888592107,1.),(1.,0.940260041314768,
1.),(1.,0.96142072096559,1.),(1.,0.970500238972907,1.),(1.,0.992409706176274,
1.),(1.,1.00002397099295,1.),(1.,1.,1.)))
REPRESENTATION_ITEM('')
SURFACE()
);
#167=(
BOUNDED_SURFACE()
B_SPLINE_SURFACE(3,2,((#26740,#26741,#26742),(#26743,#26744,#26745),(#26746,
#26747,#26748),(#26749,#26750,#26751),(#26752,#26753,#26754),(#26755,#26756,
#26757),(#26758,#26759,#26760),(#26761,#26762,#26763),(#26764,#26765,#26766),
(#26767,#26768,#26769),(#26770,#26771,#26772),(#26773,#26774,#26775),(#26776,
#26777,#26778),(#26779,#26780,#26781)),.UNSPECIFIED.,.F.,.F.,.F.)
B_SPLINE_SURFACE_WITH_KNOTS((4,2,2,2,2,2,4),(3,3),(0.00114691688133867,
0.00238785904737931,0.00362880121341994,0.00486974337946058,0.00611068554550122,
0.0085925698775825,0.0110744542096638),(0.,1.),.UNSPECIFIED.)
GEOMETRIC_REPRESENTATION_ITEM()
RATIONAL_B_SPLINE_SURFACE(((1.,0.73518030613814,1.),(1.,0.747335275388254,
1.),(1.,0.761871430108295,1.),(1.,0.79253805536247,1.),(1.,0.808614330671261,
1.),(1.,0.840725708343027,1.),(1.,0.856795297690161,1.),(1.,0.887571556502673,
1.),(1.,0.90205690439558,1.),(1.,0.941769515107753,1.),(1.,0.963202620969917,
1.),(1.,0.992355658691895,1.),(1.,1.00006184400178,1.),(1.,1.,1.)))
REPRESENTATION_ITEM('')
SURFACE()
);
#168=(
BOUNDED_SURFACE()
B_SPLINE_SURFACE(3,2,((#26783,#26784,#26785),(#26786,#26787,#26788),(#26789,
#26790,#26791),(#26792,#26793,#26794)),.UNSPECIFIED.,.F.,.F.,.F.)
B_SPLINE_SURFACE_WITH_KNOTS((4,4),(3,3),(0.,0.00117394043814939),(0.,1.),
 .UNSPECIFIED.)
GEOMETRIC_REPRESENTATION_ITEM()
RATIONAL_B_SPLINE_SURFACE(((1.,0.707106781186547,1.),(1.,0.716249811896344,
1.),(1.,0.725602237863731,1.),(1.,0.73518030613814,1.)))
REPRESENTATION_ITEM('')
SURFACE()
);
#169=(
BOUNDED_SURFACE()
B_SPLINE_SURFACE(3,2,((#26867,#26868,#26869),(#26870,#26871,#26872),(#26873,
#26874,#26875),(#26876,#26877,#26878),(#26879,#26880,#26881),(#26882,#26883,
#26884),(#26885,#26886,#26887),(#26888,#26889,#26890),(#26891,#26892,#26893),
(#26894,#26895,#26896),(#26897,#26898,#26899),(#26900,#26901,#26902)),
 .UNSPECIFIED.,.F.,.F.,.F.)
B_SPLINE_SURFACE_WITH_KNOTS((4,2,2,2,2,4),(3,3),(1.5707963267949,1.96349540849362,
2.35619449019234,2.74889357189107,2.94524311274043,3.14159265358979),(0.,
1.),.UNSPECIFIED.)
GEOMETRIC_REPRESENTATION_ITEM()
RATIONAL_B_SPLINE_SURFACE(((1.,1.,1.),(1.,1.00006916239765,1.),(1.,0.995525209532845,
1.),(1.,0.979889883266457,1.),(1.,0.968786746613394,1.),(1.,0.945974626665778,
1.),(1.,0.934399279488158,1.),(1.,0.92189217235613,1.),(1.,0.918525872087771,
1.),(1.,0.913964997467635,1.),(1.,0.912767252466775,1.),(1.,0.912773552586276,
1.)))
REPRESENTATION_ITEM('')
SURFACE()
);
#170=(
BOUNDED_SURFACE()
B_SPLINE_SURFACE(3,2,((#26979,#26980,#26981),(#26982,#26983,#26984),(#26985,
#26986,#26987),(#26988,#26989,#26990),(#26991,#26992,#26993),(#26994,#26995,
#26996),(#26997,#26998,#26999),(#27000,#27001,#27002)),.UNSPECIFIED.,.F.,
 .F.,.F.)
B_SPLINE_SURFACE_WITH_KNOTS((4,2,2,4),(3,3),(0.,0.00109785791663237,0.00219571583326473,
0.00439143166652947),(0.,1.),.UNSPECIFIED.)
GEOMETRIC_REPRESENTATION_ITEM()
RATIONAL_B_SPLINE_SURFACE(((1.,0.707106781186549,1.),(1.,0.75082909814959,
1.),(1.,0.792349205138272,1.),(1.,0.866373214279049,1.),(1.,0.897828374333773,
1.),(1.,0.973720746971429,1.),(1.,1.00018625880497,1.),(1.,1.,1.)))
REPRESENTATION_ITEM('')
SURFACE()
);
#171=(
BOUNDED_SURFACE()
B_SPLINE_SURFACE(3,2,((#27018,#27019,#27020),(#27021,#27022,#27023),(#27024,
#27025,#27026),(#27027,#27028,#27029),(#27030,#27031,#27032),(#27033,#27034,
#27035),(#27036,#27037,#27038),(#27039,#27040,#27041)),.UNSPECIFIED.,.F.,
 .F.,.F.)
B_SPLINE_SURFACE_WITH_KNOTS((4,2,2,4),(3,3),(0.,0.00109785791663237,0.00219571583326474,
0.00439143166652948),(0.,1.),.UNSPECIFIED.)
GEOMETRIC_REPRESENTATION_ITEM()
RATIONAL_B_SPLINE_SURFACE(((1.,0.707106781186548,1.),(1.,0.75082909814959,
1.),(1.,0.792349205138269,1.),(1.,0.866373214279046,1.),(1.,0.897828374333914,
1.),(1.,0.973720746971144,1.),(1.,1.00018625880519,1.),(1.,1.,1.)))
REPRESENTATION_ITEM('')
SURFACE()
);
#172=(
BOUNDED_SURFACE()
B_SPLINE_SURFACE(3,2,((#27042,#27043,#27044),(#27045,#27046,#27047),(#27048,
#27049,#27050),(#27051,#27052,#27053),(#27054,#27055,#27056),(#27057,#27058,
#27059),(#27060,#27061,#27062),(#27063,#27064,#27065)),.UNSPECIFIED.,.F.,
 .F.,.F.)
B_SPLINE_SURFACE_WITH_KNOTS((4,2,2,4),(3,3),(0.,0.00109785791663237,0.00219571583326473,
0.00439143166652947),(0.,1.),.UNSPECIFIED.)
GEOMETRIC_REPRESENTATION_ITEM()
RATIONAL_B_SPLINE_SURFACE(((1.,0.707106781186548,1.),(1.,0.750829098149542,
1.),(1.,0.79234920513833,1.),(1.,0.866373214278985,1.),(1.,0.897828374333792,
1.),(1.,0.973720746971387,1.),(1.,1.000186258805,1.),(1.,1.,1.)))
REPRESENTATION_ITEM('')
SURFACE()
);
#173=(
BOUNDED_SURFACE()
B_SPLINE_SURFACE(3,2,((#27081,#27082,#27083),(#27084,#27085,#27086),(#27087,
#27088,#27089),(#27090,#27091,#27092),(#27093,#27094,#27095),(#27096,#27097,
#27098),(#27099,#27100,#27101),(#27102,#27103,#27104)),.UNSPECIFIED.,.F.,
 .F.,.F.)
B_SPLINE_SURFACE_WITH_KNOTS((4,2,2,4),(3,3),(0.,0.00109785791663236,0.00219571583326473,
0.00439143166652946),(0.,1.),.UNSPECIFIED.)
GEOMETRIC_REPRESENTATION_ITEM()
RATIONAL_B_SPLINE_SURFACE(((1.,0.707106781186548,1.),(1.,0.750829098149437,
1.),(1.,0.792349205138475,1.),(1.,0.866373214278842,1.),(1.,0.897828374333691,
1.),(1.,0.973720746971589,1.),(1.,1.00018625880485,1.),(1.,1.,1.)))
REPRESENTATION_ITEM('')
SURFACE()
);
#174=(
BOUNDED_SURFACE()
B_SPLINE_SURFACE(3,2,((#27105,#27106,#27107),(#27108,#27109,#27110),(#27111,
#27112,#27113),(#27114,#27115,#27116),(#27117,#27118,#27119),(#27120,#27121,
#27122),(#27123,#27124,#27125),(#27126,#27127,#27128)),.UNSPECIFIED.,.F.,
 .F.,.F.)
B_SPLINE_SURFACE_WITH_KNOTS((4,2,2,4),(3,3),(0.,0.00109785791663237,0.00219571583326474,
0.00439143166652948),(0.,1.),.UNSPECIFIED.)
GEOMETRIC_REPRESENTATION_ITEM()
RATIONAL_B_SPLINE_SURFACE(((1.,0.707106781186548,1.),(1.,0.750829098149496,
1.),(1.,0.792349205138392,1.),(1.,0.866373214278923,1.),(1.,0.897828374333732,
1.),(1.,0.973720746971509,1.),(1.,1.00018625880491,1.),(1.,1.,1.)))
REPRESENTATION_ITEM('')
SURFACE()
);
#175=(
BOUNDED_SURFACE()
B_SPLINE_SURFACE(3,2,((#27141,#27142,#27143),(#27144,#27145,#27146),(#27147,
#27148,#27149),(#27150,#27151,#27152),(#27153,#27154,#27155),(#27156,#27157,
#27158),(#27159,#27160,#27161),(#27162,#27163,#27164)),.UNSPECIFIED.,.F.,
 .F.,.F.)
B_SPLINE_SURFACE_WITH_KNOTS((4,2,2,4),(3,3),(-7.58941520739853E-19,0.00109785791663237,
0.00219571583326474,0.00439143166652947),(0.,1.),.UNSPECIFIED.)
GEOMETRIC_REPRESENTATION_ITEM()
RATIONAL_B_SPLINE_SURFACE(((1.,0.707106781186548,1.),(1.,0.750829098149468,
1.),(1.,0.792349205138434,1.),(1.,0.866373214278884,1.),(1.,0.897828374333793,
1.),(1.,0.973720746971388,1.),(1.,1.000186258805,1.),(1.,1.,1.)))
REPRESENTATION_ITEM('')
SURFACE()
);
#183=(
BOUNDED_CURVE()
B_SPLINE_CURVE(2,(#11448,#11449,#11450),.UNSPECIFIED.,.F.,.F.)
B_SPLINE_CURVE_WITH_KNOTS((3,3),(1.85021493467955,2.79463772249644),
 .UNSPECIFIED.)
CURVE()
GEOMETRIC_REPRESENTATION_ITEM()
RATIONAL_B_SPLINE_CURVE((1.69747704818698,1.78740157480315,1.78740157480315))
REPRESENTATION_ITEM('')
);
#184=(
BOUNDED_CURVE()
B_SPLINE_CURVE(2,(#11451,#11452,#11453),.UNSPECIFIED.,.F.,.F.)
B_SPLINE_CURVE_WITH_KNOTS((3,3),(2.79463772249644,3.73906051031331),
 .UNSPECIFIED.)
CURVE()
GEOMETRIC_REPRESENTATION_ITEM()
RATIONAL_B_SPLINE_CURVE((1.78740157480315,1.78740157480315,1.69747704818698))
REPRESENTATION_ITEM('')
);
#185=(
BOUNDED_CURVE()
B_SPLINE_CURVE(2,(#11462,#11463,#11464),.UNSPECIFIED.,.F.,.F.)
B_SPLINE_CURVE_WITH_KNOTS((3,3),(1.85021493467955,2.79463772249643),
 .UNSPECIFIED.)
CURVE()
GEOMETRIC_REPRESENTATION_ITEM()
RATIONAL_B_SPLINE_CURVE((1.69747704818698,1.78740157480315,1.78740157480315))
REPRESENTATION_ITEM('')
);
#186=(
BOUNDED_CURVE()
B_SPLINE_CURVE(2,(#11465,#11466,#11467),.UNSPECIFIED.,.F.,.F.)
B_SPLINE_CURVE_WITH_KNOTS((3,3),(2.79463772249643,3.73906051031332),
 .UNSPECIFIED.)
CURVE()
GEOMETRIC_REPRESENTATION_ITEM()
RATIONAL_B_SPLINE_CURVE((1.78740157480315,1.78740157480315,1.69747704818698))
REPRESENTATION_ITEM('')
);
#187=(
BOUNDED_CURVE()
B_SPLINE_CURVE(2,(#11476,#11477,#11478),.UNSPECIFIED.,.F.,.F.)
B_SPLINE_CURVE_WITH_KNOTS((3,3),(1.85021493467955,2.79463772249644),
 .UNSPECIFIED.)
CURVE()
GEOMETRIC_REPRESENTATION_ITEM()
RATIONAL_B_SPLINE_CURVE((1.69747704818698,1.78740157480315,1.78740157480315))
REPRESENTATION_ITEM('')
);
#188=(
BOUNDED_CURVE()
B_SPLINE_CURVE(2,(#11479,#11480,#11481),.UNSPECIFIED.,.F.,.F.)
B_SPLINE_CURVE_WITH_KNOTS((3,3),(2.79463772249644,3.73906051031331),
 .UNSPECIFIED.)
CURVE()
GEOMETRIC_REPRESENTATION_ITEM()
RATIONAL_B_SPLINE_CURVE((1.78740157480315,1.78740157480315,1.69747704818698))
REPRESENTATION_ITEM('')
);
#189=(
BOUNDED_CURVE()
B_SPLINE_CURVE(2,(#11490,#11491,#11492),.UNSPECIFIED.,.F.,.F.)
B_SPLINE_CURVE_WITH_KNOTS((3,3),(1.85021493467955,2.79463772249643),
 .UNSPECIFIED.)
CURVE()
GEOMETRIC_REPRESENTATION_ITEM()
RATIONAL_B_SPLINE_CURVE((1.69747704818698,1.78740157480315,1.78740157480315))
REPRESENTATION_ITEM('')
);
#190=(
BOUNDED_CURVE()
B_SPLINE_CURVE(2,(#11493,#11494,#11495),.UNSPECIFIED.,.F.,.F.)
B_SPLINE_CURVE_WITH_KNOTS((3,3),(2.79463772249643,3.73906051031332),
 .UNSPECIFIED.)
CURVE()
GEOMETRIC_REPRESENTATION_ITEM()
RATIONAL_B_SPLINE_CURVE((1.78740157480315,1.78740157480315,1.69747704818698))
REPRESENTATION_ITEM('')
);
#191=(
BOUNDED_CURVE()
B_SPLINE_CURVE(2,(#11504,#11505,#11506),.UNSPECIFIED.,.F.,.F.)
B_SPLINE_CURVE_WITH_KNOTS((3,3),(1.85021493467955,2.79463772249643),
 .UNSPECIFIED.)
CURVE()
GEOMETRIC_REPRESENTATION_ITEM()
RATIONAL_B_SPLINE_CURVE((1.69747704818698,1.78740157480315,1.78740157480316))
REPRESENTATION_ITEM('')
);
#192=(
BOUNDED_CURVE()
B_SPLINE_CURVE(2,(#11507,#11508,#11509),.UNSPECIFIED.,.F.,.F.)
B_SPLINE_CURVE_WITH_KNOTS((3,3),(2.79463772249643,3.73906051031331),
 .UNSPECIFIED.)
CURVE()
GEOMETRIC_REPRESENTATION_ITEM()
RATIONAL_B_SPLINE_CURVE((1.78740157480315,1.78740157480316,1.69747704818699))
REPRESENTATION_ITEM('')
);
#193=(
BOUNDED_CURVE()
B_SPLINE_CURVE(2,(#11518,#11519,#11520),.UNSPECIFIED.,.F.,.F.)
B_SPLINE_CURVE_WITH_KNOTS((3,3),(1.85021493467955,2.79463772249643),
 .UNSPECIFIED.)
CURVE()
GEOMETRIC_REPRESENTATION_ITEM()
RATIONAL_B_SPLINE_CURVE((1.69747704818698,1.78740157480315,1.78740157480315))
REPRESENTATION_ITEM('')
);
#194=(
BOUNDED_CURVE()
B_SPLINE_CURVE(2,(#11521,#11522,#11523),.UNSPECIFIED.,.F.,.F.)
B_SPLINE_CURVE_WITH_KNOTS((3,3),(2.79463772249643,3.73906051031331),
 .UNSPECIFIED.)
CURVE()
GEOMETRIC_REPRESENTATION_ITEM()
RATIONAL_B_SPLINE_CURVE((1.78740157480315,1.78740157480315,1.69747704818698))
REPRESENTATION_ITEM('')
);
#195=(
BOUNDED_CURVE()
B_SPLINE_CURVE(2,(#14999,#15000,#15001,#15002,#15003,#15004,#15005,#15006,
#15007,#15008,#15009,#15010,#15011,#15012,#15013,#15014,#15015,#15016,#15017,
#15018,#15019,#15020,#15021,#15022,#15023,#15024,#15025,#15026,#15027,#15028,
#15029,#15030,#15031,#15032,#15033,#15034,#15035,#15036,#15037,#15038,#15039,
#15040,#15041,#15042,#15043,#15044,#15045,#15046,#15047,#15048,#15049,#15050,
#15051,#15052,#15053,#15054,#15055,#15056,#15057,#15058,#15059,#15060,#15061,
#15062,#15063,#15064,#15065,#15066,#15067,#15068,#15069,#15070,#15071,#15072,
#15073,#15074,#15075,#15076,#15077,#15078,#15079,#15080,#15081,#15082,#15083,
#15084,#15085,#15086,#15087,#15088,#15089,#15090,#15091,#15092,#15093,#15094,
#15095,#15096,#15097,#15098,#15099,#15100,#15101,#15102,#15103,#15104,#15105,
#15106,#15107,#15108,#15109,#15110,#15111,#15112,#15113,#15114,#15115,#15116,
#15117,#15118,#15119,#15120,#15121,#15122,#15123,#15124,#15125,#15126,#15127,
#15128,#15129,#15130,#15131,#15132,#15133,#15134,#15135,#15136,#15137,#15138,
#15139,#15140,#15141,#15142,#15143,#15144,#15145,#15146,#15147,#15148,#15149,
#15150,#15151,#15152,#15153,#15154,#15155,#15156,#15157,#15158,#15159,#15160,
#15161,#15162,#15163,#15164,#15165,#15166,#15167,#15168,#15169,#15170,#15171,
#15172,#15173,#15174,#15175,#15176,#15177,#15178,#15179,#15180,#15181,#15182,
#15183,#15184,#15185,#15186,#15187,#15188,#15189,#15190,#15191,#15192,#15193,
#15194,#15195,#15196,#15197,#15198,#15199,#15200,#15201,#15202,#15203,#15204,
#15205,#15206,#15207,#15208,#15209,#15210,#15211,#15212,#15213,#15214,#15215,
#15216,#15217,#15218,#15219,#15220,#15221,#15222,#15223,#15224,#15225,#15226,
#15227,#15228,#15229,#15230,#15231,#15232,#15233,#15234,#15235,#15236,#15237,
#15238,#15239,#15240,#15241,#15242,#15243,#15244,#15245,#15246,#15247,#15248,
#15249,#15250,#15251,#15252,#15253,#15254,#15255,#15256,#15257,#15258,#15259,
#15260,#15261,#15262,#15263,#15264,#15265,#15266,#15267,#15268,#15269,#15270,
#15271),.UNSPECIFIED.,.F.,.F.)
B_SPLINE_CURVE_WITH_KNOTS((3,2,2,2,2,2,2,2,2,2,2,2,2,2,2,2,2,2,2,2,2,2,
2,2,2,2,2,2,2,2,2,2,2,2,2,2,2,2,2,2,2,2,2,2,2,2,2,2,2,2,2,2,2,2,2,2,2,2,
2,2,2,2,2,2,2,2,2,2,2,2,2,2,2,2,2,2,2,2,2,2,2,2,2,2,2,2,2,2,2,2,2,2,2,2,
2,2,2,2,2,2,2,2,2,2,2,2,2,2,2,2,2,2,2,2,2,2,2,2,2,2,2,2,2,2,2,2,2,2,2,2,
2,2,2,2,2,2,3),(0.700304458117265,0.701646090534979,0.703703703703704,0.705761316872428,
0.707818930041152,0.709876543209877,0.711934156378601,0.713991769547325,
0.716049382716049,0.718106995884774,0.720164609053498,0.722222222222222,
0.724279835390947,0.726337448559671,0.728395061728395,0.730452674897119,
0.732510288065844,0.734567901234568,0.736625514403292,0.738683127572016,
0.740740740740741,0.742798353909465,0.744855967078189,0.746913580246914,
0.748971193415638,0.751028806584362,0.753086419753086,0.755144032921811,
0.757201646090535,0.759259259259259,0.761316872427984,0.763374485596708,
0.765432098765432,0.767489711934156,0.769547325102881,0.771604938271605,
0.773662551440329,0.775720164609053,0.777777777777778,0.779835390946502,
0.781893004115226,0.783950617283951,0.786008230452675,0.788065843621399,
0.790123456790123,0.792181069958848,0.794238683127572,0.796296296296296,
0.798353909465021,0.800411522633745,0.802469135802469,0.804526748971193,
0.806584362139918,0.808641975308642,0.810699588477366,0.812757201646091,
0.814814814814815,0.816872427983539,0.818930041152263,0.820987654320988,
0.823045267489712,0.825102880658436,0.827160493827161,0.829218106995885,
0.831275720164609,0.833333333333333,0.835390946502058,0.837448559670782,
0.839506172839506,0.84156378600823,0.843621399176955,0.845679012345679,
0.847736625514403,0.849794238683128,0.851851851851852,0.853909465020576,
0.8559670781893,0.858024691358025,0.860082304526749,0.862139917695473,0.864197530864197,
0.866255144032922,0.868312757201646,0.87037037037037,0.872427983539095,
0.874485596707819,0.876543209876543,0.878600823045268,0.880658436213992,
0.882716049382716,0.88477366255144,0.886831275720165,0.888888888888889,
0.890946502057613,0.893004115226337,0.895061728395062,0.897119341563786,
0.89917695473251,0.901234567901235,0.903292181069959,0.905349794238683,
0.907407407407407,0.909465020576132,0.911522633744856,0.91358024691358,
0.915637860082305,0.917695473251029,0.919753086419753,0.921810699588477,
0.923868312757202,0.925925925925926,0.92798353909465,0.930041152263374,
0.932098765432099,0.934156378600823,0.936213991769547,0.938271604938272,
0.940329218106996,0.94238683127572,0.944444444444444,0.946502057613169,
0.948559670781893,0.950617283950617,0.952674897119342,0.954732510288066,
0.95679012345679,0.958847736625514,0.960905349794239,0.962962962962963,
0.965020576131687,0.967078189300412,0.969135802469136,0.97119341563786,
0.973251028806584,0.975308641975309,0.977366255144033,0.977769992664587),
 .UNSPECIFIED.)
CURVE()
GEOMETRIC_REPRESENTATION_ITEM()
RATIONAL_B_SPLINE_CURVE((0.939206117316363,0.912644094543595,1.,0.866025403784439,
1.,0.866025403784439,1.,0.866025403784439,1.,0.866025403784439,1.,0.866025403784439,
1.,0.866025403784439,1.,0.866025403784439,1.,0.866025403784439,1.,0.866025403784439,
1.,0.866025403784439,1.,0.866025403784439,1.,0.866025403784439,1.,0.866025403784439,
1.,0.866025403784439,1.,0.866025403784439,1.,0.866025403784439,1.,0.866025403784439,
1.,0.866025403784439,1.,0.866025403784439,1.,0.866025403784439,1.,0.866025403784439,
1.,0.866025403784439,1.,0.866025403784439,1.,0.866025403784439,1.,0.866025403784439,
1.,0.866025403784439,1.,0.866025403784439,1.,0.866025403784439,1.,0.866025403784439,
1.,0.866025403784439,1.,0.866025403784439,1.,0.866025403784439,1.,0.866025403784439,
1.,0.866025403784439,1.,0.866025403784439,1.,0.866025403784439,1.,0.866025403784439,
1.,0.866025403784439,1.,0.866025403784439,1.,0.866025403784439,1.,0.866025403784439,
1.,0.866025403784439,1.,0.866025403784439,1.,0.866025403784439,1.,0.866025403784439,
1.,0.866025403784439,1.,0.866025403784439,1.,0.866025403784439,1.,0.866025403784439,
1.,0.866025403784439,1.,0.866025403784439,1.,0.866025403784439,1.,0.866025403784439,
1.,0.866025403784439,1.,0.866025403784439,1.,0.866025403784439,1.,0.866025403784439,
1.,0.866025403784439,1.,0.866025403784439,1.,0.866025403784439,1.,0.866025403784439,
1.,0.866025403784439,1.,0.866025403784439,1.,0.866025403784439,1.,0.866025403784439,
1.,0.866025403784439,1.,0.866025403784439,1.,0.866025403784439,1.,0.866025403784439,
1.,0.866025403784439,1.,0.866025403784439,1.,0.866025403784439,1.,0.866025403784439,
1.,0.866025403784439,1.,0.866025403784439,1.,0.866025403784439,1.,0.866025403784439,
1.,0.866025403784439,1.,0.866025403784439,1.,0.866025403784439,1.,0.866025403784439,
1.,0.866025403784439,1.,0.866025403784439,1.,0.866025403784439,1.,0.866025403784439,
1.,0.866025403784439,1.,0.866025403784439,1.,0.866025403784439,1.,0.866025403784439,
1.,0.866025403784439,1.,0.866025403784439,1.,0.866025403784439,1.,0.866025403784439,
1.,0.866025403784439,1.,0.866025403784439,1.,0.866025403784439,1.,0.866025403784439,
1.,0.866025403784439,1.,0.866025403784439,1.,0.866025403784439,1.,0.866025403784439,
1.,0.866025403784439,1.,0.866025403784439,1.,0.866025403784439,1.,0.866025403784439,
1.,0.866025403784439,1.,0.866025403784439,1.,0.866025403784439,1.,0.866025403784439,
1.,0.866025403784439,1.,0.866025403784439,1.,0.866025403784439,1.,0.866025403784439,
1.,0.866025403784439,1.,0.866025403784439,1.,0.866025403784439,1.,0.866025403784439,
1.,0.866025403784439,1.,0.866025403784439,1.,0.866025403784439,1.,0.866025403784439,
1.,0.866025403784439,1.,0.866025403784439,1.,0.866025403784439,1.,0.866025403784439,
1.,0.866025403784439,1.,0.866025403784439,1.,0.866025403784439,1.,0.866025403784439,
1.,0.866025403784439,1.,0.866025403784439,1.,0.866025403784439,1.,0.866025403784439,
1.,0.866025403784439,1.,0.973711982351429,0.957740246914744))
REPRESENTATION_ITEM('')
);
#196=(
BOUNDED_CURVE()
B_SPLINE_CURVE(2,(#15272,#15273,#15274,#15275,#15276,#15277,#15278,#15279,
#15280,#15281,#15282,#15283,#15284,#15285,#15286,#15287,#15288,#15289,#15290,
#15291,#15292,#15293,#15294,#15295,#15296,#15297,#15298,#15299,#15300,#15301,
#15302,#15303,#15304,#15305,#15306,#15307,#15308,#15309,#15310,#15311,#15312,
#15313,#15314,#15315,#15316,#15317,#15318,#15319,#15320,#15321,#15322,#15323,
#15324,#15325,#15326,#15327,#15328,#15329,#15330,#15331,#15332,#15333,#15334,
#15335,#15336,#15337,#15338,#15339,#15340,#15341,#15342,#15343,#15344,#15345,
#15346,#15347,#15348,#15349,#15350,#15351,#15352,#15353,#15354,#15355,#15356,
#15357,#15358,#15359,#15360,#15361,#15362,#15363,#15364,#15365,#15366,#15367,
#15368,#15369,#15370,#15371,#15372,#15373,#15374,#15375,#15376,#15377,#15378,
#15379,#15380,#15381,#15382,#15383,#15384,#15385,#15386,#15387,#15388,#15389,
#15390,#15391,#15392,#15393,#15394,#15395,#15396,#15397,#15398,#15399,#15400,
#15401,#15402,#15403,#15404,#15405,#15406,#15407,#15408,#15409,#15410,#15411,
#15412,#15413,#15414,#15415,#15416,#15417,#15418,#15419,#15420,#15421,#15422,
#15423,#15424,#15425,#15426,#15427,#15428,#15429,#15430,#15431,#15432,#15433,
#15434,#15435,#15436,#15437,#15438,#15439,#15440,#15441,#15442,#15443,#15444,
#15445,#15446,#15447,#15448,#15449,#15450,#15451,#15452,#15453,#15454,#15455,
#15456,#15457,#15458,#15459,#15460,#15461,#15462,#15463,#15464,#15465,#15466,
#15467,#15468,#15469,#15470,#15471,#15472,#15473,#15474,#15475,#15476,#15477,
#15478,#15479,#15480,#15481,#15482,#15483,#15484,#15485,#15486,#15487,#15488,
#15489,#15490,#15491,#15492,#15493,#15494,#15495,#15496,#15497,#15498,#15499,
#15500,#15501,#15502,#15503,#15504,#15505,#15506,#15507,#15508,#15509,#15510,
#15511,#15512,#15513,#15514,#15515,#15516,#15517,#15518,#15519,#15520,#15521,
#15522,#15523,#15524,#15525,#15526,#15527,#15528,#15529,#15530,#15531,#15532,
#15533,#15534,#15535,#15536,#15537,#15538,#15539,#15540,#15541,#15542,#15543,
#15544,#15545,#15546),.UNSPECIFIED.,.F.,.F.)
B_SPLINE_CURVE_WITH_KNOTS((3,2,2,2,2,2,2,2,2,2,2,2,2,2,2,2,2,2,2,2,2,2,
2,2,2,2,2,2,2,2,2,2,2,2,2,2,2,2,2,2,2,2,2,2,2,2,2,2,2,2,2,2,2,2,2,2,2,2,
2,2,2,2,2,2,2,2,2,2,2,2,2,2,2,2,2,2,2,2,2,2,2,2,2,2,2,2,2,2,2,2,2,2,2,2,
2,2,2,2,2,2,2,2,2,2,2,2,2,2,2,2,2,2,2,2,2,2,2,2,2,2,2,2,2,2,2,2,2,2,2,2,
2,2,2,2,2,2,2,3),(0.690118789609514,0.691358024691358,0.693415637860082,
0.695473251028807,0.697530864197531,0.699588477366255,0.701646090534979,
0.703703703703704,0.705761316872428,0.707818930041152,0.709876543209877,
0.711934156378601,0.713991769547325,0.716049382716049,0.718106995884774,
0.720164609053498,0.722222222222222,0.724279835390947,0.726337448559671,
0.728395061728395,0.730452674897119,0.732510288065844,0.734567901234568,
0.736625514403292,0.738683127572016,0.740740740740741,0.742798353909465,
0.744855967078189,0.746913580246914,0.748971193415638,0.751028806584362,
0.753086419753086,0.755144032921811,0.757201646090535,0.759259259259259,
0.761316872427984,0.763374485596708,0.765432098765432,0.767489711934156,
0.769547325102881,0.771604938271605,0.773662551440329,0.775720164609053,
0.777777777777778,0.779835390946502,0.781893004115226,0.783950617283951,
0.786008230452675,0.788065843621399,0.790123456790123,0.792181069958848,
0.794238683127572,0.796296296296296,0.798353909465021,0.800411522633745,
0.802469135802469,0.804526748971193,0.806584362139918,0.808641975308642,
0.810699588477366,0.812757201646091,0.814814814814815,0.816872427983539,
0.818930041152263,0.820987654320988,0.823045267489712,0.825102880658436,
0.827160493827161,0.829218106995885,0.831275720164609,0.833333333333333,
0.835390946502058,0.837448559670782,0.839506172839506,0.84156378600823,
0.843621399176955,0.845679012345679,0.847736625514403,0.849794238683128,
0.851851851851852,0.853909465020576,0.8559670781893,0.858024691358025,0.860082304526749,
0.862139917695473,0.864197530864197,0.866255144032922,0.868312757201646,
0.87037037037037,0.872427983539095,0.874485596707819,0.876543209876543,
0.878600823045268,0.880658436213992,0.882716049382716,0.88477366255144,
0.886831275720165,0.888888888888889,0.890946502057613,0.893004115226337,
0.895061728395062,0.897119341563786,0.89917695473251,0.901234567901235,
0.903292181069959,0.905349794238683,0.907407407407407,0.909465020576132,
0.911522633744856,0.91358024691358,0.915637860082305,0.917695473251029,
0.919753086419753,0.921810699588477,0.923868312757202,0.925925925925926,
0.92798353909465,0.930041152263374,0.932098765432099,0.934156378600823,
0.936213991769547,0.938271604938272,0.940329218106996,0.94238683127572,
0.944444444444444,0.946502057613169,0.948559670781893,0.950617283950617,
0.952674897119342,0.954732510288066,0.95679012345679,0.958847736625514,
0.960905349794239,0.962962962962963,0.965020576131687,0.967078189300412,
0.969135802469136,0.970064444260615),.UNSPECIFIED.)
CURVE()
GEOMETRIC_REPRESENTATION_ITEM()
RATIONAL_B_SPLINE_CURVE((0.935815127542769,0.919311354422782,1.,0.866025403784439,
1.,0.866025403784439,1.,0.866025403784439,1.,0.866025403784439,1.,0.866025403784439,
1.,0.866025403784439,1.,0.866025403784439,1.,0.866025403784439,1.,0.866025403784439,
1.,0.866025403784439,1.,0.866025403784439,1.,0.866025403784439,1.,0.866025403784439,
1.,0.866025403784439,1.,0.866025403784439,1.,0.866025403784439,1.,0.866025403784439,
1.,0.866025403784439,1.,0.866025403784439,1.,0.866025403784439,1.,0.866025403784439,
1.,0.866025403784439,1.,0.866025403784439,1.,0.866025403784439,1.,0.866025403784439,
1.,0.866025403784439,1.,0.866025403784439,1.,0.866025403784439,1.,0.866025403784439,
1.,0.866025403784439,1.,0.866025403784439,1.,0.866025403784439,1.,0.866025403784439,
1.,0.866025403784439,1.,0.866025403784439,1.,0.866025403784439,1.,0.866025403784439,
1.,0.866025403784439,1.,0.866025403784439,1.,0.866025403784439,1.,0.866025403784439,
1.,0.866025403784439,1.,0.866025403784439,1.,0.866025403784439,1.,0.866025403784439,
1.,0.866025403784439,1.,0.866025403784439,1.,0.866025403784439,1.,0.866025403784439,
1.,0.866025403784439,1.,0.866025403784439,1.,0.866025403784439,1.,0.866025403784439,
1.,0.866025403784439,1.,0.866025403784439,1.,0.866025403784439,1.,0.866025403784439,
1.,0.866025403784439,1.,0.866025403784439,1.,0.866025403784439,1.,0.866025403784439,
1.,0.866025403784439,1.,0.866025403784439,1.,0.866025403784439,1.,0.866025403784439,
1.,0.866025403784439,1.,0.866025403784439,1.,0.866025403784439,1.,0.866025403784439,
1.,0.866025403784439,1.,0.866025403784439,1.,0.866025403784439,1.,0.866025403784439,
1.,0.866025403784439,1.,0.866025403784439,1.,0.866025403784439,1.,0.866025403784439,
1.,0.866025403784439,1.,0.866025403784439,1.,0.866025403784439,1.,0.866025403784439,
1.,0.866025403784439,1.,0.866025403784439,1.,0.866025403784439,1.,0.866025403784439,
1.,0.866025403784439,1.,0.866025403784439,1.,0.866025403784439,1.,0.866025403784439,
1.,0.866025403784439,1.,0.866025403784439,1.,0.866025403784439,1.,0.866025403784439,
1.,0.866025403784439,1.,0.866025403784439,1.,0.866025403784439,1.,0.866025403784439,
1.,0.866025403784439,1.,0.866025403784439,1.,0.866025403784439,1.,0.866025403784439,
1.,0.866025403784439,1.,0.866025403784439,1.,0.866025403784439,1.,0.866025403784439,
1.,0.866025403784439,1.,0.866025403784439,1.,0.866025403784439,1.,0.866025403784439,
1.,0.866025403784439,1.,0.866025403784439,1.,0.866025403784439,1.,0.866025403784439,
1.,0.866025403784439,1.,0.866025403784439,1.,0.866025403784439,1.,0.866025403784439,
1.,0.866025403784439,1.,0.866025403784439,1.,0.866025403784439,1.,0.866025403784439,
1.,0.866025403784439,1.,0.866025403784439,1.,0.866025403784439,1.,0.866025403784439,
1.,0.866025403784439,1.,0.866025403784439,1.,0.866025403784439,1.,0.866025403784439,
1.,0.866025403784439,1.,0.866025403784439,1.,0.866025403784439,1.,0.866025403784439,
1.,0.866025403784439,1.,0.866025403784439,1.,0.939534597205461,0.933647674785266))
REPRESENTATION_ITEM('')
);
#197=(
BOUNDED_CURVE()
B_SPLINE_CURVE(2,(#21385,#21386,#21387,#21388,#21389,#21390,#21391,#21392,
#21393,#21394,#21395,#21396,#21397,#21398,#21399,#21400,#21401,#21402,#21403,
#21404,#21405,#21406,#21407,#21408,#21409,#21410,#21411,#21412,#21413,#21414,
#21415,#21416,#21417,#21418,#21419,#21420,#21421,#21422,#21423,#21424,#21425,
#21426,#21427,#21428,#21429,#21430,#21431,#21432,#21433,#21434,#21435,#21436,
#21437,#21438,#21439,#21440,#21441,#21442,#21443,#21444,#21445,#21446,#21447,
#21448,#21449,#21450,#21451,#21452,#21453,#21454,#21455,#21456,#21457,#21458,
#21459,#21460,#21461,#21462,#21463,#21464,#21465,#21466,#21467,#21468,#21469,
#21470,#21471,#21472,#21473,#21474,#21475,#21476,#21477,#21478,#21479,#21480,
#21481,#21482,#21483,#21484,#21485,#21486,#21487,#21488,#21489,#21490,#21491,
#21492,#21493,#21494,#21495,#21496,#21497,#21498,#21499,#21500,#21501,#21502,
#21503,#21504,#21505,#21506,#21507,#21508,#21509,#21510,#21511,#21512,#21513,
#21514,#21515,#21516,#21517,#21518,#21519,#21520,#21521,#21522,#21523,#21524,
#21525,#21526,#21527,#21528,#21529,#21530,#21531,#21532,#21533,#21534,#21535,
#21536,#21537,#21538,#21539,#21540,#21541,#21542,#21543,#21544,#21545,#21546,
#21547,#21548,#21549,#21550,#21551,#21552,#21553,#21554,#21555,#21556,#21557,
#21558,#21559,#21560,#21561,#21562,#21563,#21564,#21565,#21566,#21567,#21568,
#21569,#21570,#21571,#21572,#21573,#21574,#21575,#21576,#21577,#21578,#21579,
#21580,#21581,#21582,#21583,#21584,#21585,#21586,#21587,#21588,#21589,#21590,
#21591,#21592,#21593,#21594,#21595,#21596,#21597,#21598,#21599,#21600,#21601,
#21602,#21603,#21604,#21605,#21606,#21607,#21608,#21609,#21610,#21611,#21612,
#21613,#21614,#21615,#21616,#21617,#21618,#21619,#21620,#21621,#21622,#21623,
#21624,#21625,#21626,#21627,#21628,#21629,#21630,#21631,#21632,#21633,#21634,
#21635,#21636,#21637,#21638,#21639,#21640,#21641,#21642,#21643,#21644,#21645,
#21646,#21647,#21648,#21649,#21650,#21651,#21652,#21653,#21654,#21655,#21656,
#21657),.UNSPECIFIED.,.F.,.F.)
B_SPLINE_CURVE_WITH_KNOTS((3,2,2,2,2,2,2,2,2,2,2,2,2,2,2,2,2,2,2,2,2,2,
2,2,2,2,2,2,2,2,2,2,2,2,2,2,2,2,2,2,2,2,2,2,2,2,2,2,2,2,2,2,2,2,2,2,2,2,
2,2,2,2,2,2,2,2,2,2,2,2,2,2,2,2,2,2,2,2,2,2,2,2,2,2,2,2,2,2,2,2,2,2,2,2,
2,2,2,2,2,2,2,2,2,2,2,2,2,2,2,2,2,2,2,2,2,2,2,2,2,2,2,2,2,2,2,2,2,2,2,2,
2,2,2,2,2,2,3),(0.697234701114643,0.697530864197531,0.699588477366255,0.701646090534979,
0.703703703703704,0.705761316872428,0.707818930041152,0.709876543209877,
0.711934156378601,0.713991769547325,0.716049382716049,0.718106995884774,
0.720164609053498,0.722222222222222,0.724279835390947,0.726337448559671,
0.728395061728395,0.730452674897119,0.732510288065844,0.734567901234568,
0.736625514403292,0.738683127572016,0.740740740740741,0.742798353909465,
0.744855967078189,0.746913580246914,0.748971193415638,0.751028806584362,
0.753086419753086,0.755144032921811,0.757201646090535,0.759259259259259,
0.761316872427984,0.763374485596708,0.765432098765432,0.767489711934156,
0.769547325102881,0.771604938271605,0.773662551440329,0.775720164609053,
0.777777777777778,0.779835390946502,0.781893004115226,0.783950617283951,
0.786008230452675,0.788065843621399,0.790123456790123,0.792181069958848,
0.794238683127572,0.796296296296296,0.798353909465021,0.800411522633745,
0.802469135802469,0.804526748971193,0.806584362139918,0.808641975308642,
0.810699588477366,0.812757201646091,0.814814814814815,0.816872427983539,
0.818930041152263,0.820987654320988,0.823045267489712,0.825102880658436,
0.827160493827161,0.829218106995885,0.831275720164609,0.833333333333333,
0.835390946502058,0.837448559670782,0.839506172839506,0.84156378600823,
0.843621399176955,0.845679012345679,0.847736625514403,0.849794238683128,
0.851851851851852,0.853909465020576,0.8559670781893,0.858024691358025,0.860082304526749,
0.862139917695473,0.864197530864197,0.866255144032922,0.868312757201646,
0.87037037037037,0.872427983539095,0.874485596707819,0.876543209876543,
0.878600823045268,0.880658436213992,0.882716049382716,0.88477366255144,
0.886831275720165,0.888888888888889,0.890946502057613,0.893004115226337,
0.895061728395062,0.897119341563786,0.89917695473251,0.901234567901235,
0.903292181069959,0.905349794238683,0.907407407407407,0.909465020576132,
0.911522633744856,0.91358024691358,0.915637860082305,0.917695473251029,
0.919753086419753,0.921810699588477,0.923868312757202,0.925925925925926,
0.92798353909465,0.930041152263374,0.932098765432099,0.934156378600823,
0.936213991769547,0.938271604938272,0.940329218106996,0.94238683127572,
0.944444444444444,0.946502057613169,0.948559670781893,0.950617283950617,
0.952674897119342,0.954732510288066,0.95679012345679,0.958847736625514,
0.960905349794239,0.962962962962963,0.965020576131687,0.967078189300412,
0.969135802469136,0.97119341563786,0.973251028806584,0.974693312758157),
 .UNSPECIFIED.)
CURVE()
GEOMETRIC_REPRESENTATION_ITEM()
RATIONAL_B_SPLINE_CURVE((0.966983863280644,0.980716331890302,1.,0.866025403784439,
1.,0.866025403784439,1.,0.866025403784439,1.,0.866025403784439,1.,0.866025403784439,
1.,0.866025403784439,1.,0.866025403784439,1.,0.866025403784439,1.,0.866025403784439,
1.,0.866025403784439,1.,0.866025403784439,1.,0.866025403784439,1.,0.866025403784439,
1.,0.866025403784439,1.,0.866025403784439,1.,0.866025403784439,1.,0.866025403784439,
1.,0.866025403784439,1.,0.866025403784439,1.,0.866025403784439,1.,0.866025403784439,
1.,0.866025403784439,1.,0.866025403784439,1.,0.866025403784439,1.,0.866025403784439,
1.,0.866025403784439,1.,0.866025403784439,1.,0.866025403784439,1.,0.866025403784439,
1.,0.866025403784439,1.,0.866025403784439,1.,0.866025403784439,1.,0.866025403784439,
1.,0.866025403784439,1.,0.866025403784439,1.,0.866025403784439,1.,0.866025403784439,
1.,0.866025403784439,1.,0.866025403784439,1.,0.866025403784439,1.,0.866025403784439,
1.,0.866025403784439,1.,0.866025403784439,1.,0.866025403784439,1.,0.866025403784439,
1.,0.866025403784439,1.,0.866025403784439,1.,0.866025403784439,1.,0.866025403784439,
1.,0.866025403784439,1.,0.866025403784439,1.,0.866025403784439,1.,0.866025403784439,
1.,0.866025403784439,1.,0.866025403784439,1.,0.866025403784439,1.,0.866025403784439,
1.,0.866025403784439,1.,0.866025403784439,1.,0.866025403784439,1.,0.866025403784439,
1.,0.866025403784439,1.,0.866025403784439,1.,0.866025403784439,1.,0.866025403784439,
1.,0.866025403784439,1.,0.866025403784439,1.,0.866025403784439,1.,0.866025403784439,
1.,0.866025403784439,1.,0.866025403784439,1.,0.866025403784439,1.,0.866025403784439,
1.,0.866025403784439,1.,0.866025403784439,1.,0.866025403784439,1.,0.866025403784439,
1.,0.866025403784439,1.,0.866025403784439,1.,0.866025403784439,1.,0.866025403784439,
1.,0.866025403784439,1.,0.866025403784439,1.,0.866025403784439,1.,0.866025403784439,
1.,0.866025403784439,1.,0.866025403784439,1.,0.866025403784439,1.,0.866025403784439,
1.,0.866025403784439,1.,0.866025403784439,1.,0.866025403784439,1.,0.866025403784439,
1.,0.866025403784439,1.,0.866025403784439,1.,0.866025403784439,1.,0.866025403784439,
1.,0.866025403784439,1.,0.866025403784439,1.,0.866025403784439,1.,0.866025403784439,
1.,0.866025403784439,1.,0.866025403784439,1.,0.866025403784439,1.,0.866025403784439,
1.,0.866025403784439,1.,0.866025403784439,1.,0.866025403784439,1.,0.866025403784439,
1.,0.866025403784439,1.,0.866025403784439,1.,0.866025403784439,1.,0.866025403784439,
1.,0.866025403784439,1.,0.866025403784439,1.,0.866025403784439,1.,0.866025403784439,
1.,0.866025403784439,1.,0.866025403784439,1.,0.866025403784439,1.,0.866025403784439,
1.,0.866025403784439,1.,0.866025403784439,1.,0.866025403784439,1.,0.866025403784439,
1.,0.866025403784439,1.,0.866025403784439,1.,0.866025403784439,1.,0.866025403784439,
1.,0.866025403784439,1.,0.866025403784439,1.,0.866025403784439,1.,0.866025403784439,
1.,0.866025403784439,1.,0.906090506720528,0.94383273215671))
REPRESENTATION_ITEM('')
);
#249=PLANE('',#6475);
#250=PLANE('',#6482);
#251=PLANE('',#6483);
#252=PLANE('',#6484);
#253=PLANE('',#6485);
#254=PLANE('',#6486);
#255=PLANE('',#6487);
#256=PLANE('',#6488);
#257=PLANE('',#6491);
#258=PLANE('',#6493);
#259=PLANE('',#6495);
#260=PLANE('',#6500);
#261=PLANE('',#6504);
#262=PLANE('',#6505);
#263=PLANE('',#6510);
#264=PLANE('',#6512);
#265=PLANE('',#6517);
#266=PLANE('',#6521);
#267=PLANE('',#6522);
#268=PLANE('',#6526);
#269=PLANE('',#6528);
#270=PLANE('',#6530);
#271=PLANE('',#6534);
#272=PLANE('',#6538);
#273=PLANE('',#6539);
#274=PLANE('',#6545);
#275=PLANE('',#6562);
#276=PLANE('',#6563);
#335=FACE_BOUND('',#921,.T.);
#336=FACE_BOUND('',#922,.T.);
#337=FACE_BOUND('',#924,.T.);
#338=FACE_BOUND('',#932,.T.);
#339=FACE_BOUND('',#935,.T.);
#340=FACE_BOUND('',#937,.T.);
#341=FACE_BOUND('',#945,.T.);
#342=FACE_BOUND('',#953,.T.);
#343=FACE_BOUND('',#955,.T.);
#344=FACE_BOUND('',#963,.T.);
#345=FACE_BOUND('',#979,.T.);
#369=CONICAL_SURFACE('',#6448,8.326,0.785398163397447);
#370=CONICAL_SURFACE('',#6490,8.82600000000001,0.785398163397447);
#371=CONICAL_SURFACE('',#6570,10.9985226280624,1.0471975511966);
#372=CONICAL_SURFACE('',#6571,10.9985226280624,1.0471975511966);
#373=CONICAL_SURFACE('',#6572,10.9985226280624,1.0471975511966);
#374=CONICAL_SURFACE('',#6573,10.9985226280624,1.0471975511966);
#375=CONICAL_SURFACE('',#6574,10.9985226280624,1.0471975511966);
#376=CONICAL_SURFACE('',#6575,10.9985226280624,1.0471975511966);
#454=ELLIPSE('',#6439,5.07947085861221,5.00000000004167);
#455=ELLIPSE('',#6446,5.07947085864035,5.00000000005631);
#456=ELLIPSE('',#6492,155.887927744283,31.9541505812655);
#457=ELLIPSE('',#6494,155.887927068924,31.9541505120991);
#458=ELLIPSE('',#6511,155.887927258897,31.9541505315509);
#459=ELLIPSE('',#6527,155.887927546699,31.9541505609938);
#460=ELLIPSE('',#6529,155.887927788136,31.9541505857567);
#461=ELLIPSE('',#6546,155.887926302679,31.9541504336181);
#463=TOROIDAL_SURFACE('',#6422,18.05,1.);
#464=TOROIDAL_SURFACE('',#6427,18.05,1.);
#465=TOROIDAL_SURFACE('',#6432,4.,1.);
#466=TOROIDAL_SURFACE('',#6450,19.55,0.5);
#467=TOROIDAL_SURFACE('',#6453,19.55,0.5);
#468=TOROIDAL_SURFACE('',#6457,19.55,0.5);
#469=TOROIDAL_SURFACE('',#6559,19.55,0.5);
#470=TOROIDAL_SURFACE('',#6560,19.55,0.5);
#471=TOROIDAL_SURFACE('',#6561,19.55,0.5);
#472=TOROIDAL_SURFACE('',#6588,3.,1.);
#473=TOROIDAL_SURFACE('',#6595,3.,1.);
#474=TOROIDAL_SURFACE('',#6597,3.,1.);
#475=TOROIDAL_SURFACE('',#6603,3.,1.);
#476=TOROIDAL_SURFACE('',#6605,3.,1.);
#477=TOROIDAL_SURFACE('',#6611,3.,1.);
#478=TOROIDAL_SURFACE('',#6657,7.35,1.);
#479=TOROIDAL_SURFACE('',#6661,4.,1.);
#480=TOROIDAL_SURFACE('',#6665,4.,1.);
#481=TOROIDAL_SURFACE('',#6669,7.35,1.);
#482=TOROIDAL_SURFACE('',#6672,7.35,1.);
#483=TOROIDAL_SURFACE('',#6676,4.,1.);
#484=TOROIDAL_SURFACE('',#6680,4.,1.);
#485=TOROIDAL_SURFACE('',#6684,7.35,1.);
#486=TOROIDAL_SURFACE('',#6687,7.35,1.);
#487=TOROIDAL_SURFACE('',#6692,4.,1.);
#488=TOROIDAL_SURFACE('',#6696,7.35,1.);
#500=FACE_OUTER_BOUND('',#883,.T.);
#501=FACE_OUTER_BOUND('',#884,.T.);
#502=FACE_OUTER_BOUND('',#885,.T.);
#503=FACE_OUTER_BOUND('',#886,.T.);
#504=FACE_OUTER_BOUND('',#887,.T.);
#505=FACE_OUTER_BOUND('',#888,.T.);
#506=FACE_OUTER_BOUND('',#889,.T.);
#507=FACE_OUTER_BOUND('',#890,.T.);
#508=FACE_OUTER_BOUND('',#891,.T.);
#509=FACE_OUTER_BOUND('',#892,.T.);
#510=FACE_OUTER_BOUND('',#893,.T.);
#511=FACE_OUTER_BOUND('',#894,.T.);
#512=FACE_OUTER_BOUND('',#895,.T.);
#513=FACE_OUTER_BOUND('',#896,.T.);
#514=FACE_OUTER_BOUND('',#897,.T.);
#515=FACE_OUTER_BOUND('',#898,.T.);
#516=FACE_OUTER_BOUND('',#899,.T.);
#517=FACE_OUTER_BOUND('',#900,.T.);
#518=FACE_OUTER_BOUND('',#901,.T.);
#519=FACE_OUTER_BOUND('',#902,.T.);
#520=FACE_OUTER_BOUND('',#903,.T.);
#521=FACE_OUTER_BOUND('',#904,.T.);
#522=FACE_OUTER_BOUND('',#905,.T.);
#523=FACE_OUTER_BOUND('',#906,.T.);
#524=FACE_OUTER_BOUND('',#907,.T.);
#525=FACE_OUTER_BOUND('',#908,.T.);
#526=FACE_OUTER_BOUND('',#909,.T.);
#527=FACE_OUTER_BOUND('',#910,.T.);
#528=FACE_OUTER_BOUND('',#911,.T.);
#529=FACE_OUTER_BOUND('',#912,.T.);
#530=FACE_OUTER_BOUND('',#913,.T.);
#531=FACE_OUTER_BOUND('',#914,.T.);
#532=FACE_OUTER_BOUND('',#915,.T.);
#533=FACE_OUTER_BOUND('',#916,.T.);
#534=FACE_OUTER_BOUND('',#917,.T.);
#535=FACE_OUTER_BOUND('',#918,.T.);
#536=FACE_OUTER_BOUND('',#919,.T.);
#537=FACE_OUTER_BOUND('',#920,.T.);
#538=FACE_OUTER_BOUND('',#923,.T.);
#539=FACE_OUTER_BOUND('',#925,.T.);
#540=FACE_OUTER_BOUND('',#926,.T.);
#541=FACE_OUTER_BOUND('',#927,.T.);
#542=FACE_OUTER_BOUND('',#928,.T.);
#543=FACE_OUTER_BOUND('',#929,.T.);
#544=FACE_OUTER_BOUND('',#930,.T.);
#545=FACE_OUTER_BOUND('',#931,.T.);
#546=FACE_OUTER_BOUND('',#933,.T.);
#547=FACE_OUTER_BOUND('',#934,.T.);
#548=FACE_OUTER_BOUND('',#936,.T.);
#549=FACE_OUTER_BOUND('',#938,.T.);
#550=FACE_OUTER_BOUND('',#939,.T.);
#551=FACE_OUTER_BOUND('',#940,.T.);
#552=FACE_OUTER_BOUND('',#941,.T.);
#553=FACE_OUTER_BOUND('',#942,.T.);
#554=FACE_OUTER_BOUND('',#943,.T.);
#555=FACE_OUTER_BOUND('',#944,.T.);
#556=FACE_OUTER_BOUND('',#946,.T.);
#557=FACE_OUTER_BOUND('',#947,.T.);
#558=FACE_OUTER_BOUND('',#948,.T.);
#559=FACE_OUTER_BOUND('',#949,.T.);
#560=FACE_OUTER_BOUND('',#950,.T.);
#561=FACE_OUTER_BOUND('',#951,.T.);
#562=FACE_OUTER_BOUND('',#952,.T.);
#563=FACE_OUTER_BOUND('',#954,.T.);
#564=FACE_OUTER_BOUND('',#956,.T.);
#565=FACE_OUTER_BOUND('',#957,.T.);
#566=FACE_OUTER_BOUND('',#958,.T.);
#567=FACE_OUTER_BOUND('',#959,.T.);
#568=FACE_OUTER_BOUND('',#960,.T.);
#569=FACE_OUTER_BOUND('',#961,.T.);
#570=FACE_OUTER_BOUND('',#962,.T.);
#571=FACE_OUTER_BOUND('',#964,.T.);
#572=FACE_OUTER_BOUND('',#965,.T.);
#573=FACE_OUTER_BOUND('',#966,.T.);
#574=FACE_OUTER_BOUND('',#967,.T.);
#575=FACE_OUTER_BOUND('',#968,.T.);
#576=FACE_OUTER_BOUND('',#969,.T.);
#577=FACE_OUTER_BOUND('',#970,.T.);
#578=FACE_OUTER_BOUND('',#971,.T.);
#579=FACE_OUTER_BOUND('',#972,.T.);
#580=FACE_OUTER_BOUND('',#973,.T.);
#581=FACE_OUTER_BOUND('',#974,.T.);
#582=FACE_OUTER_BOUND('',#975,.T.);
#583=FACE_OUTER_BOUND('',#976,.T.);
#584=FACE_OUTER_BOUND('',#977,.T.);
#585=FACE_OUTER_BOUND('',#978,.T.);
#586=FACE_OUTER_BOUND('',#980,.T.);
#587=FACE_OUTER_BOUND('',#981,.T.);
#588=FACE_OUTER_BOUND('',#982,.T.);
#589=FACE_OUTER_BOUND('',#983,.T.);
#590=FACE_OUTER_BOUND('',#984,.T.);
#591=FACE_OUTER_BOUND('',#985,.T.);
#592=FACE_OUTER_BOUND('',#986,.T.);
#593=FACE_OUTER_BOUND('',#987,.T.);
#594=FACE_OUTER_BOUND('',#988,.T.);
#595=FACE_OUTER_BOUND('',#989,.T.);
#596=FACE_OUTER_BOUND('',#990,.T.);
#597=FACE_OUTER_BOUND('',#991,.T.);
#598=FACE_OUTER_BOUND('',#992,.T.);
#599=FACE_OUTER_BOUND('',#993,.T.);
#600=FACE_OUTER_BOUND('',#994,.T.);
#601=FACE_OUTER_BOUND('',#995,.T.);
#602=FACE_OUTER_BOUND('',#996,.T.);
#603=FACE_OUTER_BOUND('',#997,.T.);
#604=FACE_OUTER_BOUND('',#998,.T.);
#605=FACE_OUTER_BOUND('',#999,.T.);
#606=FACE_OUTER_BOUND('',#1000,.T.);
#607=FACE_OUTER_BOUND('',#1001,.T.);
#608=FACE_OUTER_BOUND('',#1002,.T.);
#609=FACE_OUTER_BOUND('',#1003,.T.);
#610=FACE_OUTER_BOUND('',#1004,.T.);
#611=FACE_OUTER_BOUND('',#1005,.T.);
#612=FACE_OUTER_BOUND('',#1006,.T.);
#613=FACE_OUTER_BOUND('',#1007,.T.);
#614=FACE_OUTER_BOUND('',#1008,.T.);
#615=FACE_OUTER_BOUND('',#1009,.T.);
#616=FACE_OUTER_BOUND('',#1010,.T.);
#617=FACE_OUTER_BOUND('',#1011,.T.);
#618=FACE_OUTER_BOUND('',#1012,.T.);
#619=FACE_OUTER_BOUND('',#1013,.T.);
#620=FACE_OUTER_BOUND('',#1014,.T.);
#621=FACE_OUTER_BOUND('',#1015,.T.);
#622=FACE_OUTER_BOUND('',#1016,.T.);
#623=FACE_OUTER_BOUND('',#1017,.T.);
#624=FACE_OUTER_BOUND('',#1018,.T.);
#625=FACE_OUTER_BOUND('',#1019,.T.);
#626=FACE_OUTER_BOUND('',#1020,.T.);
#627=FACE_OUTER_BOUND('',#1021,.T.);
#628=FACE_OUTER_BOUND('',#1022,.T.);
#629=FACE_OUTER_BOUND('',#1023,.T.);
#630=FACE_OUTER_BOUND('',#1024,.T.);
#631=FACE_OUTER_BOUND('',#1025,.T.);
#632=FACE_OUTER_BOUND('',#1026,.T.);
#633=FACE_OUTER_BOUND('',#1027,.T.);
#634=FACE_OUTER_BOUND('',#1028,.T.);
#635=FACE_OUTER_BOUND('',#1029,.T.);
#636=FACE_OUTER_BOUND('',#1030,.T.);
#637=FACE_OUTER_BOUND('',#1031,.T.);
#638=FACE_OUTER_BOUND('',#1032,.T.);
#639=FACE_OUTER_BOUND('',#1033,.T.);
#640=FACE_OUTER_BOUND('',#1034,.T.);
#641=FACE_OUTER_BOUND('',#1035,.T.);
#642=FACE_OUTER_BOUND('',#1036,.T.);
#643=FACE_OUTER_BOUND('',#1037,.T.);
#644=FACE_OUTER_BOUND('',#1038,.T.);
#645=FACE_OUTER_BOUND('',#1039,.T.);
#646=FACE_OUTER_BOUND('',#1040,.T.);
#647=FACE_OUTER_BOUND('',#1041,.T.);
#648=FACE_OUTER_BOUND('',#1042,.T.);
#649=FACE_OUTER_BOUND('',#1043,.T.);
#650=FACE_OUTER_BOUND('',#1044,.T.);
#651=FACE_OUTER_BOUND('',#1045,.T.);
#652=FACE_OUTER_BOUND('',#1046,.T.);
#653=FACE_OUTER_BOUND('',#1047,.T.);
#654=FACE_OUTER_BOUND('',#1048,.T.);
#655=FACE_OUTER_BOUND('',#1049,.T.);
#656=FACE_OUTER_BOUND('',#1050,.T.);
#657=FACE_OUTER_BOUND('',#1051,.T.);
#658=FACE_OUTER_BOUND('',#1052,.T.);
#659=FACE_OUTER_BOUND('',#1053,.T.);
#660=FACE_OUTER_BOUND('',#1054,.T.);
#661=FACE_OUTER_BOUND('',#1055,.T.);
#662=FACE_OUTER_BOUND('',#1056,.T.);
#663=FACE_OUTER_BOUND('',#1057,.T.);
#664=FACE_OUTER_BOUND('',#1058,.T.);
#665=FACE_OUTER_BOUND('',#1059,.T.);
#666=FACE_OUTER_BOUND('',#1060,.T.);
#667=FACE_OUTER_BOUND('',#1061,.T.);
#668=FACE_OUTER_BOUND('',#1062,.T.);
#669=FACE_OUTER_BOUND('',#1063,.T.);
#670=FACE_OUTER_BOUND('',#1064,.T.);
#671=FACE_OUTER_BOUND('',#1065,.T.);
#672=FACE_OUTER_BOUND('',#1066,.T.);
#673=FACE_OUTER_BOUND('',#1067,.T.);
#883=EDGE_LOOP('',(#3944,#3945,#3946,#3947,#3948,#3949,#3950,#3951));
#884=EDGE_LOOP('',(#3952,#3953,#3954,#3955));
#885=EDGE_LOOP('',(#3956,#3957,#3958,#3959));
#886=EDGE_LOOP('',(#3960,#3961,#3962,#3963));
#887=EDGE_LOOP('',(#3964,#3965,#3966,#3967));
#888=EDGE_LOOP('',(#3968,#3969,#3970,#3971));
#889=EDGE_LOOP('',(#3972,#3973,#3974,#3975));
#890=EDGE_LOOP('',(#3976,#3977,#3978,#3979));
#891=EDGE_LOOP('',(#3980,#3981,#3982,#3983));
#892=EDGE_LOOP('',(#3984,#3985,#3986,#3987));
#893=EDGE_LOOP('',(#3988,#3989,#3990,#3991));
#894=EDGE_LOOP('',(#3992,#3993,#3994,#3995));
#895=EDGE_LOOP('',(#3996,#3997,#3998,#3999));
#896=EDGE_LOOP('',(#4000,#4001,#4002,#4003));
#897=EDGE_LOOP('',(#4004,#4005,#4006,#4007));
#898=EDGE_LOOP('',(#4008,#4009,#4010,#4011));
#899=EDGE_LOOP('',(#4012,#4013,#4014,#4015));
#900=EDGE_LOOP('',(#4016,#4017,#4018,#4019));
#901=EDGE_LOOP('',(#4020,#4021,#4022,#4023));
#902=EDGE_LOOP('',(#4024,#4025,#4026,#4027));
#903=EDGE_LOOP('',(#4028,#4029,#4030,#4031));
#904=EDGE_LOOP('',(#4032,#4033,#4034,#4035));
#905=EDGE_LOOP('',(#4036,#4037,#4038,#4039,#4040));
#906=EDGE_LOOP('',(#4041,#4042,#4043,#4044,#4045));
#907=EDGE_LOOP('',(#4046,#4047,#4048,#4049));
#908=EDGE_LOOP('',(#4050,#4051,#4052,#4053,#4054));
#909=EDGE_LOOP('',(#4055,#4056,#4057,#4058));
#910=EDGE_LOOP('',(#4059,#4060,#4061,#4062));
#911=EDGE_LOOP('',(#4063,#4064,#4065,#4066,#4067));
#912=EDGE_LOOP('',(#4068,#4069,#4070,#4071));
#913=EDGE_LOOP('',(#4072,#4073,#4074,#4075,#4076,#4077,#4078));
#914=EDGE_LOOP('',(#4079,#4080,#4081,#4082,#4083));
#915=EDGE_LOOP('',(#4084,#4085,#4086,#4087));
#916=EDGE_LOOP('',(#4088,#4089,#4090,#4091));
#917=EDGE_LOOP('',(#4092,#4093,#4094,#4095));
#918=EDGE_LOOP('',(#4096,#4097,#4098,#4099));
#919=EDGE_LOOP('',(#4100,#4101,#4102,#4103));
#920=EDGE_LOOP('',(#4104,#4105,#4106,#4107,#4108,#4109,#4110,#4111,#4112,
#4113,#4114,#4115,#4116,#4117));
#921=EDGE_LOOP('',(#4118,#4119,#4120,#4121));
#922=EDGE_LOOP('',(#4122,#4123,#4124,#4125));
#923=EDGE_LOOP('',(#4126,#4127,#4128,#4129,#4130,#4131));
#924=EDGE_LOOP('',(#4132));
#925=EDGE_LOOP('',(#4133,#4134,#4135,#4136,#4137));
#926=EDGE_LOOP('',(#4138,#4139,#4140,#4141,#4142));
#927=EDGE_LOOP('',(#4143,#4144,#4145,#4146,#4147));
#928=EDGE_LOOP('',(#4148,#4149,#4150,#4151,#4152));
#929=EDGE_LOOP('',(#4153,#4154,#4155,#4156,#4157));
#930=EDGE_LOOP('',(#4158,#4159,#4160,#4161,#4162));
#931=EDGE_LOOP('',(#4163));
#932=EDGE_LOOP('',(#4164,#4165,#4166));
#933=EDGE_LOOP('',(#4167,#4168,#4169,#4170,#4171,#4172));
#934=EDGE_LOOP('',(#4173,#4174,#4175,#4176,#4177,#4178));
#935=EDGE_LOOP('',(#4179));
#936=EDGE_LOOP('',(#4180,#4181,#4182,#4183,#4184,#4185));
#937=EDGE_LOOP('',(#4186));
#938=EDGE_LOOP('',(#4187,#4188,#4189,#4190));
#939=EDGE_LOOP('',(#4191,#4192,#4193,#4194));
#940=EDGE_LOOP('',(#4195,#4196,#4197,#4198));
#941=EDGE_LOOP('',(#4199,#4200,#4201,#4202));
#942=EDGE_LOOP('',(#4203,#4204,#4205,#4206));
#943=EDGE_LOOP('',(#4207,#4208,#4209,#4210,#4211,#4212,#4213,#4214));
#944=EDGE_LOOP('',(#4215,#4216,#4217,#4218,#4219,#4220));
#945=EDGE_LOOP('',(#4221));
#946=EDGE_LOOP('',(#4222,#4223,#4224,#4225));
#947=EDGE_LOOP('',(#4226,#4227,#4228,#4229));
#948=EDGE_LOOP('',(#4230,#4231,#4232,#4233));
#949=EDGE_LOOP('',(#4234,#4235,#4236,#4237));
#950=EDGE_LOOP('',(#4238,#4239,#4240,#4241));
#951=EDGE_LOOP('',(#4242,#4243,#4244,#4245,#4246,#4247,#4248,#4249));
#952=EDGE_LOOP('',(#4250,#4251,#4252,#4253,#4254,#4255));
#953=EDGE_LOOP('',(#4256));
#954=EDGE_LOOP('',(#4257,#4258,#4259,#4260,#4261,#4262));
#955=EDGE_LOOP('',(#4263));
#956=EDGE_LOOP('',(#4264,#4265,#4266,#4267));
#957=EDGE_LOOP('',(#4268,#4269,#4270,#4271));
#958=EDGE_LOOP('',(#4272,#4273,#4274,#4275));
#959=EDGE_LOOP('',(#4276,#4277,#4278,#4279));
#960=EDGE_LOOP('',(#4280,#4281,#4282,#4283));
#961=EDGE_LOOP('',(#4284,#4285,#4286,#4287,#4288,#4289,#4290,#4291));
#962=EDGE_LOOP('',(#4292,#4293,#4294,#4295,#4296,#4297));
#963=EDGE_LOOP('',(#4298));
#964=EDGE_LOOP('',(#4299,#4300,#4301,#4302,#4303));
#965=EDGE_LOOP('',(#4304,#4305,#4306,#4307,#4308));
#966=EDGE_LOOP('',(#4309,#4310,#4311,#4312,#4313));
#967=EDGE_LOOP('',(#4314,#4315,#4316,#4317,#4318));
#968=EDGE_LOOP('',(#4319,#4320,#4321,#4322,#4323));
#969=EDGE_LOOP('',(#4324,#4325,#4326,#4327,#4328));
#970=EDGE_LOOP('',(#4329,#4330,#4331,#4332));
#971=EDGE_LOOP('',(#4333,#4334,#4335,#4336,#4337,#4338,#4339));
#972=EDGE_LOOP('',(#4340,#4341,#4342,#4343,#4344,#4345));
#973=EDGE_LOOP('',(#4346,#4347,#4348,#4349,#4350));
#974=EDGE_LOOP('',(#4351,#4352,#4353,#4354,#4355));
#975=EDGE_LOOP('',(#4356,#4357,#4358,#4359,#4360,#4361,#4362,#4363,#4364,
#4365,#4366,#4367,#4368,#4369,#4370,#4371,#4372,#4373,#4374,#4375,#4376,
#4377,#4378,#4379,#4380,#4381,#4382));
#976=EDGE_LOOP('',(#4383,#4384,#4385,#4386,#4387));
#977=EDGE_LOOP('',(#4388,#4389,#4390,#4391,#4392,#4393,#4394,#4395,#4396,
#4397,#4398,#4399,#4400,#4401,#4402,#4403,#4404,#4405,#4406,#4407,#4408,
#4409,#4410,#4411,#4412,#4413));
#978=EDGE_LOOP('',(#4414));
#979=EDGE_LOOP('',(#4415,#4416,#4417,#4418,#4419,#4420,#4421,#4422,#4423,
#4424,#4425,#4426));
#980=EDGE_LOOP('',(#4427,#4428,#4429,#4430));
#981=EDGE_LOOP('',(#4431,#4432,#4433,#4434));
#982=EDGE_LOOP('',(#4435,#4436,#4437,#4438));
#983=EDGE_LOOP('',(#4439,#4440,#4441,#4442));
#984=EDGE_LOOP('',(#4443,#4444,#4445,#4446));
#985=EDGE_LOOP('',(#4447,#4448,#4449,#4450));
#986=EDGE_LOOP('',(#4451,#4452,#4453,#4454));
#987=EDGE_LOOP('',(#4455,#4456,#4457,#4458));
#988=EDGE_LOOP('',(#4459,#4460,#4461,#4462));
#989=EDGE_LOOP('',(#4463,#4464,#4465,#4466));
#990=EDGE_LOOP('',(#4467,#4468,#4469,#4470));
#991=EDGE_LOOP('',(#4471,#4472,#4473,#4474));
#992=EDGE_LOOP('',(#4475,#4476,#4477,#4478));
#993=EDGE_LOOP('',(#4479,#4480,#4481,#4482));
#994=EDGE_LOOP('',(#4483,#4484,#4485,#4486));
#995=EDGE_LOOP('',(#4487,#4488,#4489,#4490));
#996=EDGE_LOOP('',(#4491,#4492,#4493,#4494));
#997=EDGE_LOOP('',(#4495,#4496,#4497,#4498));
#998=EDGE_LOOP('',(#4499,#4500,#4501,#4502));
#999=EDGE_LOOP('',(#4503,#4504,#4505,#4506));
#1000=EDGE_LOOP('',(#4507,#4508,#4509,#4510));
#1001=EDGE_LOOP('',(#4511,#4512,#4513,#4514));
#1002=EDGE_LOOP('',(#4515,#4516,#4517,#4518));
#1003=EDGE_LOOP('',(#4519,#4520,#4521,#4522));
#1004=EDGE_LOOP('',(#4523,#4524,#4525,#4526));
#1005=EDGE_LOOP('',(#4527,#4528,#4529));
#1006=EDGE_LOOP('',(#4530,#4531,#4532,#4533));
#1007=EDGE_LOOP('',(#4534,#4535,#4536));
#1008=EDGE_LOOP('',(#4537,#4538,#4539,#4540));
#1009=EDGE_LOOP('',(#4541,#4542,#4543,#4544));
#1010=EDGE_LOOP('',(#4545,#4546,#4547));
#1011=EDGE_LOOP('',(#4548,#4549,#4550,#4551));
#1012=EDGE_LOOP('',(#4552,#4553,#4554));
#1013=EDGE_LOOP('',(#4555,#4556,#4557,#4558));
#1014=EDGE_LOOP('',(#4559,#4560,#4561));
#1015=EDGE_LOOP('',(#4562,#4563,#4564,#4565));
#1016=EDGE_LOOP('',(#4566,#4567,#4568,#4569));
#1017=EDGE_LOOP('',(#4570,#4571,#4572));
#1018=EDGE_LOOP('',(#4573,#4574,#4575,#4576));
#1019=EDGE_LOOP('',(#4577,#4578,#4579));
#1020=EDGE_LOOP('',(#4580,#4581,#4582,#4583));
#1021=EDGE_LOOP('',(#4584,#4585,#4586));
#1022=EDGE_LOOP('',(#4587,#4588,#4589,#4590));
#1023=EDGE_LOOP('',(#4591,#4592,#4593,#4594));
#1024=EDGE_LOOP('',(#4595,#4596,#4597));
#1025=EDGE_LOOP('',(#4598,#4599,#4600,#4601));
#1026=EDGE_LOOP('',(#4602,#4603,#4604,#4605));
#1027=EDGE_LOOP('',(#4606,#4607,#4608,#4609));
#1028=EDGE_LOOP('',(#4610,#4611,#4612,#4613));
#1029=EDGE_LOOP('',(#4614,#4615,#4616));
#1030=EDGE_LOOP('',(#4617,#4618,#4619));
#1031=EDGE_LOOP('',(#4620,#4621,#4622,#4623));
#1032=EDGE_LOOP('',(#4624,#4625,#4626,#4627));
#1033=EDGE_LOOP('',(#4628,#4629,#4630,#4631));
#1034=EDGE_LOOP('',(#4632,#4633,#4634));
#1035=EDGE_LOOP('',(#4635,#4636,#4637));
#1036=EDGE_LOOP('',(#4638,#4639,#4640,#4641));
#1037=EDGE_LOOP('',(#4642,#4643,#4644,#4645));
#1038=EDGE_LOOP('',(#4646,#4647,#4648));
#1039=EDGE_LOOP('',(#4649,#4650,#4651,#4652));
#1040=EDGE_LOOP('',(#4653,#4654,#4655));
#1041=EDGE_LOOP('',(#4656,#4657,#4658,#4659));
#1042=EDGE_LOOP('',(#4660,#4661,#4662));
#1043=EDGE_LOOP('',(#4663,#4664,#4665,#4666));
#1044=EDGE_LOOP('',(#4667,#4668,#4669,#4670));
#1045=EDGE_LOOP('',(#4671,#4672,#4673,#4674));
#1046=EDGE_LOOP('',(#4675,#4676,#4677,#4678));
#1047=EDGE_LOOP('',(#4679,#4680,#4681,#4682));
#1048=EDGE_LOOP('',(#4683,#4684,#4685,#4686));
#1049=EDGE_LOOP('',(#4687,#4688,#4689,#4690));
#1050=EDGE_LOOP('',(#4691,#4692,#4693));
#1051=EDGE_LOOP('',(#4694,#4695,#4696));
#1052=EDGE_LOOP('',(#4697,#4698,#4699,#4700));
#1053=EDGE_LOOP('',(#4701,#4702,#4703,#4704));
#1054=EDGE_LOOP('',(#4705,#4706,#4707,#4708));
#1055=EDGE_LOOP('',(#4709,#4710,#4711,#4712));
#1056=EDGE_LOOP('',(#4713,#4714,#4715,#4716));
#1057=EDGE_LOOP('',(#4717,#4718,#4719,#4720));
#1058=EDGE_LOOP('',(#4721,#4722,#4723,#4724));
#1059=EDGE_LOOP('',(#4725,#4726,#4727));
#1060=EDGE_LOOP('',(#4728,#4729,#4730));
#1061=EDGE_LOOP('',(#4731,#4732,#4733,#4734));
#1062=EDGE_LOOP('',(#4735,#4736,#4737,#4738));
#1063=EDGE_LOOP('',(#4739,#4740,#4741,#4742));
#1064=EDGE_LOOP('',(#4743,#4744,#4745,#4746));
#1065=EDGE_LOOP('',(#4747,#4748,#4749,#4750));
#1066=EDGE_LOOP('',(#4751,#4752,#4753,#4754));
#1067=EDGE_LOOP('',(#4755,#4756,#4757));
#1300=CIRCLE('',#6398,8.326);
#1301=CIRCLE('',#6399,8.326);
#1302=CIRCLE('',#6421,8.326);
#1303=CIRCLE('',#6423,19.05);
#1304=CIRCLE('',#6424,19.05);
#1305=CIRCLE('',#6425,1.);
#1306=CIRCLE('',#6426,18.05);
#1307=CIRCLE('',#6428,18.05);
#1308=CIRCLE('',#6429,1.);
#1309=CIRCLE('',#6430,19.05);
#1310=CIRCLE('',#6431,19.05);
#1311=CIRCLE('',#6433,4.);
#1312=CIRCLE('',#6434,0.999999999999999);
#1313=CIRCLE('',#6435,5.);
#1314=CIRCLE('',#6436,1.);
#1315=CIRCLE('',#6438,5.);
#1316=CIRCLE('',#6441,5.);
#1317=CIRCLE('',#6443,5.);
#1318=CIRCLE('',#6444,5.);
#1319=CIRCLE('',#6447,5.);
#1320=CIRCLE('',#6449,8.82600000000003);
#1321=CIRCLE('',#6451,19.05);
#1322=CIRCLE('',#6452,19.55);
#1323=CIRCLE('',#6454,19.55);
#1324=CIRCLE('',#6455,19.05);
#1325=CIRCLE('',#6456,19.05);
#1326=CIRCLE('',#6458,19.55);
#1327=CIRCLE('',#6459,19.05);
#1328=CIRCLE('',#6462,3.2);
#1329=CIRCLE('',#6463,3.2);
#1330=CIRCLE('',#6465,3.2);
#1331=CIRCLE('',#6466,3.2);
#1332=CIRCLE('',#6468,3.2);
#1333=CIRCLE('',#6469,3.2);
#1334=CIRCLE('',#6471,19.05);
#1335=CIRCLE('',#6472,19.05);
#1336=CIRCLE('',#6473,19.05);
#1337=CIRCLE('',#6474,19.05);
#1338=CIRCLE('',#6476,10.9985226280624);
#1339=CIRCLE('',#6477,10.9985226280624);
#1340=CIRCLE('',#6478,10.9985226280624);
#1341=CIRCLE('',#6479,10.9985226280624);
#1342=CIRCLE('',#6480,10.9985226280624);
#1343=CIRCLE('',#6481,10.9985226280624);
#1344=CIRCLE('',#6489,8.82600000000001);
#1345=CIRCLE('',#6496,19.55);
#1346=CIRCLE('',#6498,3.);
#1347=CIRCLE('',#6499,3.);
#1348=CIRCLE('',#6502,5.);
#1349=CIRCLE('',#6503,5.);
#1350=CIRCLE('',#6506,7.35);
#1351=CIRCLE('',#6507,4.);
#1352=CIRCLE('',#6508,4.);
#1353=CIRCLE('',#6509,7.35);
#1354=CIRCLE('',#6513,19.55);
#1355=CIRCLE('',#6515,3.);
#1356=CIRCLE('',#6516,3.);
#1357=CIRCLE('',#6519,5.);
#1358=CIRCLE('',#6520,5.);
#1359=CIRCLE('',#6523,7.35);
#1360=CIRCLE('',#6524,4.);
#1361=CIRCLE('',#6525,7.35);
#1362=CIRCLE('',#6532,3.);
#1363=CIRCLE('',#6533,3.);
#1364=CIRCLE('',#6536,5.);
#1365=CIRCLE('',#6537,5.);
#1366=CIRCLE('',#6540,19.55);
#1367=CIRCLE('',#6541,7.35);
#1368=CIRCLE('',#6542,4.);
#1369=CIRCLE('',#6543,4.);
#1370=CIRCLE('',#6544,7.35);
#1371=CIRCLE('',#6548,6.35);
#1372=CIRCLE('',#6550,6.35);
#1373=CIRCLE('',#6552,6.35);
#1374=CIRCLE('',#6554,6.35);
#1375=CIRCLE('',#6556,6.35);
#1376=CIRCLE('',#6558,6.35);
#1377=CIRCLE('',#6564,3.);
#1378=CIRCLE('',#6565,3.);
#1379=CIRCLE('',#6566,3.);
#1380=CIRCLE('',#6567,3.);
#1381=CIRCLE('',#6568,3.);
#1382=CIRCLE('',#6569,3.);
#1383=CIRCLE('',#6577,2.);
#1384=CIRCLE('',#6579,2.);
#1385=CIRCLE('',#6581,2.);
#1386=CIRCLE('',#6583,2.);
#1387=CIRCLE('',#6585,2.);
#1388=CIRCLE('',#6587,2.);
#1389=CIRCLE('',#6589,1.);
#1390=CIRCLE('',#6590,1.);
#1391=CIRCLE('',#6592,1.);
#1392=CIRCLE('',#6594,1.);
#1393=CIRCLE('',#6596,1.);
#1394=CIRCLE('',#6598,1.);
#1395=CIRCLE('',#6600,1.);
#1396=CIRCLE('',#6602,1.);
#1397=CIRCLE('',#6604,1.);
#1398=CIRCLE('',#6606,1.);
#1399=CIRCLE('',#6608,1.);
#1400=CIRCLE('',#6610,1.);
#1401=CIRCLE('',#6613,5.);
#1402=CIRCLE('',#6614,5.);
#1403=CIRCLE('',#6616,5.);
#1404=CIRCLE('',#6619,5.);
#1405=CIRCLE('',#6620,5.);
#1406=CIRCLE('',#6622,5.);
#1407=CIRCLE('',#6623,5.);
#1408=CIRCLE('',#6625,5.);
#1409=CIRCLE('',#6628,5.);
#1410=CIRCLE('',#6629,5.);
#1411=CIRCLE('',#6631,5.);
#1412=CIRCLE('',#6632,5.);
#1413=CIRCLE('',#6634,5.);
#1414=CIRCLE('',#6637,5.);
#1415=CIRCLE('',#6638,5.);
#1416=CIRCLE('',#6639,5.);
#1417=CIRCLE('',#6640,5.);
#1418=CIRCLE('',#6645,5.);
#1419=CIRCLE('',#6646,5.);
#1420=CIRCLE('',#6647,5.);
#1421=CIRCLE('',#6648,5.);
#1422=CIRCLE('',#6651,5.);
#1423=CIRCLE('',#6653,5.);
#1424=CIRCLE('',#6655,5.);
#1425=CIRCLE('',#6656,1.);
#1426=CIRCLE('',#6658,1.);
#1427=CIRCLE('',#6660,1.);
#1428=CIRCLE('',#6662,1.);
#1429=CIRCLE('',#6664,1.);
#1430=CIRCLE('',#6666,1.);
#1431=CIRCLE('',#6668,1.);
#1432=CIRCLE('',#6670,1.);
#1433=CIRCLE('',#6671,1.);
#1434=CIRCLE('',#6673,1.);
#1435=CIRCLE('',#6675,1.);
#1436=CIRCLE('',#6677,0.999999999999998);
#1437=CIRCLE('',#6679,1.);
#1438=CIRCLE('',#6681,1.);
#1439=CIRCLE('',#6683,1.);
#1440=CIRCLE('',#6685,1.);
#1441=CIRCLE('',#6686,1.);
#1442=CIRCLE('',#6688,1.);
#1443=CIRCLE('',#6691,1.);
#1444=CIRCLE('',#6693,1.);
#1445=CIRCLE('',#6695,1.);
#1446=CIRCLE('',#6697,0.999999999999999);
#1700=B_SPLINE_CURVE_WITH_KNOTS('',3,(#9090,#9091,#9092,#9093,#9094,#9095,
#9096,#9097,#9098,#9099,#9100,#9101,#9102,#9103,#9104,#9105,#9106,#9107,
#9108,#9109,#9110,#9111,#9112,#9113,#9114,#9115,#9116,#9117,#9118,#9119,
#9120,#9121,#9122,#9123,#9124,#9125),.UNSPECIFIED.,.F.,.F.,(4,2,2,2,2,2,
2,2,2,2,2,2,2,2,2,2,2,4),(112.722377729167,112.935814461693,113.265902169001,
113.583624527612,113.914511948724,114.240430230342,114.556670232197,114.887643864478,
115.209930389785,115.530836781107,115.86192664675,116.180533848522,116.512423873419,
116.839241033721,117.155181879653,117.486063018035,117.671271477257,117.853108376992),
 .UNSPECIFIED.);
#1701=B_SPLINE_CURVE_WITH_KNOTS('',3,(#9129,#9130,#9131,#9132,#9133,#9134,
#9135,#9136),.UNSPECIFIED.,.F.,.F.,(4,2,2,4),(1.00000004377154E-6,0.311560962486637,
0.633359069276319,0.894813729390518),.UNSPECIFIED.);
#1702=B_SPLINE_CURVE_WITH_KNOTS('',3,(#9140,#9141,#9142,#9143,#9144,#9145,
#9146,#9147,#9148,#9149,#9150,#9151,#9152,#9153,#9154,#9155,#9156,#9157,
#9158,#9159,#9160,#9161,#9162,#9163,#9164,#9165,#9166,#9167,#9168,#9169,
#9170,#9171,#9172,#9173,#9174,#9175),.UNSPECIFIED.,.F.,.F.,(4,2,2,2,2,2,
2,2,2,2,2,2,2,2,2,2,2,4),(0.894813729390518,0.961776507644016,1.28158051477554,
1.61400438298121,1.93318237682149,2.25667496672185,2.5877852199457,2.90394552078605,
3.23108964694769,3.56286934127997,3.88178044788897,4.21319355178493,4.53413520601621,
4.85672792330627,5.1879222585641,5.50433651680187,5.83056456912644,6.14552138395939),
 .UNSPECIFIED.);
#1703=B_SPLINE_CURVE_WITH_KNOTS('',3,(#9180,#9181,#9182,#9183,#9184,#9185,
#9186,#9187,#9188,#9189,#9190,#9191,#9192,#9193,#9194,#9195,#9196,#9197,
#9198,#9199,#9200,#9201,#9202,#9203,#9204,#9205,#9206,#9207,#9208,#9209,
#9210,#9211,#9212,#9213,#9214,#9215),.UNSPECIFIED.,.F.,.F.,(4,2,2,2,2,2,
2,2,2,2,2,2,2,2,2,2,2,4),(107.474251326802,107.742071039885,108.06977773657,
108.385852662872,108.716717431421,109.040756337916,109.358660344358,109.691706511941,
110.012041848036,110.33795465052,110.666813251939,110.983551519639,111.314497909285,
111.639657257904,111.956665800719,112.290935661215,112.612354232963,112.722377729167),
 .UNSPECIFIED.);
#1704=B_SPLINE_CURVE_WITH_KNOTS('',3,(#9216,#9217,#9218,#9219,#9220,#9221,
#9222,#9223,#9224,#9225,#9226,#9227,#9228,#9229,#9230,#9231,#9232,#9233,
#9234,#9235,#9236,#9237,#9238,#9239,#9240,#9241,#9242,#9243,#9244,#9245,
#9246,#9247,#9248,#9249,#9250,#9251,#9252,#9253),.UNSPECIFIED.,.F.,.F.,
(4,2,2,2,2,2,2,2,2,2,2,2,2,2,2,2,2,2,4),(6.14552138395939,6.1616825653315,
6.47970395444461,6.8101094302656,7.1335439556076,7.45526154677082,7.7898524160329,
8.10698412287342,8.43244913677209,8.76360062205182,9.08061784409396,9.40978773389439,
9.73561249179691,10.0562385787091,10.3895966470178,10.7075686732502,11.0319035622572,
11.3629629626413,11.3974419742764),.UNSPECIFIED.);
#1705=B_SPLINE_CURVE_WITH_KNOTS('',3,(#9258,#9259,#9260,#9261,#9262,#9263,
#9264,#9265,#9266,#9267,#9268,#9269,#9270,#9271,#9272,#9273,#9274,#9275,
#9276,#9277,#9278,#9279,#9280,#9281,#9282,#9283,#9284,#9285,#9286,#9287,
#9288,#9289,#9290,#9291,#9292,#9293),.UNSPECIFIED.,.F.,.F.,(4,2,2,2,2,2,
2,2,2,2,2,2,2,2,2,2,2,4),(102.227174401341,102.547743819964,102.873542639389,
103.189851102933,103.520835959175,103.843004394828,104.164180871344,104.495136940484,
104.813625411964,105.146003499125,105.472676947349,105.78862297816,106.119503302266,
106.442532643452,106.761857523774,107.09378555739,107.413132348819,107.474251326802),
 .UNSPECIFIED.);
#1706=B_SPLINE_CURVE_WITH_KNOTS('',3,(#9294,#9295,#9296,#9297,#9298,#9299,
#9300,#9301,#9302,#9303,#9304,#9305,#9306,#9307,#9308,#9309,#9310,#9311,
#9312,#9313,#9314,#9315,#9316,#9317,#9318,#9319,#9320,#9321,#9322,#9323,
#9324,#9325,#9326,#9327,#9328,#9329),.UNSPECIFIED.,.F.,.F.,(4,2,2,2,2,2,
2,2,2,2,2,2,2,2,2,2,2,4),(11.3974419742764,11.6792630801897,12.00727075871,
12.3360711634136,12.6556969312119,12.9879236571427,13.3072671073346,13.6305788486675,
13.9616444153745,14.2777621917807,14.6047221098277,14.9369312253169,15.2556834570718,
15.5869211480732,15.9080804574186,16.2305142097752,16.5616756401567,16.6472530619074),
 .UNSPECIFIED.);
#1707=B_SPLINE_CURVE_WITH_KNOTS('',3,(#9334,#9335,#9336,#9337,#9338,#9339,
#9340,#9341,#9342,#9343,#9344,#9345,#9346,#9347,#9348,#9349,#9350,#9351,
#9352,#9353,#9354,#9355,#9356,#9357,#9358,#9359,#9360,#9361,#9362,#9363,
#9364,#9365,#9366,#9367,#9368,#9369,#9370,#9371),.UNSPECIFIED.,.F.,.F.,
(4,2,2,2,2,2,2,2,2,2,2,2,2,2,2,2,2,2,4),(96.9781059936184,97.0189343553572,
97.349846603863,97.673784838871,97.9919085061954,98.3248402945117,98.6450784360225,
98.9714378399046,99.3001783979141,99.6168395678662,99.9478190660389,100.272864605671,
100.590015158421,100.924158382915,101.245468653185,101.569287291419,101.899248610767,
102.216858851709,102.227174401341),.UNSPECIFIED.);
#1708=B_SPLINE_CURVE_WITH_KNOTS('',3,(#9372,#9373,#9374,#9375,#9376,#9377,
#9378,#9379,#9380,#9381,#9382,#9383,#9384,#9385,#9386,#9387,#9388,#9389,
#9390,#9391,#9392,#9393,#9394,#9395,#9396,#9397,#9398,#9399,#9400,#9401,
#9402,#9403,#9404,#9405,#9406,#9407),.UNSPECIFIED.,.F.,.F.,(4,2,2,2,2,2,
2,2,2,2,2,2,2,2,2,2,2,4),(16.6472530619074,16.8781103297922,17.2041774694477,
17.5352488180356,17.8531174701921,18.1833544127834,18.5070934055145,18.8286613021236,
19.1630825685098,19.4803064183847,19.8056156297394,20.1367557994998,20.4536485378793,
20.7826578839162,21.108875414935,21.4293624838375,21.7625626929516,21.8990645150227),
 .UNSPECIFIED.);
#1709=B_SPLINE_CURVE_WITH_KNOTS('',3,(#9412,#9413,#9414,#9415,#9416,#9417,
#9418,#9419,#9420,#9421,#9422,#9423,#9424,#9425,#9426,#9427,#9428,#9429,
#9430,#9431,#9432,#9433,#9434,#9435,#9436,#9437,#9438,#9439,#9440,#9441,
#9442,#9443,#9444,#9445,#9446,#9447),.UNSPECIFIED.,.F.,.F.,(4,2,2,2,2,2,
2,2,2,2,2,2,2,2,2,2,2,4),(91.7303443229,91.8216652436239,92.1527227435167,
92.4748328043334,92.7963468711931,93.1272302292321,93.4456586663009,93.7785962802266,
94.1051857365978,94.4212037762885,94.7521445950755,95.0750919614189,95.394705394427,
95.7265371665394,96.0458029110323,96.3752586155109,96.7028613061121,96.9781059936184),
 .UNSPECIFIED.);
#1710=B_SPLINE_CURVE_WITH_KNOTS('',3,(#9448,#9449,#9450,#9451,#9452,#9453,
#9454,#9455,#9456,#9457,#9458,#9459,#9460,#9461,#9462,#9463,#9464,#9465,
#9466,#9467,#9468,#9469,#9470,#9471,#9472,#9473,#9474,#9475,#9476,#9477,
#9478,#9479,#9480,#9481,#9482,#9483),.UNSPECIFIED.,.F.,.F.,(4,2,2,2,2,2,
2,2,2,2,2,2,2,2,2,2,2,4),(21.8990645150227,22.080704098049,22.404895807676,
22.7359583196053,23.052208146303,23.3800687533882,23.7093337294194,24.0288361082048,
24.3609225018898,24.6805048958586,25.0036915857874,25.3347732880507,25.6509147409374,
25.9777469929682,26.310465518035,26.6291148632443,26.9602352134497,27.1490940819086),
 .UNSPECIFIED.);
#1711=B_SPLINE_CURVE_WITH_KNOTS('',3,(#9488,#9489,#9490,#9491,#9492,#9493,
#9494,#9495,#9496,#9497,#9498,#9499,#9500,#9501,#9502,#9503,#9504,#9505,
#9506,#9507,#9508,#9509,#9510,#9511,#9512,#9513,#9514,#9515,#9516,#9517,
#9518,#9519,#9520,#9521,#9522,#9523),.UNSPECIFIED.,.F.,.F.,(4,2,2,2,2,2,
2,2,2,2,2,2,2,2,2,2,2,4),(86.4798314140111,86.6227800760488,86.9556609508597,
87.2758626652495,87.6027341887179,87.9314188779159,88.2480710512407,88.5791451872703,
88.904138285101,89.2214976252686,89.5555772220635,89.8768395886157,90.2010842871321,
90.5309809091133,90.848538274585,91.1794826620175,91.5052225752388,91.7303443229),
 .UNSPECIFIED.);
#1712=B_SPLINE_CURVE_WITH_KNOTS('',3,(#9524,#9525,#9526,#9527,#9528,#9529,
#9530,#9531,#9532,#9533,#9534,#9535,#9536,#9537,#9538,#9539,#9540,#9541,
#9542,#9543,#9544,#9545,#9546,#9547,#9548,#9549,#9550,#9551,#9552,#9553,
#9554,#9555,#9556,#9557,#9558,#9559),.UNSPECIFIED.,.F.,.F.,(4,2,2,2,2,2,
2,2,2,2,2,2,2,2,2,2,2,4),(27.1490940819086,27.2816841559646,27.6040159460672,
27.935205618183,28.2517271794494,28.5776912122136,28.9087772011457,29.2265497511765,
29.5566769523901,29.8807942522771,30.2022702407119,30.5365819291874,30.8539667784873,
31.1791788250368,31.5103692663226,31.82720356108,32.1561117178664,32.4014535157498),
 .UNSPECIFIED.);
#1713=B_SPLINE_CURVE_WITH_KNOTS('',3,(#9564,#9565,#9566,#9567,#9568,#9569,
#9570,#9571,#9572,#9573,#9574,#9575,#9576,#9577,#9578,#9579,#9580,#9581,
#9582,#9583,#9584,#9585,#9586,#9587,#9588,#9589,#9590,#9591,#9592,#9593,
#9594,#9595,#9596,#9597,#9598,#9599),.UNSPECIFIED.,.F.,.F.,(4,2,2,2,2,2,
2,2,2,2,2,2,2,2,2,2,2,4),(81.2303172007343,81.4251321858443,81.7560069702517,
82.0744367502896,82.4079916863948,82.7345602143883,83.0507161535853,83.3817783439728,
83.7047059180943,84.0246708033549,84.3564702037923,84.6757160394563,85.0057507119943,
85.3333120660503,85.6494509767062,85.9804718601221,86.3043712286969,86.4798314140111),
 .UNSPECIFIED.);
#1714=B_SPLINE_CURVE_WITH_KNOTS('',3,(#9600,#9601,#9602,#9603,#9604,#9605,
#9606,#9607,#9608,#9609,#9610,#9611,#9612,#9613,#9614,#9615,#9616,#9617,
#9618,#9619,#9620,#9621,#9622,#9623,#9624,#9625,#9626,#9627,#9628,#9629,
#9630,#9631,#9632,#9633,#9634,#9635),.UNSPECIFIED.,.F.,.F.,(4,2,2,2,2,2,
2,2,2,2,2,2,2,2,2,2,2,4),(32.4014535157498,32.4827954803396,32.8032018866308,
33.1363049419288,33.4546849111464,33.7787927583837,34.1099198526596,34.4261866157241,
34.7539602528262,35.0837611091104,35.4031991295255,35.735206665648,36.0550960135157,
36.3782177053124,36.709376966425,37.0256089756814,37.352374450904,37.6524303097187),
 .UNSPECIFIED.);
#1715=B_SPLINE_CURVE_WITH_KNOTS('',3,(#9640,#9641,#9642,#9643,#9644,#9645,
#9646,#9647,#9648,#9649,#9650,#9651,#9652,#9653,#9654,#9655,#9656,#9657,
#9658,#9659,#9660,#9661,#9662,#9663,#9664,#9665,#9666,#9667,#9668,#9669,
#9670,#9671,#9672,#9673,#9674,#9675),.UNSPECIFIED.,.F.,.F.,(4,2,2,2,2,2,
2,2,2,2,2,2,2,2,2,2,2,4),(75.9777376249721,76.2296477532921,76.5583412626286,
76.8750533353474,77.2062822942674,77.531286732469,77.8489168802109,78.1829985904649,
78.5042757431245,78.8290038626106,79.158900305632,79.4764665215315,79.8075318515091,
80.1332760850523,80.4499160587139,80.7811068885252,81.1032209347659,81.2303172007343),
 .UNSPECIFIED.);
#1716=B_SPLINE_CURVE_WITH_KNOTS('',3,(#9676,#9677,#9678,#9679,#9680,#9681,
#9682,#9683,#9684,#9685,#9686,#9687,#9688,#9689,#9690,#9691,#9692,#9693,
#9694,#9695,#9696,#9697,#9698,#9699,#9700,#9701,#9702,#9703,#9704,#9705,
#9706,#9707,#9708,#9709,#9710,#9711,#9712,#9713),.UNSPECIFIED.,.F.,.F.,
(4,2,2,2,2,2,2,2,2,2,2,2,2,2,2,2,2,2,4),(37.6524303097187,37.6856703367532,
38.0042764730292,38.3353416640884,38.6571458291731,38.9794363498445,39.3107157137369,
39.6273894493943,39.9533119208669,40.2844745667797,40.6022111901814,40.932291381766,
41.256852033589,41.5782973531143,41.9125634479899,42.2301750011463,42.5553521316008,
42.886654185985,42.9060171593307),.UNSPECIFIED.);
#1717=B_SPLINE_CURVE_WITH_KNOTS('',3,(#9718,#9719,#9720,#9721,#9722,#9723,
#9724,#9725,#9726,#9727,#9728,#9729,#9730,#9731,#9732,#9733,#9734,#9735,
#9736,#9737,#9738,#9739,#9740,#9741,#9742,#9743,#9744,#9745,#9746,#9747,
#9748,#9749,#9750,#9751,#9752,#9753),.UNSPECIFIED.,.F.,.F.,(4,2,2,2,2,2,
2,2,2,2,2,2,2,2,2,2,2,4),(70.7257701778119,71.0320289658823,71.3586411516273,
71.6749977042479,72.0062401831685,72.3292116408242,72.6495824341981,72.981415199054,
73.3007037729756,73.6313652344112,73.9589500206666,74.2752212361238,74.60641024243,
74.9303345803813,75.2490873252793,75.5819831233109,75.902211150012,75.9777376249721),
 .UNSPECIFIED.);
#1718=B_SPLINE_CURVE_WITH_KNOTS('',3,(#9754,#9755,#9756,#9757,#9758,#9759,
#9760,#9761,#9762,#9763,#9764,#9765,#9766,#9767,#9768,#9769,#9770,#9771,
#9772,#9773,#9774,#9775,#9776,#9777,#9778,#9779,#9780,#9781,#9782,#9783,
#9784,#9785,#9786,#9787,#9788,#9789),.UNSPECIFIED.,.F.,.F.,(4,2,2,2,2,2,
2,2,2,2,2,2,2,2,2,2,2,4),(42.9060171593307,43.2034986491151,43.5323687043631,
43.8595809104928,44.1799681785184,44.5130384264816,44.8317208112402,45.1558073806985,
45.4870599295524,45.8034112826383,46.1311614264702,46.4615563210303,46.7809917528282,
47.1129850599791,47.4332420968641,47.7563616063971,48.0876589350017,48.1589956367661),
 .UNSPECIFIED.);
#1719=B_SPLINE_CURVE_WITH_KNOTS('',3,(#9794,#9795,#9796,#9797,#9798,#9799,
#9800,#9801,#9802,#9803,#9804,#9805,#9806,#9807,#9808,#9809,#9810,#9811,
#9812,#9813,#9814,#9815,#9816,#9817,#9818,#9819,#9820,#9821,#9822,#9823,
#9824,#9825,#9826,#9827,#9828,#9829,#9830,#9831),.UNSPECIFIED.,.F.,.F.,
(4,2,2,2,2,2,2,2,2,2,2,2,2,2,2,2,2,2,4),(65.4704662597666,65.495672175373,
65.8271134020289,66.152193527227,66.4701500123141,66.804300390124,67.1256555179792,
67.4509129283782,67.7808746179128,68.0985120833682,68.4297579283883,68.7555705314816,
69.0724663315543,69.4038489357916,69.7260301625157,70.0483887785603,70.3793203104939,
70.6978137297548,70.7257701778119),.UNSPECIFIED.);
#1720=B_SPLINE_CURVE_WITH_KNOTS('',3,(#9832,#9833,#9834,#9835,#9836,#9837,
#9838,#9839,#9840,#9841,#9842,#9843,#9844,#9845,#9846,#9847,#9848,#9849,
#9850,#9851,#9852,#9853,#9854,#9855,#9856,#9857,#9858,#9859,#9860,#9861,
#9862,#9863,#9864,#9865,#9866,#9867),.UNSPECIFIED.,.F.,.F.,(4,2,2,2,2,2,
2,2,2,2,2,2,2,2,2,2,2,4),(48.1589956367661,48.4040467523655,48.7308091602174,
49.0647361611568,49.3833609345423,49.7144356594085,50.0366521626909,50.3589642243882,
50.6903935164885,51.0072814592698,51.333226046925,51.6645265155671,51.9822893424162,
52.3123875254735,52.6374457953631,52.9589234957672,53.2816759952905,53.4142923811308),
 .UNSPECIFIED.);
#1721=B_SPLINE_CURVE_WITH_KNOTS('',3,(#9872,#9873,#9874,#9875,#9876,#9877,
#9878,#9879,#9880,#9881,#9882,#9883,#9884,#9885,#9886,#9887,#9888,#9889,
#9890,#9891,#9892,#9893,#9894,#9895,#9896,#9897,#9898,#9899,#9900,#9901,
#9902,#9903,#9904,#9905,#9906,#9907),.UNSPECIFIED.,.F.,.F.,(4,2,2,2,2,2,
2,2,2,2,2,2,2,2,2,2,2,4),(60.2150166643538,60.2919896896549,60.623468135119,
60.946546784158,61.2673685979683,61.5993003656792,61.9186940219388,62.2500158622836,
62.5776890328341,62.8941555378412,63.225569156602,63.5495824617272,63.8687296591539,
64.2017066441746,64.5220238831432,64.8500653079831,65.1788329505325,65.4704662597666),
 .UNSPECIFIED.);
#1722=B_SPLINE_CURVE_WITH_KNOTS('',3,(#9908,#9909,#9910,#9911,#9912,#9913,
#9914,#9915,#9916,#9917,#9918,#9919,#9920,#9921,#9922,#9923,#9924,#9925,
#9926,#9927,#9928,#9929,#9930,#9931,#9932,#9933,#9934,#9935,#9936,#9937,
#9938,#9939,#9940,#9941,#9942,#9943),.UNSPECIFIED.,.F.,.F.,(4,2,2,2,2,2,
2,2,2,2,2,2,2,2,2,2,2,4),(53.4142923811308,53.6035626727488,53.9351146179854,
54.2541797621075,54.5873610415979,54.9146187411077,55.2311787077779,55.5626980944589,
55.8863055375212,56.2063209314299,56.5388391129682,56.8587574511558,57.1884786504444,
57.5167651433843,57.8334302207767,58.1649297922668,58.4895427229089,58.6712567519585),
 .UNSPECIFIED.);
#1723=B_SPLINE_CURVE_WITH_KNOTS('',3,(#9948,#9949,#9950,#9951,#9952,#9953,
#9954,#9955,#9956,#9957,#9958,#9959,#9960,#9961,#9962,#9963,#9964,#9965,
#9966,#9967,#9968,#9969,#9970,#9971,#9972,#9973,#9974,#9975,#9976,#9977,
#9978,#9979,#9980,#9981,#9982,#9983),.UNSPECIFIED.,.F.,.F.,(4,2,2,2,2,2,
2,2,2,2,2,2,2,2,2,2,2,4),(54.958820463279,55.0853253597811,55.4191724857657,
55.7402468059445,56.0656389533752,56.3952984859766,56.7127551628249,57.0441447347562,
57.3700887293421,57.6872929598775,58.0189223071554,58.3412329272213,58.6640792208409,
58.9951320971355,59.3137505884142,59.6486547000943,59.9753747519229,60.2150166643538),
 .UNSPECIFIED.);
#1724=B_SPLINE_CURVE_WITH_KNOTS('',3,(#9984,#9985,#9986,#9987,#9988,#9989,
#9990,#9991,#9992,#9993,#9994,#9995,#9996,#9997,#9998,#9999,#10000,#10001,
#10002,#10003,#10004,#10005,#10006,#10007,#10008,#10009,#10010,#10011,#10012,
#10013,#10014,#10015,#10016,#10017,#10018,#10019),.UNSPECIFIED.,.F.,.F.,
(4,2,2,2,2,2,2,2,2,2,2,2,2,2,2,2,2,4),(58.6712567519585,58.8081120487695,
59.1417446836893,59.4626482699573,59.789314753556,60.1187508570411,60.4360562388358,
60.7676329075686,61.0933642112501,61.4110112022744,61.7458659425563,62.0678512720903,
62.3920318907359,62.7226968235716,63.0409778752441,63.3724839946026,63.6989739681192,
63.9299842069763),.UNSPECIFIED.);
#1725=B_SPLINE_CURVE_WITH_KNOTS('',3,(#10024,#10025,#10026,#10027,#10028,
#10029,#10030,#10031,#10032,#10033,#10034,#10035,#10036,#10037,#10038,#10039,
#10040,#10041,#10042,#10043,#10044,#10045,#10046,#10047,#10048,#10049,#10050,
#10051,#10052,#10053,#10054,#10055,#10056,#10057,#10058,#10059),
 .UNSPECIFIED.,.F.,.F.,(4,2,2,2,2,2,2,2,2,2,2,2,2,2,2,2,2,4),(49.7053427805776,
49.8946649833997,50.2193889038838,50.5506783072757,50.8672681505552,51.1956719499015,
51.5241929101829,51.8441827696492,52.176801691369,52.4961122101446,52.8197929106681,
53.1510737257235,53.4673975704681,53.7947321500115,54.1113468652774,54.4426191551792,
54.7674124920873,54.958820463279),.UNSPECIFIED.);
#1726=B_SPLINE_CURVE_WITH_KNOTS('',3,(#10060,#10061,#10062,#10063,#10064,
#10065,#10066,#10067,#10068,#10069,#10070,#10071,#10072,#10073,#10074,#10075,
#10076,#10077,#10078,#10079,#10080,#10081,#10082,#10083,#10084,#10085,#10086,
#10087,#10088,#10089,#10090,#10091,#10092,#10093,#10094,#10095),
 .UNSPECIFIED.,.F.,.F.,(4,2,2,2,2,2,2,2,2,2,2,2,2,2,2,2,2,4),(63.9299842069763,
64.0158273939492,64.3474243448431,64.6702762228065,64.9918697143397,65.3235363775539,
65.6427018726441,65.9753696656186,66.3027524871346,66.6192856711435,66.9507860810698,
67.2745160647127,67.5942889179192,67.926944884661,68.2469841445378,68.576236629585,
68.9046677223753,69.1866887443586),.UNSPECIFIED.);
#1727=B_SPLINE_CURVE_WITH_KNOTS('',3,(#10100,#10101,#10102,#10103,#10104,
#10105,#10106,#10107,#10108,#10109,#10110,#10111,#10112,#10113,#10114,#10115,
#10116,#10117,#10118,#10119,#10120,#10121,#10122,#10123,#10124,#10125,#10126,
#10127,#10128,#10129,#10130,#10131,#10132,#10133,#10134,#10135),
 .UNSPECIFIED.,.F.,.F.,(4,2,2,2,2,2,2,2,2,2,2,2,2,2,2,2,2,4),(44.4491313433541,
44.6870015935932,45.0136378977987,45.3450417551313,45.6634567886658,45.9942822750444,
46.3176176911724,46.639728628672,46.9747441773675,47.2920071882406,47.61787524196,
47.949273189522,48.2666625046887,48.5962434167468,48.921870506651,49.2428780108371,
49.5766476892823,49.7053427805776),.UNSPECIFIED.);
#1728=B_SPLINE_CURVE_WITH_KNOTS('',3,(#10136,#10137,#10138,#10139,#10140,
#10141,#10142,#10143,#10144,#10145,#10146,#10147,#10148,#10149,#10150,#10151,
#10152,#10153,#10154,#10155,#10156,#10157,#10158,#10159,#10160,#10161,#10162,
#10163,#10164,#10165,#10166,#10167,#10168,#10169,#10170,#10171,#10172,#10173),
 .UNSPECIFIED.,.F.,.F.,(4,2,2,2,2,2,2,2,2,2,2,2,2,2,2,2,2,2,4),(69.1866887443586,
69.2213801122111,69.5528737530356,69.8776274198326,70.1960238834839,70.5298118984127,
70.8508520952963,71.1771217050446,71.5067159395957,71.8241430246874,72.1557282115081,
72.4816129287093,72.7991644584063,73.1341863748964,73.4563190370224,73.7801912419322,
74.1110223351671,74.429453819747,74.4454842874606),.UNSPECIFIED.);
#1729=B_SPLINE_CURVE_WITH_KNOTS('',3,(#10178,#10179,#10180,#10181,#10182,
#10183,#10184,#10185,#10186,#10187,#10188,#10189,#10190,#10191,#10192,#10193,
#10194,#10195,#10196,#10197,#10198,#10199,#10200,#10201,#10202,#10203,#10204,
#10205,#10206,#10207,#10208,#10209,#10210,#10211,#10212,#10213),
 .UNSPECIFIED.,.F.,.F.,(4,2,2,2,2,2,2,2,2,2,2,2,2,2,2,2,2,4),(39.1940267703943,
39.4837106853752,39.8123739358409,40.140615639691,40.4608409439614,40.7937158675648,
41.112947714973,41.4368674212289,41.768260888568,42.0847004092134,42.4122780772443,
42.7438288668753,43.0631402657561,43.3949808385494,43.7159177151437,44.0389137877124,
44.3703784563307,44.4491313433541),.UNSPECIFIED.);
#1730=B_SPLINE_CURVE_WITH_KNOTS('',3,(#10214,#10215,#10216,#10217,#10218,
#10219,#10220,#10221,#10222,#10223,#10224,#10225,#10226,#10227,#10228,#10229,
#10230,#10231,#10232,#10233,#10234,#10235,#10236,#10237,#10238,#10239,#10240,
#10241,#10242,#10243,#10244,#10245,#10246,#10247,#10248,#10249),
 .UNSPECIFIED.,.F.,.F.,(4,2,2,2,2,2,2,2,2,2,2,2,2,2,2,2,2,4),(74.4454842874606,
74.7610038707573,75.0876524143285,75.4044823371837,75.7361094557603,76.059117988834,
76.3804901299688,76.7123298778693,77.0316519837141,77.3638858973244,77.6914506845162,
78.0080234552417,78.3395658510996,78.6634744683095,78.98307823724,79.3159291149286,
79.636144436891,79.7030451201867),.UNSPECIFIED.);
#1731=B_SPLINE_CURVE_WITH_KNOTS('',3,(#10254,#10255,#10256,#10257,#10258,
#10259,#10260,#10261,#10262,#10263,#10264,#10265,#10266,#10267,#10268,#10269,
#10270,#10271,#10272,#10273,#10274,#10275,#10276,#10277,#10278,#10279,#10280,
#10281,#10282,#10283,#10284,#10285,#10286,#10287,#10288,#10289,#10290,#10291),
 .UNSPECIFIED.,.F.,.F.,(4,2,2,2,2,2,2,2,2,2,2,2,2,2,2,2,2,2,4),(33.9358727252235,
33.9621245083147,34.2809288568771,34.6121781063724,34.9350748526361,35.2575723609102,
35.5893508296672,35.9066695684309,36.2328023369551,36.5643384731628,36.881976653502,
37.2118280837638,37.5372450060053,37.8585010955848,38.1925414770318,38.510544921809,
38.8355231435545,39.1669372659656,39.1940267703943),.UNSPECIFIED.);
#1732=B_SPLINE_CURVE_WITH_KNOTS('',3,(#10292,#10293,#10294,#10295,#10296,
#10297,#10298,#10299,#10300,#10301,#10302,#10303,#10304,#10305,#10306,#10307,
#10308,#10309,#10310,#10311,#10312,#10313,#10314,#10315,#10316,#10317,#10318,
#10319,#10320,#10321,#10322,#10323,#10324,#10325,#10326,#10327),
 .UNSPECIFIED.,.F.,.F.,(4,2,2,2,2,2,2,2,2,2,2,2,2,2,2,2,2,4),(79.7030451201867,
79.9650097989887,80.2936411166196,80.6104655377856,80.9420139501394,81.2669633105644,
81.5852589459215,81.9192583194259,82.2404892582695,82.5664436673889,82.896250644087,
83.2138610400208,83.5455152139737,83.8716073734113,84.189133085679,84.5243772521638,
84.8467106050261,84.9624042671722),.UNSPECIFIED.);
#1733=B_SPLINE_CURVE_WITH_KNOTS('',3,(#10332,#10333,#10334,#10335,#10336,
#10337,#10338,#10339,#10340,#10341,#10342,#10343,#10344,#10345,#10346,#10347,
#10348,#10349,#10350,#10351,#10352,#10353,#10354,#10355,#10356,#10357,#10358,
#10359,#10360,#10361,#10362,#10363,#10364,#10365,#10366,#10367),
 .UNSPECIFIED.,.F.,.F.,(4,2,2,2,2,2,2,2,2,2,2,2,2,2,2,2,2,4),(28.6778433505252,
28.751513892831,29.0720320491282,29.4052222858157,29.7244522500093,30.0486692456809,
30.3802402592666,30.6968635486887,31.0247433023543,31.356055628844,31.6756433970708,
32.0077807707016,32.3286652307542,32.6519398567504,32.9835714209526,33.3003193076007,
33.6272377323579,33.9358727252235),.UNSPECIFIED.);
#1734=B_SPLINE_CURVE_WITH_KNOTS('',3,(#10368,#10369,#10370,#10371,#10372,
#10373,#10374,#10375,#10376,#10377,#10378,#10379,#10380,#10381,#10382,#10383,
#10384,#10385,#10386,#10387,#10388,#10389,#10390,#10391,#10392,#10393,#10394,
#10395,#10396,#10397,#10398,#10399,#10400,#10401,#10402,#10403),
 .UNSPECIFIED.,.F.,.F.,(4,2,2,2,2,2,2,2,2,2,2,2,2,2,2,2,2,4),(84.9624042671722,
85.1703540448489,85.5014052173264,85.8200393157319,86.1516925680166,86.4785528419088,
86.7954247866363,87.1271416154083,87.4503592344816,87.7715856592211,88.1036516073096,
88.4231817863373,88.7550702706801,89.0828684670286,89.3995444073536,89.7311877492214,
90.0553258055558,90.2220141793614),.UNSPECIFIED.);
#1735=B_SPLINE_CURVE_WITH_KNOTS('',3,(#10408,#10409,#10410,#10411,#10412,
#10413,#10414,#10415,#10416,#10417,#10418,#10419,#10420,#10421,#10422,#10423,
#10424,#10425,#10426,#10427,#10428,#10429,#10430,#10431,#10432,#10433,#10434,
#10435,#10436,#10437,#10438,#10439,#10440,#10441,#10442,#10443),
 .UNSPECIFIED.,.F.,.F.,(4,2,2,2,2,2,2,2,2,2,2,2,2,2,2,2,2,4),(23.4194570300931,
23.5448375458363,23.8672296315852,24.1987821581931,24.5158120140399,24.8418376691952,
25.1732575822623,25.4911009723972,25.8212799176309,26.1465728220054,26.468133988391,
26.8025033396155,27.1205676123453,27.4458573583117,27.777460695228,28.0944829929136,
28.423463545569,28.6778433505252),.UNSPECIFIED.);
#1736=B_SPLINE_CURVE_WITH_KNOTS('',3,(#10444,#10445,#10446,#10447,#10448,
#10449,#10450,#10451,#10452,#10453,#10454,#10455,#10456,#10457,#10458,#10459,
#10460,#10461,#10462,#10463,#10464,#10465,#10466,#10467,#10468,#10469,#10470,
#10471,#10472,#10473,#10474,#10475,#10476,#10477,#10478,#10479),
 .UNSPECIFIED.,.F.,.F.,(4,2,2,2,2,2,2,2,2,2,2,2,2,2,2,2,2,4),(90.2220141793614,
90.3748353736429,90.7079326119538,91.0283739647954,91.3569409816704,91.6858224287003,
92.0028189133833,92.3344804973216,92.6596749253133,92.9779419941321,93.3122027564306,
93.633673155364,93.959399049641,94.2894674880067,94.6073164436775,94.9390974276225,
95.2654453128683,95.4826145482641),.UNSPECIFIED.);
#1737=B_SPLINE_CURVE_WITH_KNOTS('',3,(#10484,#10485,#10486,#10487,#10488,
#10489,#10490,#10491,#10492,#10493,#10494,#10495,#10496,#10497,#10498,#10499,
#10500,#10501,#10502,#10503,#10504,#10505,#10506,#10507,#10508,#10509,#10510,
#10511,#10512,#10513,#10514,#10515,#10516,#10517,#10518,#10519),
 .UNSPECIFIED.,.F.,.F.,(4,2,2,2,2,2,2,2,2,2,2,2,2,2,2,2,2,4),(18.1643899839031,
18.3379240397195,18.6620768943873,18.9934447562906,19.3098966760481,19.6377132453628,
19.9683761687022,20.2878829729932,20.6199467688078,20.9403963553448,21.2635882727924,
21.5950049811214,21.9115161728676,22.2383515620108,22.5725584681035,22.8912614297431,
23.2224142667495,23.4194570300931),.UNSPECIFIED.);
#1738=B_SPLINE_CURVE_WITH_KNOTS('',3,(#10520,#10521,#10522,#10523,#10524,
#10525,#10526,#10527,#10528,#10529,#10530,#10531,#10532,#10533,#10534,#10535,
#10536,#10537,#10538,#10539,#10540,#10541,#10542,#10543,#10544,#10545,#10546,
#10547,#10548,#10549,#10550,#10551,#10552,#10553,#10554,#10555),
 .UNSPECIFIED.,.F.,.F.,(4,2,2,2,2,2,2,2,2,2,2,2,2,2,2,2,2,4),(95.4826145482641,
95.5830131784909,95.9150352583438,96.2377453618514,96.5609337305379,96.8923988013166,
97.2114126750681,97.5466420806929,97.873770877236,98.1907566599105,98.5226293845204,
98.8461121465705,99.1672791546219,99.4996279190605,99.8194212411041,100.151068073815,
100.47915443311,100.745055882445),.UNSPECIFIED.);
#1739=B_SPLINE_CURVE_WITH_KNOTS('',3,(#10560,#10561,#10562,#10563,#10564,
#10565,#10566,#10567,#10568,#10569,#10570,#10571,#10572,#10573,#10574,#10575,
#10576,#10577,#10578,#10579,#10580,#10581,#10582,#10583,#10584,#10585,#10586,
#10587,#10588,#10589,#10590,#10591,#10592,#10593,#10594,#10595),
 .UNSPECIFIED.,.F.,.F.,(4,2,2,2,2,2,2,2,2,2,2,2,2,2,2,2,2,4),(12.9085896449044,
13.1319654813851,13.4579477094742,13.7892099133384,14.1070063349617,14.4371455212647,
14.7619252560797,15.0834330090954,15.4177596038885,15.7355181257431,16.0607572042731,
16.3921701425435,16.7090911171914,17.0380229391824,17.3654819678967,17.6859353124529,
18.0190701048524,18.1643899839031),.UNSPECIFIED.);
#1740=B_SPLINE_CURVE_WITH_KNOTS('',3,(#10596,#10597,#10598,#10599,#10600,
#10601,#10602,#10603,#10604,#10605,#10606,#10607,#10608,#10609,#10610,#10611,
#10612,#10613,#10614,#10615,#10616,#10617,#10618,#10619,#10620,#10621,#10622,
#10623,#10624,#10625,#10626,#10627,#10628,#10629,#10630,#10631,#10632,#10633),
 .UNSPECIFIED.,.F.,.F.,(4,2,2,2,2,2,2,2,2,2,2,2,2,2,2,2,2,2,4),(100.745055882445,
100.796001734715,101.127811382384,101.452233014914,101.771732249291,102.105130527508,
102.425851249821,102.754222181351,103.083406799012,103.400638353147,103.732477635844,
104.057969677998,104.37628762465,104.710862903123,105.032624730452,105.358220131125,
105.688601838775,106.006642269571,106.007580002483),.UNSPECIFIED.);
#1741=B_SPLINE_CURVE_WITH_KNOTS('',3,(#10638,#10639,#10640,#10641,#10642,
#10643,#10644,#10645,#10646,#10647,#10648,#10649,#10650,#10651,#10652,#10653,
#10654,#10655,#10656,#10657,#10658,#10659,#10660,#10661,#10662,#10663,#10664,
#10665,#10666,#10667,#10668,#10669,#10670,#10671,#10672,#10673),
 .UNSPECIFIED.,.F.,.F.,(4,2,2,2,2,2,2,2,2,2,2,2,2,2,2,2,2,4),(7.65580643120489,
7.92903377067465,8.25685231429426,8.586904928944,8.90639349536678,9.23844967293158,
9.55851322774851,9.88168615770634,10.2129451312994,10.5292795485054,10.8560965326263,
11.1896576540031,11.508321254098,11.8394428317127,12.1614368336248,12.4837863523509,
12.8151694339259,12.9085896449044),.UNSPECIFIED.);
#1742=B_SPLINE_CURVE_WITH_KNOTS('',3,(#10674,#10675,#10676,#10677,#10678,
#10679,#10680,#10681,#10682,#10683,#10684,#10685,#10686,#10687,#10688,#10689,
#10690,#10691,#10692,#10693,#10694,#10695,#10696,#10697,#10698,#10699,#10700,
#10701,#10702,#10703,#10704,#10705,#10706,#10707,#10708,#10709),
 .UNSPECIFIED.,.F.,.F.,(4,2,2,2,2,2,2,2,2,2,2,2,2,2,2,2,2,4),(106.007580002483,
106.338291050777,106.664517770686,106.981785151794,107.313569075925,107.63615988381,
107.958865999156,108.290220246233,108.609119030096,108.943662487344,109.270693914527,
109.587430237008,109.919075729356,110.242461649198,110.563183930418,110.895444456502,
111.215142893136,111.266831993831),.UNSPECIFIED.);
#1743=B_SPLINE_CURVE_WITH_KNOTS('',3,(#10715,#10716,#10717,#10718,#10719,
#10720,#10721,#10722,#10723,#10724,#10725,#10726),.UNSPECIFIED.,.F.,.F.,
(4,2,2,2,2,4),(116.52588314767,116.750177738512,117.080505043093,117.398484542365,
117.660053024643,117.93068616261),.UNSPECIFIED.);
#1744=B_SPLINE_CURVE_WITH_KNOTS('',3,(#10729,#10730,#10731,#10732,#10733,
#10734,#10735,#10736,#10737,#10738,#10739,#10740,#10741,#10742,#10743,#10744,
#10745,#10746),.UNSPECIFIED.,.F.,.F.,(4,2,2,2,2,2,2,2,4),(1.00000002753453E-6,
0.230913164999998,0.461176488336289,0.782795083268026,1.10516503507019,
1.43643805917748,1.75306071300765,2.07906337640022,2.40199466308743),
 .UNSPECIFIED.);
#1745=B_SPLINE_CURVE_WITH_KNOTS('',3,(#10781,#10782,#10783,#10784,#10785,
#10786,#10787,#10788,#10789,#10790,#10791,#10792,#10793,#10794,#10795,#10796,
#10797,#10798,#10799,#10800,#10801,#10802,#10803,#10804,#10805,#10806,#10807,
#10808,#10809,#10810,#10811,#10812,#10813,#10814,#10815,#10816,#10817,#10818,
#10819,#10820,#10821,#10822,#10823,#10824,#10825,#10826,#10827,#10828,#10829,
#10830,#10831,#10832,#10833,#10834,#10835),.UNSPECIFIED.,.F.,.F.,(4,3,3,
3,3,3,3,3,3,3,3,3,3,3,3,3,3,3,4),(1.5707963267949,1.64242105278282,1.71479015258711,
1.78837553839344,1.86258767446152,1.93745389192044,1.96813996588655,2.04189099921108,
2.1192539697587,2.19381715259638,2.26806604838722,2.34147638917228,2.35134288140155,
2.42596150493344,2.50323613885248,2.57624208460566,2.64856017426106,2.72000077351568,
2.73506004060959),.UNSPECIFIED.);
#1746=B_SPLINE_CURVE_WITH_KNOTS('',3,(#10854,#10855,#10856,#10857,#10858,
#10859,#10860,#10861,#10862,#10863,#10864,#10865,#10866,#10867,#10868,#10869,
#10870,#10871,#10872,#10873,#10874,#10875,#10876,#10877,#10878,#10879,#10880,
#10881,#10882,#10883,#10884,#10885,#10886,#10887,#10888,#10889,#10890,#10891,
#10892,#10893,#10894,#10895,#10896,#10897,#10898,#10899,#10900,#10901,#10902,
#10903,#10904,#10905,#10906,#10907,#10908),.UNSPECIFIED.,.F.,.F.,(4,3,3,
3,3,3,3,3,3,3,3,3,3,3,3,3,3,3,4),(1.5707963267949,1.64242105278141,1.71479015258438,
1.78837553839004,1.86258767445774,1.93745389191671,1.96813996588634,2.04189099921108,
2.11925396975866,2.19381715259688,2.26806604838803,2.34147638917343,2.35134288140141,
2.42596150493384,2.50323613885278,2.57624208460631,2.64856017426199,2.72000077351667,
2.73506004060958),.UNSPECIFIED.);
#1747=B_SPLINE_CURVE_WITH_KNOTS('',3,(#10922,#10923,#10924,#10925,#10926,
#10927,#10928,#10929,#10930,#10931,#10932,#10933,#10934,#10935,#10936,#10937,
#10938,#10939,#10940,#10941,#10942,#10943,#10944,#10945,#10946,#10947,#10948,
#10949,#10950,#10951,#10952,#10953,#10954,#10955,#10956,#10957,#10958,#10959,
#10960,#10961,#10962,#10963,#10964,#10965,#10966,#10967),.UNSPECIFIED.,
 .F.,.F.,(4,3,3,3,3,3,3,3,3,3,3,3,3,3,3,4),(0.,0.000102625409859305,0.000209255998910644,
0.000322661982762533,0.000440290006433478,0.000564825588011048,0.000629111603363879,
0.00077150452647986,0.0008514190604454,0.0009068473692292,0.000932968415359167,
0.00114800502221307,0.00137019159493578,0.00141082079820418,0.00163330152526633,
0.00183019574357075),.UNSPECIFIED.);
#1748=B_SPLINE_CURVE_WITH_KNOTS('',3,(#10969,#10970,#10971,#10972,#10973,
#10974,#10975,#10976,#10977,#10978,#10979,#10980,#10981,#10982,#10983,#10984,
#10985,#10986,#10987,#10988,#10989,#10990,#10991,#10992,#10993,#10994,#10995,
#10996,#10997,#10998,#10999,#11000,#11001,#11002,#11003,#11004,#11005,#11006,
#11007,#11008,#11009,#11010,#11011,#11012,#11013,#11014,#11015,#11016,#11017,
#11018,#11019,#11020),.UNSPECIFIED.,.F.,.F.,(4,3,3,3,3,3,3,3,3,3,3,3,3,
3,3,3,3,4),(0.00183019700058168,0.0021246721247389,0.00232004474458504,
0.00265469094004782,0.0030060000015604,0.00333449619907014,0.00369804959273491,
0.00408054678755802,0.00447405832991094,0.00488126280004193,0.00494084368376952,
0.00544455820475954,0.00560720862373659,0.00609214785612222,0.00662068586019803,
0.00717627308542189,0.00775568315893149,0.00805149036695734),
 .UNSPECIFIED.);
#1749=B_SPLINE_CURVE_WITH_KNOTS('',3,(#11024,#11025,#11026,#11027,#11028,
#11029,#11030,#11031,#11032,#11033,#11034,#11035,#11036,#11037,#11038,#11039,
#11040,#11041,#11042,#11043,#11044,#11045,#11046,#11047,#11048,#11049,#11050,
#11051,#11052,#11053,#11054,#11055,#11056,#11057,#11058,#11059,#11060,#11061,
#11062,#11063,#11064,#11065,#11066,#11067,#11068,#11069,#11070,#11071,#11072,
#11073,#11074,#11075,#11076,#11077,#11078,#11079,#11080,#11081,#11082,#11083,
#11084,#11085,#11086,#11087,#11088,#11089,#11090,#11091,#11092,#11093,#11094,
#11095,#11096,#11097,#11098,#11099,#11100,#11101,#11102,#11103,#11104,#11105,
#11106,#11107,#11108,#11109,#11110,#11111,#11112,#11113,#11114),
 .UNSPECIFIED.,.F.,.F.,(4,3,3,3,3,3,3,3,3,3,3,3,3,3,3,3,3,3,3,3,3,3,3,3,
3,3,3,3,3,3,4),(-2.02092030439988E-5,0.000556049295526959,0.0011217165797188,
0.00167096865970714,0.00219205980753922,0.00242674993854338,0.00286892709473989,
0.00328265444055326,0.00359051333580498,0.00399833809851151,0.00437342345628195,
0.00468974844460364,0.00504885723392668,0.00539155487814984,0.0057022315709967,
0.00596953869846673,0.00600761174928926,0.00621566605302231,0.00641489721149064,
0.00660361036059914,0.00661412836995897,0.00681882170159619,0.00701224857467813,
0.00717494882539777,0.007333188837526,0.00739068892409821,0.0075472380430904,
0.00769433317592032,0.00783806436270165,0.00797708941084355,0.008016885400067),
 .UNSPECIFIED.);
#1750=B_SPLINE_CURVE_WITH_KNOTS('',3,(#11116,#11117,#11118,#11119,#11120,
#11121,#11122),.UNSPECIFIED.,.F.,.F.,(4,3,4),(0.,0.000319771717876966,0.000495697630009108),
 .UNSPECIFIED.);
#1751=B_SPLINE_CURVE_WITH_KNOTS('',3,(#11125,#11126,#11127,#11128,#11129,
#11130,#11131),.UNSPECIFIED.,.F.,.F.,(4,3,4),(0.,0.000319771718042548,0.000495697630009101),
 .UNSPECIFIED.);
#1752=B_SPLINE_CURVE_WITH_KNOTS('',3,(#11137,#11138,#11139,#11140,#11141,
#11142,#11143,#11144,#11145,#11146,#11147,#11148,#11149,#11150,#11151,#11152,
#11153,#11154,#11155,#11156,#11157,#11158,#11159,#11160,#11161,#11162,#11163,
#11164,#11165,#11166,#11167,#11168,#11169,#11170,#11171,#11172,#11173,#11174,
#11175,#11176),.UNSPECIFIED.,.F.,.F.,(4,3,3,3,3,3,3,3,3,3,3,3,3,4),(4.33680868994202E-19,
0.000224425374774483,0.000451595406483904,0.000691860819919334,0.000897701499097931,
0.000980242722923433,0.00133024746973674,0.00170122585014586,0.00187037776501358,
0.00196048544584687,0.00235337437521485,0.00279968089622725,0.00329820841760096,
0.00392097089169373),.UNSPECIFIED.);
#1753=B_SPLINE_CURVE_WITH_KNOTS('',3,(#11181,#11182,#11183,#11184,#11185,
#11186,#11187,#11188,#11189,#11190,#11191,#11192,#11193,#11194,#11195,#11196,
#11197,#11198,#11199,#11200,#11201,#11202,#11203,#11204,#11205,#11206,#11207,
#11208,#11209,#11210,#11211,#11212,#11213,#11214,#11215,#11216,#11217,#11218,
#11219,#11220,#11221,#11222,#11223),.UNSPECIFIED.,.F.,.F.,(4,3,3,3,3,3,
3,3,3,3,3,3,3,3,4),(-1.52431972735595E-5,0.000577208203721174,0.00105830978507474,
0.00150240305417916,0.00189185074719465,0.00194649632328358,0.00203665697126435,
0.00241070485831859,0.0027626461229275,0.00292736608356214,0.00300995787129902,
0.00325030870484351,0.00348216857793155,0.00370167549193661,0.00390823584384071),
 .UNSPECIFIED.);
#1754=B_SPLINE_CURVE_WITH_KNOTS('',3,(#11229,#11230,#11231,#11232,#11233,
#11234,#11235,#11236,#11237,#11238,#11239,#11240,#11241,#11242,#11243,#11244,
#11245,#11246,#11247,#11248,#11249,#11250,#11251,#11252,#11253,#11254,#11255,
#11256,#11257,#11258,#11259,#11260,#11261,#11262,#11263,#11264,#11265,#11266,
#11267,#11268),.UNSPECIFIED.,.F.,.F.,(4,3,3,3,3,3,3,3,3,3,3,3,3,4),(0.,
0.000224425374774487,0.000451595406490086,0.000691860819931689,0.000897701499097949,
0.000980242722923432,0.00133024746979985,0.0017012258502438,0.00187037776501362,
0.00196048544584686,0.00235337437512353,0.00279968089602665,0.00329820841722131,
0.00392097089169373),.UNSPECIFIED.);
#1755=B_SPLINE_CURVE_WITH_KNOTS('',3,(#11271,#11272,#11273,#11274,#11275,
#11276,#11277,#11278,#11279,#11280,#11281,#11282,#11283,#11284,#11285,#11286,
#11287,#11288,#11289,#11290,#11291,#11292,#11293,#11294,#11295,#11296,#11297,
#11298,#11299,#11300,#11301,#11302,#11303,#11304,#11305,#11306,#11307,#11308,
#11309,#11310,#11311,#11312,#11313),.UNSPECIFIED.,.F.,.F.,(4,3,3,3,3,3,
3,3,3,3,3,3,3,3,4),(-1.52431972735601E-5,0.000577208204035659,0.00105830978563783,
0.0015024030544607,0.0018918507477027,0.00194649632328357,0.00203665697126436,
0.00241070485830986,0.00276264612288319,0.00292736608356214,0.00300995787129895,
0.00325030870484637,0.00348216857793754,0.00370167549194714,0.0039082358438407),
 .UNSPECIFIED.);
#1756=B_SPLINE_CURVE_WITH_KNOTS('',3,(#11315,#11316,#11317,#11318,#11319,
#11320,#11321,#11322,#11323,#11324,#11325,#11326,#11327,#11328,#11329,#11330,
#11331,#11332,#11333,#11334,#11335,#11336,#11337,#11338,#11339,#11340,#11341,
#11342,#11343,#11344,#11345,#11346,#11347,#11348,#11349,#11350,#11351,#11352),
 .UNSPECIFIED.,.F.,.F.,(4,2,2,2,2,2,2,2,2,2,2,2,2,2,2,2,2,2,4),(2.40199466308743,
2.41022829061081,2.72804014342947,3.05820492223309,3.38252194159165,3.70403954337583,
4.03838990610341,4.3559009458349,4.68115375921356,5.01243500977675,5.32932288323347,
5.65827132582605,5.98518396240259,6.30563559995583,6.63878133247469,6.95731312617532,
7.28146604930193,7.6126886063725,7.65580643120489),.UNSPECIFIED.);
#1757=B_SPLINE_CURVE_WITH_KNOTS('',3,(#11353,#11354,#11355,#11356,#11357,
#11358,#11359,#11360,#11361,#11362,#11363,#11364,#11365,#11366,#11367,#11368,
#11369,#11370,#11371,#11372,#11373,#11374,#11375,#11376,#11377,#11378,#11379,
#11380,#11381,#11382,#11383,#11384,#11385,#11386,#11387,#11388),
 .UNSPECIFIED.,.F.,.F.,(4,2,2,2,2,2,2,2,2,2,2,2,2,2,2,2,2,4),(111.266831993831,
111.546133142784,111.874141801841,112.19080377709,112.52239771137,112.846740900166,
113.165853021345,113.499181039949,113.819822891596,114.147593945405,114.476715222664,
114.793830501138,115.125466606025,115.450893587892,115.768893554885,116.103411184789,
116.425105464923,116.52588314767),.UNSPECIFIED.);
#1758=B_SPLINE_CURVE_WITH_KNOTS('',3,(#11527,#11528,#11529,#11530,#11531,
#11532,#11533,#11534,#11535,#11536,#11537,#11538,#11539,#11540),
 .UNSPECIFIED.,.F.,.F.,(4,2,2,2,2,2,4),(-1.10452810243334,-0.974933410506299,
-0.837207473665695,-0.613047163496973,-0.39375324246162,-0.222767201532269,
-1.00000002589695E-6),.UNSPECIFIED.);
#1759=B_SPLINE_CURVE_WITH_KNOTS('',3,(#11542,#11543,#11544,#11545,#11546,
#11547,#11548,#11549,#11550,#11551,#11552,#11553,#11554,#11555),
 .UNSPECIFIED.,.F.,.F.,(4,2,2,2,2,2,4),(-1.30358759250105,-1.10825126792048,
-0.956598415540384,-0.727542338165497,-0.426865540585114,-0.212508103920413,
-1.35447209004269E-14),.UNSPECIFIED.);
#1760=B_SPLINE_CURVE_WITH_KNOTS('',3,(#11559,#11560,#11561,#11562,#11563,
#11564,#11565,#11566,#11567,#11568,#11569,#11570,#11571,#11572,#11573,#11574,
#11575,#11576),.UNSPECIFIED.,.F.,.F.,(4,2,2,2,2,2,2,2,4),(9.99983121677346E-7,
0.000271322710449146,0.000517114380161633,0.000867591142278511,0.00130908967571248,
0.00208383766110333,0.00540070491534943,0.0164991372137869,0.0397725131276181),
 .UNSPECIFIED.);
#1761=B_SPLINE_CURVE_WITH_KNOTS('',3,(#11577,#11578,#11579,#11580,#11581,
#11582),.UNSPECIFIED.,.F.,.F.,(4,2,4),(0.,0.271067367187735,0.499520314311641),
 .UNSPECIFIED.);
#1762=B_SPLINE_CURVE_WITH_KNOTS('',3,(#11584,#11585,#11586,#11587,#11588,
#11589,#11590,#11591,#11592,#11593,#11594,#11595,#11596,#11597,#11598,#11599),
 .UNSPECIFIED.,.F.,.F.,(4,2,2,2,2,2,2,4),(1.00000001479692E-6,0.262243555324206,
0.507346056711276,0.828287498988696,0.998760751432299,1.30961651062506,
1.47837958130377,1.65229555251206),.UNSPECIFIED.);
#1763=B_SPLINE_CURVE_WITH_KNOTS('',3,(#11600,#11601,#11602,#11603,#11604,
#11605),.UNSPECIFIED.,.F.,.F.,(4,2,4),(0.,0.172721058240164,0.344957068700543),
 .UNSPECIFIED.);
#1764=B_SPLINE_CURVE_WITH_KNOTS('',3,(#11802,#11803,#11804,#11805,#11806,
#11807,#11808,#11809,#11810,#11811,#11812,#11813,#11814,#11815,#11816,#11817,
#11818,#11819,#11820,#11821,#11822,#11823,#11824,#11825,#11826,#11827,#11828,
#11829,#11830,#11831,#11832,#11833,#11834,#11835,#11836,#11837,#11838,#11839,
#11840,#11841),.UNSPECIFIED.,.F.,.F.,(4,3,3,3,3,3,3,3,3,3,3,3,3,4),(-1.31423244832839E-5,
0.000535751919476727,0.00105440309977669,0.00152703982999462,0.00193278669513403,
0.00195362085609606,0.00231730204515171,0.00265300264582922,0.00290575120494268,
0.00292287708750121,0.00323755006403241,0.00353412708051367,0.00381242976596417,
0.00387871571475133),.UNSPECIFIED.);
#1765=B_SPLINE_CURVE_WITH_KNOTS('',3,(#11843,#11844,#11845,#11846,#11847,
#11848,#11849,#11850,#11851,#11852,#11853,#11854,#11855,#11856,#11857,#11858,
#11859,#11860,#11861,#11862,#11863,#11864,#11865,#11866,#11867,#11868,#11869,
#11870,#11871,#11872,#11873,#11874,#11875,#11876,#11877,#11878,#11879,#11880,
#11881,#11882,#11883,#11884,#11885,#11886,#11887,#11888,#11889,#11890,#11891,
#11892,#11893,#11894,#11895,#11896,#11897,#11898,#11899,#11900,#11901,#11902,
#11903,#11904,#11905,#11906,#11907,#11908,#11909,#11910,#11911,#11912,#11913,
#11914,#11915,#11916,#11917,#11918,#11919,#11920,#11921),.UNSPECIFIED.,
 .F.,.F.,(4,3,3,3,3,3,3,3,3,3,3,3,3,3,3,3,3,3,3,3,3,3,3,3,3,3,4),(8.67361737988404E-19,
0.000202743010865249,0.000410514286400591,0.000626630076752085,0.000743751984502465,
0.000896895697750054,0.00116850905342267,0.00144756822847459,0.00154043258165819,
0.00179379139550011,0.00205677592735176,0.00233242599985497,0.00239862131095936,
0.00272711606086079,0.00307220744579522,0.003305634398149,0.00358758279100021,
0.00401837140737556,0.00424614693708929,0.00468203334964349,0.00515625220928118,
0.00521101431097261,0.00538137418650031,0.0060186616833771,0.00627826988425036,
0.00676573329680739,0.00717516558200042),.UNSPECIFIED.);
#1766=B_SPLINE_CURVE_WITH_KNOTS('',3,(#11925,#11926,#11927,#11928,#11929,
#11930,#11931,#11932,#11933,#11934,#11935,#11936,#11937,#11938,#11939,#11940,
#11941,#11942,#11943,#11944,#11945,#11946,#11947,#11948,#11949,#11950,#11951,
#11952,#11953,#11954,#11955,#11956,#11957,#11958,#11959,#11960,#11961,#11962,
#11963,#11964),.UNSPECIFIED.,.F.,.F.,(4,3,3,3,3,3,3,3,3,3,3,3,3,4),(4.33680868994202E-19,
0.000280621540973947,0.000573887525893564,0.000891635349190541,0.000951755207402115,
0.000968821950376569,0.00129993329989977,0.00165663590864014,0.00191687066807321,
0.00193764390075314,0.00253097521482023,0.00313046488108132,0.00374040674088882,
0.00387528780150628),.UNSPECIFIED.);
#1767=B_SPLINE_CURVE_WITH_KNOTS('',3,(#11965,#11966,#11967,#11968,#11969,
#11970,#11971,#11972,#11973,#11974,#11975,#11976,#11977,#11978,#11979,#11980,
#11981,#11982,#11983,#11984,#11985,#11986,#11987,#11988,#11989,#11990,#11991,
#11992,#11993,#11994,#11995,#11996,#11997,#11998,#11999,#12000,#12001,#12002,
#12003,#12004,#12005,#12006,#12007,#12008,#12009,#12010,#12011,#12012,#12013,
#12014,#12015,#12016,#12017,#12018,#12019,#12020,#12021,#12022,#12023,#12024,
#12025,#12026,#12027,#12028,#12029,#12030,#12031,#12032,#12033,#12034,#12035,
#12036,#12037,#12038,#12039,#12040),.UNSPECIFIED.,.F.,.F.,(4,3,3,3,3,3,
3,3,3,3,3,3,3,3,3,3,3,3,3,3,3,3,3,3,3,4),(-1.48622659852799E-5,0.000610199395319616,
0.00119886177892042,0.00174545418326133,0.00178752416252122,0.00196068261362535,
0.00248416090974261,0.00298752987926026,0.00346663178416926,0.00358991059102772,
0.00387008960346663,0.0042497114937252,0.00449110380528096,0.00477985713902406,
0.00508715459760339,0.00539229701953421,0.00564558051974503,0.00589575931921666,
0.00613544593423836,0.00629349023378746,0.00645448223380467,0.00664036590499829,
0.00682033260015863,0.006994867143252,0.00716251291548491,0.00719468344804071),
 .UNSPECIFIED.);
#1768=B_SPLINE_CURVE_WITH_KNOTS('',3,(#12043,#12044,#12045,#12046,#12047,
#12048,#12049,#12050,#12051,#12052,#12053,#12054,#12055,#12056,#12057,#12058,
#12059,#12060,#12061,#12062,#12063,#12064,#12065,#12066,#12067,#12068,#12069,
#12070,#12071,#12072,#12073,#12074,#12075,#12076,#12077,#12078,#12079,#12080,
#12081,#12082),.UNSPECIFIED.,.F.,.F.,(4,3,3,3,3,3,3,3,3,3,3,3,3,4),(-1.31423244832953E-5,
0.000535751918458696,0.00105440310099963,0.00152703983355165,0.00193278669513403,
0.00195362085609607,0.00231730204521729,0.00265300264592743,0.00290575120494269,
0.00292287708750123,0.00323755006402069,0.00353412708048685,0.00381242976591801,
0.00387871571475135),.UNSPECIFIED.);
#1769=B_SPLINE_CURVE_WITH_KNOTS('',3,(#12084,#12085,#12086,#12087,#12088,
#12089,#12090,#12091,#12092,#12093,#12094,#12095,#12096,#12097,#12098,#12099,
#12100,#12101,#12102,#12103,#12104,#12105,#12106,#12107,#12108,#12109,#12110,
#12111,#12112,#12113,#12114,#12115,#12116,#12117,#12118,#12119,#12120,#12121,
#12122,#12123,#12124,#12125,#12126,#12127,#12128,#12129,#12130,#12131,#12132,
#12133,#12134,#12135,#12136,#12137,#12138,#12139,#12140,#12141,#12142,#12143,
#12144,#12145,#12146,#12147,#12148,#12149,#12150,#12151,#12152,#12153,#12154,
#12155,#12156,#12157,#12158,#12159,#12160,#12161,#12162),.UNSPECIFIED.,
 .F.,.F.,(4,3,3,3,3,3,3,3,3,3,3,3,3,3,3,3,3,3,3,3,3,3,3,3,3,3,4),(0.,0.000202743010861385,
0.000410514286393132,0.000626630076741744,0.000743751984502566,0.000896895697750052,
0.00116850905341496,0.00144756822846688,0.00154043258165826,0.0017937913955001,
0.00205677592735273,0.00233242599985535,0.00239862131095943,0.00272711606085617,
0.00307220744578745,0.00330563439814887,0.00358758279100021,0.00401837140748574,
0.00424614693708857,0.0046820333497003,0.0051562522094217,0.00521101431097235,
0.00538137418650031,0.00601866167817585,0.00627826988425036,0.00676573329750569,
0.00717516558200041),.UNSPECIFIED.);
#1770=B_SPLINE_CURVE_WITH_KNOTS('',3,(#12166,#12167,#12168,#12169,#12170,
#12171,#12172,#12173,#12174,#12175,#12176,#12177,#12178,#12179,#12180,#12181,
#12182,#12183,#12184,#12185,#12186,#12187,#12188,#12189,#12190,#12191,#12192,
#12193,#12194,#12195,#12196,#12197,#12198,#12199,#12200,#12201,#12202,#12203,
#12204,#12205),.UNSPECIFIED.,.F.,.F.,(4,3,3,3,3,3,3,3,3,3,3,3,3,4),(8.67361737988404E-19,
0.000280621540991916,0.000573887525927214,0.000891635349236454,0.000951755207402113,
0.000968821950376574,0.00129993329989704,0.00165663590861034,0.00191687066807323,
0.00193764390075315,0.00253097520314591,0.00313046485777404,0.0037404067077475,
0.00387528780150629),.UNSPECIFIED.);
#1771=B_SPLINE_CURVE_WITH_KNOTS('',3,(#12206,#12207,#12208,#12209,#12210,
#12211,#12212,#12213,#12214,#12215,#12216,#12217,#12218,#12219,#12220,#12221,
#12222,#12223,#12224,#12225,#12226,#12227,#12228,#12229,#12230,#12231,#12232,
#12233,#12234,#12235,#12236,#12237,#12238,#12239,#12240,#12241,#12242,#12243,
#12244,#12245,#12246,#12247,#12248,#12249,#12250,#12251,#12252,#12253,#12254,
#12255,#12256,#12257,#12258,#12259,#12260,#12261,#12262,#12263,#12264,#12265,
#12266,#12267,#12268,#12269,#12270,#12271,#12272,#12273,#12274,#12275,#12276,
#12277,#12278,#12279,#12280,#12281),.UNSPECIFIED.,.F.,.F.,(4,3,3,3,3,3,
3,3,3,3,3,3,3,3,3,3,3,3,3,3,3,3,3,3,3,4),(-1.48622659852334E-5,0.000610199394906132,
0.00119886177871369,0.00174545418209242,0.00178752416252126,0.0019606826136253,
0.00248416090948471,0.00298752987876159,0.00346663178346203,0.00358991059102774,
0.00387008960346665,0.0042497114937369,0.00449110380528099,0.00477985713902429,
0.00508715459758098,0.00539229701953424,0.0056455805197453,0.00589575931922801,
0.00613544593426095,0.00629349023378748,0.00645448223380473,0.00664036590499971,
0.00682033260016142,0.00699486714325674,0.00716251291549094,0.00719468344804073),
 .UNSPECIFIED.);
#1772=B_SPLINE_CURVE_WITH_KNOTS('',3,(#12284,#12285,#12286,#12287,#12288,
#12289,#12290,#12291,#12292,#12293,#12294,#12295,#12296,#12297,#12298,#12299,
#12300,#12301,#12302,#12303,#12304,#12305,#12306,#12307,#12308,#12309,#12310,
#12311,#12312,#12313,#12314,#12315,#12316,#12317,#12318,#12319,#12320,#12321,
#12322,#12323),.UNSPECIFIED.,.F.,.F.,(4,3,3,3,3,3,3,3,3,3,3,3,3,4),(-1.31423244832926E-5,
0.000535751919828975,0.00105440309942062,0.00152703982893435,0.00193278669513403,
0.00195362085609607,0.0023173020450886,0.00265300264570622,0.00290575120494269,
0.00292287708750123,0.00323755006398503,0.00353412708041696,0.00381242976581613,
0.00387871571475135),.UNSPECIFIED.);
#1773=B_SPLINE_CURVE_WITH_KNOTS('',3,(#12325,#12326,#12327,#12328,#12329,
#12330,#12331,#12332,#12333,#12334,#12335,#12336,#12337,#12338,#12339,#12340,
#12341,#12342,#12343,#12344,#12345,#12346,#12347,#12348,#12349,#12350,#12351,
#12352,#12353,#12354,#12355,#12356,#12357,#12358,#12359,#12360,#12361,#12362,
#12363,#12364,#12365,#12366,#12367,#12368,#12369,#12370,#12371,#12372,#12373,
#12374,#12375,#12376,#12377,#12378,#12379,#12380,#12381,#12382,#12383,#12384,
#12385,#12386,#12387,#12388,#12389,#12390,#12391,#12392,#12393,#12394,#12395,
#12396,#12397,#12398,#12399,#12400,#12401,#12402,#12403),.UNSPECIFIED.,
 .F.,.F.,(4,3,3,3,3,3,3,3,3,3,3,3,3,3,3,3,3,3,3,3,3,3,3,3,3,3,4),(4.33680868994202E-19,
0.00020274301087834,0.000410514286426467,0.0006266300767902,0.000743751984502697,
0.000896895697750054,0.00116850905345097,0.00144756822853142,0.0015404325816583,
0.00179379139550011,0.0020567759273478,0.00233242599984708,0.00239862131095955,
0.0027271160608669,0.00307220744580637,0.003305634398149,0.00358758279100022,
0.00401837140744728,0.00424614693708873,0.00468203334971685,0.00515625220941641,
0.00521101431097258,0.00538137418650032,0.00601866168041985,0.00627826988425037,
0.00676573329696348,0.00717516558200042),.UNSPECIFIED.);
#1774=B_SPLINE_CURVE_WITH_KNOTS('',3,(#12407,#12408,#12409,#12410,#12411,
#12412,#12413,#12414,#12415,#12416,#12417,#12418,#12419,#12420,#12421,#12422,
#12423,#12424,#12425,#12426,#12427,#12428,#12429,#12430,#12431,#12432,#12433,
#12434,#12435,#12436,#12437,#12438,#12439,#12440,#12441,#12442,#12443,#12444,
#12445,#12446),.UNSPECIFIED.,.F.,.F.,(4,3,3,3,3,3,3,3,3,3,3,3,3,4),(0.,
0.000280621541007288,0.000573887525957151,0.000891635349279514,0.000951755207402121,
0.000968821950376574,0.00129993329992634,0.00165663590867474,0.00191687066807322,
0.00193764390075315,0.00253097521731032,0.00313046488602104,0.00374040674787271,
0.00387528780150629),.UNSPECIFIED.);
#1775=B_SPLINE_CURVE_WITH_KNOTS('',3,(#12447,#12448,#12449,#12450,#12451,
#12452,#12453,#12454,#12455,#12456,#12457,#12458,#12459,#12460,#12461,#12462,
#12463,#12464,#12465,#12466,#12467,#12468,#12469,#12470,#12471,#12472,#12473,
#12474,#12475,#12476,#12477,#12478,#12479,#12480,#12481,#12482,#12483,#12484,
#12485,#12486,#12487,#12488,#12489,#12490,#12491,#12492,#12493,#12494,#12495,
#12496,#12497,#12498,#12499,#12500,#12501,#12502,#12503,#12504,#12505,#12506,
#12507,#12508,#12509,#12510,#12511,#12512,#12513,#12514,#12515,#12516,#12517,
#12518,#12519,#12520,#12521,#12522),.UNSPECIFIED.,.F.,.F.,(4,3,3,3,3,3,
3,3,3,3,3,3,3,3,3,3,3,3,3,3,3,3,3,3,3,4),(-1.48622659852434E-5,0.000610199394349477,
0.00119886177843536,0.00174545418627758,0.00178752416252125,0.00196068261362537,
0.00248416090955126,0.00298752987889132,0.00346663178364606,0.00358991059102774,
0.00387008960346671,0.00424971149374217,0.00449110380528099,0.00477985713902425,
0.00508715459758174,0.00539229701953423,0.0056455805197453,0.00589575931922186,
0.00613544593424759,0.00629349023378747,0.00645448223380475,0.00664036590499189,
0.00682033260014577,0.00699486714323308,0.00716251291545963,0.00719468344804072),
 .UNSPECIFIED.);
#1776=B_SPLINE_CURVE_WITH_KNOTS('',3,(#12524,#12525,#12526,#12527,#12528,
#12529,#12530,#12531,#12532,#12533,#12534,#12535,#12536,#12537,#12538,#12539,
#12540,#12541,#12542,#12543,#12544,#12545,#12546,#12547,#12548,#12549,#12550,
#12551,#12552,#12553,#12554,#12555,#12556,#12557,#12558,#12559,#12560,#12561,
#12562,#12563,#12564,#12565,#12566),.UNSPECIFIED.,.F.,.F.,(4,3,3,3,3,3,
3,3,3,3,3,3,3,3,4),(-1.52431972734697E-5,0.000577208204163697,0.00105830978603858,
0.00150240305466112,0.00189185074812808,0.00194649632328366,0.00203665697126444,
0.00241070485830692,0.00276264612286663,0.00292736608356222,0.00300995787129907,
0.0032503087048446,0.00348216857793395,0.00370167549194112,0.00390823584384079),
 .UNSPECIFIED.);
#1777=B_SPLINE_CURVE_WITH_KNOTS('',3,(#12567,#12568,#12569,#12570,#12571,
#12572,#12573,#12574,#12575,#12576,#12577,#12578,#12579,#12580,#12581,#12582,
#12583,#12584,#12585,#12586,#12587,#12588,#12589,#12590,#12591,#12592,#12593,
#12594,#12595,#12596,#12597,#12598,#12599,#12600,#12601,#12602,#12603,#12604,
#12605,#12606),.UNSPECIFIED.,.F.,.F.,(4,3,3,3,3,3,3,3,3,3,3,3,3,4),(0.,
0.000224425374774488,0.000451595406488995,0.000691860819929039,0.000897701499097952,
0.000980242722923431,0.00133024746974078,0.00170122585016282,0.00187037776501363,
0.00196048544584686,0.00235337437541891,0.00279968089665459,0.00329820841838201,
0.00392097089169372),.UNSPECIFIED.);
#1778=B_SPLINE_CURVE_WITH_KNOTS('',3,(#12609,#12610,#12611,#12612,#12613,
#12614,#12615,#12616,#12617,#12618,#12619,#12620,#12621,#12622,#12623,#12624,
#12625,#12626,#12627,#12628,#12629,#12630,#12631,#12632,#12633,#12634,#12635,
#12636,#12637,#12638,#12639,#12640,#12641,#12642,#12643,#12644,#12645,#12646,
#12647,#12648,#12649,#12650,#12651,#12652,#12653,#12654,#12655,#12656,#12657,
#12658,#12659,#12660,#12661,#12662,#12663,#12664,#12665,#12666,#12667,#12668,
#12669,#12670,#12671,#12672,#12673,#12674,#12675,#12676,#12677,#12678,#12679,
#12680,#12681,#12682,#12683,#12684,#12685,#12686,#12687,#12688,#12689,#12690,
#12691,#12692,#12693,#12694,#12695,#12696,#12697,#12698,#12699),
 .UNSPECIFIED.,.F.,.F.,(4,3,3,3,3,3,3,3,3,3,3,3,3,3,3,3,3,3,3,3,3,3,3,3,
3,3,3,3,3,3,4),(-2.02092030442042E-5,0.000556049295986959,0.00112171658044497,
0.00167096866058992,0.00219205980848149,0.00242674993854397,0.00286892709477413,
0.0032826544405976,0.00359051333580462,0.0039983380985113,0.00437342345626924,
0.00468974844460317,0.00504885723393916,0.00539155487817727,0.00570223157099643,
0.00596953869846973,0.00600761174928905,0.00621566605302244,0.00641489721149056,
0.00660361036060121,0.00661412836995868,0.00681882170158418,0.00701224857467793,
0.00717494882538604,0.00733318883750038,0.00739068892409895,0.00754723804309091,
0.00769433317590785,0.00783806436267558,0.00797708941080271,0.0080168854000668),
 .UNSPECIFIED.);
#1779=B_SPLINE_CURVE_WITH_KNOTS('',3,(#12700,#12701,#12702,#12703,#12704,
#12705,#12706),.UNSPECIFIED.,.F.,.F.,(4,3,4),(0.,0.000319771717937602,0.000495697630009084),
 .UNSPECIFIED.);
#1780=B_SPLINE_CURVE_WITH_KNOTS('',3,(#12708,#12709,#12710,#12711,#12712,
#12713,#12714),.UNSPECIFIED.,.F.,.F.,(4,3,4),(0.,0.000319771717612993,0.000495697630009086),
 .UNSPECIFIED.);
#1781=B_SPLINE_CURVE_WITH_KNOTS('',3,(#12715,#12716,#12717,#12718,#12719,
#12720,#12721,#12722,#12723,#12724,#12725,#12726,#12727,#12728,#12729,#12730,
#12731,#12732,#12733,#12734,#12735,#12736,#12737,#12738,#12739,#12740,#12741,
#12742,#12743,#12744,#12745,#12746,#12747,#12748,#12749,#12750,#12751,#12752,
#12753,#12754,#12755,#12756,#12757,#12758,#12759,#12760,#12761,#12762,#12763,
#12764,#12765,#12766,#12767,#12768,#12769,#12770,#12771,#12772,#12773,#12774,
#12775,#12776,#12777,#12778,#12779,#12780,#12781,#12782,#12783,#12784,#12785,
#12786,#12787,#12788,#12789,#12790,#12791,#12792,#12793,#12794,#12795,#12796,
#12797,#12798,#12799,#12800,#12801,#12802,#12803,#12804,#12805),
 .UNSPECIFIED.,.F.,.F.,(4,3,3,3,3,3,3,3,3,3,3,3,3,3,3,3,3,3,3,3,3,3,3,3,
3,3,3,3,3,3,4),(0.,0.000104117546061403,0.000212237259616963,0.000327080569137136,
0.000446149861995263,0.000572039848833935,0.000627770356649805,0.0007725910708947,
0.000921601146177619,0.00100643629586967,0.00123003713212734,0.00141082154631894,
0.00163414234169981,0.00186714353407499,0.00201287259173934,0.00230575771617008,
0.00232230404187754,0.00265209606179006,0.00299833864625774,0.00334106762005192,
0.00370526339370595,0.00402574518347867,0.00448446651998587,0.0049581923982794,
0.00545452540823567,0.00560736333266499,0.00603861777521801,0.00657098900349448,
0.00713145773781003,0.00771983125198687,0.00805149036695735),
 .UNSPECIFIED.);
#1782=B_SPLINE_CURVE_WITH_KNOTS('',3,(#12808,#12809,#12810,#12811,#12812,
#12813,#12814),.UNSPECIFIED.,.F.,.F.,(4,3,4),(4.9065389333868E-18,0.000319771718109916,
0.000495697630009092),.UNSPECIFIED.);
#1783=B_SPLINE_CURVE_WITH_KNOTS('',3,(#12815,#12816,#12817,#12818,#12819,
#12820,#12821,#12822,#12823,#12824,#12825,#12826,#12827,#12828,#12829,#12830,
#12831,#12832,#12833,#12834,#12835,#12836,#12837,#12838,#12839,#12840,#12841,
#12842,#12843,#12844,#12845,#12846,#12847,#12848,#12849,#12850,#12851,#12852,
#12853,#12854,#12855,#12856,#12857,#12858,#12859,#12860,#12861,#12862,#12863,
#12864,#12865,#12866,#12867,#12868,#12869,#12870,#12871,#12872,#12873,#12874,
#12875,#12876,#12877,#12878,#12879,#12880,#12881,#12882,#12883,#12884,#12885,
#12886,#12887,#12888,#12889,#12890,#12891,#12892,#12893,#12894,#12895,#12896,
#12897,#12898,#12899,#12900,#12901,#12902,#12903,#12904,#12905),
 .UNSPECIFIED.,.F.,.F.,(4,3,3,3,3,3,3,3,3,3,3,3,3,3,3,3,3,3,3,3,3,3,3,3,
3,3,3,3,3,3,4),(0.,0.000104117546066811,0.000212237259628058,0.000327080569154219,
0.000446149862018597,0.000572039848863917,0.000627770356652624,0.000772591070908048,
0.00092160114620273,0.00100643629586967,0.00123003713212771,0.00141082154631876,
0.00163414234169305,0.00186714353406425,0.00201287259173934,0.00230575771615584,
0.00232230404187742,0.00265209606176781,0.0029983386462177,0.00334106762005204,
0.0037052633937103,0.00402574518347868,0.00448446651999,0.00495819239828445,
0.00545452540823168,0.00560736333266521,0.00603861777521801,0.00657098900708674,
0.00713145774710329,0.00771983127025435,0.00805149036695735),
 .UNSPECIFIED.);
#1784=B_SPLINE_CURVE_WITH_KNOTS('',3,(#12907,#12908,#12909,#12910,#12911,
#12912,#12913,#12914,#12915,#12916,#12917,#12918,#12919,#12920,#12921,#12922,
#12923,#12924,#12925,#12926,#12927,#12928,#12929,#12930,#12931,#12932,#12933,
#12934,#12935,#12936,#12937,#12938,#12939,#12940,#12941,#12942,#12943,#12944,
#12945,#12946,#12947,#12948,#12949,#12950,#12951,#12952,#12953,#12954,#12955,
#12956,#12957,#12958,#12959,#12960,#12961,#12962,#12963,#12964,#12965,#12966,
#12967,#12968,#12969,#12970,#12971,#12972,#12973,#12974,#12975,#12976,#12977,
#12978,#12979,#12980,#12981,#12982,#12983,#12984,#12985,#12986,#12987,#12988,
#12989,#12990,#12991,#12992,#12993,#12994,#12995,#12996,#12997),
 .UNSPECIFIED.,.F.,.F.,(4,3,3,3,3,3,3,3,3,3,3,3,3,3,3,3,3,3,3,3,3,3,3,3,
3,3,3,3,3,3,4),(-2.02092030439489E-5,0.0005560492961748,0.00112171658075715,
0.00167096866098397,0.00219205980893471,0.00242674993854208,0.00286892709480559,
0.00328265444065681,0.00359051333580469,0.00399833809851155,0.0043734234562713,
0.00468974844460377,0.00504885723393179,0.00539155487816009,0.00570223157099668,
0.00596953869847231,0.0060076117492893,0.00621566605302207,0.00641489721149059,
0.00660361036059884,0.00661412836995911,0.0068188217015917,0.00701224857467817,
0.00717494882540412,0.00733318883753838,0.00739068892409721,0.00754723804308967,
0.0076943331759223,0.00783806436270549,0.0079770894108481,0.00801688540006705),
 .UNSPECIFIED.);
#1785=B_SPLINE_CURVE_WITH_KNOTS('',3,(#12998,#12999,#13000,#13001,#13002,
#13003,#13004),.UNSPECIFIED.,.F.,.F.,(4,3,4),(0.,0.000319771717956473,0.00049569763000909),
 .UNSPECIFIED.);
#1786=B_SPLINE_CURVE_WITH_KNOTS('',3,(#13007,#13008,#13009,#13010,#13011,
#13012),.UNSPECIFIED.,.F.,.F.,(4,2,4),(-0.142729181026185,-0.071107498865174,
-1.0000000814081E-6),.UNSPECIFIED.);
#1787=B_SPLINE_CURVE_WITH_KNOTS('',3,(#13014,#13015,#13016,#13017,#13018,
#13019,#13020,#13021,#13022,#13023,#13024,#13025,#13026,#13027,#13028,#13029),
 .UNSPECIFIED.,.F.,.F.,(4,2,2,2,2,2,2,4),(-2.43104855077894,-1.90349401615095,
-1.45644570848823,-1.0906282720009,-0.723808102624486,-0.376722226194699,
-0.186648168518619,0.),.UNSPECIFIED.);
#1788=B_SPLINE_CURVE_WITH_KNOTS('',3,(#13031,#13032,#13033,#13034,#13035,
#13036,#13037,#13038,#13039,#13040,#13041,#13042,#13043,#13044,#13045,#13046),
 .UNSPECIFIED.,.F.,.F.,(4,2,2,2,2,2,2,4),(-1.61608002817239,-1.45775061306008,
-1.2995571050224,-1.06365376510753,-0.82576780359447,-0.617872986252087,
-0.355668197463031,0.),.UNSPECIFIED.);
#1789=B_SPLINE_CURVE_WITH_KNOTS('',3,(#13047,#13048,#13049,#13050,#13051,
#13052),.UNSPECIFIED.,.F.,.F.,(4,2,4),(-0.152773347352654,-0.0766837717947395,
0.),.UNSPECIFIED.);
#1790=B_SPLINE_CURVE_WITH_KNOTS('',3,(#25576,#25577,#25578,#25579,#25580,
#25581,#25582,#25583,#25584,#25585),.UNSPECIFIED.,.F.,.F.,(4,2,2,2,4),(0.263724731228934,
0.278450074781171,0.366228167882972,0.454006260984773,0.46873160453701),
 .UNSPECIFIED.);
#1791=B_SPLINE_CURVE_WITH_KNOTS('',3,(#25587,#25588,#25589,#25590,#25591,
#25592,#25593,#25594,#25595,#25596),.UNSPECIFIED.,.F.,.F.,(4,2,2,2,4),(0.263724731228934,
0.27845007478117,0.366228167882972,0.454006260984773,0.468731604537009),
 .UNSPECIFIED.);
#1792=B_SPLINE_CURVE_WITH_KNOTS('',3,(#25598,#25599,#25600,#25601,#25602,
#25603,#25604,#25605,#25606,#25607),.UNSPECIFIED.,.F.,.F.,(4,2,2,2,4),(0.263724731228934,
0.27845007478117,0.366228167882972,0.454006260984773,0.468731604537009),
 .UNSPECIFIED.);
#1793=B_SPLINE_CURVE_WITH_KNOTS('',3,(#25609,#25610,#25611,#25612,#25613,
#25614,#25615,#25616,#25617,#25618),.UNSPECIFIED.,.F.,.F.,(4,2,2,2,4),(0.263724731228934,
0.27845007478117,0.366228167882972,0.454006260984773,0.46873160453701),
 .UNSPECIFIED.);
#1794=B_SPLINE_CURVE_WITH_KNOTS('',3,(#25620,#25621,#25622,#25623,#25624,
#25625,#25626,#25627,#25628,#25629),.UNSPECIFIED.,.F.,.F.,(4,2,2,2,4),(0.263724731228934,
0.278450074781171,0.366228167882972,0.454006260984773,0.46873160453701),
 .UNSPECIFIED.);
#1795=B_SPLINE_CURVE_WITH_KNOTS('',3,(#25631,#25632,#25633,#25634,#25635,
#25636,#25637,#25638,#25639,#25640),.UNSPECIFIED.,.F.,.F.,(4,2,2,2,4),(0.263724731228934,
0.27845007478117,0.366228167882972,0.454006260984773,0.46873160453701),
 .UNSPECIFIED.);
#1796=B_SPLINE_CURVE_WITH_KNOTS('',3,(#25683,#25684,#25685,#25686,#25687,
#25688,#25689,#25690,#25691,#25692,#25693,#25694,#25695,#25696,#25697,#25698,
#25699,#25700,#25701,#25702,#25703,#25704,#25705,#25706,#25707,#25708,#25709,
#25710,#25711,#25712,#25713,#25714,#25715,#25716,#25717,#25718,#25719,#25720,
#25721,#25722,#25723,#25724,#25725,#25726,#25727,#25728,#25729,#25730,#25731,
#25732,#25733,#25734,#25735,#25736,#25737,#25738,#25739,#25740,#25741,#25742,
#25743,#25744,#25745,#25746,#25747,#25748,#25749,#25750,#25751,#25752),
 .UNSPECIFIED.,.F.,.F.,(4,3,3,3,3,3,3,3,3,3,3,3,3,3,3,3,3,3,3,3,3,3,3,4),
(3.14159265358979,3.21339939141241,3.28586680785268,3.35121436883213,3.42308378055159,
3.49600214093481,3.54876098024507,3.62076596894727,3.69731507009814,3.77134555075139,
3.84915396215108,3.92696237355076,4.00138616900808,4.07733349290367,4.15127434963696,
4.2282249071137,4.30037597555225,4.30517546459045,4.37937215290707,4.45279559418716,
4.52509277844413,4.59683140040149,4.66795343860946,4.71238898038469),
 .UNSPECIFIED.);
#1797=B_SPLINE_CURVE_WITH_KNOTS('',3,(#25789,#25790,#25791,#25792,#25793,
#25794,#25795,#25796,#25797,#25798,#25799,#25800,#25801,#25802,#25803,#25804,
#25805,#25806,#25807,#25808,#25809,#25810,#25811,#25812,#25813,#25814,#25815,
#25816,#25817,#25818,#25819,#25820,#25821,#25822,#25823,#25824,#25825,#25826,
#25827,#25828,#25829,#25830,#25831,#25832,#25833,#25834,#25835,#25836,#25837,
#25838,#25839,#25840,#25841,#25842,#25843,#25844,#25845,#25846,#25847,#25848,
#25849,#25850,#25851,#25852,#25853,#25854,#25855,#25856,#25857,#25858),
 .UNSPECIFIED.,.F.,.F.,(4,3,3,3,3,3,3,3,3,3,3,3,3,3,3,3,3,3,3,3,3,3,3,4),
(3.14159265358979,3.21339939141199,3.28586680785193,3.35121436883206,3.42308378055094,
3.49600214093364,3.54876098024493,3.62076596894664,3.69731507009761,3.77134555075049,
3.84915396215049,3.92696237355049,4.00138616900755,4.0773334929032,4.15127434963635,
4.22822490711326,4.30037597555205,4.30517546459017,4.37937215290745,4.4527955941884,
4.52509277844676,4.59683140040586,4.6679534386157,4.71238898038469),
 .UNSPECIFIED.);
#1798=B_SPLINE_CURVE_WITH_KNOTS('',3,(#25922,#25923,#25924,#25925,#25926,
#25927,#25928,#25929,#25930,#25931,#25932,#25933,#25934,#25935,#25936,#25937,
#25938,#25939,#25940,#25941,#25942,#25943,#25944,#25945,#25946,#25947,#25948,
#25949,#25950,#25951,#25952,#25953,#25954,#25955,#25956,#25957,#25958,#25959,
#25960,#25961,#25962,#25963,#25964,#25965,#25966,#25967,#25968,#25969,#25970,
#25971,#25972,#25973,#25974,#25975,#25976,#25977,#25978,#25979,#25980,#25981,
#25982,#25983,#25984,#25985,#25986,#25987,#25988,#25989,#25990,#25991),
 .UNSPECIFIED.,.F.,.F.,(4,3,3,3,3,3,3,3,3,3,3,3,3,3,3,3,3,3,3,3,3,3,3,4),
(1.5707963267949,1.64187501429286,1.71337342981178,1.78582694190062,1.8589079472425,
1.93301112893021,1.9780098425893,2.05029693877859,2.12677843749119,2.20103698011073,
2.27862995686985,2.35622293362897,2.43057368240882,2.50653634354026,2.58022474803207,
2.65321980989102,2.72512224828116,2.73442432693459,2.80750100759831,2.87952975922344,
2.93197093834749,3.00457650346194,3.07649190731354,3.14159265358979),
 .UNSPECIFIED.);
#1799=B_SPLINE_CURVE_WITH_KNOTS('',3,(#26028,#26029,#26030,#26031,#26032,
#26033,#26034,#26035,#26036,#26037,#26038,#26039,#26040,#26041,#26042,#26043,
#26044,#26045,#26046,#26047,#26048,#26049,#26050,#26051,#26052,#26053,#26054,
#26055,#26056,#26057,#26058,#26059,#26060,#26061,#26062,#26063,#26064,#26065,
#26066,#26067,#26068,#26069,#26070,#26071,#26072,#26073,#26074,#26075,#26076,
#26077,#26078,#26079,#26080,#26081,#26082,#26083,#26084,#26085,#26086,#26087,
#26088,#26089,#26090,#26091,#26092,#26093,#26094,#26095,#26096,#26097),
 .UNSPECIFIED.,.F.,.F.,(4,3,3,3,3,3,3,3,3,3,3,3,3,3,3,3,3,3,3,3,3,3,3,4),
(1.5707963267949,1.64187501429421,1.71337342981444,1.78582694190426,1.85890794724695,
1.93301112893518,1.97800984258945,2.05029693877866,2.12677843749128,2.20103698011052,
2.27862995686982,2.35622293362912,2.43057368240835,2.50653634353993,2.5802247480312,
2.65321980988953,2.7251222482791,2.73442432693468,2.80750100759807,2.8795297592228,
2.93197093834753,3.00457650346134,3.07649190731224,3.14159265358979),
 .UNSPECIFIED.);
#1800=B_SPLINE_CURVE_WITH_KNOTS('',3,(#26167,#26168,#26169,#26170,#26171,
#26172,#26173,#26174,#26175,#26176,#26177,#26178,#26179,#26180,#26181,#26182,
#26183,#26184,#26185,#26186,#26187,#26188,#26189,#26190,#26191,#26192,#26193,
#26194,#26195,#26196,#26197,#26198,#26199,#26200,#26201,#26202,#26203,#26204,
#26205,#26206,#26207,#26208,#26209,#26210,#26211,#26212,#26213,#26214,#26215,
#26216,#26217,#26218,#26219,#26220,#26221,#26222,#26223,#26224,#26225,#26226,
#26227,#26228,#26229,#26230,#26231,#26232,#26233,#26234,#26235,#26236),
 .UNSPECIFIED.,.F.,.F.,(4,3,3,3,3,3,3,3,3,3,3,3,3,3,3,3,3,3,3,3,3,3,3,4),
(1.5707963267949,1.64187501429494,1.7133734298158,1.78582694190613,1.85890794724926,
1.93301112893768,1.97800984258967,2.0502969387789,2.1267784374915,2.20103698011077,
2.27862995687003,2.35622293362928,2.43057368240896,2.50653634354039,2.58022474803194,
2.65321980989038,2.72512224827995,2.7344243269347,2.80750100759699,2.87952975922006,
2.93197093834751,3.00457650346208,3.07649190731386,3.14159265358979),
 .UNSPECIFIED.);
#1801=B_SPLINE_CURVE_WITH_KNOTS('',3,(#26273,#26274,#26275,#26276,#26277,
#26278,#26279,#26280,#26281,#26282,#26283,#26284,#26285,#26286,#26287,#26288,
#26289,#26290,#26291,#26292,#26293,#26294,#26295,#26296,#26297,#26298,#26299,
#26300,#26301,#26302,#26303,#26304,#26305,#26306,#26307,#26308,#26309,#26310,
#26311,#26312,#26313,#26314,#26315,#26316,#26317,#26318,#26319,#26320,#26321,
#26322,#26323,#26324,#26325,#26326,#26327,#26328,#26329,#26330,#26331,#26332,
#26333,#26334,#26335,#26336,#26337,#26338,#26339,#26340,#26341,#26342),
 .UNSPECIFIED.,.F.,.F.,(4,3,3,3,3,3,3,3,3,3,3,3,3,3,3,3,3,3,3,3,3,3,3,4),
(1.5707963267949,1.64187501429417,1.71337342981437,1.7858269419042,1.85890794724684,
1.9330111289351,1.97800984258951,2.05029693877879,2.12677843749138,2.20103698011076,
2.27862995686996,2.35622293362916,2.43057368240866,2.50653634354016,2.58022474803158,
2.6532198098899,2.72512224827938,2.73442432693467,2.80750100759708,2.87952975922029,
2.93197093834752,3.00457650346242,3.07649190731442,3.14159265358979),
 .UNSPECIFIED.);
#1802=B_SPLINE_CURVE_WITH_KNOTS('',3,(#26463,#26464,#26465,#26466,#26467,
#26468,#26469,#26470,#26471,#26472,#26473,#26474,#26475,#26476,#26477,#26478,
#26479,#26480,#26481,#26482,#26483,#26484,#26485,#26486,#26487,#26488,#26489,
#26490,#26491,#26492,#26493,#26494,#26495,#26496,#26497,#26498,#26499,#26500,
#26501,#26502,#26503,#26504,#26505,#26506,#26507,#26508,#26509,#26510,#26511,
#26512,#26513,#26514,#26515,#26516,#26517,#26518,#26519,#26520,#26521,#26522,
#26523,#26524,#26525,#26526,#26527,#26528,#26529,#26530,#26531,#26532),
 .UNSPECIFIED.,.F.,.F.,(4,3,3,3,3,3,3,3,3,3,3,3,3,3,3,3,3,3,3,3,3,3,3,4),
(1.5707963267949,1.64187501429396,1.71337342981397,1.78582694190369,1.85890794724632,
1.93301112893457,1.97800984258952,2.050296938779,2.12677843749157,2.20103698011112,
2.27862995687019,2.35622293362926,2.43057368240902,2.50653634354047,2.5802247480321,
2.65321980989075,2.72512224828034,2.73442432693481,2.8075010075973,2.87952975922036,
2.93197093834763,3.00457650346015,3.07649190730919,3.14159265358979),
 .UNSPECIFIED.);
#1803=B_SPLINE_CURVE_WITH_KNOTS('',3,(#26607,#26608,#26609,#26610,#26611,
#26612,#26613,#26614,#26615,#26616,#26617,#26618,#26619,#26620,#26621,#26622,
#26623,#26624,#26625,#26626,#26627,#26628,#26629,#26630,#26631,#26632,#26633,
#26634,#26635,#26636,#26637,#26638,#26639,#26640,#26641,#26642,#26643,#26644,
#26645,#26646,#26647,#26648,#26649,#26650,#26651,#26652,#26653,#26654,#26655,
#26656,#26657,#26658,#26659,#26660,#26661,#26662,#26663,#26664,#26665,#26666,
#26667,#26668,#26669,#26670,#26671,#26672,#26673,#26674,#26675,#26676),
 .UNSPECIFIED.,.F.,.F.,(4,3,3,3,3,3,3,3,3,3,3,3,3,3,3,3,3,3,3,3,3,3,3,4),
(1.5707963267949,1.64187501429392,1.7133734298141,1.78582694190386,1.85890794724665,
1.93301112893493,1.97800984258952,2.05029693877883,2.12677843749144,2.20103698011099,
2.27862995687012,2.35622293362926,2.43057368240907,2.50653634354051,2.5802247480322,
2.65321980989064,2.72512224828023,2.73442432693482,2.8075010075969,2.87952975921948,
2.93197093834763,3.00457650346027,3.07649190730933,3.14159265358979),
 .UNSPECIFIED.);
#1804=B_SPLINE_CURVE_WITH_KNOTS('',3,(#26797,#26798,#26799,#26800,#26801,
#26802,#26803,#26804,#26805,#26806,#26807,#26808,#26809,#26810,#26811,#26812,
#26813,#26814,#26815,#26816,#26817,#26818,#26819,#26820,#26821,#26822,#26823,
#26824,#26825,#26826,#26827,#26828,#26829,#26830,#26831,#26832,#26833,#26834,
#26835,#26836,#26837,#26838,#26839,#26840,#26841,#26842,#26843,#26844,#26845,
#26846,#26847,#26848,#26849,#26850,#26851,#26852,#26853,#26854,#26855,#26856,
#26857,#26858,#26859,#26860,#26861,#26862,#26863,#26864,#26865,#26866),
 .UNSPECIFIED.,.F.,.F.,(4,3,3,3,3,3,3,3,3,3,3,3,3,3,3,3,3,3,3,3,3,3,3,4),
(1.5707963267949,1.6418750142939,1.71337342981391,1.78582694190352,1.85890794724598,
1.93301112893406,1.97800984258953,2.05029693877889,2.12677843749147,2.20103698011073,
2.27862995686996,2.3562229336292,2.43057368240849,2.50653634354004,2.58022474803132,
2.65321980988968,2.72512224827939,2.73442432693471,2.80750100759801,2.87952975922287,
2.93197093834755,3.00457650346109,3.07649190731183,3.14159265358979),
 .UNSPECIFIED.);
#1805=B_SPLINE_CURVE_WITH_KNOTS('',3,(#26903,#26904,#26905,#26906,#26907,
#26908,#26909,#26910,#26911,#26912,#26913,#26914,#26915,#26916,#26917,#26918,
#26919,#26920,#26921,#26922,#26923,#26924,#26925,#26926,#26927,#26928,#26929,
#26930,#26931,#26932,#26933,#26934,#26935,#26936,#26937,#26938,#26939,#26940,
#26941,#26942,#26943,#26944,#26945,#26946,#26947,#26948,#26949,#26950,#26951,
#26952,#26953,#26954,#26955,#26956,#26957,#26958,#26959,#26960,#26961,#26962,
#26963,#26964,#26965,#26966,#26967,#26968,#26969,#26970,#26971,#26972),
 .UNSPECIFIED.,.F.,.F.,(4,3,3,3,3,3,3,3,3,3,3,3,3,3,3,3,3,3,3,3,3,3,3,4),
(1.5707963267949,1.64187501429531,1.71337342981643,1.78582694190706,1.85890794725031,
1.9330111289389,1.97800984258968,2.05029693877943,2.12677843749192,2.2010369801112,
2.27862995687028,2.35622293362937,2.4305736824087,2.50653634354023,2.5802247480316,
2.65321980989009,2.72512224827981,2.73442432693483,2.80750100759733,2.87952975922097,
2.93197093834762,3.00457650346007,3.0764919073093,3.14159265358979),
 .UNSPECIFIED.);
#1827=LINE('',#9088,#2145);
#1828=LINE('',#9138,#2146);
#1829=LINE('',#9179,#2147);
#1830=LINE('',#9257,#2148);
#1831=LINE('',#9333,#2149);
#1832=LINE('',#9411,#2150);
#1833=LINE('',#9487,#2151);
#1834=LINE('',#9563,#2152);
#1835=LINE('',#9639,#2153);
#1836=LINE('',#9717,#2154);
#1837=LINE('',#9793,#2155);
#1838=LINE('',#9871,#2156);
#1839=LINE('',#9947,#2157);
#1840=LINE('',#10023,#2158);
#1841=LINE('',#10099,#2159);
#1842=LINE('',#10177,#2160);
#1843=LINE('',#10253,#2161);
#1844=LINE('',#10331,#2162);
#1845=LINE('',#10407,#2163);
#1846=LINE('',#10483,#2164);
#1847=LINE('',#10559,#2165);
#1848=LINE('',#10637,#2166);
#1849=LINE('',#10713,#2167);
#1850=LINE('',#10777,#2168);
#1851=LINE('',#10836,#2169);
#1852=LINE('',#10839,#2170);
#1853=LINE('',#10841,#2171);
#1854=LINE('',#10847,#2172);
#1855=LINE('',#10850,#2173);
#1856=LINE('',#10912,#2174);
#1857=LINE('',#10914,#2175);
#1858=LINE('',#10917,#2176);
#1859=LINE('',#11393,#2177);
#1860=LINE('',#11399,#2178);
#1861=LINE('',#11405,#2179);
#1862=LINE('',#11408,#2180);
#1863=LINE('',#11410,#2181);
#1864=LINE('',#11413,#2182);
#1865=LINE('',#11416,#2183);
#1866=LINE('',#11418,#2184);
#1867=LINE('',#11421,#2185);
#1868=LINE('',#11423,#2186);
#1869=LINE('',#11425,#2187);
#1870=LINE('',#11443,#2188);
#1871=LINE('',#11445,#2189);
#1872=LINE('',#11447,#2190);
#1873=LINE('',#11457,#2191);
#1874=LINE('',#11459,#2192);
#1875=LINE('',#11461,#2193);
#1876=LINE('',#11471,#2194);
#1877=LINE('',#11473,#2195);
#1878=LINE('',#11475,#2196);
#1879=LINE('',#11485,#2197);
#1880=LINE('',#11487,#2198);
#1881=LINE('',#11489,#2199);
#1882=LINE('',#11499,#2200);
#1883=LINE('',#11501,#2201);
#1884=LINE('',#11503,#2202);
#1885=LINE('',#11513,#2203);
#1886=LINE('',#11515,#2204);
#1887=LINE('',#11517,#2205);
#1888=LINE('',#11609,#2206);
#1889=LINE('',#11611,#2207);
#1890=LINE('',#11613,#2208);
#1891=LINE('',#11617,#2209);
#1892=LINE('',#11618,#2210);
#1893=LINE('',#11622,#2211);
#1894=LINE('',#11624,#2212);
#1895=LINE('',#11626,#2213);
#1896=LINE('',#11628,#2214);
#1897=LINE('',#11630,#2215);
#1898=LINE('',#11635,#2216);
#1899=LINE('',#11637,#2217);
#1900=LINE('',#11640,#2218);
#1901=LINE('',#11644,#2219);
#1902=LINE('',#11650,#2220);
#1903=LINE('',#11651,#2221);
#1904=LINE('',#11652,#2222);
#1905=LINE('',#11656,#2223);
#1906=LINE('',#11661,#2224);
#1907=LINE('',#11663,#2225);
#1908=LINE('',#11664,#2226);
#1909=LINE('',#11669,#2227);
#1910=LINE('',#11673,#2228);
#1911=LINE('',#11677,#2229);
#1912=LINE('',#11682,#2230);
#1913=LINE('',#11684,#2231);
#1914=LINE('',#11686,#2232);
#1915=LINE('',#11690,#2233);
#1916=LINE('',#11691,#2234);
#1917=LINE('',#11695,#2235);
#1918=LINE('',#11697,#2236);
#1919=LINE('',#11700,#2237);
#1920=LINE('',#11704,#2238);
#1921=LINE('',#11708,#2239);
#1922=LINE('',#11709,#2240);
#1923=LINE('',#11713,#2241);
#1924=LINE('',#11717,#2242);
#1925=LINE('',#11718,#2243);
#1926=LINE('',#11723,#2244);
#1927=LINE('',#11726,#2245);
#1928=LINE('',#11728,#2246);
#1929=LINE('',#11733,#2247);
#1930=LINE('',#11734,#2248);
#1931=LINE('',#11736,#2249);
#1932=LINE('',#11740,#2250);
#1933=LINE('',#11742,#2251);
#1934=LINE('',#11745,#2252);
#1935=LINE('',#11749,#2253);
#1936=LINE('',#11750,#2254);
#1937=LINE('',#11751,#2255);
#1938=LINE('',#11755,#2256);
#1939=LINE('',#11759,#2257);
#1940=LINE('',#11760,#2258);
#1941=LINE('',#11764,#2259);
#1942=LINE('',#11768,#2260);
#1943=LINE('',#11769,#2261);
#1944=LINE('',#11777,#2262);
#1945=LINE('',#11781,#2263);
#1946=LINE('',#11785,#2264);
#1947=LINE('',#11790,#2265);
#1948=LINE('',#11792,#2266);
#1949=LINE('',#11794,#2267);
#1950=LINE('',#11796,#2268);
#1951=LINE('',#11798,#2269);
#1952=LINE('',#25553,#2270);
#1953=LINE('',#25557,#2271);
#1954=LINE('',#25561,#2272);
#1955=LINE('',#25565,#2273);
#1956=LINE('',#25569,#2274);
#1957=LINE('',#25573,#2275);
#2145=VECTOR('',#7191,8.326);
#2146=VECTOR('',#7194,8.326);
#2147=VECTOR('',#7199,8.326);
#2148=VECTOR('',#7202,8.326);
#2149=VECTOR('',#7205,8.326);
#2150=VECTOR('',#7208,8.326);
#2151=VECTOR('',#7211,8.326);
#2152=VECTOR('',#7214,8.326);
#2153=VECTOR('',#7217,8.326);
#2154=VECTOR('',#7220,8.326);
#2155=VECTOR('',#7223,8.326);
#2156=VECTOR('',#7226,8.326);
#2157=VECTOR('',#7229,8.326);
#2158=VECTOR('',#7232,8.326);
#2159=VECTOR('',#7235,8.326);
#2160=VECTOR('',#7238,8.326);
#2161=VECTOR('',#7241,8.326);
#2162=VECTOR('',#7244,8.326);
#2163=VECTOR('',#7247,8.326);
#2164=VECTOR('',#7250,8.326);
#2165=VECTOR('',#7253,8.326);
#2166=VECTOR('',#7256,8.326);
#2167=VECTOR('',#7259,8.326);
#2168=VECTOR('',#7296,1000.);
#2169=VECTOR('',#7299,1000.);
#2170=VECTOR('',#7302,1000.);
#2171=VECTOR('',#7305,1000.);
#2172=VECTOR('',#7310,1000.);
#2173=VECTOR('',#7313,1000.);
#2174=VECTOR('',#7318,1000.);
#2175=VECTOR('',#7321,1000.);
#2176=VECTOR('',#7324,8.326);
#2177=VECTOR('',#7353,3.2);
#2178=VECTOR('',#7360,3.2);
#2179=VECTOR('',#7367,3.2);
#2180=VECTOR('',#7372,19.05);
#2181=VECTOR('',#7373,1000.);
#2182=VECTOR('',#7376,19.05);
#2183=VECTOR('',#7379,1000.);
#2184=VECTOR('',#7380,1000.);
#2185=VECTOR('',#7383,1000.);
#2186=VECTOR('',#7384,1000.);
#2187=VECTOR('',#7385,1000.);
#2188=VECTOR('',#7404,1000.);
#2189=VECTOR('',#7405,1000.);
#2190=VECTOR('',#7406,1000.);
#2191=VECTOR('',#7409,1000.);
#2192=VECTOR('',#7410,1000.);
#2193=VECTOR('',#7411,1000.);
#2194=VECTOR('',#7414,1000.);
#2195=VECTOR('',#7415,1000.);
#2196=VECTOR('',#7416,1000.);
#2197=VECTOR('',#7419,1000.);
#2198=VECTOR('',#7420,1000.);
#2199=VECTOR('',#7421,1000.);
#2200=VECTOR('',#7424,1000.);
#2201=VECTOR('',#7425,1000.);
#2202=VECTOR('',#7426,1000.);
#2203=VECTOR('',#7429,1000.);
#2204=VECTOR('',#7430,1000.);
#2205=VECTOR('',#7431,1000.);
#2206=VECTOR('',#7440,1000.);
#2207=VECTOR('',#7441,1000.);
#2208=VECTOR('',#7442,1000.);
#2209=VECTOR('',#7445,1000.);
#2210=VECTOR('',#7446,1000.);
#2211=VECTOR('',#7449,1000.);
#2212=VECTOR('',#7450,1000.);
#2213=VECTOR('',#7451,1000.);
#2214=VECTOR('',#7452,1000.);
#2215=VECTOR('',#7453,1000.);
#2216=VECTOR('',#7458,1000.);
#2217=VECTOR('',#7459,1000.);
#2218=VECTOR('',#7462,1000.);
#2219=VECTOR('',#7465,1000.);
#2220=VECTOR('',#7472,1000.);
#2221=VECTOR('',#7473,1000.);
#2222=VECTOR('',#7474,1000.);
#2223=VECTOR('',#7477,1000.);
#2224=VECTOR('',#7484,1000.);
#2225=VECTOR('',#7485,1000.);
#2226=VECTOR('',#7486,1000.);
#2227=VECTOR('',#7491,1000.);
#2228=VECTOR('',#7494,1000.);
#2229=VECTOR('',#7497,1000.);
#2230=VECTOR('',#7502,1000.);
#2231=VECTOR('',#7503,1000.);
#2232=VECTOR('',#7504,1000.);
#2233=VECTOR('',#7507,1000.);
#2234=VECTOR('',#7508,1000.);
#2235=VECTOR('',#7511,1000.);
#2236=VECTOR('',#7512,1000.);
#2237=VECTOR('',#7515,1000.);
#2238=VECTOR('',#7520,1000.);
#2239=VECTOR('',#7525,1000.);
#2240=VECTOR('',#7526,1000.);
#2241=VECTOR('',#7531,1000.);
#2242=VECTOR('',#7536,1000.);
#2243=VECTOR('',#7537,1000.);
#2244=VECTOR('',#7542,1000.);
#2245=VECTOR('',#7545,1000.);
#2246=VECTOR('',#7546,1000.);
#2247=VECTOR('',#7551,1000.);
#2248=VECTOR('',#7552,1000.);
#2249=VECTOR('',#7553,1000.);
#2250=VECTOR('',#7558,1000.);
#2251=VECTOR('',#7559,1000.);
#2252=VECTOR('',#7562,1000.);
#2253=VECTOR('',#7565,1000.);
#2254=VECTOR('',#7566,1000.);
#2255=VECTOR('',#7567,1000.);
#2256=VECTOR('',#7572,1000.);
#2257=VECTOR('',#7577,1000.);
#2258=VECTOR('',#7578,1000.);
#2259=VECTOR('',#7583,1000.);
#2260=VECTOR('',#7588,1000.);
#2261=VECTOR('',#7589,1000.);
#2262=VECTOR('',#7596,1000.);
#2263=VECTOR('',#7599,1000.);
#2264=VECTOR('',#7602,1000.);
#2265=VECTOR('',#7607,1000.);
#2266=VECTOR('',#7608,1000.);
#2267=VECTOR('',#7609,1000.);
#2268=VECTOR('',#7610,1000.);
#2269=VECTOR('',#7611,1000.);
#2270=VECTOR('',#7648,1000.);
#2271=VECTOR('',#7651,1000.);
#2272=VECTOR('',#7654,1000.);
#2273=VECTOR('',#7657,1000.);
#2274=VECTOR('',#7660,1000.);
#2275=VECTOR('',#7663,1000.);
#2463=VERTEX_POINT('',#9086);
#2464=VERTEX_POINT('',#9087);
#2465=VERTEX_POINT('',#9089);
#2466=VERTEX_POINT('',#9126);
#2467=VERTEX_POINT('',#9128);
#2468=VERTEX_POINT('',#9137);
#2469=VERTEX_POINT('',#9177);
#2470=VERTEX_POINT('',#9178);
#2471=VERTEX_POINT('',#9255);
#2472=VERTEX_POINT('',#9256);
#2473=VERTEX_POINT('',#9331);
#2474=VERTEX_POINT('',#9332);
#2475=VERTEX_POINT('',#9409);
#2476=VERTEX_POINT('',#9410);
#2477=VERTEX_POINT('',#9485);
#2478=VERTEX_POINT('',#9486);
#2479=VERTEX_POINT('',#9561);
#2480=VERTEX_POINT('',#9562);
#2481=VERTEX_POINT('',#9637);
#2482=VERTEX_POINT('',#9638);
#2483=VERTEX_POINT('',#9715);
#2484=VERTEX_POINT('',#9716);
#2485=VERTEX_POINT('',#9791);
#2486=VERTEX_POINT('',#9792);
#2487=VERTEX_POINT('',#9869);
#2488=VERTEX_POINT('',#9870);
#2489=VERTEX_POINT('',#9945);
#2490=VERTEX_POINT('',#9946);
#2491=VERTEX_POINT('',#10021);
#2492=VERTEX_POINT('',#10022);
#2493=VERTEX_POINT('',#10097);
#2494=VERTEX_POINT('',#10098);
#2495=VERTEX_POINT('',#10175);
#2496=VERTEX_POINT('',#10176);
#2497=VERTEX_POINT('',#10251);
#2498=VERTEX_POINT('',#10252);
#2499=VERTEX_POINT('',#10329);
#2500=VERTEX_POINT('',#10330);
#2501=VERTEX_POINT('',#10405);
#2502=VERTEX_POINT('',#10406);
#2503=VERTEX_POINT('',#10481);
#2504=VERTEX_POINT('',#10482);
#2505=VERTEX_POINT('',#10557);
#2506=VERTEX_POINT('',#10558);
#2507=VERTEX_POINT('',#10635);
#2508=VERTEX_POINT('',#10636);
#2509=VERTEX_POINT('',#10711);
#2510=VERTEX_POINT('',#10712);
#2511=VERTEX_POINT('',#10714);
#2512=VERTEX_POINT('',#10727);
#2513=VERTEX_POINT('',#10748);
#2514=VERTEX_POINT('',#10749);
#2515=VERTEX_POINT('',#10752);
#2516=VERTEX_POINT('',#10756);
#2517=VERTEX_POINT('',#10758);
#2518=VERTEX_POINT('',#10760);
#2519=VERTEX_POINT('',#10764);
#2520=VERTEX_POINT('',#10765);
#2521=VERTEX_POINT('',#10767);
#2522=VERTEX_POINT('',#10769);
#2523=VERTEX_POINT('',#10773);
#2524=VERTEX_POINT('',#10774);
#2525=VERTEX_POINT('',#10776);
#2526=VERTEX_POINT('',#10778);
#2527=VERTEX_POINT('',#10780);
#2528=VERTEX_POINT('',#10838);
#2529=VERTEX_POINT('',#10843);
#2530=VERTEX_POINT('',#10844);
#2531=VERTEX_POINT('',#10846);
#2532=VERTEX_POINT('',#10848);
#2533=VERTEX_POINT('',#10852);
#2534=VERTEX_POINT('',#10853);
#2535=VERTEX_POINT('',#10909);
#2536=VERTEX_POINT('',#10911);
#2537=VERTEX_POINT('',#10916);
#2538=VERTEX_POINT('',#10920);
#2539=VERTEX_POINT('',#10921);
#2540=VERTEX_POINT('',#10968);
#2541=VERTEX_POINT('',#11021);
#2542=VERTEX_POINT('',#11023);
#2543=VERTEX_POINT('',#11115);
#2544=VERTEX_POINT('',#11123);
#2545=VERTEX_POINT('',#11133);
#2546=VERTEX_POINT('',#11134);
#2547=VERTEX_POINT('',#11136);
#2548=VERTEX_POINT('',#11177);
#2549=VERTEX_POINT('',#11179);
#2550=VERTEX_POINT('',#11225);
#2551=VERTEX_POINT('',#11226);
#2552=VERTEX_POINT('',#11228);
#2553=VERTEX_POINT('',#11269);
#2554=VERTEX_POINT('',#11390);
#2555=VERTEX_POINT('',#11392);
#2556=VERTEX_POINT('',#11396);
#2557=VERTEX_POINT('',#11398);
#2558=VERTEX_POINT('',#11402);
#2559=VERTEX_POINT('',#11404);
#2560=VERTEX_POINT('',#11409);
#2561=VERTEX_POINT('',#11411);
#2562=VERTEX_POINT('',#11414);
#2563=VERTEX_POINT('',#11417);
#2564=VERTEX_POINT('',#11419);
#2565=VERTEX_POINT('',#11422);
#2566=VERTEX_POINT('',#11424);
#2567=VERTEX_POINT('',#11428);
#2568=VERTEX_POINT('',#11429);
#2569=VERTEX_POINT('',#11431);
#2570=VERTEX_POINT('',#11433);
#2571=VERTEX_POINT('',#11435);
#2572=VERTEX_POINT('',#11437);
#2573=VERTEX_POINT('',#11441);
#2574=VERTEX_POINT('',#11442);
#2575=VERTEX_POINT('',#11444);
#2576=VERTEX_POINT('',#11446);
#2577=VERTEX_POINT('',#11455);
#2578=VERTEX_POINT('',#11456);
#2579=VERTEX_POINT('',#11458);
#2580=VERTEX_POINT('',#11460);
#2581=VERTEX_POINT('',#11469);
#2582=VERTEX_POINT('',#11470);
#2583=VERTEX_POINT('',#11472);
#2584=VERTEX_POINT('',#11474);
#2585=VERTEX_POINT('',#11483);
#2586=VERTEX_POINT('',#11484);
#2587=VERTEX_POINT('',#11486);
#2588=VERTEX_POINT('',#11488);
#2589=VERTEX_POINT('',#11497);
#2590=VERTEX_POINT('',#11498);
#2591=VERTEX_POINT('',#11500);
#2592=VERTEX_POINT('',#11502);
#2593=VERTEX_POINT('',#11511);
#2594=VERTEX_POINT('',#11512);
#2595=VERTEX_POINT('',#11514);
#2596=VERTEX_POINT('',#11516);
#2597=VERTEX_POINT('',#11525);
#2598=VERTEX_POINT('',#11526);
#2599=VERTEX_POINT('',#11541);
#2600=VERTEX_POINT('',#11558);
#2601=VERTEX_POINT('',#11583);
#2602=VERTEX_POINT('',#11607);
#2603=VERTEX_POINT('',#11608);
#2604=VERTEX_POINT('',#11610);
#2605=VERTEX_POINT('',#11612);
#2606=VERTEX_POINT('',#11614);
#2607=VERTEX_POINT('',#11616);
#2608=VERTEX_POINT('',#11620);
#2609=VERTEX_POINT('',#11621);
#2610=VERTEX_POINT('',#11623);
#2611=VERTEX_POINT('',#11625);
#2612=VERTEX_POINT('',#11627);
#2613=VERTEX_POINT('',#11629);
#2614=VERTEX_POINT('',#11633);
#2615=VERTEX_POINT('',#11634);
#2616=VERTEX_POINT('',#11636);
#2617=VERTEX_POINT('',#11638);
#2618=VERTEX_POINT('',#11642);
#2619=VERTEX_POINT('',#11643);
#2620=VERTEX_POINT('',#11648);
#2621=VERTEX_POINT('',#11649);
#2622=VERTEX_POINT('',#11654);
#2623=VERTEX_POINT('',#11655);
#2624=VERTEX_POINT('',#11660);
#2625=VERTEX_POINT('',#11662);
#2626=VERTEX_POINT('',#11666);
#2627=VERTEX_POINT('',#11668);
#2628=VERTEX_POINT('',#11670);
#2629=VERTEX_POINT('',#11672);
#2630=VERTEX_POINT('',#11674);
#2631=VERTEX_POINT('',#11676);
#2632=VERTEX_POINT('',#11680);
#2633=VERTEX_POINT('',#11681);
#2634=VERTEX_POINT('',#11683);
#2635=VERTEX_POINT('',#11685);
#2636=VERTEX_POINT('',#11687);
#2637=VERTEX_POINT('',#11689);
#2638=VERTEX_POINT('',#11693);
#2639=VERTEX_POINT('',#11694);
#2640=VERTEX_POINT('',#11696);
#2641=VERTEX_POINT('',#11698);
#2642=VERTEX_POINT('',#11703);
#2643=VERTEX_POINT('',#11707);
#2644=VERTEX_POINT('',#11712);
#2645=VERTEX_POINT('',#11716);
#2646=VERTEX_POINT('',#11720);
#2647=VERTEX_POINT('',#11722);
#2648=VERTEX_POINT('',#11724);
#2649=VERTEX_POINT('',#11727);
#2650=VERTEX_POINT('',#11731);
#2651=VERTEX_POINT('',#11732);
#2652=VERTEX_POINT('',#11735);
#2653=VERTEX_POINT('',#11739);
#2654=VERTEX_POINT('',#11741);
#2655=VERTEX_POINT('',#11743);
#2656=VERTEX_POINT('',#11747);
#2657=VERTEX_POINT('',#11748);
#2658=VERTEX_POINT('',#11753);
#2659=VERTEX_POINT('',#11758);
#2660=VERTEX_POINT('',#11762);
#2661=VERTEX_POINT('',#11767);
#2662=VERTEX_POINT('',#11771);
#2663=VERTEX_POINT('',#11772);
#2664=VERTEX_POINT('',#11774);
#2665=VERTEX_POINT('',#11776);
#2666=VERTEX_POINT('',#11778);
#2667=VERTEX_POINT('',#11780);
#2668=VERTEX_POINT('',#11782);
#2669=VERTEX_POINT('',#11784);
#2670=VERTEX_POINT('',#11788);
#2671=VERTEX_POINT('',#11789);
#2672=VERTEX_POINT('',#11791);
#2673=VERTEX_POINT('',#11793);
#2674=VERTEX_POINT('',#11795);
#2675=VERTEX_POINT('',#11797);
#2676=VERTEX_POINT('',#11801);
#2677=VERTEX_POINT('',#11923);
#2678=VERTEX_POINT('',#12042);
#2679=VERTEX_POINT('',#12164);
#2680=VERTEX_POINT('',#12283);
#2681=VERTEX_POINT('',#12405);
#2682=VERTEX_POINT('',#12608);
#2683=VERTEX_POINT('',#12707);
#2684=VERTEX_POINT('',#12807);
#2685=VERTEX_POINT('',#12906);
#2686=VERTEX_POINT('',#13006);
#2687=VERTEX_POINT('',#13013);
#2688=VERTEX_POINT('',#13030);
#2689=VERTEX_POINT('',#25551);
#2690=VERTEX_POINT('',#25552);
#2691=VERTEX_POINT('',#25554);
#2692=VERTEX_POINT('',#25556);
#2693=VERTEX_POINT('',#25558);
#2694=VERTEX_POINT('',#25560);
#2695=VERTEX_POINT('',#25562);
#2696=VERTEX_POINT('',#25564);
#2697=VERTEX_POINT('',#25566);
#2698=VERTEX_POINT('',#25568);
#2699=VERTEX_POINT('',#25570);
#2700=VERTEX_POINT('',#25572);
#3024=EDGE_CURVE('',#2463,#2464,#1827,.T.);
#3025=EDGE_CURVE('',#2464,#2465,#1700,.T.);
#3026=EDGE_CURVE('',#2466,#2465,#1300,.T.);
#3027=EDGE_CURVE('',#2466,#2467,#1701,.T.);
#3028=EDGE_CURVE('',#2467,#2468,#1828,.T.);
#3029=EDGE_CURVE('',#2468,#2468,#1301,.T.);
#3030=EDGE_CURVE('',#2467,#2463,#1702,.T.);
#3031=EDGE_CURVE('',#2469,#2470,#1829,.T.);
#3032=EDGE_CURVE('',#2470,#2464,#1703,.T.);
#3033=EDGE_CURVE('',#2463,#2469,#1704,.T.);
#3034=EDGE_CURVE('',#2471,#2472,#1830,.T.);
#3035=EDGE_CURVE('',#2472,#2470,#1705,.T.);
#3036=EDGE_CURVE('',#2469,#2471,#1706,.T.);
#3037=EDGE_CURVE('',#2473,#2474,#1831,.T.);
#3038=EDGE_CURVE('',#2474,#2472,#1707,.T.);
#3039=EDGE_CURVE('',#2471,#2473,#1708,.T.);
#3040=EDGE_CURVE('',#2475,#2476,#1832,.T.);
#3041=EDGE_CURVE('',#2476,#2474,#1709,.T.);
#3042=EDGE_CURVE('',#2473,#2475,#1710,.T.);
#3043=EDGE_CURVE('',#2477,#2478,#1833,.T.);
#3044=EDGE_CURVE('',#2478,#2476,#1711,.T.);
#3045=EDGE_CURVE('',#2475,#2477,#1712,.T.);
#3046=EDGE_CURVE('',#2479,#2480,#1834,.T.);
#3047=EDGE_CURVE('',#2480,#2478,#1713,.T.);
#3048=EDGE_CURVE('',#2477,#2479,#1714,.T.);
#3049=EDGE_CURVE('',#2481,#2482,#1835,.T.);
#3050=EDGE_CURVE('',#2482,#2480,#1715,.T.);
#3051=EDGE_CURVE('',#2479,#2481,#1716,.T.);
#3052=EDGE_CURVE('',#2483,#2484,#1836,.T.);
#3053=EDGE_CURVE('',#2484,#2482,#1717,.T.);
#3054=EDGE_CURVE('',#2481,#2483,#1718,.T.);
#3055=EDGE_CURVE('',#2485,#2486,#1837,.T.);
#3056=EDGE_CURVE('',#2486,#2484,#1719,.T.);
#3057=EDGE_CURVE('',#2483,#2485,#1720,.T.);
#3058=EDGE_CURVE('',#2487,#2488,#1838,.T.);
#3059=EDGE_CURVE('',#2488,#2486,#1721,.T.);
#3060=EDGE_CURVE('',#2485,#2487,#1722,.T.);
#3061=EDGE_CURVE('',#2489,#2490,#1839,.T.);
#3062=EDGE_CURVE('',#2490,#2488,#1723,.T.);
#3063=EDGE_CURVE('',#2487,#2489,#1724,.T.);
#3064=EDGE_CURVE('',#2491,#2492,#1840,.T.);
#3065=EDGE_CURVE('',#2492,#2490,#1725,.T.);
#3066=EDGE_CURVE('',#2489,#2491,#1726,.T.);
#3067=EDGE_CURVE('',#2493,#2494,#1841,.T.);
#3068=EDGE_CURVE('',#2494,#2492,#1727,.T.);
#3069=EDGE_CURVE('',#2491,#2493,#1728,.T.);
#3070=EDGE_CURVE('',#2495,#2496,#1842,.T.);
#3071=EDGE_CURVE('',#2496,#2494,#1729,.T.);
#3072=EDGE_CURVE('',#2493,#2495,#1730,.T.);
#3073=EDGE_CURVE('',#2497,#2498,#1843,.T.);
#3074=EDGE_CURVE('',#2498,#2496,#1731,.T.);
#3075=EDGE_CURVE('',#2495,#2497,#1732,.T.);
#3076=EDGE_CURVE('',#2499,#2500,#1844,.T.);
#3077=EDGE_CURVE('',#2500,#2498,#1733,.T.);
#3078=EDGE_CURVE('',#2497,#2499,#1734,.T.);
#3079=EDGE_CURVE('',#2501,#2502,#1845,.T.);
#3080=EDGE_CURVE('',#2502,#2500,#1735,.T.);
#3081=EDGE_CURVE('',#2499,#2501,#1736,.T.);
#3082=EDGE_CURVE('',#2503,#2504,#1846,.T.);
#3083=EDGE_CURVE('',#2504,#2502,#1737,.T.);
#3084=EDGE_CURVE('',#2501,#2503,#1738,.T.);
#3085=EDGE_CURVE('',#2505,#2506,#1847,.T.);
#3086=EDGE_CURVE('',#2506,#2504,#1739,.T.);
#3087=EDGE_CURVE('',#2503,#2505,#1740,.T.);
#3088=EDGE_CURVE('',#2507,#2508,#1848,.T.);
#3089=EDGE_CURVE('',#2508,#2506,#1741,.T.);
#3090=EDGE_CURVE('',#2505,#2507,#1742,.T.);
#3091=EDGE_CURVE('',#2509,#2510,#1849,.T.);
#3092=EDGE_CURVE('',#2509,#2511,#1743,.T.);
#3093=EDGE_CURVE('',#2511,#2512,#1302,.T.);
#3094=EDGE_CURVE('',#2512,#2510,#1744,.T.);
#3095=EDGE_CURVE('',#2513,#2514,#1303,.T.);
#3096=EDGE_CURVE('',#2514,#2513,#1304,.T.);
#3097=EDGE_CURVE('',#2514,#2515,#1305,.T.);
#3098=EDGE_CURVE('',#2515,#2515,#1306,.T.);
#3099=EDGE_CURVE('',#2516,#2516,#1307,.T.);
#3100=EDGE_CURVE('',#2516,#2517,#1308,.T.);
#3101=EDGE_CURVE('',#2518,#2517,#1309,.T.);
#3102=EDGE_CURVE('',#2517,#2518,#1310,.T.);
#3103=EDGE_CURVE('',#2519,#2520,#1311,.T.);
#3104=EDGE_CURVE('',#2521,#2519,#1312,.T.);
#3105=EDGE_CURVE('',#2522,#2521,#1313,.T.);
#3106=EDGE_CURVE('',#2522,#2520,#1314,.T.);
#3107=EDGE_CURVE('',#2523,#2524,#1315,.T.);
#3108=EDGE_CURVE('',#2525,#2524,#1850,.T.);
#3109=EDGE_CURVE('',#2526,#2525,#454,.T.);
#3110=EDGE_CURVE('',#2527,#2526,#1745,.T.);
#3111=EDGE_CURVE('',#2523,#2527,#1851,.T.);
#3112=EDGE_CURVE('',#2528,#2521,#1852,.T.);
#3113=EDGE_CURVE('',#2523,#2528,#1316,.T.);
#3114=EDGE_CURVE('',#2522,#2523,#1853,.T.);
#3115=EDGE_CURVE('',#2529,#2530,#1317,.T.);
#3116=EDGE_CURVE('',#2531,#2530,#1854,.T.);
#3117=EDGE_CURVE('',#2531,#2532,#1318,.T.);
#3118=EDGE_CURVE('',#2529,#2532,#1855,.T.);
#3119=EDGE_CURVE('',#2533,#2534,#1746,.T.);
#3120=EDGE_CURVE('',#2534,#2535,#455,.T.);
#3121=EDGE_CURVE('',#2536,#2535,#1856,.T.);
#3122=EDGE_CURVE('',#2529,#2536,#1319,.T.);
#3123=EDGE_CURVE('',#2533,#2529,#1857,.T.);
#3124=EDGE_CURVE('',#2468,#2537,#1858,.T.);
#3125=EDGE_CURVE('',#2537,#2537,#1320,.T.);
#3126=EDGE_CURVE('',#2538,#2539,#1747,.T.);
#3127=EDGE_CURVE('',#2539,#2540,#1748,.T.);
#3128=EDGE_CURVE('',#2541,#2540,#1321,.T.);
#3129=EDGE_CURVE('',#2541,#2542,#1749,.T.);
#3130=EDGE_CURVE('',#2542,#2543,#1750,.T.);
#3131=EDGE_CURVE('',#2544,#2543,#1322,.T.);
#3132=EDGE_CURVE('',#2544,#2538,#1751,.T.);
#3133=EDGE_CURVE('',#2545,#2546,#1323,.T.);
#3134=EDGE_CURVE('',#2545,#2547,#1752,.T.);
#3135=EDGE_CURVE('',#2548,#2547,#1324,.T.);
#3136=EDGE_CURVE('',#2549,#2548,#1325,.T.);
#3137=EDGE_CURVE('',#2549,#2546,#1753,.T.);
#3138=EDGE_CURVE('',#2550,#2551,#1326,.T.);
#3139=EDGE_CURVE('',#2550,#2552,#1754,.T.);
#3140=EDGE_CURVE('',#2553,#2552,#1327,.T.);
#3141=EDGE_CURVE('',#2553,#2551,#1755,.T.);
#3142=EDGE_CURVE('',#2510,#2508,#1756,.T.);
#3143=EDGE_CURVE('',#2507,#2509,#1757,.T.);
#3144=EDGE_CURVE('',#2554,#2554,#1328,.T.);
#3145=EDGE_CURVE('',#2554,#2555,#1859,.T.);
#3146=EDGE_CURVE('',#2555,#2555,#1329,.T.);
#3147=EDGE_CURVE('',#2556,#2556,#1330,.T.);
#3148=EDGE_CURVE('',#2556,#2557,#1860,.T.);
#3149=EDGE_CURVE('',#2557,#2557,#1331,.T.);
#3150=EDGE_CURVE('',#2558,#2558,#1332,.T.);
#3151=EDGE_CURVE('',#2558,#2559,#1861,.T.);
#3152=EDGE_CURVE('',#2559,#2559,#1333,.T.);
#3153=EDGE_CURVE('',#2513,#2548,#1862,.T.);
#3154=EDGE_CURVE('',#2547,#2560,#1863,.T.);
#3155=EDGE_CURVE('',#2560,#2561,#1334,.T.);
#3156=EDGE_CURVE('',#2561,#2518,#1864,.T.);
#3157=EDGE_CURVE('',#2561,#2562,#1335,.T.);
#3158=EDGE_CURVE('',#2562,#2549,#1865,.T.);
#3159=EDGE_CURVE('',#2540,#2563,#1866,.T.);
#3160=EDGE_CURVE('',#2563,#2564,#1336,.T.);
#3161=EDGE_CURVE('',#2564,#2541,#1867,.T.);
#3162=EDGE_CURVE('',#2565,#2553,#1868,.T.);
#3163=EDGE_CURVE('',#2552,#2566,#1869,.T.);
#3164=EDGE_CURVE('',#2566,#2565,#1337,.T.);
#3165=EDGE_CURVE('',#2567,#2568,#1338,.T.);
#3166=EDGE_CURVE('',#2568,#2569,#1339,.T.);
#3167=EDGE_CURVE('',#2569,#2570,#1340,.T.);
#3168=EDGE_CURVE('',#2570,#2571,#1341,.T.);
#3169=EDGE_CURVE('',#2571,#2572,#1342,.T.);
#3170=EDGE_CURVE('',#2572,#2567,#1343,.T.);
#3171=EDGE_CURVE('',#2573,#2574,#1870,.T.);
#3172=EDGE_CURVE('',#2574,#2575,#1871,.T.);
#3173=EDGE_CURVE('',#2575,#2576,#1872,.T.);
#3174=EDGE_CURVE('',#2576,#2568,#183,.T.);
#3175=EDGE_CURVE('',#2568,#2573,#184,.T.);
#3176=EDGE_CURVE('',#2577,#2578,#1873,.T.);
#3177=EDGE_CURVE('',#2578,#2579,#1874,.T.);
#3178=EDGE_CURVE('',#2579,#2580,#1875,.T.);
#3179=EDGE_CURVE('',#2580,#2567,#185,.T.);
#3180=EDGE_CURVE('',#2567,#2577,#186,.T.);
#3181=EDGE_CURVE('',#2581,#2582,#1876,.T.);
#3182=EDGE_CURVE('',#2582,#2583,#1877,.T.);
#3183=EDGE_CURVE('',#2583,#2584,#1878,.T.);
#3184=EDGE_CURVE('',#2584,#2572,#187,.T.);
#3185=EDGE_CURVE('',#2572,#2581,#188,.T.);
#3186=EDGE_CURVE('',#2585,#2586,#1879,.T.);
#3187=EDGE_CURVE('',#2586,#2587,#1880,.T.);
#3188=EDGE_CURVE('',#2587,#2588,#1881,.T.);
#3189=EDGE_CURVE('',#2588,#2571,#189,.T.);
#3190=EDGE_CURVE('',#2571,#2585,#190,.T.);
#3191=EDGE_CURVE('',#2589,#2590,#1882,.T.);
#3192=EDGE_CURVE('',#2590,#2591,#1883,.T.);
#3193=EDGE_CURVE('',#2591,#2592,#1884,.T.);
#3194=EDGE_CURVE('',#2592,#2570,#191,.T.);
#3195=EDGE_CURVE('',#2570,#2589,#192,.T.);
#3196=EDGE_CURVE('',#2593,#2594,#1885,.T.);
#3197=EDGE_CURVE('',#2594,#2595,#1886,.T.);
#3198=EDGE_CURVE('',#2595,#2596,#1887,.T.);
#3199=EDGE_CURVE('',#2596,#2569,#193,.T.);
#3200=EDGE_CURVE('',#2569,#2593,#194,.T.);
#3201=EDGE_CURVE('',#2597,#2598,#1758,.T.);
#3202=EDGE_CURVE('',#2599,#2597,#1759,.T.);
#3203=EDGE_CURVE('',#2599,#2598,#1344,.T.);
#3204=EDGE_CURVE('',#2511,#2600,#1760,.T.);
#3205=EDGE_CURVE('',#2600,#2598,#1761,.T.);
#3206=EDGE_CURVE('',#2599,#2601,#1762,.T.);
#3207=EDGE_CURVE('',#2601,#2512,#1763,.T.);
#3208=EDGE_CURVE('',#2602,#2603,#1888,.T.);
#3209=EDGE_CURVE('',#2603,#2604,#1889,.T.);
#3210=EDGE_CURVE('',#2604,#2605,#1890,.T.);
#3211=EDGE_CURVE('',#2605,#2606,#456,.T.);
#3212=EDGE_CURVE('',#2606,#2607,#1891,.T.);
#3213=EDGE_CURVE('',#2607,#2602,#1892,.T.);
#3214=EDGE_CURVE('',#2608,#2609,#1893,.T.);
#3215=EDGE_CURVE('',#2609,#2610,#1894,.T.);
#3216=EDGE_CURVE('',#2610,#2611,#1895,.T.);
#3217=EDGE_CURVE('',#2611,#2612,#1896,.T.);
#3218=EDGE_CURVE('',#2612,#2613,#1897,.T.);
#3219=EDGE_CURVE('',#2613,#2608,#457,.T.);
#3220=EDGE_CURVE('',#2614,#2615,#1898,.T.);
#3221=EDGE_CURVE('',#2614,#2616,#1899,.T.);
#3222=EDGE_CURVE('',#2616,#2617,#1345,.T.);
#3223=EDGE_CURVE('',#2617,#2615,#1900,.T.);
#3224=EDGE_CURVE('',#2618,#2619,#1901,.T.);
#3225=EDGE_CURVE('',#2618,#2614,#1346,.T.);
#3226=EDGE_CURVE('',#2615,#2619,#1347,.T.);
#3227=EDGE_CURVE('',#2620,#2621,#1902,.T.);
#3228=EDGE_CURVE('',#2620,#2618,#1903,.T.);
#3229=EDGE_CURVE('',#2619,#2621,#1904,.T.);
#3230=EDGE_CURVE('',#2622,#2623,#1905,.T.);
#3231=EDGE_CURVE('',#2622,#2620,#1348,.T.);
#3232=EDGE_CURVE('',#2621,#2623,#1349,.T.);
#3233=EDGE_CURVE('',#2623,#2624,#1906,.T.);
#3234=EDGE_CURVE('',#2624,#2625,#1907,.T.);
#3235=EDGE_CURVE('',#2625,#2622,#1908,.T.);
#3236=EDGE_CURVE('',#2551,#2626,#1350,.T.);
#3237=EDGE_CURVE('',#2626,#2627,#1909,.T.);
#3238=EDGE_CURVE('',#2627,#2628,#1351,.T.);
#3239=EDGE_CURVE('',#2628,#2629,#1910,.T.);
#3240=EDGE_CURVE('',#2629,#2630,#1352,.T.);
#3241=EDGE_CURVE('',#2630,#2631,#1911,.T.);
#3242=EDGE_CURVE('',#2631,#2550,#1353,.T.);
#3243=EDGE_CURVE('',#2632,#2633,#1912,.T.);
#3244=EDGE_CURVE('',#2633,#2634,#1913,.T.);
#3245=EDGE_CURVE('',#2634,#2635,#1914,.T.);
#3246=EDGE_CURVE('',#2635,#2636,#458,.T.);
#3247=EDGE_CURVE('',#2636,#2637,#1915,.T.);
#3248=EDGE_CURVE('',#2637,#2632,#1916,.T.);
#3249=EDGE_CURVE('',#2638,#2639,#1917,.T.);
#3250=EDGE_CURVE('',#2638,#2640,#1918,.T.);
#3251=EDGE_CURVE('',#2640,#2641,#1354,.T.);
#3252=EDGE_CURVE('',#2641,#2639,#1919,.T.);
#3253=EDGE_CURVE('',#2639,#2525,#1355,.T.);
#3254=EDGE_CURVE('',#2642,#2525,#1920,.T.);
#3255=EDGE_CURVE('',#2642,#2638,#1356,.T.);
#3256=EDGE_CURVE('',#2643,#2524,#1921,.T.);
#3257=EDGE_CURVE('',#2643,#2642,#1922,.T.);
#3258=EDGE_CURVE('',#2524,#2528,#1357,.T.);
#3259=EDGE_CURVE('',#2644,#2528,#1923,.T.);
#3260=EDGE_CURVE('',#2644,#2643,#1358,.T.);
#3261=EDGE_CURVE('',#2521,#2645,#1924,.T.);
#3262=EDGE_CURVE('',#2645,#2644,#1925,.T.);
#3263=EDGE_CURVE('',#2546,#2646,#1359,.T.);
#3264=EDGE_CURVE('',#2646,#2647,#1926,.T.);
#3265=EDGE_CURVE('',#2647,#2648,#1360,.T.);
#3266=EDGE_CURVE('',#2648,#2519,#1927,.T.);
#3267=EDGE_CURVE('',#2520,#2649,#1928,.T.);
#3268=EDGE_CURVE('',#2649,#2545,#1361,.T.);
#3269=EDGE_CURVE('',#2650,#2651,#1929,.T.);
#3270=EDGE_CURVE('',#2651,#2522,#1930,.T.);
#3271=EDGE_CURVE('',#2527,#2652,#1931,.T.);
#3272=EDGE_CURVE('',#2652,#2650,#459,.T.);
#3273=EDGE_CURVE('',#2532,#2653,#1932,.T.);
#3274=EDGE_CURVE('',#2653,#2654,#1933,.T.);
#3275=EDGE_CURVE('',#2654,#2655,#460,.T.);
#3276=EDGE_CURVE('',#2655,#2533,#1934,.T.);
#3277=EDGE_CURVE('',#2656,#2657,#1935,.T.);
#3278=EDGE_CURVE('',#2656,#2544,#1936,.T.);
#3279=EDGE_CURVE('',#2543,#2657,#1937,.T.);
#3280=EDGE_CURVE('',#2657,#2658,#1362,.T.);
#3281=EDGE_CURVE('',#2535,#2658,#1938,.T.);
#3282=EDGE_CURVE('',#2535,#2656,#1363,.T.);
#3283=EDGE_CURVE('',#2658,#2659,#1939,.T.);
#3284=EDGE_CURVE('',#2536,#2659,#1940,.T.);
#3285=EDGE_CURVE('',#2659,#2660,#1364,.T.);
#3286=EDGE_CURVE('',#2530,#2660,#1941,.T.);
#3287=EDGE_CURVE('',#2530,#2536,#1365,.T.);
#3288=EDGE_CURVE('',#2660,#2661,#1942,.T.);
#3289=EDGE_CURVE('',#2661,#2531,#1943,.T.);
#3290=EDGE_CURVE('',#2662,#2663,#1366,.T.);
#3291=EDGE_CURVE('',#2663,#2664,#1367,.T.);
#3292=EDGE_CURVE('',#2664,#2665,#1944,.T.);
#3293=EDGE_CURVE('',#2665,#2666,#1368,.T.);
#3294=EDGE_CURVE('',#2666,#2667,#1945,.T.);
#3295=EDGE_CURVE('',#2667,#2668,#1369,.T.);
#3296=EDGE_CURVE('',#2668,#2669,#1946,.T.);
#3297=EDGE_CURVE('',#2669,#2662,#1370,.T.);
#3298=EDGE_CURVE('',#2670,#2671,#1947,.T.);
#3299=EDGE_CURVE('',#2671,#2672,#1948,.T.);
#3300=EDGE_CURVE('',#2672,#2673,#1949,.T.);
#3301=EDGE_CURVE('',#2673,#2674,#1950,.T.);
#3302=EDGE_CURVE('',#2674,#2675,#1951,.T.);
#3303=EDGE_CURVE('',#2675,#2670,#461,.T.);
#3304=EDGE_CURVE('',#2552,#2676,#1764,.T.);
#3305=EDGE_CURVE('',#2676,#2609,#1371,.T.);
#3306=EDGE_CURVE('',#2608,#2566,#1765,.T.);
#3307=EDGE_CURVE('',#2653,#2677,#1372,.T.);
#3308=EDGE_CURVE('',#2677,#2563,#1766,.T.);
#3309=EDGE_CURVE('',#2540,#2654,#1767,.T.);
#3310=EDGE_CURVE('',#2564,#2678,#1768,.T.);
#3311=EDGE_CURVE('',#2678,#2671,#1373,.T.);
#3312=EDGE_CURVE('',#2670,#2541,#1769,.T.);
#3313=EDGE_CURVE('',#2634,#2679,#1374,.T.);
#3314=EDGE_CURVE('',#2679,#2549,#1770,.T.);
#3315=EDGE_CURVE('',#2562,#2635,#1771,.T.);
#3316=EDGE_CURVE('',#2547,#2680,#1772,.T.);
#3317=EDGE_CURVE('',#2680,#2651,#1375,.T.);
#3318=EDGE_CURVE('',#2650,#2560,#1773,.T.);
#3319=EDGE_CURVE('',#2604,#2681,#1376,.T.);
#3320=EDGE_CURVE('',#2681,#2553,#1774,.T.);
#3321=EDGE_CURVE('',#2565,#2605,#1775,.T.);
#3322=EDGE_CURVE('',#2563,#2663,#1776,.T.);
#3323=EDGE_CURVE('',#2662,#2564,#1777,.T.);
#3324=EDGE_CURVE('',#2560,#2682,#1778,.T.);
#3325=EDGE_CURVE('',#2682,#2641,#1779,.T.);
#3326=EDGE_CURVE('',#2640,#2683,#1780,.T.);
#3327=EDGE_CURVE('',#2683,#2562,#1781,.T.);
#3328=EDGE_CURVE('',#2616,#2684,#1782,.T.);
#3329=EDGE_CURVE('',#2684,#2565,#1783,.T.);
#3330=EDGE_CURVE('',#2566,#2685,#1784,.T.);
#3331=EDGE_CURVE('',#2685,#2617,#1785,.T.);
#3332=EDGE_CURVE('',#2686,#2465,#1786,.T.);
#3333=EDGE_CURVE('',#2687,#2686,#1787,.T.);
#3334=EDGE_CURVE('',#2688,#2687,#1788,.T.);
#3335=EDGE_CURVE('',#2466,#2688,#1789,.T.);
#3336=EDGE_CURVE('',#2600,#2688,#195,.T.);
#3337=EDGE_CURVE('',#2597,#2687,#196,.T.);
#3338=EDGE_CURVE('',#2601,#2686,#197,.T.);
#3339=EDGE_CURVE('',#2689,#2690,#1952,.T.);
#3340=EDGE_CURVE('',#2690,#2691,#1377,.T.);
#3341=EDGE_CURVE('',#2691,#2692,#1953,.T.);
#3342=EDGE_CURVE('',#2692,#2693,#1378,.T.);
#3343=EDGE_CURVE('',#2693,#2694,#1954,.T.);
#3344=EDGE_CURVE('',#2694,#2695,#1379,.T.);
#3345=EDGE_CURVE('',#2695,#2696,#1955,.T.);
#3346=EDGE_CURVE('',#2696,#2697,#1380,.T.);
#3347=EDGE_CURVE('',#2697,#2698,#1956,.T.);
#3348=EDGE_CURVE('',#2698,#2699,#1381,.T.);
#3349=EDGE_CURVE('',#2699,#2700,#1957,.T.);
#3350=EDGE_CURVE('',#2700,#2689,#1382,.T.);
#3351=EDGE_CURVE('',#2576,#2593,#1790,.T.);
#3352=EDGE_CURVE('',#2596,#2589,#1791,.T.);
#3353=EDGE_CURVE('',#2592,#2585,#1792,.T.);
#3354=EDGE_CURVE('',#2588,#2581,#1793,.T.);
#3355=EDGE_CURVE('',#2584,#2577,#1794,.T.);
#3356=EDGE_CURVE('',#2580,#2573,#1795,.T.);
#3357=EDGE_CURVE('',#2583,#2578,#1383,.T.);
#3358=EDGE_CURVE('',#2587,#2582,#1384,.T.);
#3359=EDGE_CURVE('',#2591,#2586,#1385,.T.);
#3360=EDGE_CURVE('',#2595,#2590,#1386,.T.);
#3361=EDGE_CURVE('',#2575,#2594,#1387,.T.);
#3362=EDGE_CURVE('',#2579,#2574,#1388,.T.);
#3363=EDGE_CURVE('',#2594,#2696,#1389,.T.);
#3364=EDGE_CURVE('',#2697,#2575,#1390,.T.);
#3365=EDGE_CURVE('',#2698,#2574,#1391,.T.);
#3366=EDGE_CURVE('',#2595,#2695,#1392,.T.);
#3367=EDGE_CURVE('',#2699,#2579,#1393,.T.);
#3368=EDGE_CURVE('',#2590,#2694,#1394,.T.);
#3369=EDGE_CURVE('',#2700,#2578,#1395,.T.);
#3370=EDGE_CURVE('',#2591,#2693,#1396,.T.);
#3371=EDGE_CURVE('',#2689,#2583,#1397,.T.);
#3372=EDGE_CURVE('',#2586,#2692,#1398,.T.);
#3373=EDGE_CURVE('',#2690,#2582,#1399,.T.);
#3374=EDGE_CURVE('',#2587,#2691,#1400,.T.);
#3375=EDGE_CURVE('',#2625,#2603,#1401,.T.);
#3376=EDGE_CURVE('',#2622,#2602,#1402,.T.);
#3377=EDGE_CURVE('',#2620,#2602,#1403,.T.);
#3378=EDGE_CURVE('',#2618,#2607,#1796,.T.);
#3379=EDGE_CURVE('',#2614,#2607,#1797,.T.);
#3380=EDGE_CURVE('',#2616,#2606,#1404,.T.);
#3381=EDGE_CURVE('',#2684,#2605,#1405,.T.);
#3382=EDGE_CURVE('',#2610,#2624,#1406,.T.);
#3383=EDGE_CURVE('',#2611,#2623,#1407,.T.);
#3384=EDGE_CURVE('',#2611,#2621,#1408,.T.);
#3385=EDGE_CURVE('',#2612,#2619,#1798,.T.);
#3386=EDGE_CURVE('',#2612,#2615,#1799,.T.);
#3387=EDGE_CURVE('',#2613,#2617,#1409,.T.);
#3388=EDGE_CURVE('',#2608,#2685,#1410,.T.);
#3389=EDGE_CURVE('',#2672,#2661,#1411,.T.);
#3390=EDGE_CURVE('',#2673,#2660,#1412,.T.);
#3391=EDGE_CURVE('',#2673,#2659,#1413,.T.);
#3392=EDGE_CURVE('',#2674,#2658,#1800,.T.);
#3393=EDGE_CURVE('',#2674,#2657,#1801,.T.);
#3394=EDGE_CURVE('',#2675,#2543,#1414,.T.);
#3395=EDGE_CURVE('',#2670,#2542,#1415,.T.);
#3396=EDGE_CURVE('',#2654,#2538,#1416,.T.);
#3397=EDGE_CURVE('',#2655,#2544,#1417,.T.);
#3398=EDGE_CURVE('',#2533,#2656,#1802,.T.);
#3399=EDGE_CURVE('',#2527,#2639,#1803,.T.);
#3400=EDGE_CURVE('',#2652,#2641,#1418,.T.);
#3401=EDGE_CURVE('',#2650,#2682,#1419,.T.);
#3402=EDGE_CURVE('',#2635,#2683,#1420,.T.);
#3403=EDGE_CURVE('',#2636,#2640,#1421,.T.);
#3404=EDGE_CURVE('',#2637,#2638,#1804,.T.);
#3405=EDGE_CURVE('',#2637,#2642,#1805,.T.);
#3406=EDGE_CURVE('',#2632,#2643,#1422,.T.);
#3407=EDGE_CURVE('',#2632,#2644,#1423,.T.);
#3408=EDGE_CURVE('',#2645,#2633,#1424,.T.);
#3409=EDGE_CURVE('',#2551,#2681,#1425,.T.);
#3410=EDGE_CURVE('',#2626,#2604,#1426,.T.);
#3411=EDGE_CURVE('',#2627,#2603,#1427,.T.);
#3412=EDGE_CURVE('',#2628,#2625,#1428,.T.);
#3413=EDGE_CURVE('',#2629,#2624,#1429,.T.);
#3414=EDGE_CURVE('',#2630,#2610,#1430,.T.);
#3415=EDGE_CURVE('',#2631,#2609,#1431,.T.);
#3416=EDGE_CURVE('',#2550,#2676,#1432,.T.);
#3417=EDGE_CURVE('',#2678,#2662,#1433,.T.);
#3418=EDGE_CURVE('',#2671,#2669,#1434,.T.);
#3419=EDGE_CURVE('',#2672,#2668,#1435,.T.);
#3420=EDGE_CURVE('',#2661,#2667,#1436,.T.);
#3421=EDGE_CURVE('',#2531,#2666,#1437,.T.);
#3422=EDGE_CURVE('',#2532,#2665,#1438,.T.);
#3423=EDGE_CURVE('',#2653,#2664,#1439,.T.);
#3424=EDGE_CURVE('',#2677,#2663,#1440,.T.);
#3425=EDGE_CURVE('',#2680,#2545,#1441,.T.);
#3426=EDGE_CURVE('',#2651,#2649,#1442,.T.);
#3427=EDGE_CURVE('',#2645,#2648,#1443,.T.);
#3428=EDGE_CURVE('',#2633,#2647,#1444,.T.);
#3429=EDGE_CURVE('',#2634,#2646,#1445,.T.);
#3430=EDGE_CURVE('',#2679,#2546,#1446,.T.);
#3944=ORIENTED_EDGE('',*,*,#3024,.T.);
#3945=ORIENTED_EDGE('',*,*,#3025,.T.);
#3946=ORIENTED_EDGE('',*,*,#3026,.F.);
#3947=ORIENTED_EDGE('',*,*,#3027,.T.);
#3948=ORIENTED_EDGE('',*,*,#3028,.T.);
#3949=ORIENTED_EDGE('',*,*,#3029,.T.);
#3950=ORIENTED_EDGE('',*,*,#3028,.F.);
#3951=ORIENTED_EDGE('',*,*,#3030,.T.);
#3952=ORIENTED_EDGE('',*,*,#3031,.T.);
#3953=ORIENTED_EDGE('',*,*,#3032,.T.);
#3954=ORIENTED_EDGE('',*,*,#3024,.F.);
#3955=ORIENTED_EDGE('',*,*,#3033,.T.);
#3956=ORIENTED_EDGE('',*,*,#3034,.T.);
#3957=ORIENTED_EDGE('',*,*,#3035,.T.);
#3958=ORIENTED_EDGE('',*,*,#3031,.F.);
#3959=ORIENTED_EDGE('',*,*,#3036,.T.);
#3960=ORIENTED_EDGE('',*,*,#3037,.T.);
#3961=ORIENTED_EDGE('',*,*,#3038,.T.);
#3962=ORIENTED_EDGE('',*,*,#3034,.F.);
#3963=ORIENTED_EDGE('',*,*,#3039,.T.);
#3964=ORIENTED_EDGE('',*,*,#3040,.T.);
#3965=ORIENTED_EDGE('',*,*,#3041,.T.);
#3966=ORIENTED_EDGE('',*,*,#3037,.F.);
#3967=ORIENTED_EDGE('',*,*,#3042,.T.);
#3968=ORIENTED_EDGE('',*,*,#3043,.T.);
#3969=ORIENTED_EDGE('',*,*,#3044,.T.);
#3970=ORIENTED_EDGE('',*,*,#3040,.F.);
#3971=ORIENTED_EDGE('',*,*,#3045,.T.);
#3972=ORIENTED_EDGE('',*,*,#3046,.T.);
#3973=ORIENTED_EDGE('',*,*,#3047,.T.);
#3974=ORIENTED_EDGE('',*,*,#3043,.F.);
#3975=ORIENTED_EDGE('',*,*,#3048,.T.);
#3976=ORIENTED_EDGE('',*,*,#3049,.T.);
#3977=ORIENTED_EDGE('',*,*,#3050,.T.);
#3978=ORIENTED_EDGE('',*,*,#3046,.F.);
#3979=ORIENTED_EDGE('',*,*,#3051,.T.);
#3980=ORIENTED_EDGE('',*,*,#3052,.T.);
#3981=ORIENTED_EDGE('',*,*,#3053,.T.);
#3982=ORIENTED_EDGE('',*,*,#3049,.F.);
#3983=ORIENTED_EDGE('',*,*,#3054,.T.);
#3984=ORIENTED_EDGE('',*,*,#3055,.T.);
#3985=ORIENTED_EDGE('',*,*,#3056,.T.);
#3986=ORIENTED_EDGE('',*,*,#3052,.F.);
#3987=ORIENTED_EDGE('',*,*,#3057,.T.);
#3988=ORIENTED_EDGE('',*,*,#3058,.T.);
#3989=ORIENTED_EDGE('',*,*,#3059,.T.);
#3990=ORIENTED_EDGE('',*,*,#3055,.F.);
#3991=ORIENTED_EDGE('',*,*,#3060,.T.);
#3992=ORIENTED_EDGE('',*,*,#3061,.T.);
#3993=ORIENTED_EDGE('',*,*,#3062,.T.);
#3994=ORIENTED_EDGE('',*,*,#3058,.F.);
#3995=ORIENTED_EDGE('',*,*,#3063,.T.);
#3996=ORIENTED_EDGE('',*,*,#3064,.T.);
#3997=ORIENTED_EDGE('',*,*,#3065,.T.);
#3998=ORIENTED_EDGE('',*,*,#3061,.F.);
#3999=ORIENTED_EDGE('',*,*,#3066,.T.);
#4000=ORIENTED_EDGE('',*,*,#3067,.T.);
#4001=ORIENTED_EDGE('',*,*,#3068,.T.);
#4002=ORIENTED_EDGE('',*,*,#3064,.F.);
#4003=ORIENTED_EDGE('',*,*,#3069,.T.);
#4004=ORIENTED_EDGE('',*,*,#3070,.T.);
#4005=ORIENTED_EDGE('',*,*,#3071,.T.);
#4006=ORIENTED_EDGE('',*,*,#3067,.F.);
#4007=ORIENTED_EDGE('',*,*,#3072,.T.);
#4008=ORIENTED_EDGE('',*,*,#3073,.T.);
#4009=ORIENTED_EDGE('',*,*,#3074,.T.);
#4010=ORIENTED_EDGE('',*,*,#3070,.F.);
#4011=ORIENTED_EDGE('',*,*,#3075,.T.);
#4012=ORIENTED_EDGE('',*,*,#3076,.T.);
#4013=ORIENTED_EDGE('',*,*,#3077,.T.);
#4014=ORIENTED_EDGE('',*,*,#3073,.F.);
#4015=ORIENTED_EDGE('',*,*,#3078,.T.);
#4016=ORIENTED_EDGE('',*,*,#3079,.T.);
#4017=ORIENTED_EDGE('',*,*,#3080,.T.);
#4018=ORIENTED_EDGE('',*,*,#3076,.F.);
#4019=ORIENTED_EDGE('',*,*,#3081,.T.);
#4020=ORIENTED_EDGE('',*,*,#3082,.T.);
#4021=ORIENTED_EDGE('',*,*,#3083,.T.);
#4022=ORIENTED_EDGE('',*,*,#3079,.F.);
#4023=ORIENTED_EDGE('',*,*,#3084,.T.);
#4024=ORIENTED_EDGE('',*,*,#3085,.T.);
#4025=ORIENTED_EDGE('',*,*,#3086,.T.);
#4026=ORIENTED_EDGE('',*,*,#3082,.F.);
#4027=ORIENTED_EDGE('',*,*,#3087,.T.);
#4028=ORIENTED_EDGE('',*,*,#3088,.T.);
#4029=ORIENTED_EDGE('',*,*,#3089,.T.);
#4030=ORIENTED_EDGE('',*,*,#3085,.F.);
#4031=ORIENTED_EDGE('',*,*,#3090,.T.);
#4032=ORIENTED_EDGE('',*,*,#3091,.F.);
#4033=ORIENTED_EDGE('',*,*,#3092,.T.);
#4034=ORIENTED_EDGE('',*,*,#3093,.T.);
#4035=ORIENTED_EDGE('',*,*,#3094,.T.);
#4036=ORIENTED_EDGE('',*,*,#3095,.F.);
#4037=ORIENTED_EDGE('',*,*,#3096,.F.);
#4038=ORIENTED_EDGE('',*,*,#3097,.T.);
#4039=ORIENTED_EDGE('',*,*,#3098,.F.);
#4040=ORIENTED_EDGE('',*,*,#3097,.F.);
#4041=ORIENTED_EDGE('',*,*,#3099,.F.);
#4042=ORIENTED_EDGE('',*,*,#3100,.T.);
#4043=ORIENTED_EDGE('',*,*,#3101,.F.);
#4044=ORIENTED_EDGE('',*,*,#3102,.F.);
#4045=ORIENTED_EDGE('',*,*,#3100,.F.);
#4046=ORIENTED_EDGE('',*,*,#3103,.F.);
#4047=ORIENTED_EDGE('',*,*,#3104,.F.);
#4048=ORIENTED_EDGE('',*,*,#3105,.F.);
#4049=ORIENTED_EDGE('',*,*,#3106,.T.);
#4050=ORIENTED_EDGE('',*,*,#3107,.T.);
#4051=ORIENTED_EDGE('',*,*,#3108,.F.);
#4052=ORIENTED_EDGE('',*,*,#3109,.F.);
#4053=ORIENTED_EDGE('',*,*,#3110,.F.);
#4054=ORIENTED_EDGE('',*,*,#3111,.F.);
#4055=ORIENTED_EDGE('',*,*,#3105,.T.);
#4056=ORIENTED_EDGE('',*,*,#3112,.F.);
#4057=ORIENTED_EDGE('',*,*,#3113,.F.);
#4058=ORIENTED_EDGE('',*,*,#3114,.F.);
#4059=ORIENTED_EDGE('',*,*,#3115,.T.);
#4060=ORIENTED_EDGE('',*,*,#3116,.F.);
#4061=ORIENTED_EDGE('',*,*,#3117,.T.);
#4062=ORIENTED_EDGE('',*,*,#3118,.F.);
#4063=ORIENTED_EDGE('',*,*,#3119,.T.);
#4064=ORIENTED_EDGE('',*,*,#3120,.T.);
#4065=ORIENTED_EDGE('',*,*,#3121,.F.);
#4066=ORIENTED_EDGE('',*,*,#3122,.F.);
#4067=ORIENTED_EDGE('',*,*,#3123,.F.);
#4068=ORIENTED_EDGE('',*,*,#3029,.F.);
#4069=ORIENTED_EDGE('',*,*,#3124,.T.);
#4070=ORIENTED_EDGE('',*,*,#3125,.F.);
#4071=ORIENTED_EDGE('',*,*,#3124,.F.);
#4072=ORIENTED_EDGE('',*,*,#3126,.T.);
#4073=ORIENTED_EDGE('',*,*,#3127,.T.);
#4074=ORIENTED_EDGE('',*,*,#3128,.F.);
#4075=ORIENTED_EDGE('',*,*,#3129,.T.);
#4076=ORIENTED_EDGE('',*,*,#3130,.T.);
#4077=ORIENTED_EDGE('',*,*,#3131,.F.);
#4078=ORIENTED_EDGE('',*,*,#3132,.T.);
#4079=ORIENTED_EDGE('',*,*,#3133,.F.);
#4080=ORIENTED_EDGE('',*,*,#3134,.T.);
#4081=ORIENTED_EDGE('',*,*,#3135,.F.);
#4082=ORIENTED_EDGE('',*,*,#3136,.F.);
#4083=ORIENTED_EDGE('',*,*,#3137,.T.);
#4084=ORIENTED_EDGE('',*,*,#3138,.F.);
#4085=ORIENTED_EDGE('',*,*,#3139,.T.);
#4086=ORIENTED_EDGE('',*,*,#3140,.F.);
#4087=ORIENTED_EDGE('',*,*,#3141,.T.);
#4088=ORIENTED_EDGE('',*,*,#3091,.T.);
#4089=ORIENTED_EDGE('',*,*,#3142,.T.);
#4090=ORIENTED_EDGE('',*,*,#3088,.F.);
#4091=ORIENTED_EDGE('',*,*,#3143,.T.);
#4092=ORIENTED_EDGE('',*,*,#3144,.T.);
#4093=ORIENTED_EDGE('',*,*,#3145,.T.);
#4094=ORIENTED_EDGE('',*,*,#3146,.F.);
#4095=ORIENTED_EDGE('',*,*,#3145,.F.);
#4096=ORIENTED_EDGE('',*,*,#3147,.T.);
#4097=ORIENTED_EDGE('',*,*,#3148,.T.);
#4098=ORIENTED_EDGE('',*,*,#3149,.F.);
#4099=ORIENTED_EDGE('',*,*,#3148,.F.);
#4100=ORIENTED_EDGE('',*,*,#3150,.T.);
#4101=ORIENTED_EDGE('',*,*,#3151,.T.);
#4102=ORIENTED_EDGE('',*,*,#3152,.F.);
#4103=ORIENTED_EDGE('',*,*,#3151,.F.);
#4104=ORIENTED_EDGE('',*,*,#3095,.T.);
#4105=ORIENTED_EDGE('',*,*,#3096,.T.);
#4106=ORIENTED_EDGE('',*,*,#3153,.T.);
#4107=ORIENTED_EDGE('',*,*,#3135,.T.);
#4108=ORIENTED_EDGE('',*,*,#3154,.T.);
#4109=ORIENTED_EDGE('',*,*,#3155,.T.);
#4110=ORIENTED_EDGE('',*,*,#3156,.T.);
#4111=ORIENTED_EDGE('',*,*,#3101,.T.);
#4112=ORIENTED_EDGE('',*,*,#3102,.T.);
#4113=ORIENTED_EDGE('',*,*,#3156,.F.);
#4114=ORIENTED_EDGE('',*,*,#3157,.T.);
#4115=ORIENTED_EDGE('',*,*,#3158,.T.);
#4116=ORIENTED_EDGE('',*,*,#3136,.T.);
#4117=ORIENTED_EDGE('',*,*,#3153,.F.);
#4118=ORIENTED_EDGE('',*,*,#3128,.T.);
#4119=ORIENTED_EDGE('',*,*,#3159,.T.);
#4120=ORIENTED_EDGE('',*,*,#3160,.T.);
#4121=ORIENTED_EDGE('',*,*,#3161,.T.);
#4122=ORIENTED_EDGE('',*,*,#3162,.T.);
#4123=ORIENTED_EDGE('',*,*,#3140,.T.);
#4124=ORIENTED_EDGE('',*,*,#3163,.T.);
#4125=ORIENTED_EDGE('',*,*,#3164,.T.);
#4126=ORIENTED_EDGE('',*,*,#3165,.T.);
#4127=ORIENTED_EDGE('',*,*,#3166,.T.);
#4128=ORIENTED_EDGE('',*,*,#3167,.T.);
#4129=ORIENTED_EDGE('',*,*,#3168,.T.);
#4130=ORIENTED_EDGE('',*,*,#3169,.T.);
#4131=ORIENTED_EDGE('',*,*,#3170,.T.);
#4132=ORIENTED_EDGE('',*,*,#3125,.T.);
#4133=ORIENTED_EDGE('',*,*,#3171,.T.);
#4134=ORIENTED_EDGE('',*,*,#3172,.T.);
#4135=ORIENTED_EDGE('',*,*,#3173,.T.);
#4136=ORIENTED_EDGE('',*,*,#3174,.T.);
#4137=ORIENTED_EDGE('',*,*,#3175,.T.);
#4138=ORIENTED_EDGE('',*,*,#3176,.T.);
#4139=ORIENTED_EDGE('',*,*,#3177,.T.);
#4140=ORIENTED_EDGE('',*,*,#3178,.T.);
#4141=ORIENTED_EDGE('',*,*,#3179,.T.);
#4142=ORIENTED_EDGE('',*,*,#3180,.T.);
#4143=ORIENTED_EDGE('',*,*,#3181,.T.);
#4144=ORIENTED_EDGE('',*,*,#3182,.T.);
#4145=ORIENTED_EDGE('',*,*,#3183,.T.);
#4146=ORIENTED_EDGE('',*,*,#3184,.T.);
#4147=ORIENTED_EDGE('',*,*,#3185,.T.);
#4148=ORIENTED_EDGE('',*,*,#3186,.T.);
#4149=ORIENTED_EDGE('',*,*,#3187,.T.);
#4150=ORIENTED_EDGE('',*,*,#3188,.T.);
#4151=ORIENTED_EDGE('',*,*,#3189,.T.);
#4152=ORIENTED_EDGE('',*,*,#3190,.T.);
#4153=ORIENTED_EDGE('',*,*,#3191,.T.);
#4154=ORIENTED_EDGE('',*,*,#3192,.T.);
#4155=ORIENTED_EDGE('',*,*,#3193,.T.);
#4156=ORIENTED_EDGE('',*,*,#3194,.T.);
#4157=ORIENTED_EDGE('',*,*,#3195,.T.);
#4158=ORIENTED_EDGE('',*,*,#3196,.T.);
#4159=ORIENTED_EDGE('',*,*,#3197,.T.);
#4160=ORIENTED_EDGE('',*,*,#3198,.T.);
#4161=ORIENTED_EDGE('',*,*,#3199,.T.);
#4162=ORIENTED_EDGE('',*,*,#3200,.T.);
#4163=ORIENTED_EDGE('',*,*,#3098,.T.);
#4164=ORIENTED_EDGE('',*,*,#3201,.F.);
#4165=ORIENTED_EDGE('',*,*,#3202,.F.);
#4166=ORIENTED_EDGE('',*,*,#3203,.T.);
#4167=ORIENTED_EDGE('',*,*,#3204,.T.);
#4168=ORIENTED_EDGE('',*,*,#3205,.T.);
#4169=ORIENTED_EDGE('',*,*,#3203,.F.);
#4170=ORIENTED_EDGE('',*,*,#3206,.T.);
#4171=ORIENTED_EDGE('',*,*,#3207,.T.);
#4172=ORIENTED_EDGE('',*,*,#3093,.F.);
#4173=ORIENTED_EDGE('',*,*,#3208,.T.);
#4174=ORIENTED_EDGE('',*,*,#3209,.T.);
#4175=ORIENTED_EDGE('',*,*,#3210,.T.);
#4176=ORIENTED_EDGE('',*,*,#3211,.T.);
#4177=ORIENTED_EDGE('',*,*,#3212,.T.);
#4178=ORIENTED_EDGE('',*,*,#3213,.T.);
#4179=ORIENTED_EDGE('',*,*,#3150,.F.);
#4180=ORIENTED_EDGE('',*,*,#3214,.T.);
#4181=ORIENTED_EDGE('',*,*,#3215,.T.);
#4182=ORIENTED_EDGE('',*,*,#3216,.T.);
#4183=ORIENTED_EDGE('',*,*,#3217,.T.);
#4184=ORIENTED_EDGE('',*,*,#3218,.T.);
#4185=ORIENTED_EDGE('',*,*,#3219,.T.);
#4186=ORIENTED_EDGE('',*,*,#3152,.T.);
#4187=ORIENTED_EDGE('',*,*,#3220,.F.);
#4188=ORIENTED_EDGE('',*,*,#3221,.T.);
#4189=ORIENTED_EDGE('',*,*,#3222,.T.);
#4190=ORIENTED_EDGE('',*,*,#3223,.T.);
#4191=ORIENTED_EDGE('',*,*,#3224,.F.);
#4192=ORIENTED_EDGE('',*,*,#3225,.T.);
#4193=ORIENTED_EDGE('',*,*,#3220,.T.);
#4194=ORIENTED_EDGE('',*,*,#3226,.T.);
#4195=ORIENTED_EDGE('',*,*,#3227,.F.);
#4196=ORIENTED_EDGE('',*,*,#3228,.T.);
#4197=ORIENTED_EDGE('',*,*,#3224,.T.);
#4198=ORIENTED_EDGE('',*,*,#3229,.T.);
#4199=ORIENTED_EDGE('',*,*,#3230,.F.);
#4200=ORIENTED_EDGE('',*,*,#3231,.T.);
#4201=ORIENTED_EDGE('',*,*,#3227,.T.);
#4202=ORIENTED_EDGE('',*,*,#3232,.T.);
#4203=ORIENTED_EDGE('',*,*,#3233,.T.);
#4204=ORIENTED_EDGE('',*,*,#3234,.T.);
#4205=ORIENTED_EDGE('',*,*,#3235,.T.);
#4206=ORIENTED_EDGE('',*,*,#3230,.T.);
#4207=ORIENTED_EDGE('',*,*,#3138,.T.);
#4208=ORIENTED_EDGE('',*,*,#3236,.T.);
#4209=ORIENTED_EDGE('',*,*,#3237,.T.);
#4210=ORIENTED_EDGE('',*,*,#3238,.T.);
#4211=ORIENTED_EDGE('',*,*,#3239,.T.);
#4212=ORIENTED_EDGE('',*,*,#3240,.T.);
#4213=ORIENTED_EDGE('',*,*,#3241,.T.);
#4214=ORIENTED_EDGE('',*,*,#3242,.T.);
#4215=ORIENTED_EDGE('',*,*,#3243,.T.);
#4216=ORIENTED_EDGE('',*,*,#3244,.T.);
#4217=ORIENTED_EDGE('',*,*,#3245,.T.);
#4218=ORIENTED_EDGE('',*,*,#3246,.T.);
#4219=ORIENTED_EDGE('',*,*,#3247,.T.);
#4220=ORIENTED_EDGE('',*,*,#3248,.T.);
#4221=ORIENTED_EDGE('',*,*,#3147,.F.);
#4222=ORIENTED_EDGE('',*,*,#3249,.F.);
#4223=ORIENTED_EDGE('',*,*,#3250,.T.);
#4224=ORIENTED_EDGE('',*,*,#3251,.T.);
#4225=ORIENTED_EDGE('',*,*,#3252,.T.);
#4226=ORIENTED_EDGE('',*,*,#3249,.T.);
#4227=ORIENTED_EDGE('',*,*,#3253,.T.);
#4228=ORIENTED_EDGE('',*,*,#3254,.F.);
#4229=ORIENTED_EDGE('',*,*,#3255,.T.);
#4230=ORIENTED_EDGE('',*,*,#3254,.T.);
#4231=ORIENTED_EDGE('',*,*,#3108,.T.);
#4232=ORIENTED_EDGE('',*,*,#3256,.F.);
#4233=ORIENTED_EDGE('',*,*,#3257,.T.);
#4234=ORIENTED_EDGE('',*,*,#3256,.T.);
#4235=ORIENTED_EDGE('',*,*,#3258,.T.);
#4236=ORIENTED_EDGE('',*,*,#3259,.F.);
#4237=ORIENTED_EDGE('',*,*,#3260,.T.);
#4238=ORIENTED_EDGE('',*,*,#3112,.T.);
#4239=ORIENTED_EDGE('',*,*,#3261,.T.);
#4240=ORIENTED_EDGE('',*,*,#3262,.T.);
#4241=ORIENTED_EDGE('',*,*,#3259,.T.);
#4242=ORIENTED_EDGE('',*,*,#3133,.T.);
#4243=ORIENTED_EDGE('',*,*,#3263,.T.);
#4244=ORIENTED_EDGE('',*,*,#3264,.T.);
#4245=ORIENTED_EDGE('',*,*,#3265,.T.);
#4246=ORIENTED_EDGE('',*,*,#3266,.T.);
#4247=ORIENTED_EDGE('',*,*,#3103,.T.);
#4248=ORIENTED_EDGE('',*,*,#3267,.T.);
#4249=ORIENTED_EDGE('',*,*,#3268,.T.);
#4250=ORIENTED_EDGE('',*,*,#3269,.T.);
#4251=ORIENTED_EDGE('',*,*,#3270,.T.);
#4252=ORIENTED_EDGE('',*,*,#3114,.T.);
#4253=ORIENTED_EDGE('',*,*,#3111,.T.);
#4254=ORIENTED_EDGE('',*,*,#3271,.T.);
#4255=ORIENTED_EDGE('',*,*,#3272,.T.);
#4256=ORIENTED_EDGE('',*,*,#3149,.T.);
#4257=ORIENTED_EDGE('',*,*,#3118,.T.);
#4258=ORIENTED_EDGE('',*,*,#3273,.T.);
#4259=ORIENTED_EDGE('',*,*,#3274,.T.);
#4260=ORIENTED_EDGE('',*,*,#3275,.T.);
#4261=ORIENTED_EDGE('',*,*,#3276,.T.);
#4262=ORIENTED_EDGE('',*,*,#3123,.T.);
#4263=ORIENTED_EDGE('',*,*,#3144,.F.);
#4264=ORIENTED_EDGE('',*,*,#3277,.F.);
#4265=ORIENTED_EDGE('',*,*,#3278,.T.);
#4266=ORIENTED_EDGE('',*,*,#3131,.T.);
#4267=ORIENTED_EDGE('',*,*,#3279,.T.);
#4268=ORIENTED_EDGE('',*,*,#3277,.T.);
#4269=ORIENTED_EDGE('',*,*,#3280,.T.);
#4270=ORIENTED_EDGE('',*,*,#3281,.F.);
#4271=ORIENTED_EDGE('',*,*,#3282,.T.);
#4272=ORIENTED_EDGE('',*,*,#3281,.T.);
#4273=ORIENTED_EDGE('',*,*,#3283,.T.);
#4274=ORIENTED_EDGE('',*,*,#3284,.F.);
#4275=ORIENTED_EDGE('',*,*,#3121,.T.);
#4276=ORIENTED_EDGE('',*,*,#3284,.T.);
#4277=ORIENTED_EDGE('',*,*,#3285,.T.);
#4278=ORIENTED_EDGE('',*,*,#3286,.F.);
#4279=ORIENTED_EDGE('',*,*,#3287,.T.);
#4280=ORIENTED_EDGE('',*,*,#3288,.T.);
#4281=ORIENTED_EDGE('',*,*,#3289,.T.);
#4282=ORIENTED_EDGE('',*,*,#3116,.T.);
#4283=ORIENTED_EDGE('',*,*,#3286,.T.);
#4284=ORIENTED_EDGE('',*,*,#3290,.T.);
#4285=ORIENTED_EDGE('',*,*,#3291,.T.);
#4286=ORIENTED_EDGE('',*,*,#3292,.T.);
#4287=ORIENTED_EDGE('',*,*,#3293,.T.);
#4288=ORIENTED_EDGE('',*,*,#3294,.T.);
#4289=ORIENTED_EDGE('',*,*,#3295,.T.);
#4290=ORIENTED_EDGE('',*,*,#3296,.T.);
#4291=ORIENTED_EDGE('',*,*,#3297,.T.);
#4292=ORIENTED_EDGE('',*,*,#3298,.T.);
#4293=ORIENTED_EDGE('',*,*,#3299,.T.);
#4294=ORIENTED_EDGE('',*,*,#3300,.T.);
#4295=ORIENTED_EDGE('',*,*,#3301,.T.);
#4296=ORIENTED_EDGE('',*,*,#3302,.T.);
#4297=ORIENTED_EDGE('',*,*,#3303,.T.);
#4298=ORIENTED_EDGE('',*,*,#3146,.T.);
#4299=ORIENTED_EDGE('',*,*,#3163,.F.);
#4300=ORIENTED_EDGE('',*,*,#3304,.T.);
#4301=ORIENTED_EDGE('',*,*,#3305,.T.);
#4302=ORIENTED_EDGE('',*,*,#3214,.F.);
#4303=ORIENTED_EDGE('',*,*,#3306,.T.);
#4304=ORIENTED_EDGE('',*,*,#3307,.T.);
#4305=ORIENTED_EDGE('',*,*,#3308,.T.);
#4306=ORIENTED_EDGE('',*,*,#3159,.F.);
#4307=ORIENTED_EDGE('',*,*,#3309,.T.);
#4308=ORIENTED_EDGE('',*,*,#3274,.F.);
#4309=ORIENTED_EDGE('',*,*,#3161,.F.);
#4310=ORIENTED_EDGE('',*,*,#3310,.T.);
#4311=ORIENTED_EDGE('',*,*,#3311,.T.);
#4312=ORIENTED_EDGE('',*,*,#3298,.F.);
#4313=ORIENTED_EDGE('',*,*,#3312,.T.);
#4314=ORIENTED_EDGE('',*,*,#3313,.T.);
#4315=ORIENTED_EDGE('',*,*,#3314,.T.);
#4316=ORIENTED_EDGE('',*,*,#3158,.F.);
#4317=ORIENTED_EDGE('',*,*,#3315,.T.);
#4318=ORIENTED_EDGE('',*,*,#3245,.F.);
#4319=ORIENTED_EDGE('',*,*,#3154,.F.);
#4320=ORIENTED_EDGE('',*,*,#3316,.T.);
#4321=ORIENTED_EDGE('',*,*,#3317,.T.);
#4322=ORIENTED_EDGE('',*,*,#3269,.F.);
#4323=ORIENTED_EDGE('',*,*,#3318,.T.);
#4324=ORIENTED_EDGE('',*,*,#3319,.T.);
#4325=ORIENTED_EDGE('',*,*,#3320,.T.);
#4326=ORIENTED_EDGE('',*,*,#3162,.F.);
#4327=ORIENTED_EDGE('',*,*,#3321,.T.);
#4328=ORIENTED_EDGE('',*,*,#3210,.F.);
#4329=ORIENTED_EDGE('',*,*,#3160,.F.);
#4330=ORIENTED_EDGE('',*,*,#3322,.T.);
#4331=ORIENTED_EDGE('',*,*,#3290,.F.);
#4332=ORIENTED_EDGE('',*,*,#3323,.T.);
#4333=ORIENTED_EDGE('',*,*,#3155,.F.);
#4334=ORIENTED_EDGE('',*,*,#3324,.T.);
#4335=ORIENTED_EDGE('',*,*,#3325,.T.);
#4336=ORIENTED_EDGE('',*,*,#3251,.F.);
#4337=ORIENTED_EDGE('',*,*,#3326,.T.);
#4338=ORIENTED_EDGE('',*,*,#3327,.T.);
#4339=ORIENTED_EDGE('',*,*,#3157,.F.);
#4340=ORIENTED_EDGE('',*,*,#3328,.T.);
#4341=ORIENTED_EDGE('',*,*,#3329,.T.);
#4342=ORIENTED_EDGE('',*,*,#3164,.F.);
#4343=ORIENTED_EDGE('',*,*,#3330,.T.);
#4344=ORIENTED_EDGE('',*,*,#3331,.T.);
#4345=ORIENTED_EDGE('',*,*,#3222,.F.);
#4346=ORIENTED_EDGE('',*,*,#3026,.T.);
#4347=ORIENTED_EDGE('',*,*,#3332,.F.);
#4348=ORIENTED_EDGE('',*,*,#3333,.F.);
#4349=ORIENTED_EDGE('',*,*,#3334,.F.);
#4350=ORIENTED_EDGE('',*,*,#3335,.F.);
#4351=ORIENTED_EDGE('',*,*,#3201,.T.);
#4352=ORIENTED_EDGE('',*,*,#3205,.F.);
#4353=ORIENTED_EDGE('',*,*,#3336,.T.);
#4354=ORIENTED_EDGE('',*,*,#3334,.T.);
#4355=ORIENTED_EDGE('',*,*,#3337,.F.);
#4356=ORIENTED_EDGE('',*,*,#3335,.T.);
#4357=ORIENTED_EDGE('',*,*,#3336,.F.);
#4358=ORIENTED_EDGE('',*,*,#3204,.F.);
#4359=ORIENTED_EDGE('',*,*,#3092,.F.);
#4360=ORIENTED_EDGE('',*,*,#3143,.F.);
#4361=ORIENTED_EDGE('',*,*,#3090,.F.);
#4362=ORIENTED_EDGE('',*,*,#3087,.F.);
#4363=ORIENTED_EDGE('',*,*,#3084,.F.);
#4364=ORIENTED_EDGE('',*,*,#3081,.F.);
#4365=ORIENTED_EDGE('',*,*,#3078,.F.);
#4366=ORIENTED_EDGE('',*,*,#3075,.F.);
#4367=ORIENTED_EDGE('',*,*,#3072,.F.);
#4368=ORIENTED_EDGE('',*,*,#3069,.F.);
#4369=ORIENTED_EDGE('',*,*,#3066,.F.);
#4370=ORIENTED_EDGE('',*,*,#3063,.F.);
#4371=ORIENTED_EDGE('',*,*,#3060,.F.);
#4372=ORIENTED_EDGE('',*,*,#3057,.F.);
#4373=ORIENTED_EDGE('',*,*,#3054,.F.);
#4374=ORIENTED_EDGE('',*,*,#3051,.F.);
#4375=ORIENTED_EDGE('',*,*,#3048,.F.);
#4376=ORIENTED_EDGE('',*,*,#3045,.F.);
#4377=ORIENTED_EDGE('',*,*,#3042,.F.);
#4378=ORIENTED_EDGE('',*,*,#3039,.F.);
#4379=ORIENTED_EDGE('',*,*,#3036,.F.);
#4380=ORIENTED_EDGE('',*,*,#3033,.F.);
#4381=ORIENTED_EDGE('',*,*,#3030,.F.);
#4382=ORIENTED_EDGE('',*,*,#3027,.F.);
#4383=ORIENTED_EDGE('',*,*,#3202,.T.);
#4384=ORIENTED_EDGE('',*,*,#3337,.T.);
#4385=ORIENTED_EDGE('',*,*,#3333,.T.);
#4386=ORIENTED_EDGE('',*,*,#3338,.F.);
#4387=ORIENTED_EDGE('',*,*,#3206,.F.);
#4388=ORIENTED_EDGE('',*,*,#3207,.F.);
#4389=ORIENTED_EDGE('',*,*,#3338,.T.);
#4390=ORIENTED_EDGE('',*,*,#3332,.T.);
#4391=ORIENTED_EDGE('',*,*,#3025,.F.);
#4392=ORIENTED_EDGE('',*,*,#3032,.F.);
#4393=ORIENTED_EDGE('',*,*,#3035,.F.);
#4394=ORIENTED_EDGE('',*,*,#3038,.F.);
#4395=ORIENTED_EDGE('',*,*,#3041,.F.);
#4396=ORIENTED_EDGE('',*,*,#3044,.F.);
#4397=ORIENTED_EDGE('',*,*,#3047,.F.);
#4398=ORIENTED_EDGE('',*,*,#3050,.F.);
#4399=ORIENTED_EDGE('',*,*,#3053,.F.);
#4400=ORIENTED_EDGE('',*,*,#3056,.F.);
#4401=ORIENTED_EDGE('',*,*,#3059,.F.);
#4402=ORIENTED_EDGE('',*,*,#3062,.F.);
#4403=ORIENTED_EDGE('',*,*,#3065,.F.);
#4404=ORIENTED_EDGE('',*,*,#3068,.F.);
#4405=ORIENTED_EDGE('',*,*,#3071,.F.);
#4406=ORIENTED_EDGE('',*,*,#3074,.F.);
#4407=ORIENTED_EDGE('',*,*,#3077,.F.);
#4408=ORIENTED_EDGE('',*,*,#3080,.F.);
#4409=ORIENTED_EDGE('',*,*,#3083,.F.);
#4410=ORIENTED_EDGE('',*,*,#3086,.F.);
#4411=ORIENTED_EDGE('',*,*,#3089,.F.);
#4412=ORIENTED_EDGE('',*,*,#3142,.F.);
#4413=ORIENTED_EDGE('',*,*,#3094,.F.);
#4414=ORIENTED_EDGE('',*,*,#3099,.T.);
#4415=ORIENTED_EDGE('',*,*,#3339,.T.);
#4416=ORIENTED_EDGE('',*,*,#3340,.T.);
#4417=ORIENTED_EDGE('',*,*,#3341,.T.);
#4418=ORIENTED_EDGE('',*,*,#3342,.T.);
#4419=ORIENTED_EDGE('',*,*,#3343,.T.);
#4420=ORIENTED_EDGE('',*,*,#3344,.T.);
#4421=ORIENTED_EDGE('',*,*,#3345,.T.);
#4422=ORIENTED_EDGE('',*,*,#3346,.T.);
#4423=ORIENTED_EDGE('',*,*,#3347,.T.);
#4424=ORIENTED_EDGE('',*,*,#3348,.T.);
#4425=ORIENTED_EDGE('',*,*,#3349,.T.);
#4426=ORIENTED_EDGE('',*,*,#3350,.T.);
#4427=ORIENTED_EDGE('',*,*,#3174,.F.);
#4428=ORIENTED_EDGE('',*,*,#3351,.T.);
#4429=ORIENTED_EDGE('',*,*,#3200,.F.);
#4430=ORIENTED_EDGE('',*,*,#3166,.F.);
#4431=ORIENTED_EDGE('',*,*,#3199,.F.);
#4432=ORIENTED_EDGE('',*,*,#3352,.T.);
#4433=ORIENTED_EDGE('',*,*,#3195,.F.);
#4434=ORIENTED_EDGE('',*,*,#3167,.F.);
#4435=ORIENTED_EDGE('',*,*,#3194,.F.);
#4436=ORIENTED_EDGE('',*,*,#3353,.T.);
#4437=ORIENTED_EDGE('',*,*,#3190,.F.);
#4438=ORIENTED_EDGE('',*,*,#3168,.F.);
#4439=ORIENTED_EDGE('',*,*,#3189,.F.);
#4440=ORIENTED_EDGE('',*,*,#3354,.T.);
#4441=ORIENTED_EDGE('',*,*,#3185,.F.);
#4442=ORIENTED_EDGE('',*,*,#3169,.F.);
#4443=ORIENTED_EDGE('',*,*,#3184,.F.);
#4444=ORIENTED_EDGE('',*,*,#3355,.T.);
#4445=ORIENTED_EDGE('',*,*,#3180,.F.);
#4446=ORIENTED_EDGE('',*,*,#3170,.F.);
#4447=ORIENTED_EDGE('',*,*,#3179,.F.);
#4448=ORIENTED_EDGE('',*,*,#3356,.T.);
#4449=ORIENTED_EDGE('',*,*,#3175,.F.);
#4450=ORIENTED_EDGE('',*,*,#3165,.F.);
#4451=ORIENTED_EDGE('',*,*,#3183,.F.);
#4452=ORIENTED_EDGE('',*,*,#3357,.T.);
#4453=ORIENTED_EDGE('',*,*,#3176,.F.);
#4454=ORIENTED_EDGE('',*,*,#3355,.F.);
#4455=ORIENTED_EDGE('',*,*,#3188,.F.);
#4456=ORIENTED_EDGE('',*,*,#3358,.T.);
#4457=ORIENTED_EDGE('',*,*,#3181,.F.);
#4458=ORIENTED_EDGE('',*,*,#3354,.F.);
#4459=ORIENTED_EDGE('',*,*,#3193,.F.);
#4460=ORIENTED_EDGE('',*,*,#3359,.T.);
#4461=ORIENTED_EDGE('',*,*,#3186,.F.);
#4462=ORIENTED_EDGE('',*,*,#3353,.F.);
#4463=ORIENTED_EDGE('',*,*,#3198,.F.);
#4464=ORIENTED_EDGE('',*,*,#3360,.T.);
#4465=ORIENTED_EDGE('',*,*,#3191,.F.);
#4466=ORIENTED_EDGE('',*,*,#3352,.F.);
#4467=ORIENTED_EDGE('',*,*,#3173,.F.);
#4468=ORIENTED_EDGE('',*,*,#3361,.T.);
#4469=ORIENTED_EDGE('',*,*,#3196,.F.);
#4470=ORIENTED_EDGE('',*,*,#3351,.F.);
#4471=ORIENTED_EDGE('',*,*,#3178,.F.);
#4472=ORIENTED_EDGE('',*,*,#3362,.T.);
#4473=ORIENTED_EDGE('',*,*,#3171,.F.);
#4474=ORIENTED_EDGE('',*,*,#3356,.F.);
#4475=ORIENTED_EDGE('',*,*,#3363,.F.);
#4476=ORIENTED_EDGE('',*,*,#3361,.F.);
#4477=ORIENTED_EDGE('',*,*,#3364,.F.);
#4478=ORIENTED_EDGE('',*,*,#3346,.F.);
#4479=ORIENTED_EDGE('',*,*,#3364,.T.);
#4480=ORIENTED_EDGE('',*,*,#3172,.F.);
#4481=ORIENTED_EDGE('',*,*,#3365,.F.);
#4482=ORIENTED_EDGE('',*,*,#3347,.F.);
#4483=ORIENTED_EDGE('',*,*,#3363,.T.);
#4484=ORIENTED_EDGE('',*,*,#3345,.F.);
#4485=ORIENTED_EDGE('',*,*,#3366,.F.);
#4486=ORIENTED_EDGE('',*,*,#3197,.F.);
#4487=ORIENTED_EDGE('',*,*,#3365,.T.);
#4488=ORIENTED_EDGE('',*,*,#3362,.F.);
#4489=ORIENTED_EDGE('',*,*,#3367,.F.);
#4490=ORIENTED_EDGE('',*,*,#3348,.F.);
#4491=ORIENTED_EDGE('',*,*,#3366,.T.);
#4492=ORIENTED_EDGE('',*,*,#3344,.F.);
#4493=ORIENTED_EDGE('',*,*,#3368,.F.);
#4494=ORIENTED_EDGE('',*,*,#3360,.F.);
#4495=ORIENTED_EDGE('',*,*,#3367,.T.);
#4496=ORIENTED_EDGE('',*,*,#3177,.F.);
#4497=ORIENTED_EDGE('',*,*,#3369,.F.);
#4498=ORIENTED_EDGE('',*,*,#3349,.F.);
#4499=ORIENTED_EDGE('',*,*,#3368,.T.);
#4500=ORIENTED_EDGE('',*,*,#3343,.F.);
#4501=ORIENTED_EDGE('',*,*,#3370,.F.);
#4502=ORIENTED_EDGE('',*,*,#3192,.F.);
#4503=ORIENTED_EDGE('',*,*,#3369,.T.);
#4504=ORIENTED_EDGE('',*,*,#3357,.F.);
#4505=ORIENTED_EDGE('',*,*,#3371,.F.);
#4506=ORIENTED_EDGE('',*,*,#3350,.F.);
#4507=ORIENTED_EDGE('',*,*,#3370,.T.);
#4508=ORIENTED_EDGE('',*,*,#3342,.F.);
#4509=ORIENTED_EDGE('',*,*,#3372,.F.);
#4510=ORIENTED_EDGE('',*,*,#3359,.F.);
#4511=ORIENTED_EDGE('',*,*,#3371,.T.);
#4512=ORIENTED_EDGE('',*,*,#3182,.F.);
#4513=ORIENTED_EDGE('',*,*,#3373,.F.);
#4514=ORIENTED_EDGE('',*,*,#3339,.F.);
#4515=ORIENTED_EDGE('',*,*,#3372,.T.);
#4516=ORIENTED_EDGE('',*,*,#3341,.F.);
#4517=ORIENTED_EDGE('',*,*,#3374,.F.);
#4518=ORIENTED_EDGE('',*,*,#3187,.F.);
#4519=ORIENTED_EDGE('',*,*,#3373,.T.);
#4520=ORIENTED_EDGE('',*,*,#3358,.F.);
#4521=ORIENTED_EDGE('',*,*,#3374,.T.);
#4522=ORIENTED_EDGE('',*,*,#3340,.F.);
#4523=ORIENTED_EDGE('',*,*,#3235,.F.);
#4524=ORIENTED_EDGE('',*,*,#3375,.T.);
#4525=ORIENTED_EDGE('',*,*,#3208,.F.);
#4526=ORIENTED_EDGE('',*,*,#3376,.F.);
#4527=ORIENTED_EDGE('',*,*,#3231,.F.);
#4528=ORIENTED_EDGE('',*,*,#3376,.T.);
#4529=ORIENTED_EDGE('',*,*,#3377,.F.);
#4530=ORIENTED_EDGE('',*,*,#3377,.T.);
#4531=ORIENTED_EDGE('',*,*,#3213,.F.);
#4532=ORIENTED_EDGE('',*,*,#3378,.F.);
#4533=ORIENTED_EDGE('',*,*,#3228,.F.);
#4534=ORIENTED_EDGE('',*,*,#3225,.F.);
#4535=ORIENTED_EDGE('',*,*,#3378,.T.);
#4536=ORIENTED_EDGE('',*,*,#3379,.F.);
#4537=ORIENTED_EDGE('',*,*,#3379,.T.);
#4538=ORIENTED_EDGE('',*,*,#3212,.F.);
#4539=ORIENTED_EDGE('',*,*,#3380,.F.);
#4540=ORIENTED_EDGE('',*,*,#3221,.F.);
#4541=ORIENTED_EDGE('',*,*,#3380,.T.);
#4542=ORIENTED_EDGE('',*,*,#3211,.F.);
#4543=ORIENTED_EDGE('',*,*,#3381,.F.);
#4544=ORIENTED_EDGE('',*,*,#3328,.F.);
#4545=ORIENTED_EDGE('',*,*,#3321,.F.);
#4546=ORIENTED_EDGE('',*,*,#3329,.F.);
#4547=ORIENTED_EDGE('',*,*,#3381,.T.);
#4548=ORIENTED_EDGE('',*,*,#3216,.F.);
#4549=ORIENTED_EDGE('',*,*,#3382,.T.);
#4550=ORIENTED_EDGE('',*,*,#3233,.F.);
#4551=ORIENTED_EDGE('',*,*,#3383,.F.);
#4552=ORIENTED_EDGE('',*,*,#3383,.T.);
#4553=ORIENTED_EDGE('',*,*,#3232,.F.);
#4554=ORIENTED_EDGE('',*,*,#3384,.F.);
#4555=ORIENTED_EDGE('',*,*,#3384,.T.);
#4556=ORIENTED_EDGE('',*,*,#3229,.F.);
#4557=ORIENTED_EDGE('',*,*,#3385,.F.);
#4558=ORIENTED_EDGE('',*,*,#3217,.F.);
#4559=ORIENTED_EDGE('',*,*,#3385,.T.);
#4560=ORIENTED_EDGE('',*,*,#3226,.F.);
#4561=ORIENTED_EDGE('',*,*,#3386,.F.);
#4562=ORIENTED_EDGE('',*,*,#3386,.T.);
#4563=ORIENTED_EDGE('',*,*,#3223,.F.);
#4564=ORIENTED_EDGE('',*,*,#3387,.F.);
#4565=ORIENTED_EDGE('',*,*,#3218,.F.);
#4566=ORIENTED_EDGE('',*,*,#3387,.T.);
#4567=ORIENTED_EDGE('',*,*,#3331,.F.);
#4568=ORIENTED_EDGE('',*,*,#3388,.F.);
#4569=ORIENTED_EDGE('',*,*,#3219,.F.);
#4570=ORIENTED_EDGE('',*,*,#3388,.T.);
#4571=ORIENTED_EDGE('',*,*,#3330,.F.);
#4572=ORIENTED_EDGE('',*,*,#3306,.F.);
#4573=ORIENTED_EDGE('',*,*,#3300,.F.);
#4574=ORIENTED_EDGE('',*,*,#3389,.T.);
#4575=ORIENTED_EDGE('',*,*,#3288,.F.);
#4576=ORIENTED_EDGE('',*,*,#3390,.F.);
#4577=ORIENTED_EDGE('',*,*,#3390,.T.);
#4578=ORIENTED_EDGE('',*,*,#3285,.F.);
#4579=ORIENTED_EDGE('',*,*,#3391,.F.);
#4580=ORIENTED_EDGE('',*,*,#3391,.T.);
#4581=ORIENTED_EDGE('',*,*,#3283,.F.);
#4582=ORIENTED_EDGE('',*,*,#3392,.F.);
#4583=ORIENTED_EDGE('',*,*,#3301,.F.);
#4584=ORIENTED_EDGE('',*,*,#3392,.T.);
#4585=ORIENTED_EDGE('',*,*,#3280,.F.);
#4586=ORIENTED_EDGE('',*,*,#3393,.F.);
#4587=ORIENTED_EDGE('',*,*,#3393,.T.);
#4588=ORIENTED_EDGE('',*,*,#3279,.F.);
#4589=ORIENTED_EDGE('',*,*,#3394,.F.);
#4590=ORIENTED_EDGE('',*,*,#3302,.F.);
#4591=ORIENTED_EDGE('',*,*,#3394,.T.);
#4592=ORIENTED_EDGE('',*,*,#3130,.F.);
#4593=ORIENTED_EDGE('',*,*,#3395,.F.);
#4594=ORIENTED_EDGE('',*,*,#3303,.F.);
#4595=ORIENTED_EDGE('',*,*,#3395,.T.);
#4596=ORIENTED_EDGE('',*,*,#3129,.F.);
#4597=ORIENTED_EDGE('',*,*,#3312,.F.);
#4598=ORIENTED_EDGE('',*,*,#3309,.F.);
#4599=ORIENTED_EDGE('',*,*,#3127,.F.);
#4600=ORIENTED_EDGE('',*,*,#3126,.F.);
#4601=ORIENTED_EDGE('',*,*,#3396,.F.);
#4602=ORIENTED_EDGE('',*,*,#3396,.T.);
#4603=ORIENTED_EDGE('',*,*,#3132,.F.);
#4604=ORIENTED_EDGE('',*,*,#3397,.F.);
#4605=ORIENTED_EDGE('',*,*,#3275,.F.);
#4606=ORIENTED_EDGE('',*,*,#3397,.T.);
#4607=ORIENTED_EDGE('',*,*,#3278,.F.);
#4608=ORIENTED_EDGE('',*,*,#3398,.F.);
#4609=ORIENTED_EDGE('',*,*,#3276,.F.);
#4610=ORIENTED_EDGE('',*,*,#3398,.T.);
#4611=ORIENTED_EDGE('',*,*,#3282,.F.);
#4612=ORIENTED_EDGE('',*,*,#3120,.F.);
#4613=ORIENTED_EDGE('',*,*,#3119,.F.);
#4614=ORIENTED_EDGE('',*,*,#3122,.T.);
#4615=ORIENTED_EDGE('',*,*,#3287,.F.);
#4616=ORIENTED_EDGE('',*,*,#3115,.F.);
#4617=ORIENTED_EDGE('',*,*,#3113,.T.);
#4618=ORIENTED_EDGE('',*,*,#3258,.F.);
#4619=ORIENTED_EDGE('',*,*,#3107,.F.);
#4620=ORIENTED_EDGE('',*,*,#3110,.T.);
#4621=ORIENTED_EDGE('',*,*,#3109,.T.);
#4622=ORIENTED_EDGE('',*,*,#3253,.F.);
#4623=ORIENTED_EDGE('',*,*,#3399,.F.);
#4624=ORIENTED_EDGE('',*,*,#3399,.T.);
#4625=ORIENTED_EDGE('',*,*,#3252,.F.);
#4626=ORIENTED_EDGE('',*,*,#3400,.F.);
#4627=ORIENTED_EDGE('',*,*,#3271,.F.);
#4628=ORIENTED_EDGE('',*,*,#3400,.T.);
#4629=ORIENTED_EDGE('',*,*,#3325,.F.);
#4630=ORIENTED_EDGE('',*,*,#3401,.F.);
#4631=ORIENTED_EDGE('',*,*,#3272,.F.);
#4632=ORIENTED_EDGE('',*,*,#3401,.T.);
#4633=ORIENTED_EDGE('',*,*,#3324,.F.);
#4634=ORIENTED_EDGE('',*,*,#3318,.F.);
#4635=ORIENTED_EDGE('',*,*,#3315,.F.);
#4636=ORIENTED_EDGE('',*,*,#3327,.F.);
#4637=ORIENTED_EDGE('',*,*,#3402,.F.);
#4638=ORIENTED_EDGE('',*,*,#3402,.T.);
#4639=ORIENTED_EDGE('',*,*,#3326,.F.);
#4640=ORIENTED_EDGE('',*,*,#3403,.F.);
#4641=ORIENTED_EDGE('',*,*,#3246,.F.);
#4642=ORIENTED_EDGE('',*,*,#3403,.T.);
#4643=ORIENTED_EDGE('',*,*,#3250,.F.);
#4644=ORIENTED_EDGE('',*,*,#3404,.F.);
#4645=ORIENTED_EDGE('',*,*,#3247,.F.);
#4646=ORIENTED_EDGE('',*,*,#3404,.T.);
#4647=ORIENTED_EDGE('',*,*,#3255,.F.);
#4648=ORIENTED_EDGE('',*,*,#3405,.F.);
#4649=ORIENTED_EDGE('',*,*,#3405,.T.);
#4650=ORIENTED_EDGE('',*,*,#3257,.F.);
#4651=ORIENTED_EDGE('',*,*,#3406,.F.);
#4652=ORIENTED_EDGE('',*,*,#3248,.F.);
#4653=ORIENTED_EDGE('',*,*,#3406,.T.);
#4654=ORIENTED_EDGE('',*,*,#3260,.F.);
#4655=ORIENTED_EDGE('',*,*,#3407,.F.);
#4656=ORIENTED_EDGE('',*,*,#3262,.F.);
#4657=ORIENTED_EDGE('',*,*,#3408,.T.);
#4658=ORIENTED_EDGE('',*,*,#3243,.F.);
#4659=ORIENTED_EDGE('',*,*,#3407,.T.);
#4660=ORIENTED_EDGE('',*,*,#3141,.F.);
#4661=ORIENTED_EDGE('',*,*,#3320,.F.);
#4662=ORIENTED_EDGE('',*,*,#3409,.F.);
#4663=ORIENTED_EDGE('',*,*,#3409,.T.);
#4664=ORIENTED_EDGE('',*,*,#3319,.F.);
#4665=ORIENTED_EDGE('',*,*,#3410,.F.);
#4666=ORIENTED_EDGE('',*,*,#3236,.F.);
#4667=ORIENTED_EDGE('',*,*,#3410,.T.);
#4668=ORIENTED_EDGE('',*,*,#3209,.F.);
#4669=ORIENTED_EDGE('',*,*,#3411,.F.);
#4670=ORIENTED_EDGE('',*,*,#3237,.F.);
#4671=ORIENTED_EDGE('',*,*,#3411,.T.);
#4672=ORIENTED_EDGE('',*,*,#3375,.F.);
#4673=ORIENTED_EDGE('',*,*,#3412,.F.);
#4674=ORIENTED_EDGE('',*,*,#3238,.F.);
#4675=ORIENTED_EDGE('',*,*,#3412,.T.);
#4676=ORIENTED_EDGE('',*,*,#3234,.F.);
#4677=ORIENTED_EDGE('',*,*,#3413,.F.);
#4678=ORIENTED_EDGE('',*,*,#3239,.F.);
#4679=ORIENTED_EDGE('',*,*,#3413,.T.);
#4680=ORIENTED_EDGE('',*,*,#3382,.F.);
#4681=ORIENTED_EDGE('',*,*,#3414,.F.);
#4682=ORIENTED_EDGE('',*,*,#3240,.F.);
#4683=ORIENTED_EDGE('',*,*,#3414,.T.);
#4684=ORIENTED_EDGE('',*,*,#3215,.F.);
#4685=ORIENTED_EDGE('',*,*,#3415,.F.);
#4686=ORIENTED_EDGE('',*,*,#3241,.F.);
#4687=ORIENTED_EDGE('',*,*,#3415,.T.);
#4688=ORIENTED_EDGE('',*,*,#3305,.F.);
#4689=ORIENTED_EDGE('',*,*,#3416,.F.);
#4690=ORIENTED_EDGE('',*,*,#3242,.F.);
#4691=ORIENTED_EDGE('',*,*,#3304,.F.);
#4692=ORIENTED_EDGE('',*,*,#3139,.F.);
#4693=ORIENTED_EDGE('',*,*,#3416,.T.);
#4694=ORIENTED_EDGE('',*,*,#3310,.F.);
#4695=ORIENTED_EDGE('',*,*,#3323,.F.);
#4696=ORIENTED_EDGE('',*,*,#3417,.F.);
#4697=ORIENTED_EDGE('',*,*,#3417,.T.);
#4698=ORIENTED_EDGE('',*,*,#3297,.F.);
#4699=ORIENTED_EDGE('',*,*,#3418,.F.);
#4700=ORIENTED_EDGE('',*,*,#3311,.F.);
#4701=ORIENTED_EDGE('',*,*,#3418,.T.);
#4702=ORIENTED_EDGE('',*,*,#3296,.F.);
#4703=ORIENTED_EDGE('',*,*,#3419,.F.);
#4704=ORIENTED_EDGE('',*,*,#3299,.F.);
#4705=ORIENTED_EDGE('',*,*,#3419,.T.);
#4706=ORIENTED_EDGE('',*,*,#3295,.F.);
#4707=ORIENTED_EDGE('',*,*,#3420,.F.);
#4708=ORIENTED_EDGE('',*,*,#3389,.F.);
#4709=ORIENTED_EDGE('',*,*,#3420,.T.);
#4710=ORIENTED_EDGE('',*,*,#3294,.F.);
#4711=ORIENTED_EDGE('',*,*,#3421,.F.);
#4712=ORIENTED_EDGE('',*,*,#3289,.F.);
#4713=ORIENTED_EDGE('',*,*,#3421,.T.);
#4714=ORIENTED_EDGE('',*,*,#3293,.F.);
#4715=ORIENTED_EDGE('',*,*,#3422,.F.);
#4716=ORIENTED_EDGE('',*,*,#3117,.F.);
#4717=ORIENTED_EDGE('',*,*,#3422,.T.);
#4718=ORIENTED_EDGE('',*,*,#3292,.F.);
#4719=ORIENTED_EDGE('',*,*,#3423,.F.);
#4720=ORIENTED_EDGE('',*,*,#3273,.F.);
#4721=ORIENTED_EDGE('',*,*,#3423,.T.);
#4722=ORIENTED_EDGE('',*,*,#3291,.F.);
#4723=ORIENTED_EDGE('',*,*,#3424,.F.);
#4724=ORIENTED_EDGE('',*,*,#3307,.F.);
#4725=ORIENTED_EDGE('',*,*,#3424,.T.);
#4726=ORIENTED_EDGE('',*,*,#3322,.F.);
#4727=ORIENTED_EDGE('',*,*,#3308,.F.);
#4728=ORIENTED_EDGE('',*,*,#3316,.F.);
#4729=ORIENTED_EDGE('',*,*,#3134,.F.);
#4730=ORIENTED_EDGE('',*,*,#3425,.F.);
#4731=ORIENTED_EDGE('',*,*,#3425,.T.);
#4732=ORIENTED_EDGE('',*,*,#3268,.F.);
#4733=ORIENTED_EDGE('',*,*,#3426,.F.);
#4734=ORIENTED_EDGE('',*,*,#3317,.F.);
#4735=ORIENTED_EDGE('',*,*,#3426,.T.);
#4736=ORIENTED_EDGE('',*,*,#3267,.F.);
#4737=ORIENTED_EDGE('',*,*,#3106,.F.);
#4738=ORIENTED_EDGE('',*,*,#3270,.F.);
#4739=ORIENTED_EDGE('',*,*,#3104,.T.);
#4740=ORIENTED_EDGE('',*,*,#3266,.F.);
#4741=ORIENTED_EDGE('',*,*,#3427,.F.);
#4742=ORIENTED_EDGE('',*,*,#3261,.F.);
#4743=ORIENTED_EDGE('',*,*,#3427,.T.);
#4744=ORIENTED_EDGE('',*,*,#3265,.F.);
#4745=ORIENTED_EDGE('',*,*,#3428,.F.);
#4746=ORIENTED_EDGE('',*,*,#3408,.F.);
#4747=ORIENTED_EDGE('',*,*,#3428,.T.);
#4748=ORIENTED_EDGE('',*,*,#3264,.F.);
#4749=ORIENTED_EDGE('',*,*,#3429,.F.);
#4750=ORIENTED_EDGE('',*,*,#3244,.F.);
#4751=ORIENTED_EDGE('',*,*,#3429,.T.);
#4752=ORIENTED_EDGE('',*,*,#3263,.F.);
#4753=ORIENTED_EDGE('',*,*,#3430,.F.);
#4754=ORIENTED_EDGE('',*,*,#3313,.F.);
#4755=ORIENTED_EDGE('',*,*,#3430,.T.);
#4756=ORIENTED_EDGE('',*,*,#3137,.F.);
#4757=ORIENTED_EDGE('',*,*,#3314,.F.);
#5784=CYLINDRICAL_SURFACE('',#6397,8.326);
#5785=CYLINDRICAL_SURFACE('',#6400,8.326);
#5786=CYLINDRICAL_SURFACE('',#6401,8.326);
#5787=CYLINDRICAL_SURFACE('',#6402,8.326);
#5788=CYLINDRICAL_SURFACE('',#6403,8.326);
#5789=CYLINDRICAL_SURFACE('',#6404,8.326);
#5790=CYLINDRICAL_SURFACE('',#6405,8.326);
#5791=CYLINDRICAL_SURFACE('',#6406,8.326);
#5792=CYLINDRICAL_SURFACE('',#6407,8.326);
#5793=CYLINDRICAL_SURFACE('',#6408,8.326);
#5794=CYLINDRICAL_SURFACE('',#6409,8.326);
#5795=CYLINDRICAL_SURFACE('',#6410,8.326);
#5796=CYLINDRICAL_SURFACE('',#6411,8.326);
#5797=CYLINDRICAL_SURFACE('',#6412,8.326);
#5798=CYLINDRICAL_SURFACE('',#6413,8.326);
#5799=CYLINDRICAL_SURFACE('',#6414,8.326);
#5800=CYLINDRICAL_SURFACE('',#6415,8.326);
#5801=CYLINDRICAL_SURFACE('',#6416,8.326);
#5802=CYLINDRICAL_SURFACE('',#6417,8.326);
#5803=CYLINDRICAL_SURFACE('',#6418,8.326);
#5804=CYLINDRICAL_SURFACE('',#6419,8.326);
#5805=CYLINDRICAL_SURFACE('',#6420,8.326);
#5806=CYLINDRICAL_SURFACE('',#6437,5.);
#5807=CYLINDRICAL_SURFACE('',#6440,5.);
#5808=CYLINDRICAL_SURFACE('',#6442,5.);
#5809=CYLINDRICAL_SURFACE('',#6445,5.);
#5810=CYLINDRICAL_SURFACE('',#6460,8.326);
#5811=CYLINDRICAL_SURFACE('',#6461,3.2);
#5812=CYLINDRICAL_SURFACE('',#6464,3.2);
#5813=CYLINDRICAL_SURFACE('',#6467,3.2);
#5814=CYLINDRICAL_SURFACE('',#6470,19.05);
#5815=CYLINDRICAL_SURFACE('',#6497,3.);
#5816=CYLINDRICAL_SURFACE('',#6501,5.);
#5817=CYLINDRICAL_SURFACE('',#6514,3.);
#5818=CYLINDRICAL_SURFACE('',#6518,5.);
#5819=CYLINDRICAL_SURFACE('',#6531,3.00000000000001);
#5820=CYLINDRICAL_SURFACE('',#6535,5.00000000000001);
#5821=CYLINDRICAL_SURFACE('',#6547,6.35);
#5822=CYLINDRICAL_SURFACE('',#6549,6.35);
#5823=CYLINDRICAL_SURFACE('',#6551,6.35);
#5824=CYLINDRICAL_SURFACE('',#6553,6.35);
#5825=CYLINDRICAL_SURFACE('',#6555,6.35);
#5826=CYLINDRICAL_SURFACE('',#6557,6.35);
#5827=CYLINDRICAL_SURFACE('',#6576,2.);
#5828=CYLINDRICAL_SURFACE('',#6578,2.);
#5829=CYLINDRICAL_SURFACE('',#6580,2.);
#5830=CYLINDRICAL_SURFACE('',#6582,2.);
#5831=CYLINDRICAL_SURFACE('',#6584,2.);
#5832=CYLINDRICAL_SURFACE('',#6586,2.);
#5833=CYLINDRICAL_SURFACE('',#6591,1.);
#5834=CYLINDRICAL_SURFACE('',#6593,1.);
#5835=CYLINDRICAL_SURFACE('',#6599,1.);
#5836=CYLINDRICAL_SURFACE('',#6601,1.);
#5837=CYLINDRICAL_SURFACE('',#6607,1.);
#5838=CYLINDRICAL_SURFACE('',#6609,1.);
#5839=CYLINDRICAL_SURFACE('',#6612,5.);
#5840=CYLINDRICAL_SURFACE('',#6617,5.);
#5841=CYLINDRICAL_SURFACE('',#6618,5.);
#5842=CYLINDRICAL_SURFACE('',#6621,5.);
#5843=CYLINDRICAL_SURFACE('',#6626,5.);
#5844=CYLINDRICAL_SURFACE('',#6627,5.);
#5845=CYLINDRICAL_SURFACE('',#6630,5.);
#5846=CYLINDRICAL_SURFACE('',#6635,5.);
#5847=CYLINDRICAL_SURFACE('',#6636,5.);
#5848=CYLINDRICAL_SURFACE('',#6641,5.);
#5849=CYLINDRICAL_SURFACE('',#6644,5.);
#5850=CYLINDRICAL_SURFACE('',#6649,5.);
#5851=CYLINDRICAL_SURFACE('',#6650,5.);
#5852=CYLINDRICAL_SURFACE('',#6654,5.);
#5853=CYLINDRICAL_SURFACE('',#6659,1.);
#5854=CYLINDRICAL_SURFACE('',#6663,1.);
#5855=CYLINDRICAL_SURFACE('',#6667,1.);
#5856=CYLINDRICAL_SURFACE('',#6674,1.);
#5857=CYLINDRICAL_SURFACE('',#6678,1.);
#5858=CYLINDRICAL_SURFACE('',#6682,1.);
#5859=CYLINDRICAL_SURFACE('',#6689,1.);
#5860=CYLINDRICAL_SURFACE('',#6690,1.);
#5861=CYLINDRICAL_SURFACE('',#6694,1.);
#5915=ADVANCED_FACE('',(#500),#5784,.F.);
#5916=ADVANCED_FACE('',(#501),#5785,.F.);
#5917=ADVANCED_FACE('',(#502),#5786,.F.);
#5918=ADVANCED_FACE('',(#503),#5787,.F.);
#5919=ADVANCED_FACE('',(#504),#5788,.F.);
#5920=ADVANCED_FACE('',(#505),#5789,.F.);
#5921=ADVANCED_FACE('',(#506),#5790,.F.);
#5922=ADVANCED_FACE('',(#507),#5791,.F.);
#5923=ADVANCED_FACE('',(#508),#5792,.F.);
#5924=ADVANCED_FACE('',(#509),#5793,.F.);
#5925=ADVANCED_FACE('',(#510),#5794,.F.);
#5926=ADVANCED_FACE('',(#511),#5795,.F.);
#5927=ADVANCED_FACE('',(#512),#5796,.F.);
#5928=ADVANCED_FACE('',(#513),#5797,.F.);
#5929=ADVANCED_FACE('',(#514),#5798,.F.);
#5930=ADVANCED_FACE('',(#515),#5799,.F.);
#5931=ADVANCED_FACE('',(#516),#5800,.F.);
#5932=ADVANCED_FACE('',(#517),#5801,.F.);
#5933=ADVANCED_FACE('',(#518),#5802,.F.);
#5934=ADVANCED_FACE('',(#519),#5803,.F.);
#5935=ADVANCED_FACE('',(#520),#5804,.F.);
#5936=ADVANCED_FACE('',(#521),#5805,.F.);
#5937=ADVANCED_FACE('',(#522),#463,.T.);
#5938=ADVANCED_FACE('',(#523),#464,.T.);
#5939=ADVANCED_FACE('',(#524),#465,.T.);
#5940=ADVANCED_FACE('',(#525),#5806,.T.);
#5941=ADVANCED_FACE('',(#526),#5807,.T.);
#5942=ADVANCED_FACE('',(#527),#5808,.T.);
#5943=ADVANCED_FACE('',(#528),#5809,.T.);
#5944=ADVANCED_FACE('',(#529),#369,.F.);
#5945=ADVANCED_FACE('',(#530),#466,.F.);
#5946=ADVANCED_FACE('',(#531),#467,.F.);
#5947=ADVANCED_FACE('',(#532),#468,.F.);
#5948=ADVANCED_FACE('',(#533),#5810,.F.);
#5949=ADVANCED_FACE('',(#534),#5811,.F.);
#5950=ADVANCED_FACE('',(#535),#5812,.F.);
#5951=ADVANCED_FACE('',(#536),#5813,.F.);
#5952=ADVANCED_FACE('',(#537,#335,#336),#5814,.T.);
#5953=ADVANCED_FACE('',(#538,#337),#249,.T.);
#5954=ADVANCED_FACE('',(#539),#250,.T.);
#5955=ADVANCED_FACE('',(#540),#251,.T.);
#5956=ADVANCED_FACE('',(#541),#252,.T.);
#5957=ADVANCED_FACE('',(#542),#253,.T.);
#5958=ADVANCED_FACE('',(#543),#254,.T.);
#5959=ADVANCED_FACE('',(#544),#255,.T.);
#5960=ADVANCED_FACE('',(#545,#338),#256,.F.);
#5961=ADVANCED_FACE('',(#546),#370,.F.);
#5962=ADVANCED_FACE('',(#547,#339),#257,.F.);
#5963=ADVANCED_FACE('',(#548,#340),#258,.T.);
#5964=ADVANCED_FACE('',(#549),#259,.F.);
#5965=ADVANCED_FACE('',(#550),#5815,.T.);
#5966=ADVANCED_FACE('',(#551),#260,.F.);
#5967=ADVANCED_FACE('',(#552),#5816,.T.);
#5968=ADVANCED_FACE('',(#553),#261,.F.);
#5969=ADVANCED_FACE('',(#554),#262,.F.);
#5970=ADVANCED_FACE('',(#555,#341),#263,.F.);
#5971=ADVANCED_FACE('',(#556),#264,.F.);
#5972=ADVANCED_FACE('',(#557),#5817,.T.);
#5973=ADVANCED_FACE('',(#558),#265,.F.);
#5974=ADVANCED_FACE('',(#559),#5818,.T.);
#5975=ADVANCED_FACE('',(#560),#266,.F.);
#5976=ADVANCED_FACE('',(#561),#267,.F.);
#5977=ADVANCED_FACE('',(#562,#342),#268,.T.);
#5978=ADVANCED_FACE('',(#563,#343),#269,.F.);
#5979=ADVANCED_FACE('',(#564),#270,.F.);
#5980=ADVANCED_FACE('',(#565),#5819,.T.);
#5981=ADVANCED_FACE('',(#566),#271,.F.);
#5982=ADVANCED_FACE('',(#567),#5820,.T.);
#5983=ADVANCED_FACE('',(#568),#272,.F.);
#5984=ADVANCED_FACE('',(#569),#273,.F.);
#5985=ADVANCED_FACE('',(#570,#344),#274,.T.);
#5986=ADVANCED_FACE('',(#571),#5821,.F.);
#5987=ADVANCED_FACE('',(#572),#5822,.F.);
#5988=ADVANCED_FACE('',(#573),#5823,.F.);
#5989=ADVANCED_FACE('',(#574),#5824,.F.);
#5990=ADVANCED_FACE('',(#575),#5825,.F.);
#5991=ADVANCED_FACE('',(#576),#5826,.F.);
#5992=ADVANCED_FACE('',(#577),#469,.F.);
#5993=ADVANCED_FACE('',(#578),#470,.F.);
#5994=ADVANCED_FACE('',(#579),#471,.F.);
#5995=ADVANCED_FACE('',(#580),#275,.T.);
#5996=ADVANCED_FACE('',(#581),#148,.T.);
#5997=ADVANCED_FACE('',(#582),#149,.T.);
#5998=ADVANCED_FACE('',(#583),#150,.T.);
#5999=ADVANCED_FACE('',(#584),#151,.T.);
#6000=ADVANCED_FACE('',(#585,#345),#276,.T.);
#6001=ADVANCED_FACE('',(#586),#371,.T.);
#6002=ADVANCED_FACE('',(#587),#372,.T.);
#6003=ADVANCED_FACE('',(#588),#373,.T.);
#6004=ADVANCED_FACE('',(#589),#374,.T.);
#6005=ADVANCED_FACE('',(#590),#375,.T.);
#6006=ADVANCED_FACE('',(#591),#376,.T.);
#6007=ADVANCED_FACE('',(#592),#5827,.T.);
#6008=ADVANCED_FACE('',(#593),#5828,.T.);
#6009=ADVANCED_FACE('',(#594),#5829,.T.);
#6010=ADVANCED_FACE('',(#595),#5830,.T.);
#6011=ADVANCED_FACE('',(#596),#5831,.T.);
#6012=ADVANCED_FACE('',(#597),#5832,.T.);
#6013=ADVANCED_FACE('',(#598),#472,.F.);
#6014=ADVANCED_FACE('',(#599),#5833,.F.);
#6015=ADVANCED_FACE('',(#600),#5834,.F.);
#6016=ADVANCED_FACE('',(#601),#473,.F.);
#6017=ADVANCED_FACE('',(#602),#474,.F.);
#6018=ADVANCED_FACE('',(#603),#5835,.F.);
#6019=ADVANCED_FACE('',(#604),#5836,.F.);
#6020=ADVANCED_FACE('',(#605),#475,.F.);
#6021=ADVANCED_FACE('',(#606),#476,.F.);
#6022=ADVANCED_FACE('',(#607),#5837,.F.);
#6023=ADVANCED_FACE('',(#608),#5838,.F.);
#6024=ADVANCED_FACE('',(#609),#477,.F.);
#6025=ADVANCED_FACE('',(#610),#5839,.T.);
#6026=ADVANCED_FACE('',(#611),#139,.T.);
#6027=ADVANCED_FACE('',(#612),#5840,.T.);
#6028=ADVANCED_FACE('',(#613),#152,.T.);
#6029=ADVANCED_FACE('',(#614),#5841,.T.);
#6030=ADVANCED_FACE('',(#615),#153,.T.);
#6031=ADVANCED_FACE('',(#616),#154,.T.);
#6032=ADVANCED_FACE('',(#617),#5842,.T.);
#6033=ADVANCED_FACE('',(#618),#140,.T.);
#6034=ADVANCED_FACE('',(#619),#5843,.T.);
#6035=ADVANCED_FACE('',(#620),#155,.T.);
#6036=ADVANCED_FACE('',(#621),#5844,.T.);
#6037=ADVANCED_FACE('',(#622),#156,.T.);
#6038=ADVANCED_FACE('',(#623),#157,.T.);
#6039=ADVANCED_FACE('',(#624),#5845,.T.);
#6040=ADVANCED_FACE('',(#625),#141,.T.);
#6041=ADVANCED_FACE('',(#626),#5846,.T.);
#6042=ADVANCED_FACE('',(#627),#158,.T.);
#6043=ADVANCED_FACE('',(#628),#5847,.T.);
#6044=ADVANCED_FACE('',(#629),#159,.T.);
#6045=ADVANCED_FACE('',(#630),#160,.T.);
#6046=ADVANCED_FACE('',(#631),#161,.T.);
#6047=ADVANCED_FACE('',(#632),#162,.T.);
#6048=ADVANCED_FACE('',(#633),#5848,.T.);
#6049=ADVANCED_FACE('',(#634),#163,.T.);
#6050=ADVANCED_FACE('',(#635),#142,.T.);
#6051=ADVANCED_FACE('',(#636),#143,.T.);
#6052=ADVANCED_FACE('',(#637),#164,.T.);
#6053=ADVANCED_FACE('',(#638),#5849,.T.);
#6054=ADVANCED_FACE('',(#639),#165,.T.);
#6055=ADVANCED_FACE('',(#640),#166,.T.);
#6056=ADVANCED_FACE('',(#641),#167,.T.);
#6057=ADVANCED_FACE('',(#642),#168,.T.);
#6058=ADVANCED_FACE('',(#643),#5850,.T.);
#6059=ADVANCED_FACE('',(#644),#169,.T.);
#6060=ADVANCED_FACE('',(#645),#5851,.T.);
#6061=ADVANCED_FACE('',(#646),#144,.T.);
#6062=ADVANCED_FACE('',(#647),#5852,.T.);
#6063=ADVANCED_FACE('',(#648),#170,.T.);
#6064=ADVANCED_FACE('',(#649),#478,.T.);
#6065=ADVANCED_FACE('',(#650),#5853,.T.);
#6066=ADVANCED_FACE('',(#651),#479,.T.);
#6067=ADVANCED_FACE('',(#652),#5854,.T.);
#6068=ADVANCED_FACE('',(#653),#480,.T.);
#6069=ADVANCED_FACE('',(#654),#5855,.T.);
#6070=ADVANCED_FACE('',(#655),#481,.T.);
#6071=ADVANCED_FACE('',(#656),#171,.T.);
#6072=ADVANCED_FACE('',(#657),#172,.T.);
#6073=ADVANCED_FACE('',(#658),#482,.T.);
#6074=ADVANCED_FACE('',(#659),#5856,.T.);
#6075=ADVANCED_FACE('',(#660),#483,.T.);
#6076=ADVANCED_FACE('',(#661),#5857,.T.);
#6077=ADVANCED_FACE('',(#662),#484,.T.);
#6078=ADVANCED_FACE('',(#663),#5858,.T.);
#6079=ADVANCED_FACE('',(#664),#485,.T.);
#6080=ADVANCED_FACE('',(#665),#173,.T.);
#6081=ADVANCED_FACE('',(#666),#174,.T.);
#6082=ADVANCED_FACE('',(#667),#486,.T.);
#6083=ADVANCED_FACE('',(#668),#5859,.T.);
#6084=ADVANCED_FACE('',(#669),#5860,.T.);
#6085=ADVANCED_FACE('',(#670),#487,.T.);
#6086=ADVANCED_FACE('',(#671),#5861,.T.);
#6087=ADVANCED_FACE('',(#672),#488,.T.);
#6088=ADVANCED_FACE('',(#673),#175,.T.);
#6298=CLOSED_SHELL('',(#5915,#5916,#5917,#5918,#5919,#5920,#5921,#5922,
#5923,#5924,#5925,#5926,#5927,#5928,#5929,#5930,#5931,#5932,#5933,#5934,
#5935,#5936,#5937,#5938,#5939,#5940,#5941,#5942,#5943,#5944,#5945,#5946,
#5947,#5948,#5949,#5950,#5951,#5952,#5953,#5954,#5955,#5956,#5957,#5958,
#5959,#5960,#5961,#5962,#5963,#5964,#5965,#5966,#5967,#5968,#5969,#5970,
#5971,#5972,#5973,#5974,#5975,#5976,#5977,#5978,#5979,#5980,#5981,#5982,
#5983,#5984,#5985,#5986,#5987,#5988,#5989,#5990,#5991,#5992,#5993,#5994,
#5995,#5996,#5997,#5998,#5999,#6000,#6001,#6002,#6003,#6004,#6005,#6006,
#6007,#6008,#6009,#6010,#6011,#6012,#6013,#6014,#6015,#6016,#6017,#6018,
#6019,#6020,#6021,#6022,#6023,#6024,#6025,#6026,#6027,#6028,#6029,#6030,
#6031,#6032,#6033,#6034,#6035,#6036,#6037,#6038,#6039,#6040,#6041,#6042,
#6043,#6044,#6045,#6046,#6047,#6048,#6049,#6050,#6051,#6052,#6053,#6054,
#6055,#6056,#6057,#6058,#6059,#6060,#6061,#6062,#6063,#6064,#6065,#6066,
#6067,#6068,#6069,#6070,#6071,#6072,#6073,#6074,#6075,#6076,#6077,#6078,
#6079,#6080,#6081,#6082,#6083,#6084,#6085,#6086,#6087,#6088));
#6396=AXIS2_PLACEMENT_3D('',#9084,#7187,#7188);
#6397=AXIS2_PLACEMENT_3D('',#9085,#7189,#7190);
#6398=AXIS2_PLACEMENT_3D('',#9127,#7192,#7193);
#6399=AXIS2_PLACEMENT_3D('',#9139,#7195,#7196);
#6400=AXIS2_PLACEMENT_3D('',#9176,#7197,#7198);
#6401=AXIS2_PLACEMENT_3D('',#9254,#7200,#7201);
#6402=AXIS2_PLACEMENT_3D('',#9330,#7203,#7204);
#6403=AXIS2_PLACEMENT_3D('',#9408,#7206,#7207);
#6404=AXIS2_PLACEMENT_3D('',#9484,#7209,#7210);
#6405=AXIS2_PLACEMENT_3D('',#9560,#7212,#7213);
#6406=AXIS2_PLACEMENT_3D('',#9636,#7215,#7216);
#6407=AXIS2_PLACEMENT_3D('',#9714,#7218,#7219);
#6408=AXIS2_PLACEMENT_3D('',#9790,#7221,#7222);
#6409=AXIS2_PLACEMENT_3D('',#9868,#7224,#7225);
#6410=AXIS2_PLACEMENT_3D('',#9944,#7227,#7228);
#6411=AXIS2_PLACEMENT_3D('',#10020,#7230,#7231);
#6412=AXIS2_PLACEMENT_3D('',#10096,#7233,#7234);
#6413=AXIS2_PLACEMENT_3D('',#10174,#7236,#7237);
#6414=AXIS2_PLACEMENT_3D('',#10250,#7239,#7240);
#6415=AXIS2_PLACEMENT_3D('',#10328,#7242,#7243);
#6416=AXIS2_PLACEMENT_3D('',#10404,#7245,#7246);
#6417=AXIS2_PLACEMENT_3D('',#10480,#7248,#7249);
#6418=AXIS2_PLACEMENT_3D('',#10556,#7251,#7252);
#6419=AXIS2_PLACEMENT_3D('',#10634,#7254,#7255);
#6420=AXIS2_PLACEMENT_3D('',#10710,#7257,#7258);
#6421=AXIS2_PLACEMENT_3D('',#10728,#7260,#7261);
#6422=AXIS2_PLACEMENT_3D('',#10747,#7262,#7263);
#6423=AXIS2_PLACEMENT_3D('',#10750,#7264,#7265);
#6424=AXIS2_PLACEMENT_3D('',#10751,#7266,#7267);
#6425=AXIS2_PLACEMENT_3D('',#10753,#7268,#7269);
#6426=AXIS2_PLACEMENT_3D('',#10754,#7270,#7271);
#6427=AXIS2_PLACEMENT_3D('',#10755,#7272,#7273);
#6428=AXIS2_PLACEMENT_3D('',#10757,#7274,#7275);
#6429=AXIS2_PLACEMENT_3D('',#10759,#7276,#7277);
#6430=AXIS2_PLACEMENT_3D('',#10761,#7278,#7279);
#6431=AXIS2_PLACEMENT_3D('',#10762,#7280,#7281);
#6432=AXIS2_PLACEMENT_3D('',#10763,#7282,#7283);
#6433=AXIS2_PLACEMENT_3D('',#10766,#7284,#7285);
#6434=AXIS2_PLACEMENT_3D('',#10768,#7286,#7287);
#6435=AXIS2_PLACEMENT_3D('',#10770,#7288,#7289);
#6436=AXIS2_PLACEMENT_3D('',#10771,#7290,#7291);
#6437=AXIS2_PLACEMENT_3D('',#10772,#7292,#7293);
#6438=AXIS2_PLACEMENT_3D('',#10775,#7294,#7295);
#6439=AXIS2_PLACEMENT_3D('',#10779,#7297,#7298);
#6440=AXIS2_PLACEMENT_3D('',#10837,#7300,#7301);
#6441=AXIS2_PLACEMENT_3D('',#10840,#7303,#7304);
#6442=AXIS2_PLACEMENT_3D('',#10842,#7306,#7307);
#6443=AXIS2_PLACEMENT_3D('',#10845,#7308,#7309);
#6444=AXIS2_PLACEMENT_3D('',#10849,#7311,#7312);
#6445=AXIS2_PLACEMENT_3D('',#10851,#7314,#7315);
#6446=AXIS2_PLACEMENT_3D('',#10910,#7316,#7317);
#6447=AXIS2_PLACEMENT_3D('',#10913,#7319,#7320);
#6448=AXIS2_PLACEMENT_3D('',#10915,#7322,#7323);
#6449=AXIS2_PLACEMENT_3D('',#10918,#7325,#7326);
#6450=AXIS2_PLACEMENT_3D('',#10919,#7327,#7328);
#6451=AXIS2_PLACEMENT_3D('',#11022,#7329,#7330);
#6452=AXIS2_PLACEMENT_3D('',#11124,#7331,#7332);
#6453=AXIS2_PLACEMENT_3D('',#11132,#7333,#7334);
#6454=AXIS2_PLACEMENT_3D('',#11135,#7335,#7336);
#6455=AXIS2_PLACEMENT_3D('',#11178,#7337,#7338);
#6456=AXIS2_PLACEMENT_3D('',#11180,#7339,#7340);
#6457=AXIS2_PLACEMENT_3D('',#11224,#7341,#7342);
#6458=AXIS2_PLACEMENT_3D('',#11227,#7343,#7344);
#6459=AXIS2_PLACEMENT_3D('',#11270,#7345,#7346);
#6460=AXIS2_PLACEMENT_3D('',#11314,#7347,#7348);
#6461=AXIS2_PLACEMENT_3D('',#11389,#7349,#7350);
#6462=AXIS2_PLACEMENT_3D('',#11391,#7351,#7352);
#6463=AXIS2_PLACEMENT_3D('',#11394,#7354,#7355);
#6464=AXIS2_PLACEMENT_3D('',#11395,#7356,#7357);
#6465=AXIS2_PLACEMENT_3D('',#11397,#7358,#7359);
#6466=AXIS2_PLACEMENT_3D('',#11400,#7361,#7362);
#6467=AXIS2_PLACEMENT_3D('',#11401,#7363,#7364);
#6468=AXIS2_PLACEMENT_3D('',#11403,#7365,#7366);
#6469=AXIS2_PLACEMENT_3D('',#11406,#7368,#7369);
#6470=AXIS2_PLACEMENT_3D('',#11407,#7370,#7371);
#6471=AXIS2_PLACEMENT_3D('',#11412,#7374,#7375);
#6472=AXIS2_PLACEMENT_3D('',#11415,#7377,#7378);
#6473=AXIS2_PLACEMENT_3D('',#11420,#7381,#7382);
#6474=AXIS2_PLACEMENT_3D('',#11426,#7386,#7387);
#6475=AXIS2_PLACEMENT_3D('',#11427,#7388,#7389);
#6476=AXIS2_PLACEMENT_3D('',#11430,#7390,#7391);
#6477=AXIS2_PLACEMENT_3D('',#11432,#7392,#7393);
#6478=AXIS2_PLACEMENT_3D('',#11434,#7394,#7395);
#6479=AXIS2_PLACEMENT_3D('',#11436,#7396,#7397);
#6480=AXIS2_PLACEMENT_3D('',#11438,#7398,#7399);
#6481=AXIS2_PLACEMENT_3D('',#11439,#7400,#7401);
#6482=AXIS2_PLACEMENT_3D('',#11440,#7402,#7403);
#6483=AXIS2_PLACEMENT_3D('',#11454,#7407,#7408);
#6484=AXIS2_PLACEMENT_3D('',#11468,#7412,#7413);
#6485=AXIS2_PLACEMENT_3D('',#11482,#7417,#7418);
#6486=AXIS2_PLACEMENT_3D('',#11496,#7422,#7423);
#6487=AXIS2_PLACEMENT_3D('',#11510,#7427,#7428);
#6488=AXIS2_PLACEMENT_3D('',#11524,#7432,#7433);
#6489=AXIS2_PLACEMENT_3D('',#11556,#7434,#7435);
#6490=AXIS2_PLACEMENT_3D('',#11557,#7436,#7437);
#6491=AXIS2_PLACEMENT_3D('',#11606,#7438,#7439);
#6492=AXIS2_PLACEMENT_3D('',#11615,#7443,#7444);
#6493=AXIS2_PLACEMENT_3D('',#11619,#7447,#7448);
#6494=AXIS2_PLACEMENT_3D('',#11631,#7454,#7455);
#6495=AXIS2_PLACEMENT_3D('',#11632,#7456,#7457);
#6496=AXIS2_PLACEMENT_3D('',#11639,#7460,#7461);
#6497=AXIS2_PLACEMENT_3D('',#11641,#7463,#7464);
#6498=AXIS2_PLACEMENT_3D('',#11645,#7466,#7467);
#6499=AXIS2_PLACEMENT_3D('',#11646,#7468,#7469);
#6500=AXIS2_PLACEMENT_3D('',#11647,#7470,#7471);
#6501=AXIS2_PLACEMENT_3D('',#11653,#7475,#7476);
#6502=AXIS2_PLACEMENT_3D('',#11657,#7478,#7479);
#6503=AXIS2_PLACEMENT_3D('',#11658,#7480,#7481);
#6504=AXIS2_PLACEMENT_3D('',#11659,#7482,#7483);
#6505=AXIS2_PLACEMENT_3D('',#11665,#7487,#7488);
#6506=AXIS2_PLACEMENT_3D('',#11667,#7489,#7490);
#6507=AXIS2_PLACEMENT_3D('',#11671,#7492,#7493);
#6508=AXIS2_PLACEMENT_3D('',#11675,#7495,#7496);
#6509=AXIS2_PLACEMENT_3D('',#11678,#7498,#7499);
#6510=AXIS2_PLACEMENT_3D('',#11679,#7500,#7501);
#6511=AXIS2_PLACEMENT_3D('',#11688,#7505,#7506);
#6512=AXIS2_PLACEMENT_3D('',#11692,#7509,#7510);
#6513=AXIS2_PLACEMENT_3D('',#11699,#7513,#7514);
#6514=AXIS2_PLACEMENT_3D('',#11701,#7516,#7517);
#6515=AXIS2_PLACEMENT_3D('',#11702,#7518,#7519);
#6516=AXIS2_PLACEMENT_3D('',#11705,#7521,#7522);
#6517=AXIS2_PLACEMENT_3D('',#11706,#7523,#7524);
#6518=AXIS2_PLACEMENT_3D('',#11710,#7527,#7528);
#6519=AXIS2_PLACEMENT_3D('',#11711,#7529,#7530);
#6520=AXIS2_PLACEMENT_3D('',#11714,#7532,#7533);
#6521=AXIS2_PLACEMENT_3D('',#11715,#7534,#7535);
#6522=AXIS2_PLACEMENT_3D('',#11719,#7538,#7539);
#6523=AXIS2_PLACEMENT_3D('',#11721,#7540,#7541);
#6524=AXIS2_PLACEMENT_3D('',#11725,#7543,#7544);
#6525=AXIS2_PLACEMENT_3D('',#11729,#7547,#7548);
#6526=AXIS2_PLACEMENT_3D('',#11730,#7549,#7550);
#6527=AXIS2_PLACEMENT_3D('',#11737,#7554,#7555);
#6528=AXIS2_PLACEMENT_3D('',#11738,#7556,#7557);
#6529=AXIS2_PLACEMENT_3D('',#11744,#7560,#7561);
#6530=AXIS2_PLACEMENT_3D('',#11746,#7563,#7564);
#6531=AXIS2_PLACEMENT_3D('',#11752,#7568,#7569);
#6532=AXIS2_PLACEMENT_3D('',#11754,#7570,#7571);
#6533=AXIS2_PLACEMENT_3D('',#11756,#7573,#7574);
#6534=AXIS2_PLACEMENT_3D('',#11757,#7575,#7576);
#6535=AXIS2_PLACEMENT_3D('',#11761,#7579,#7580);
#6536=AXIS2_PLACEMENT_3D('',#11763,#7581,#7582);
#6537=AXIS2_PLACEMENT_3D('',#11765,#7584,#7585);
#6538=AXIS2_PLACEMENT_3D('',#11766,#7586,#7587);
#6539=AXIS2_PLACEMENT_3D('',#11770,#7590,#7591);
#6540=AXIS2_PLACEMENT_3D('',#11773,#7592,#7593);
#6541=AXIS2_PLACEMENT_3D('',#11775,#7594,#7595);
#6542=AXIS2_PLACEMENT_3D('',#11779,#7597,#7598);
#6543=AXIS2_PLACEMENT_3D('',#11783,#7600,#7601);
#6544=AXIS2_PLACEMENT_3D('',#11786,#7603,#7604);
#6545=AXIS2_PLACEMENT_3D('',#11787,#7605,#7606);
#6546=AXIS2_PLACEMENT_3D('',#11799,#7612,#7613);
#6547=AXIS2_PLACEMENT_3D('',#11800,#7614,#7615);
#6548=AXIS2_PLACEMENT_3D('',#11842,#7616,#7617);
#6549=AXIS2_PLACEMENT_3D('',#11922,#7618,#7619);
#6550=AXIS2_PLACEMENT_3D('',#11924,#7620,#7621);
#6551=AXIS2_PLACEMENT_3D('',#12041,#7622,#7623);
#6552=AXIS2_PLACEMENT_3D('',#12083,#7624,#7625);
#6553=AXIS2_PLACEMENT_3D('',#12163,#7626,#7627);
#6554=AXIS2_PLACEMENT_3D('',#12165,#7628,#7629);
#6555=AXIS2_PLACEMENT_3D('',#12282,#7630,#7631);
#6556=AXIS2_PLACEMENT_3D('',#12324,#7632,#7633);
#6557=AXIS2_PLACEMENT_3D('',#12404,#7634,#7635);
#6558=AXIS2_PLACEMENT_3D('',#12406,#7636,#7637);
#6559=AXIS2_PLACEMENT_3D('',#12523,#7638,#7639);
#6560=AXIS2_PLACEMENT_3D('',#12607,#7640,#7641);
#6561=AXIS2_PLACEMENT_3D('',#12806,#7642,#7643);
#6562=AXIS2_PLACEMENT_3D('',#13005,#7644,#7645);
#6563=AXIS2_PLACEMENT_3D('',#25550,#7646,#7647);
#6564=AXIS2_PLACEMENT_3D('',#25555,#7649,#7650);
#6565=AXIS2_PLACEMENT_3D('',#25559,#7652,#7653);
#6566=AXIS2_PLACEMENT_3D('',#25563,#7655,#7656);
#6567=AXIS2_PLACEMENT_3D('',#25567,#7658,#7659);
#6568=AXIS2_PLACEMENT_3D('',#25571,#7661,#7662);
#6569=AXIS2_PLACEMENT_3D('',#25574,#7664,#7665);
#6570=AXIS2_PLACEMENT_3D('',#25575,#7666,#7667);
#6571=AXIS2_PLACEMENT_3D('',#25586,#7668,#7669);
#6572=AXIS2_PLACEMENT_3D('',#25597,#7670,#7671);
#6573=AXIS2_PLACEMENT_3D('',#25608,#7672,#7673);
#6574=AXIS2_PLACEMENT_3D('',#25619,#7674,#7675);
#6575=AXIS2_PLACEMENT_3D('',#25630,#7676,#7677);
#6576=AXIS2_PLACEMENT_3D('',#25641,#7678,#7679);
#6577=AXIS2_PLACEMENT_3D('',#25642,#7680,#7681);
#6578=AXIS2_PLACEMENT_3D('',#25643,#7682,#7683);
#6579=AXIS2_PLACEMENT_3D('',#25644,#7684,#7685);
#6580=AXIS2_PLACEMENT_3D('',#25645,#7686,#7687);
#6581=AXIS2_PLACEMENT_3D('',#25646,#7688,#7689);
#6582=AXIS2_PLACEMENT_3D('',#25647,#7690,#7691);
#6583=AXIS2_PLACEMENT_3D('',#25648,#7692,#7693);
#6584=AXIS2_PLACEMENT_3D('',#25649,#7694,#7695);
#6585=AXIS2_PLACEMENT_3D('',#25650,#7696,#7697);
#6586=AXIS2_PLACEMENT_3D('',#25651,#7698,#7699);
#6587=AXIS2_PLACEMENT_3D('',#25652,#7700,#7701);
#6588=AXIS2_PLACEMENT_3D('',#25653,#7702,#7703);
#6589=AXIS2_PLACEMENT_3D('',#25654,#7704,#7705);
#6590=AXIS2_PLACEMENT_3D('',#25655,#7706,#7707);
#6591=AXIS2_PLACEMENT_3D('',#25656,#7708,#7709);
#6592=AXIS2_PLACEMENT_3D('',#25657,#7710,#7711);
#6593=AXIS2_PLACEMENT_3D('',#25658,#7712,#7713);
#6594=AXIS2_PLACEMENT_3D('',#25659,#7714,#7715);
#6595=AXIS2_PLACEMENT_3D('',#25660,#7716,#7717);
#6596=AXIS2_PLACEMENT_3D('',#25661,#7718,#7719);
#6597=AXIS2_PLACEMENT_3D('',#25662,#7720,#7721);
#6598=AXIS2_PLACEMENT_3D('',#25663,#7722,#7723);
#6599=AXIS2_PLACEMENT_3D('',#25664,#7724,#7725);
#6600=AXIS2_PLACEMENT_3D('',#25665,#7726,#7727);
#6601=AXIS2_PLACEMENT_3D('',#25666,#7728,#7729);
#6602=AXIS2_PLACEMENT_3D('',#25667,#7730,#7731);
#6603=AXIS2_PLACEMENT_3D('',#25668,#7732,#7733);
#6604=AXIS2_PLACEMENT_3D('',#25669,#7734,#7735);
#6605=AXIS2_PLACEMENT_3D('',#25670,#7736,#7737);
#6606=AXIS2_PLACEMENT_3D('',#25671,#7738,#7739);
#6607=AXIS2_PLACEMENT_3D('',#25672,#7740,#7741);
#6608=AXIS2_PLACEMENT_3D('',#25673,#7742,#7743);
#6609=AXIS2_PLACEMENT_3D('',#25674,#7744,#7745);
#6610=AXIS2_PLACEMENT_3D('',#25675,#7746,#7747);
#6611=AXIS2_PLACEMENT_3D('',#25676,#7748,#7749);
#6612=AXIS2_PLACEMENT_3D('',#25677,#7750,#7751);
#6613=AXIS2_PLACEMENT_3D('',#25678,#7752,#7753);
#6614=AXIS2_PLACEMENT_3D('',#25679,#7754,#7755);
#6615=AXIS2_PLACEMENT_3D('',#25680,#7756,#7757);
#6616=AXIS2_PLACEMENT_3D('',#25681,#7758,#7759);
#6617=AXIS2_PLACEMENT_3D('',#25682,#7760,#7761);
#6618=AXIS2_PLACEMENT_3D('',#25859,#7762,#7763);
#6619=AXIS2_PLACEMENT_3D('',#25860,#7764,#7765);
#6620=AXIS2_PLACEMENT_3D('',#25873,#7766,#7767);
#6621=AXIS2_PLACEMENT_3D('',#25916,#7768,#7769);
#6622=AXIS2_PLACEMENT_3D('',#25917,#7770,#7771);
#6623=AXIS2_PLACEMENT_3D('',#25918,#7772,#7773);
#6624=AXIS2_PLACEMENT_3D('',#25919,#7774,#7775);
#6625=AXIS2_PLACEMENT_3D('',#25920,#7776,#7777);
#6626=AXIS2_PLACEMENT_3D('',#25921,#7778,#7779);
#6627=AXIS2_PLACEMENT_3D('',#26098,#7780,#7781);
#6628=AXIS2_PLACEMENT_3D('',#26099,#7782,#7783);
#6629=AXIS2_PLACEMENT_3D('',#26112,#7784,#7785);
#6630=AXIS2_PLACEMENT_3D('',#26161,#7786,#7787);
#6631=AXIS2_PLACEMENT_3D('',#26162,#7788,#7789);
#6632=AXIS2_PLACEMENT_3D('',#26163,#7790,#7791);
#6633=AXIS2_PLACEMENT_3D('',#26164,#7792,#7793);
#6634=AXIS2_PLACEMENT_3D('',#26165,#7794,#7795);
#6635=AXIS2_PLACEMENT_3D('',#26166,#7796,#7797);
#6636=AXIS2_PLACEMENT_3D('',#26343,#7798,#7799);
#6637=AXIS2_PLACEMENT_3D('',#26344,#7800,#7801);
#6638=AXIS2_PLACEMENT_3D('',#26357,#7802,#7803);
#6639=AXIS2_PLACEMENT_3D('',#26448,#7804,#7805);
#6640=AXIS2_PLACEMENT_3D('',#26461,#7806,#7807);
#6641=AXIS2_PLACEMENT_3D('',#26462,#7808,#7809);
#6642=AXIS2_PLACEMENT_3D('',#26569,#7810,#7811);
#6643=AXIS2_PLACEMENT_3D('',#26570,#7812,#7813);
#6644=AXIS2_PLACEMENT_3D('',#26677,#7814,#7815);
#6645=AXIS2_PLACEMENT_3D('',#26678,#7816,#7817);
#6646=AXIS2_PLACEMENT_3D('',#26691,#7818,#7819);
#6647=AXIS2_PLACEMENT_3D('',#26782,#7820,#7821);
#6648=AXIS2_PLACEMENT_3D('',#26795,#7822,#7823);
#6649=AXIS2_PLACEMENT_3D('',#26796,#7824,#7825);
#6650=AXIS2_PLACEMENT_3D('',#26973,#7826,#7827);
#6651=AXIS2_PLACEMENT_3D('',#26974,#7828,#7829);
#6652=AXIS2_PLACEMENT_3D('',#26975,#7830,#7831);
#6653=AXIS2_PLACEMENT_3D('',#26976,#7832,#7833);
#6654=AXIS2_PLACEMENT_3D('',#26977,#7834,#7835);
#6655=AXIS2_PLACEMENT_3D('',#26978,#7836,#7837);
#6656=AXIS2_PLACEMENT_3D('',#27003,#7838,#7839);
#6657=AXIS2_PLACEMENT_3D('',#27004,#7840,#7841);
#6658=AXIS2_PLACEMENT_3D('',#27005,#7842,#7843);
#6659=AXIS2_PLACEMENT_3D('',#27006,#7844,#7845);
#6660=AXIS2_PLACEMENT_3D('',#27007,#7846,#7847);
#6661=AXIS2_PLACEMENT_3D('',#27008,#7848,#7849);
#6662=AXIS2_PLACEMENT_3D('',#27009,#7850,#7851);
#6663=AXIS2_PLACEMENT_3D('',#27010,#7852,#7853);
#6664=AXIS2_PLACEMENT_3D('',#27011,#7854,#7855);
#6665=AXIS2_PLACEMENT_3D('',#27012,#7856,#7857);
#6666=AXIS2_PLACEMENT_3D('',#27013,#7858,#7859);
#6667=AXIS2_PLACEMENT_3D('',#27014,#7860,#7861);
#6668=AXIS2_PLACEMENT_3D('',#27015,#7862,#7863);
#6669=AXIS2_PLACEMENT_3D('',#27016,#7864,#7865);
#6670=AXIS2_PLACEMENT_3D('',#27017,#7866,#7867);
#6671=AXIS2_PLACEMENT_3D('',#27066,#7868,#7869);
#6672=AXIS2_PLACEMENT_3D('',#27067,#7870,#7871);
#6673=AXIS2_PLACEMENT_3D('',#27068,#7872,#7873);
#6674=AXIS2_PLACEMENT_3D('',#27069,#7874,#7875);
#6675=AXIS2_PLACEMENT_3D('',#27070,#7876,#7877);
#6676=AXIS2_PLACEMENT_3D('',#27071,#7878,#7879);
#6677=AXIS2_PLACEMENT_3D('',#27072,#7880,#7881);
#6678=AXIS2_PLACEMENT_3D('',#27073,#7882,#7883);
#6679=AXIS2_PLACEMENT_3D('',#27074,#7884,#7885);
#6680=AXIS2_PLACEMENT_3D('',#27075,#7886,#7887);
#6681=AXIS2_PLACEMENT_3D('',#27076,#7888,#7889);
#6682=AXIS2_PLACEMENT_3D('',#27077,#7890,#7891);
#6683=AXIS2_PLACEMENT_3D('',#27078,#7892,#7893);
#6684=AXIS2_PLACEMENT_3D('',#27079,#7894,#7895);
#6685=AXIS2_PLACEMENT_3D('',#27080,#7896,#7897);
#6686=AXIS2_PLACEMENT_3D('',#27129,#7898,#7899);
#6687=AXIS2_PLACEMENT_3D('',#27130,#7900,#7901);
#6688=AXIS2_PLACEMENT_3D('',#27131,#7902,#7903);
#6689=AXIS2_PLACEMENT_3D('',#27132,#7904,#7905);
#6690=AXIS2_PLACEMENT_3D('',#27133,#7906,#7907);
#6691=AXIS2_PLACEMENT_3D('',#27134,#7908,#7909);
#6692=AXIS2_PLACEMENT_3D('',#27135,#7910,#7911);
#6693=AXIS2_PLACEMENT_3D('',#27136,#7912,#7913);
#6694=AXIS2_PLACEMENT_3D('',#27137,#7914,#7915);
#6695=AXIS2_PLACEMENT_3D('',#27138,#7916,#7917);
#6696=AXIS2_PLACEMENT_3D('',#27139,#7918,#7919);
#6697=AXIS2_PLACEMENT_3D('',#27140,#7920,#7921);
#7187=DIRECTION('axis',(0.,0.,1.));
#7188=DIRECTION('refdir',(1.,0.,0.));
#7189=DIRECTION('center_axis',(0.,1.,0.));
#7190=DIRECTION('ref_axis',(0.,0.,1.));
#7191=DIRECTION('',(0.,1.,0.));
#7192=DIRECTION('center_axis',(0.,1.,0.));
#7193=DIRECTION('ref_axis',(0.,0.,-1.));
#7194=DIRECTION('',(0.,1.,0.));
#7195=DIRECTION('center_axis',(0.,1.,0.));
#7196=DIRECTION('ref_axis',(0.,0.,1.));
#7197=DIRECTION('center_axis',(0.,1.,0.));
#7198=DIRECTION('ref_axis',(0.,0.,1.));
#7199=DIRECTION('',(0.,1.,0.));
#7200=DIRECTION('center_axis',(0.,1.,0.));
#7201=DIRECTION('ref_axis',(0.,0.,1.));
#7202=DIRECTION('',(0.,1.,0.));
#7203=DIRECTION('center_axis',(0.,1.,0.));
#7204=DIRECTION('ref_axis',(0.,0.,1.));
#7205=DIRECTION('',(0.,1.,0.));
#7206=DIRECTION('center_axis',(0.,1.,0.));
#7207=DIRECTION('ref_axis',(0.,0.,1.));
#7208=DIRECTION('',(0.,1.,0.));
#7209=DIRECTION('center_axis',(0.,1.,0.));
#7210=DIRECTION('ref_axis',(0.,0.,1.));
#7211=DIRECTION('',(0.,1.,0.));
#7212=DIRECTION('center_axis',(0.,1.,0.));
#7213=DIRECTION('ref_axis',(0.,0.,1.));
#7214=DIRECTION('',(0.,1.,0.));
#7215=DIRECTION('center_axis',(0.,1.,0.));
#7216=DIRECTION('ref_axis',(0.,0.,1.));
#7217=DIRECTION('',(0.,1.,0.));
#7218=DIRECTION('center_axis',(0.,1.,0.));
#7219=DIRECTION('ref_axis',(0.,0.,1.));
#7220=DIRECTION('',(0.,1.,0.));
#7221=DIRECTION('center_axis',(0.,1.,0.));
#7222=DIRECTION('ref_axis',(0.,0.,1.));
#7223=DIRECTION('',(0.,1.,0.));
#7224=DIRECTION('center_axis',(0.,1.,0.));
#7225=DIRECTION('ref_axis',(0.,0.,1.));
#7226=DIRECTION('',(0.,1.,0.));
#7227=DIRECTION('center_axis',(0.,1.,0.));
#7228=DIRECTION('ref_axis',(0.,0.,1.));
#7229=DIRECTION('',(0.,1.,0.));
#7230=DIRECTION('center_axis',(0.,1.,0.));
#7231=DIRECTION('ref_axis',(0.,0.,1.));
#7232=DIRECTION('',(0.,1.,0.));
#7233=DIRECTION('center_axis',(0.,1.,0.));
#7234=DIRECTION('ref_axis',(0.,0.,1.));
#7235=DIRECTION('',(0.,1.,0.));
#7236=DIRECTION('center_axis',(0.,1.,0.));
#7237=DIRECTION('ref_axis',(0.,0.,1.));
#7238=DIRECTION('',(0.,1.,0.));
#7239=DIRECTION('center_axis',(0.,1.,0.));
#7240=DIRECTION('ref_axis',(0.,0.,1.));
#7241=DIRECTION('',(0.,1.,0.));
#7242=DIRECTION('center_axis',(0.,1.,0.));
#7243=DIRECTION('ref_axis',(0.,0.,1.));
#7244=DIRECTION('',(0.,1.,0.));
#7245=DIRECTION('center_axis',(0.,1.,0.));
#7246=DIRECTION('ref_axis',(0.,0.,1.));
#7247=DIRECTION('',(0.,1.,0.));
#7248=DIRECTION('center_axis',(0.,1.,0.));
#7249=DIRECTION('ref_axis',(0.,0.,1.));
#7250=DIRECTION('',(0.,1.,0.));
#7251=DIRECTION('center_axis',(0.,1.,0.));
#7252=DIRECTION('ref_axis',(0.,0.,1.));
#7253=DIRECTION('',(0.,1.,0.));
#7254=DIRECTION('center_axis',(0.,1.,0.));
#7255=DIRECTION('ref_axis',(0.,0.,1.));
#7256=DIRECTION('',(0.,1.,0.));
#7257=DIRECTION('center_axis',(0.,1.,0.));
#7258=DIRECTION('ref_axis',(0.,0.,1.));
#7259=DIRECTION('',(0.,1.,0.));
#7260=DIRECTION('center_axis',(0.,-1.,0.));
#7261=DIRECTION('ref_axis',(1.77635683940025E-15,0.,1.));
#7262=DIRECTION('center_axis',(0.,1.,0.));
#7263=DIRECTION('ref_axis',(0.,0.,1.));
#7264=DIRECTION('center_axis',(0.,1.,0.));
#7265=DIRECTION('ref_axis',(0.,0.,1.));
#7266=DIRECTION('center_axis',(0.,1.,0.));
#7267=DIRECTION('ref_axis',(0.,0.,1.));
#7268=DIRECTION('center_axis',(-1.,0.,1.22464679914735E-16));
#7269=DIRECTION('ref_axis',(-1.22464679914735E-16,0.,-1.));
#7270=DIRECTION('center_axis',(0.,-1.,0.));
#7271=DIRECTION('ref_axis',(0.,0.,1.));
#7272=DIRECTION('center_axis',(0.,1.,0.));
#7273=DIRECTION('ref_axis',(0.,0.,1.));
#7274=DIRECTION('center_axis',(0.,1.,0.));
#7275=DIRECTION('ref_axis',(0.,0.,1.));
#7276=DIRECTION('center_axis',(-1.,0.,1.22464679914735E-16));
#7277=DIRECTION('ref_axis',(-1.22464679914735E-16,0.,-1.));
#7278=DIRECTION('center_axis',(0.,-1.,0.));
#7279=DIRECTION('ref_axis',(0.,0.,1.));
#7280=DIRECTION('center_axis',(0.,-1.,0.));
#7281=DIRECTION('ref_axis',(0.,0.,1.));
#7282=DIRECTION('center_axis',(9.81918948666102E-17,1.,1.70073350800434E-16));
#7283=DIRECTION('ref_axis',(0.,0.,1.));
#7284=DIRECTION('center_axis',(-9.81918948666102E-17,-1.,-1.70073350800434E-16));
#7285=DIRECTION('ref_axis',(-1.66998245814083E-32,-1.70073350800434E-16,
1.));
#7286=DIRECTION('center_axis',(0.866025403784444,0.,-0.499999999999991));
#7287=DIRECTION('ref_axis',(-0.499999999999991,0.,-0.866025403784444));
#7288=DIRECTION('center_axis',(9.81918948666102E-17,1.,1.70073350800434E-16));
#7289=DIRECTION('ref_axis',(-1.66998245814083E-32,-1.70073350800434E-16,
1.));
#7290=DIRECTION('center_axis',(0.499999999999993,2.60208521396517E-15,0.866025403784443));
#7291=DIRECTION('ref_axis',(0.866025403784443,2.19996346842361E-31,-0.499999999999993));
#7292=DIRECTION('center_axis',(-0.333155558300967,0.745673853566471,-0.577042353801262));
#7293=DIRECTION('ref_axis',(-2.59234872084442E-17,0.612005054639087,0.790853850655232));
#7294=DIRECTION('center_axis',(-0.333155558300967,0.745673853566471,-0.577042353801262));
#7295=DIRECTION('ref_axis',(-3.14843324929394E-17,0.612005054639087,0.790853850655232));
#7296=DIRECTION('',(0.333155558300967,-0.745673853566471,0.577042353801262));
#7297=DIRECTION('center_axis',(-0.393636804027377,0.616603816125408,-0.681798944304475));
#7298=DIRECTION('ref_axis',(0.308301907969892,0.787273608054776,0.533994568888617));
#7299=DIRECTION('',(-0.333155558300967,0.745673853566471,-0.577042353801262));
#7300=DIRECTION('center_axis',(0.,1.,0.));
#7301=DIRECTION('ref_axis',(0.,0.,1.));
#7302=DIRECTION('',(0.,-1.,0.));
#7303=DIRECTION('center_axis',(0.,1.,0.));
#7304=DIRECTION('ref_axis',(0.,0.,1.));
#7305=DIRECTION('',(0.,1.,0.));
#7306=DIRECTION('center_axis',(0.,-1.,0.));
#7307=DIRECTION('ref_axis',(0.,0.,-1.));
#7308=DIRECTION('center_axis',(0.,-1.,0.));
#7309=DIRECTION('ref_axis',(0.,0.,-1.));
#7310=DIRECTION('',(0.,1.,0.));
#7311=DIRECTION('center_axis',(9.81918948666125E-17,1.,-1.70073350800433E-16));
#7312=DIRECTION('ref_axis',(1.66998245814086E-32,1.70073350800433E-16,1.));
#7313=DIRECTION('',(0.,-1.,0.));
#7314=DIRECTION('center_axis',(0.333155558300975,-0.745673853566471,-0.577042353801257));
#7315=DIRECTION('ref_axis',(-7.49624866032534E-17,0.612005054639084,-0.790853850655234));
#7316=DIRECTION('center_axis',(0.393636804027381,-0.616603816125443,-0.681798944304441));
#7317=DIRECTION('ref_axis',(0.308301907935341,0.787273608054748,-0.533994568908606));
#7318=DIRECTION('',(-0.333155558300975,0.745673853566471,0.577042353801257));
#7319=DIRECTION('center_axis',(0.333155558300975,-0.745673853566471,-0.577042353801257));
#7320=DIRECTION('ref_axis',(-2.33037419662539E-17,0.612005054639083,-0.790853850655235));
#7321=DIRECTION('',(0.333155558300975,-0.745673853566471,-0.577042353801257));
#7322=DIRECTION('center_axis',(0.,1.,0.));
#7323=DIRECTION('ref_axis',(0.,0.,1.));
#7324=DIRECTION('',(-8.65956056235492E-17,0.707106781186549,-0.707106781186546));
#7325=DIRECTION('center_axis',(0.,-1.,0.));
#7326=DIRECTION('ref_axis',(0.,0.,1.));
#7327=DIRECTION('center_axis',(0.,-1.,0.));
#7328=DIRECTION('ref_axis',(0.,0.,-1.));
#7329=DIRECTION('center_axis',(0.,1.,0.));
#7330=DIRECTION('ref_axis',(8.88178419700125E-16,0.,-1.));
#7331=DIRECTION('center_axis',(0.,-1.,0.));
#7332=DIRECTION('ref_axis',(0.,0.,-1.));
#7333=DIRECTION('center_axis',(9.81918948666102E-17,1.,1.70073350800434E-16));
#7334=DIRECTION('ref_axis',(2.91276184253032E-34,-1.77192702184564E-16,
1.));
#7335=DIRECTION('center_axis',(9.81918948666102E-17,1.,1.70073350800434E-16));
#7336=DIRECTION('ref_axis',(7.25831191047442E-34,-1.70073350800434E-16,
1.));
#7337=DIRECTION('center_axis',(-9.81918948666102E-17,-1.,-1.70073350800434E-16));
#7338=DIRECTION('ref_axis',(-1.77635683940025E-15,-1.70073350800434E-16,
1.));
#7339=DIRECTION('center_axis',(-9.81918948666102E-17,-1.,-1.70073350800434E-16));
#7340=DIRECTION('ref_axis',(-1.77635683940025E-15,-1.70073350800434E-16,
1.));
#7341=DIRECTION('center_axis',(-1.96383789733223E-16,1.,0.));
#7342=DIRECTION('ref_axis',(-1.,-1.77192702184564E-16,0.));
#7343=DIRECTION('center_axis',(-1.96383789733223E-16,1.,0.));
#7344=DIRECTION('ref_axis',(-1.,-1.96383789733223E-16,0.));
#7345=DIRECTION('center_axis',(1.96383789733223E-16,-1.,0.));
#7346=DIRECTION('ref_axis',(-1.,-1.96383789733223E-16,-3.5527136788005E-15));
#7347=DIRECTION('center_axis',(0.,1.,0.));
#7348=DIRECTION('ref_axis',(0.,0.,1.));
#7349=DIRECTION('center_axis',(0.866025403784436,0.,0.500000000000004));
#7350=DIRECTION('ref_axis',(0.500000000000004,0.,-0.866025403784436));
#7351=DIRECTION('center_axis',(-0.866025403784436,0.,-0.500000000000004));
#7352=DIRECTION('ref_axis',(-0.500000000000004,0.,0.866025403784436));
#7353=DIRECTION('',(0.866025403784436,0.,0.500000000000004));
#7354=DIRECTION('center_axis',(-0.866025403784436,0.,-0.500000000000004));
#7355=DIRECTION('ref_axis',(-0.500000000000004,0.,0.866025403784436));
#7356=DIRECTION('center_axis',(-0.866025403784443,0.,0.499999999999992));
#7357=DIRECTION('ref_axis',(0.499999999999992,0.,0.866025403784443));
#7358=DIRECTION('center_axis',(0.866025403784443,0.,-0.499999999999992));
#7359=DIRECTION('ref_axis',(-0.499999999999992,0.,-0.866025403784443));
#7360=DIRECTION('',(-0.866025403784443,0.,0.499999999999992));
#7361=DIRECTION('center_axis',(0.866025403784443,0.,-0.499999999999992));
#7362=DIRECTION('ref_axis',(-0.499999999999992,0.,-0.866025403784443));
#7363=DIRECTION('center_axis',(0.,0.,-1.));
#7364=DIRECTION('ref_axis',(-1.,0.,0.));
#7365=DIRECTION('center_axis',(0.,0.,1.));
#7366=DIRECTION('ref_axis',(1.,0.,0.));
#7367=DIRECTION('',(0.,0.,-1.));
#7368=DIRECTION('center_axis',(0.,0.,1.));
#7369=DIRECTION('ref_axis',(1.,0.,0.));
#7370=DIRECTION('center_axis',(0.,-1.,0.));
#7371=DIRECTION('ref_axis',(0.,0.,-1.));
#7372=DIRECTION('',(0.,1.,0.));
#7373=DIRECTION('',(0.,1.,0.));
#7374=DIRECTION('center_axis',(0.,1.,0.));
#7375=DIRECTION('ref_axis',(-8.88178419700125E-16,0.,-1.));
#7376=DIRECTION('',(0.,1.,0.));
#7377=DIRECTION('center_axis',(0.,1.,0.));
#7378=DIRECTION('ref_axis',(-8.88178419700125E-16,0.,-1.));
#7379=DIRECTION('',(0.,-1.,0.));
#7380=DIRECTION('',(0.,-1.,0.));
#7381=DIRECTION('center_axis',(-9.81918948666125E-17,-1.,1.70073350800433E-16));
#7382=DIRECTION('ref_axis',(-1.18319748428791E-33,1.70073350800433E-16,
1.));
#7383=DIRECTION('',(0.,1.,0.));
#7384=DIRECTION('',(0.,-1.,0.));
#7385=DIRECTION('',(0.,1.,0.));
#7386=DIRECTION('center_axis',(0.,1.,0.));
#7387=DIRECTION('ref_axis',(0.,0.,-1.));
#7388=DIRECTION('center_axis',(0.,1.,0.));
#7389=DIRECTION('ref_axis',(0.,0.,1.));
#7390=DIRECTION('center_axis',(0.,1.,0.));
#7391=DIRECTION('ref_axis',(0.,0.,1.));
#7392=DIRECTION('center_axis',(0.,1.,0.));
#7393=DIRECTION('ref_axis',(0.,0.,1.));
#7394=DIRECTION('center_axis',(0.,1.,0.));
#7395=DIRECTION('ref_axis',(0.,0.,1.));
#7396=DIRECTION('center_axis',(0.,1.,0.));
#7397=DIRECTION('ref_axis',(0.,0.,1.));
#7398=DIRECTION('center_axis',(0.,1.,0.));
#7399=DIRECTION('ref_axis',(0.,0.,1.));
#7400=DIRECTION('center_axis',(0.,1.,0.));
#7401=DIRECTION('ref_axis',(0.,0.,1.));
#7402=DIRECTION('center_axis',(-1.36592399683213E-16,0.,1.));
#7403=DIRECTION('ref_axis',(1.,0.,1.36592399683213E-16));
#7404=DIRECTION('',(0.,-1.,0.));
#7405=DIRECTION('',(1.,0.,1.36592399683213E-16));
#7406=DIRECTION('',(0.,1.,0.));
#7407=DIRECTION('center_axis',(-0.866025403784439,0.,0.5));
#7408=DIRECTION('ref_axis',(0.5,0.,0.866025403784439));
#7409=DIRECTION('',(0.,-1.,0.));
#7410=DIRECTION('',(0.5,0.,0.866025403784439));
#7411=DIRECTION('',(0.,1.,0.));
#7412=DIRECTION('center_axis',(-0.866025403784439,0.,-0.5));
#7413=DIRECTION('ref_axis',(-0.5,0.,0.866025403784439));
#7414=DIRECTION('',(0.,-1.,0.));
#7415=DIRECTION('',(-0.5,0.,0.866025403784439));
#7416=DIRECTION('',(0.,1.,0.));
#7417=DIRECTION('center_axis',(0.,0.,-1.));
#7418=DIRECTION('ref_axis',(-1.,0.,0.));
#7419=DIRECTION('',(0.,-1.,0.));
#7420=DIRECTION('',(-1.,0.,0.));
#7421=DIRECTION('',(0.,1.,0.));
#7422=DIRECTION('center_axis',(0.866025403784439,0.,-0.5));
#7423=DIRECTION('ref_axis',(-0.5,0.,-0.866025403784439));
#7424=DIRECTION('',(0.,-1.,0.));
#7425=DIRECTION('',(-0.5,0.,-0.866025403784439));
#7426=DIRECTION('',(0.,1.,0.));
#7427=DIRECTION('center_axis',(0.866025403784439,0.,0.5));
#7428=DIRECTION('ref_axis',(0.5,0.,-0.866025403784439));
#7429=DIRECTION('',(0.,-1.,0.));
#7430=DIRECTION('',(0.5,0.,-0.866025403784439));
#7431=DIRECTION('',(0.,1.,0.));
#7432=DIRECTION('center_axis',(0.,1.,0.));
#7433=DIRECTION('ref_axis',(0.,0.,1.));
#7434=DIRECTION('center_axis',(0.,1.,0.));
#7435=DIRECTION('ref_axis',(0.,0.,1.));
#7436=DIRECTION('center_axis',(0.,-1.,0.));
#7437=DIRECTION('ref_axis',(-0.297077312093106,0.,0.954853428877718));
#7438=DIRECTION('center_axis',(0.,0.,-1.));
#7439=DIRECTION('ref_axis',(-1.,0.,0.));
#7440=DIRECTION('',(0.,-1.,0.));
#7441=DIRECTION('',(1.,1.96383789733223E-16,0.));
#7442=DIRECTION('',(0.,1.,0.));
#7443=DIRECTION('center_axis',(0.,0.,-1.));
#7444=DIRECTION('ref_axis',(-0.0422331972043614,0.99910778049913,0.));
#7445=DIRECTION('',(-1.,0.,0.));
#7446=DIRECTION('',(-0.666311116601944,-0.745673853566471,0.));
#7447=DIRECTION('center_axis',(0.,0.,-1.));
#7448=DIRECTION('ref_axis',(-1.,0.,0.));
#7449=DIRECTION('',(0.,-1.,0.));
#7450=DIRECTION('',(-1.,-1.96383789733223E-16,0.));
#7451=DIRECTION('',(0.,1.,0.));
#7452=DIRECTION('',(0.666311116601944,0.745673853566471,0.));
#7453=DIRECTION('',(1.,0.,0.));
#7454=DIRECTION('center_axis',(0.,0.,1.));
#7455=DIRECTION('ref_axis',(0.0422331972609955,-0.999107780496736,0.));
#7456=DIRECTION('center_axis',(0.,-1.,0.));
#7457=DIRECTION('ref_axis',(0.,0.,-1.));
#7458=DIRECTION('',(0.,0.,-1.));
#7459=DIRECTION('',(1.,0.,0.));
#7460=DIRECTION('center_axis',(0.,-1.,0.));
#7461=DIRECTION('ref_axis',(0.,0.,-1.));
#7462=DIRECTION('',(-1.,0.,0.));
#7463=DIRECTION('center_axis',(0.,0.,-1.));
#7464=DIRECTION('ref_axis',(-1.,0.,0.));
#7465=DIRECTION('',(0.,0.,-1.));
#7466=DIRECTION('center_axis',(0.,0.,-1.));
#7467=DIRECTION('ref_axis',(-1.,0.,0.));
#7468=DIRECTION('center_axis',(0.,0.,1.));
#7469=DIRECTION('ref_axis',(1.,0.,0.));
#7470=DIRECTION('center_axis',(0.745673853566471,-0.666311116601944,0.));
#7471=DIRECTION('ref_axis',(0.666311116601944,0.745673853566471,0.));
#7472=DIRECTION('',(0.,0.,-1.));
#7473=DIRECTION('',(0.666311116601944,0.745673853566471,0.));
#7474=DIRECTION('',(-0.666311116601944,-0.745673853566471,0.));
#7475=DIRECTION('center_axis',(0.,0.,-1.));
#7476=DIRECTION('ref_axis',(-1.,0.,0.));
#7477=DIRECTION('',(0.,0.,-1.));
#7478=DIRECTION('center_axis',(0.,0.,-1.));
#7479=DIRECTION('ref_axis',(-1.,0.,0.));
#7480=DIRECTION('center_axis',(0.,0.,1.));
#7481=DIRECTION('ref_axis',(-1.,-1.04083408558608E-15,0.));
#7482=DIRECTION('center_axis',(1.,0.,0.));
#7483=DIRECTION('ref_axis',(0.,0.,-1.));
#7484=DIRECTION('',(0.,-1.,0.));
#7485=DIRECTION('',(0.,0.,1.));
#7486=DIRECTION('',(0.,1.,0.));
#7487=DIRECTION('center_axis',(-1.96383789733223E-16,1.,0.));
#7488=DIRECTION('ref_axis',(-1.,-1.96383789733223E-16,0.));
#7489=DIRECTION('center_axis',(-1.96383789733223E-16,1.,0.));
#7490=DIRECTION('ref_axis',(-1.,-1.96383789733223E-16,0.));
#7491=DIRECTION('',(-1.,-1.96383789733223E-16,0.));
#7492=DIRECTION('center_axis',(1.96383789733223E-16,-1.,0.));
#7493=DIRECTION('ref_axis',(-1.,-1.96383789733223E-16,0.));
#7494=DIRECTION('',(0.,0.,-1.));
#7495=DIRECTION('center_axis',(1.96383789733223E-16,-1.,0.));
#7496=DIRECTION('ref_axis',(-1.,-1.96383789733223E-16,0.));
#7497=DIRECTION('',(1.,1.96383789733223E-16,0.));
#7498=DIRECTION('center_axis',(-1.96383789733223E-16,1.,0.));
#7499=DIRECTION('ref_axis',(-1.,-1.96383789733223E-16,0.));
#7500=DIRECTION('center_axis',(-0.866025403784443,0.,0.499999999999992));
#7501=DIRECTION('ref_axis',(0.499999999999992,0.,0.866025403784443));
#7502=DIRECTION('',(0.,-1.,0.));
#7503=DIRECTION('',(-0.499999999999992,1.96383789733223E-16,-0.866025403784443));
#7504=DIRECTION('',(0.,1.,0.));
#7505=DIRECTION('center_axis',(-0.86602540378444,6.35182550169207E-14,0.499999999999998));
#7506=DIRECTION('ref_axis',(-0.0211165986195528,-0.999107780497666,-0.0365750216919776));
#7507=DIRECTION('',(0.499999999999992,0.,0.866025403784443));
#7508=DIRECTION('',(0.333155558300967,-0.745673853566471,0.577042353801262));
#7509=DIRECTION('center_axis',(0.,-1.,0.));
#7510=DIRECTION('ref_axis',(-0.866025403784443,0.,0.499999999999992));
#7511=DIRECTION('',(-0.866025403784443,0.,0.499999999999992));
#7512=DIRECTION('',(-0.499999999999992,0.,-0.866025403784443));
#7513=DIRECTION('center_axis',(0.,-1.,0.));
#7514=DIRECTION('ref_axis',(0.,0.,-1.));
#7515=DIRECTION('',(0.499999999999992,0.,0.866025403784443));
#7516=DIRECTION('center_axis',(-0.866025403784443,0.,0.499999999999992));
#7517=DIRECTION('ref_axis',(0.499999999999992,0.,0.866025403784443));
#7518=DIRECTION('center_axis',(0.866025403784444,0.,-0.499999999999991));
#7519=DIRECTION('ref_axis',(-0.499999999999991,0.,-0.866025403784444));
#7520=DIRECTION('',(-0.866025403784443,0.,0.499999999999992));
#7521=DIRECTION('center_axis',(-0.866025403784443,5.78241158658927E-16,
0.499999999999992));
#7522=DIRECTION('ref_axis',(0.499999999999992,-2.45729362005254E-31,0.866025403784443));
#7523=DIRECTION('center_axis',(-0.372836926783229,-0.666311116601944,-0.645772500126405));
#7524=DIRECTION('ref_axis',(-0.333155558300967,0.745673853566471,-0.577042353801262));
#7525=DIRECTION('',(-0.866025403784443,0.,0.499999999999992));
#7526=DIRECTION('',(-0.333155558300967,0.745673853566471,-0.577042353801262));
#7527=DIRECTION('center_axis',(-0.866025403784443,0.,0.499999999999992));
#7528=DIRECTION('ref_axis',(0.499999999999992,0.,0.866025403784443));
#7529=DIRECTION('center_axis',(0.866025403784443,0.,-0.499999999999992));
#7530=DIRECTION('ref_axis',(0.499999999999992,-2.77555756156289E-15,0.866025403784443));
#7531=DIRECTION('',(-0.866025403784443,0.,0.499999999999992));
#7532=DIRECTION('center_axis',(-0.866025403784443,0.,0.499999999999992));
#7533=DIRECTION('ref_axis',(0.499999999999992,0.,0.866025403784443));
#7534=DIRECTION('center_axis',(-0.499999999999992,0.,-0.866025403784443));
#7535=DIRECTION('ref_axis',(-0.866025403784443,0.,0.499999999999992));
#7536=DIRECTION('',(0.866025403784443,-1.23259516440783E-32,-0.499999999999992));
#7537=DIRECTION('',(0.,1.,0.));
#7538=DIRECTION('center_axis',(9.81918948666102E-17,1.,1.70073350800434E-16));
#7539=DIRECTION('ref_axis',(0.499999999999992,-1.96383789733223E-16,0.866025403784443));
#7540=DIRECTION('center_axis',(9.81918948666102E-17,1.,1.70073350800434E-16));
#7541=DIRECTION('ref_axis',(-1.66998245814083E-32,-1.70073350800434E-16,
1.));
#7542=DIRECTION('',(0.499999999999992,-1.96383789733223E-16,0.866025403784443));
#7543=DIRECTION('center_axis',(-9.81918948666102E-17,-1.,-1.70073350800434E-16));
#7544=DIRECTION('ref_axis',(-1.66998245814083E-32,-1.70073350800434E-16,
1.));
#7545=DIRECTION('',(-0.866025403784443,1.23259516440783E-32,0.499999999999992));
#7546=DIRECTION('',(-0.499999999999992,1.96383789733223E-16,-0.866025403784443));
#7547=DIRECTION('center_axis',(9.81918948666102E-17,1.,1.70073350800434E-16));
#7548=DIRECTION('ref_axis',(-1.66998245814083E-32,-1.70073350800434E-16,
1.));
#7549=DIRECTION('center_axis',(-0.866025403784443,0.,0.499999999999992));
#7550=DIRECTION('ref_axis',(0.499999999999992,0.,0.866025403784443));
#7551=DIRECTION('',(0.,-1.,0.));
#7552=DIRECTION('',(0.499999999999992,-1.96383789733223E-16,0.866025403784443));
#7553=DIRECTION('',(-0.499999999999992,0.,-0.866025403784443));
#7554=DIRECTION('center_axis',(0.866025403784441,-2.51426426109907E-14,
-0.499999999999997));
#7555=DIRECTION('ref_axis',(0.021116598590189,0.999107780500145,0.0365750216411948));
#7556=DIRECTION('center_axis',(0.866025403784436,0.,0.500000000000004));
#7557=DIRECTION('ref_axis',(0.500000000000004,0.,-0.866025403784436));
#7558=DIRECTION('',(-0.500000000000004,1.96383789733224E-16,0.866025403784436));
#7559=DIRECTION('',(0.,1.,0.));
#7560=DIRECTION('center_axis',(0.866025403784437,-2.51426426109492E-14,
0.500000000000004));
#7561=DIRECTION('ref_axis',(-0.0211165986015709,-0.999107780499183,0.0365750216609081));
#7562=DIRECTION('',(0.500000000000004,0.,-0.866025403784436));
#7563=DIRECTION('center_axis',(0.,-1.,0.));
#7564=DIRECTION('ref_axis',(0.866025403784436,0.,0.500000000000004));
#7565=DIRECTION('',(0.866025403784436,0.,0.500000000000004));
#7566=DIRECTION('',(-0.500000000000004,0.,0.866025403784436));
#7567=DIRECTION('',(0.500000000000004,0.,-0.866025403784436));
#7568=DIRECTION('center_axis',(0.866025403784436,0.,0.500000000000004));
#7569=DIRECTION('ref_axis',(0.500000000000004,0.,-0.866025403784436));
#7570=DIRECTION('center_axis',(-0.866025403784434,0.,-0.500000000000008));
#7571=DIRECTION('ref_axis',(-0.500000000000008,0.,0.866025403784434));
#7572=DIRECTION('',(0.866025403784436,0.,0.500000000000004));
#7573=DIRECTION('center_axis',(0.866025403784436,-6.55710784405496E-16,
0.500000000000004));
#7574=DIRECTION('ref_axis',(0.500000000000004,1.88743283563644E-31,-0.866025403784436));
#7575=DIRECTION('center_axis',(-0.372836926783238,-0.666311116601944,0.6457725001264));
#7576=DIRECTION('ref_axis',(-0.333155558300975,0.745673853566471,0.577042353801257));
#7577=DIRECTION('',(0.333155558300975,-0.745673853566471,-0.577042353801257));
#7578=DIRECTION('',(0.866025403784436,0.,0.500000000000004));
#7579=DIRECTION('center_axis',(0.866025403784436,0.,0.500000000000004));
#7580=DIRECTION('ref_axis',(0.500000000000004,0.,-0.866025403784436));
#7581=DIRECTION('center_axis',(-0.866025403784436,0.,-0.500000000000004));
#7582=DIRECTION('ref_axis',(0.500000000000004,0.,-0.866025403784436));
#7583=DIRECTION('',(0.866025403784436,0.,0.500000000000004));
#7584=DIRECTION('center_axis',(0.866025403784436,0.,0.500000000000004));
#7585=DIRECTION('ref_axis',(0.500000000000004,0.,-0.866025403784436));
#7586=DIRECTION('center_axis',(-0.500000000000004,0.,0.866025403784436));
#7587=DIRECTION('ref_axis',(0.866025403784436,0.,0.500000000000004));
#7588=DIRECTION('',(0.,-1.,0.));
#7589=DIRECTION('',(-0.866025403784436,-1.23259516440783E-32,-0.500000000000004));
#7590=DIRECTION('center_axis',(9.81918948666125E-17,1.,-1.70073350800433E-16));
#7591=DIRECTION('ref_axis',(0.500000000000004,-1.96383789733223E-16,-0.866025403784436));
#7592=DIRECTION('center_axis',(9.81918948666125E-17,1.,-1.70073350800433E-16));
#7593=DIRECTION('ref_axis',(-7.25831191047587E-34,1.70073350800433E-16,
1.));
#7594=DIRECTION('center_axis',(9.81918948666125E-17,1.,-1.70073350800433E-16));
#7595=DIRECTION('ref_axis',(1.66998245814086E-32,1.70073350800433E-16,1.));
#7596=DIRECTION('',(0.500000000000004,-1.96383789733224E-16,-0.866025403784436));
#7597=DIRECTION('center_axis',(-9.81918948666125E-17,-1.,1.70073350800433E-16));
#7598=DIRECTION('ref_axis',(1.66998245814086E-32,1.70073350800433E-16,1.));
#7599=DIRECTION('',(0.866025403784436,1.23259516440783E-32,0.500000000000004));
#7600=DIRECTION('center_axis',(-9.81918948666125E-17,-1.,1.70073350800433E-16));
#7601=DIRECTION('ref_axis',(1.73472347597681E-15,1.70073350800433E-16,1.));
#7602=DIRECTION('',(-0.500000000000004,1.96383789733224E-16,0.866025403784436));
#7603=DIRECTION('center_axis',(9.81918948666125E-17,1.,-1.70073350800433E-16));
#7604=DIRECTION('ref_axis',(1.66998245814086E-32,1.70073350800433E-16,1.));
#7605=DIRECTION('center_axis',(0.866025403784436,0.,0.500000000000004));
#7606=DIRECTION('ref_axis',(0.500000000000004,0.,-0.866025403784436));
#7607=DIRECTION('',(0.,-1.,0.));
#7608=DIRECTION('',(0.500000000000004,-1.96383789733224E-16,-0.866025403784436));
#7609=DIRECTION('',(0.,1.,0.));
#7610=DIRECTION('',(-0.333155558300975,0.745673853566471,0.577042353801257));
#7611=DIRECTION('',(-0.500000000000004,0.,0.866025403784436));
#7612=DIRECTION('center_axis',(-0.866025403784436,-2.24960486516661E-14,
-0.500000000000004));
#7613=DIRECTION('ref_axis',(0.0211165986566772,0.999107780494521,-0.0365750217564501));
#7614=DIRECTION('center_axis',(0.,-1.,0.));
#7615=DIRECTION('ref_axis',(0.,0.,-1.));
#7616=DIRECTION('center_axis',(1.96383789733223E-16,-1.,0.));
#7617=DIRECTION('ref_axis',(-1.,-1.96383789733223E-16,6.01006558606138E-15));
#7618=DIRECTION('center_axis',(0.,-1.,0.));
#7619=DIRECTION('ref_axis',(0.,0.,-1.));
#7620=DIRECTION('center_axis',(-9.81918948666125E-17,-1.,1.70073350800433E-16));
#7621=DIRECTION('ref_axis',(2.48598167423448E-14,1.7007335080043E-16,1.));
#7622=DIRECTION('center_axis',(0.,-1.,0.));
#7623=DIRECTION('ref_axis',(0.,0.,-1.));
#7624=DIRECTION('center_axis',(-9.81918948666125E-17,-1.,1.70073350800433E-16));
#7625=DIRECTION('ref_axis',(-1.63910879619856E-15,1.70073350800433E-16,
1.));
#7626=DIRECTION('center_axis',(0.,-1.,0.));
#7627=DIRECTION('ref_axis',(0.,0.,-1.));
#7628=DIRECTION('center_axis',(-9.81918948666102E-17,-1.,-1.70073350800434E-16));
#7629=DIRECTION('ref_axis',(-1.66998245814083E-32,-1.70073350800434E-16,
1.));
#7630=DIRECTION('center_axis',(0.,-1.,0.));
#7631=DIRECTION('ref_axis',(0.,0.,-1.));
#7632=DIRECTION('center_axis',(-9.81918948666102E-17,-1.,-1.70073350800434E-16));
#7633=DIRECTION('ref_axis',(-1.06542071752906E-14,-1.70073350800433E-16,
1.));
#7634=DIRECTION('center_axis',(0.,-1.,0.));
#7635=DIRECTION('ref_axis',(0.,0.,-1.));
#7636=DIRECTION('center_axis',(1.96383789733223E-16,-1.,0.));
#7637=DIRECTION('ref_axis',(-1.,-1.96383789733223E-16,-1.63910879619856E-15));
#7638=DIRECTION('center_axis',(9.81918948666125E-17,1.,-1.70073350800433E-16));
#7639=DIRECTION('ref_axis',(0.500000000000005,-1.77192702184564E-16,-0.866025403784436));
#7640=DIRECTION('center_axis',(0.,-1.,0.));
#7641=DIRECTION('ref_axis',(0.499999999999993,0.,0.866025403784443));
#7642=DIRECTION('center_axis',(0.,-1.,0.));
#7643=DIRECTION('ref_axis',(0.,0.,-1.));
#7644=DIRECTION('center_axis',(0.,-1.,0.));
#7645=DIRECTION('ref_axis',(0.,0.,-1.));
#7646=DIRECTION('center_axis',(0.,1.,0.));
#7647=DIRECTION('ref_axis',(0.,0.,1.));
#7648=DIRECTION('',(0.5,0.,-0.866025403784439));
#7649=DIRECTION('center_axis',(0.,-1.,0.));
#7650=DIRECTION('ref_axis',(1.73472347597681E-15,0.,1.));
#7651=DIRECTION('',(1.,0.,0.));
#7652=DIRECTION('center_axis',(0.,-1.,0.));
#7653=DIRECTION('ref_axis',(2.60208521396521E-15,0.,1.));
#7654=DIRECTION('',(0.5,0.,0.866025403784439));
#7655=DIRECTION('center_axis',(0.,-1.,0.));
#7656=DIRECTION('ref_axis',(1.73472347597681E-15,0.,1.));
#7657=DIRECTION('',(-0.5,0.,0.866025403784439));
#7658=DIRECTION('center_axis',(0.,-1.,0.));
#7659=DIRECTION('ref_axis',(-3.46944695195362E-15,0.,1.));
#7660=DIRECTION('',(-1.,0.,-1.36592399683213E-16));
#7661=DIRECTION('center_axis',(0.,-1.,0.));
#7662=DIRECTION('ref_axis',(0.,0.,1.));
#7663=DIRECTION('',(-0.5,0.,-0.866025403784439));
#7664=DIRECTION('center_axis',(0.,-1.,0.));
#7665=DIRECTION('ref_axis',(0.,0.,1.));
#7666=DIRECTION('center_axis',(0.,-1.,0.));
#7667=DIRECTION('ref_axis',(0.,0.,1.));
#7668=DIRECTION('center_axis',(0.,-1.,0.));
#7669=DIRECTION('ref_axis',(0.,0.,1.));
#7670=DIRECTION('center_axis',(0.,-1.,0.));
#7671=DIRECTION('ref_axis',(0.,0.,1.));
#7672=DIRECTION('center_axis',(0.,-1.,0.));
#7673=DIRECTION('ref_axis',(0.,0.,1.));
#7674=DIRECTION('center_axis',(0.,-1.,0.));
#7675=DIRECTION('ref_axis',(0.,0.,1.));
#7676=DIRECTION('center_axis',(0.,-1.,0.));
#7677=DIRECTION('ref_axis',(0.,0.,1.));
#7678=DIRECTION('center_axis',(0.,1.,0.));
#7679=DIRECTION('ref_axis',(0.,0.,1.));
#7680=DIRECTION('center_axis',(0.,1.,0.));
#7681=DIRECTION('ref_axis',(0.,0.,1.));
#7682=DIRECTION('center_axis',(0.,1.,0.));
#7683=DIRECTION('ref_axis',(0.,0.,1.));
#7684=DIRECTION('center_axis',(0.,1.,0.));
#7685=DIRECTION('ref_axis',(0.,0.,1.));
#7686=DIRECTION('center_axis',(0.,1.,0.));
#7687=DIRECTION('ref_axis',(0.,0.,1.));
#7688=DIRECTION('center_axis',(0.,1.,0.));
#7689=DIRECTION('ref_axis',(0.,0.,1.));
#7690=DIRECTION('center_axis',(0.,1.,0.));
#7691=DIRECTION('ref_axis',(0.,0.,1.));
#7692=DIRECTION('center_axis',(0.,1.,0.));
#7693=DIRECTION('ref_axis',(0.,0.,1.));
#7694=DIRECTION('center_axis',(0.,1.,0.));
#7695=DIRECTION('ref_axis',(0.,0.,1.));
#7696=DIRECTION('center_axis',(0.,1.,0.));
#7697=DIRECTION('ref_axis',(0.,0.,1.));
#7698=DIRECTION('center_axis',(0.,1.,0.));
#7699=DIRECTION('ref_axis',(0.,0.,1.));
#7700=DIRECTION('center_axis',(0.,1.,0.));
#7701=DIRECTION('ref_axis',(0.,0.,1.));
#7702=DIRECTION('center_axis',(0.,1.,0.));
#7703=DIRECTION('ref_axis',(0.,0.,1.));
#7704=DIRECTION('center_axis',(-0.499999999999999,1.93599546773136E-15,
0.866025403784439));
#7705=DIRECTION('ref_axis',(0.866025403784439,9.70515073617369E-31,0.499999999999999));
#7706=DIRECTION('center_axis',(1.,0.,0.));
#7707=DIRECTION('ref_axis',(0.,0.,-1.));
#7708=DIRECTION('center_axis',(-1.,0.,-1.36592399683213E-16));
#7709=DIRECTION('ref_axis',(-1.36592399683213E-16,0.,1.));
#7710=DIRECTION('center_axis',(1.,0.,0.));
#7711=DIRECTION('ref_axis',(0.,0.,-1.));
#7712=DIRECTION('center_axis',(-0.5,0.,0.866025403784439));
#7713=DIRECTION('ref_axis',(0.866025403784439,0.,0.5));
#7714=DIRECTION('center_axis',(-0.5,2.29809145050324E-15,0.866025403784439));
#7715=DIRECTION('ref_axis',(0.866025403784439,6.9389298859906E-31,0.5));
#7716=DIRECTION('center_axis',(0.,1.,0.));
#7717=DIRECTION('ref_axis',(0.,0.,1.));
#7718=DIRECTION('center_axis',(0.5,0.,0.866025403784438));
#7719=DIRECTION('ref_axis',(0.866025403784438,0.,-0.5));
#7720=DIRECTION('center_axis',(0.,1.,0.));
#7721=DIRECTION('ref_axis',(0.,0.,1.));
#7722=DIRECTION('center_axis',(0.5,0.,0.866025403784439));
#7723=DIRECTION('ref_axis',(0.866025403784439,0.,-0.5));
#7724=DIRECTION('center_axis',(-0.5,0.,-0.866025403784439));
#7725=DIRECTION('ref_axis',(-0.866025403784439,0.,0.5));
#7726=DIRECTION('center_axis',(0.5,0.,0.866025403784439));
#7727=DIRECTION('ref_axis',(0.866025403784439,0.,-0.5));
#7728=DIRECTION('center_axis',(0.5,0.,0.866025403784439));
#7729=DIRECTION('ref_axis',(0.866025403784439,0.,-0.5));
#7730=DIRECTION('center_axis',(0.5,4.33680868994203E-16,0.866025403784438));
#7731=DIRECTION('ref_axis',(0.866025403784438,5.77289724224632E-33,-0.5));
#7732=DIRECTION('center_axis',(0.,1.,0.));
#7733=DIRECTION('ref_axis',(0.,0.,1.));
#7734=DIRECTION('center_axis',(-0.5,0.,0.866025403784439));
#7735=DIRECTION('ref_axis',(0.866025403784439,0.,0.5));
#7736=DIRECTION('center_axis',(0.,1.,0.));
#7737=DIRECTION('ref_axis',(0.,0.,1.));
#7738=DIRECTION('center_axis',(1.,0.,0.));
#7739=DIRECTION('ref_axis',(0.,0.,-1.));
#7740=DIRECTION('center_axis',(0.5,0.,-0.866025403784439));
#7741=DIRECTION('ref_axis',(-0.866025403784439,0.,-0.5));
#7742=DIRECTION('center_axis',(-0.5,0.,0.866025403784439));
#7743=DIRECTION('ref_axis',(0.866025403784439,0.,0.5));
#7744=DIRECTION('center_axis',(1.,0.,0.));
#7745=DIRECTION('ref_axis',(0.,0.,-1.));
#7746=DIRECTION('center_axis',(1.,0.,0.));
#7747=DIRECTION('ref_axis',(0.,0.,-1.));
#7748=DIRECTION('center_axis',(0.,1.,0.));
#7749=DIRECTION('ref_axis',(0.,0.,1.));
#7750=DIRECTION('center_axis',(0.,-1.,0.));
#7751=DIRECTION('ref_axis',(0.,0.,-1.));
#7752=DIRECTION('center_axis',(-1.96383789733223E-16,1.,0.));
#7753=DIRECTION('ref_axis',(-1.,-1.96383789733223E-16,0.));
#7754=DIRECTION('center_axis',(0.,1.,0.));
#7755=DIRECTION('ref_axis',(0.,0.,1.));
#7756=DIRECTION('center_axis',(0.,1.,0.));
#7757=DIRECTION('ref_axis',(-1.,0.,0.));
#7758=DIRECTION('center_axis',(0.666311116601944,0.745673853566471,0.));
#7759=DIRECTION('ref_axis',(-0.745673853566471,0.666311116601944,0.));
#7760=DIRECTION('center_axis',(-0.666311116601944,-0.745673853566471,0.));
#7761=DIRECTION('ref_axis',(0.745673853566471,-0.666311116601944,0.));
#7762=DIRECTION('center_axis',(-1.,0.,0.));
#7763=DIRECTION('ref_axis',(0.,0.,1.));
#7764=DIRECTION('center_axis',(1.,0.,0.));
#7765=DIRECTION('ref_axis',(0.,0.,-1.));
#7766=DIRECTION('center_axis',(0.984161952974649,0.177271685040576,2.82385335648104E-15));
#7767=DIRECTION('ref_axis',(-0.177271685040576,0.984161952974649,-4.640930146752E-31));
#7768=DIRECTION('center_axis',(0.,1.,0.));
#7769=DIRECTION('ref_axis',(0.,0.,1.));
#7770=DIRECTION('center_axis',(-1.96383789733223E-16,1.,0.));
#7771=DIRECTION('ref_axis',(-1.,-1.96383789733223E-16,0.));
#7772=DIRECTION('center_axis',(0.,1.,0.));
#7773=DIRECTION('ref_axis',(0.,0.,1.));
#7774=DIRECTION('center_axis',(0.,1.,0.));
#7775=DIRECTION('ref_axis',(-1.,0.,0.));
#7776=DIRECTION('center_axis',(0.666311116601944,0.745673853566471,0.));
#7777=DIRECTION('ref_axis',(-0.745673853566471,0.666311116601944,0.));
#7778=DIRECTION('center_axis',(0.666311116601944,0.745673853566471,0.));
#7779=DIRECTION('ref_axis',(-0.745673853566471,0.666311116601944,0.));
#7780=DIRECTION('center_axis',(1.,0.,0.));
#7781=DIRECTION('ref_axis',(0.,0.,-1.));
#7782=DIRECTION('center_axis',(1.,0.,0.));
#7783=DIRECTION('ref_axis',(0.,0.,-1.));
#7784=DIRECTION('center_axis',(0.984161952974649,0.177271685040574,0.));
#7785=DIRECTION('ref_axis',(-0.177271685040574,0.984161952974649,0.));
#7786=DIRECTION('center_axis',(0.,1.,0.));
#7787=DIRECTION('ref_axis',(0.,0.,1.));
#7788=DIRECTION('center_axis',(9.81918948666125E-17,1.,-1.70073350800433E-16));
#7789=DIRECTION('ref_axis',(1.66998245814086E-32,1.70073350800433E-16,1.));
#7790=DIRECTION('center_axis',(0.,1.,0.));
#7791=DIRECTION('ref_axis',(0.,0.,1.));
#7792=DIRECTION('center_axis',(0.,1.,0.));
#7793=DIRECTION('ref_axis',(0.500000000000005,0.,-0.866025403784436));
#7794=DIRECTION('center_axis',(-0.333155558300976,0.74567385356647,0.577042353801258));
#7795=DIRECTION('ref_axis',(-8.34044259913248E-17,-0.612005054639085,0.790853850655234));
#7796=DIRECTION('center_axis',(-0.333155558300975,0.745673853566471,0.577042353801257));
#7797=DIRECTION('ref_axis',(7.49624866032534E-17,-0.612005054639084,0.790853850655234));
#7798=DIRECTION('center_axis',(-0.500000000000004,0.,0.866025403784436));
#7799=DIRECTION('ref_axis',(0.866025403784436,0.,0.500000000000004));
#7800=DIRECTION('center_axis',(-0.500000000000004,-9.29635508958665E-17,
0.866025403784436));
#7801=DIRECTION('ref_axis',(0.866025403784436,2.67365344803013E-32,0.500000000000004));
#7802=DIRECTION('center_axis',(-0.492080976487329,0.177271685040574,0.85230925271415));
#7803=DIRECTION('ref_axis',(0.866025403784436,9.07442760845917E-18,0.500000000000004));
#7804=DIRECTION('center_axis',(0.492080976487328,-0.177271685040574,-0.85230925271415));
#7805=DIRECTION('ref_axis',(-0.866025403784436,1.51531198058906E-18,-0.500000000000004));
#7806=DIRECTION('center_axis',(0.500000000000004,-4.33680868994205E-16,
-0.866025403784436));
#7807=DIRECTION('ref_axis',(-0.866025403784436,-4.66515379724155E-32,-0.500000000000004));
#7808=DIRECTION('center_axis',(0.500000000000004,0.,-0.866025403784436));
#7809=DIRECTION('ref_axis',(-0.866025403784436,0.,-0.500000000000004));
#7810=DIRECTION('center_axis',(0.,1.,0.));
#7811=DIRECTION('ref_axis',(0.500000000000004,0.,-0.866025403784436));
#7812=DIRECTION('center_axis',(0.,1.,0.));
#7813=DIRECTION('ref_axis',(0.499999999999993,0.,0.866025403784443));
#7814=DIRECTION('center_axis',(-0.499999999999992,0.,-0.866025403784443));
#7815=DIRECTION('ref_axis',(-0.866025403784443,0.,0.499999999999992));
#7816=DIRECTION('center_axis',(-0.499999999999992,3.46944695195356E-16,
-0.866025403784443));
#7817=DIRECTION('ref_axis',(-0.866025403784443,3.51994154947752E-32,0.499999999999992));
#7818=DIRECTION('center_axis',(-0.492080976487317,0.177271685040573,-0.852309252714157));
#7819=DIRECTION('ref_axis',(-0.866025403784443,6.20279384261769E-18,0.499999999999992));
#7820=DIRECTION('center_axis',(0.492080976487317,-0.177271685040574,0.852309252714157));
#7821=DIRECTION('ref_axis',(0.866025403784443,8.18616803104063E-18,-0.499999999999992));
#7822=DIRECTION('center_axis',(0.499999999999992,3.00462919747434E-16,0.866025403784443));
#7823=DIRECTION('ref_axis',(0.866025403784443,-2.69630192211791E-33,-0.499999999999992));
#7824=DIRECTION('center_axis',(0.499999999999992,0.,0.866025403784443));
#7825=DIRECTION('ref_axis',(0.866025403784443,0.,-0.499999999999992));
#7826=DIRECTION('center_axis',(0.333155558300967,-0.745673853566471,0.577042353801262));
#7827=DIRECTION('ref_axis',(2.59234872084442E-17,-0.612005054639087,-0.790853850655232));
#7828=DIRECTION('center_axis',(0.333155558300966,-0.745673853566471,0.577042353801261));
#7829=DIRECTION('ref_axis',(-1.20939466035638E-17,-0.612005054639087,-0.790853850655232));
#7830=DIRECTION('center_axis',(0.,1.,0.));
#7831=DIRECTION('ref_axis',(0.499999999999991,0.,0.866025403784444));
#7832=DIRECTION('center_axis',(0.,-1.,0.));
#7833=DIRECTION('ref_axis',(0.,0.,-1.));
#7834=DIRECTION('center_axis',(0.,-1.,0.));
#7835=DIRECTION('ref_axis',(0.,0.,-1.));
#7836=DIRECTION('center_axis',(9.81918948666102E-17,1.,1.70073350800434E-16));
#7837=DIRECTION('ref_axis',(-1.66998245814083E-32,-1.70073350800434E-16,
1.));
#7838=DIRECTION('center_axis',(-0.986265445452608,8.54626199733501E-15,
-0.165168008724958));
#7839=DIRECTION('ref_axis',(-0.165168008724958,-6.85891870706028E-33,0.986265445452608));
#7840=DIRECTION('center_axis',(-1.96383789733223E-16,1.,0.));
#7841=DIRECTION('ref_axis',(-1.,0.,0.));
#7842=DIRECTION('center_axis',(-1.,0.,0.));
#7843=DIRECTION('ref_axis',(0.,0.,1.));
#7844=DIRECTION('center_axis',(1.,1.96383789733223E-16,0.));
#7845=DIRECTION('ref_axis',(-1.96383789733223E-16,1.,0.));
#7846=DIRECTION('center_axis',(-1.,0.,0.));
#7847=DIRECTION('ref_axis',(0.,0.,1.));
#7848=DIRECTION('center_axis',(-1.96383789733223E-16,1.,0.));
#7849=DIRECTION('ref_axis',(-1.,0.,0.));
#7850=DIRECTION('center_axis',(0.,0.,-1.));
#7851=DIRECTION('ref_axis',(-1.,0.,0.));
#7852=DIRECTION('center_axis',(0.,0.,-1.));
#7853=DIRECTION('ref_axis',(-1.,0.,0.));
#7854=DIRECTION('center_axis',(0.,0.,-1.));
#7855=DIRECTION('ref_axis',(-1.,0.,0.));
#7856=DIRECTION('center_axis',(-1.96383789733223E-16,1.,0.));
#7857=DIRECTION('ref_axis',(-1.,0.,0.));
#7858=DIRECTION('center_axis',(1.,0.,0.));
#7859=DIRECTION('ref_axis',(0.,0.,-1.));
#7860=DIRECTION('center_axis',(-1.,-1.96383789733223E-16,0.));
#7861=DIRECTION('ref_axis',(1.96383789733223E-16,-1.,0.));
#7862=DIRECTION('center_axis',(1.,0.,0.));
#7863=DIRECTION('ref_axis',(0.,0.,-1.));
#7864=DIRECTION('center_axis',(-1.96383789733223E-16,1.,0.));
#7865=DIRECTION('ref_axis',(-1.,0.,0.));
#7866=DIRECTION('center_axis',(0.986265445452611,0.,-0.165168008724946));
#7867=DIRECTION('ref_axis',(-0.165168008724946,0.,-0.98626544545261));
#7868=DIRECTION('center_axis',(0.350093031278016,8.12470694020607E-16,-0.936714934999208));
#7869=DIRECTION('ref_axis',(-0.936714934999208,-6.70893457146978E-32,-0.350093031278016));
#7870=DIRECTION('center_axis',(9.81918948666125E-17,1.,-1.70073350800433E-16));
#7871=DIRECTION('ref_axis',(0.,0.,1.));
#7872=DIRECTION('center_axis',(0.500000000000005,-1.50231459873715E-15,
-0.866025403784436));
#7873=DIRECTION('ref_axis',(-0.866025403784435,2.19556013660713E-32,-0.500000000000005));
#7874=DIRECTION('center_axis',(0.500000000000004,-1.96383789733224E-16,
-0.866025403784436));
#7875=DIRECTION('ref_axis',(-0.866025403784436,1.62736006015126E-32,-0.500000000000004));
#7876=DIRECTION('center_axis',(0.500000000000007,0.,-0.866025403784435));
#7877=DIRECTION('ref_axis',(-0.866025403784435,0.,-0.500000000000007));
#7878=DIRECTION('center_axis',(9.81918948666125E-17,1.,-1.70073350800433E-16));
#7879=DIRECTION('ref_axis',(0.,0.,1.));
#7880=DIRECTION('center_axis',(-0.866025403784438,-3.46944695195362E-15,
-0.500000000000002));
#7881=DIRECTION('ref_axis',(-0.500000000000001,3.32427446512172E-33,0.866025403784438));
#7882=DIRECTION('center_axis',(0.866025403784436,1.23259516440783E-32,0.500000000000004));
#7883=DIRECTION('ref_axis',(0.500000000000004,-2.42099675731877E-49,-0.866025403784436));
#7884=DIRECTION('center_axis',(-0.866025403784436,-4.64817754479332E-16,
-0.500000000000004));
#7885=DIRECTION('ref_axis',(-0.500000000000004,5.15704192091073E-32,0.866025403784436));
#7886=DIRECTION('center_axis',(9.81918948666125E-17,1.,-1.70073350800433E-16));
#7887=DIRECTION('ref_axis',(-0.258819045102516,0.,-0.96592582628907));
#7888=DIRECTION('center_axis',(-0.500000000000007,8.67361737988414E-16,
0.866025403784435));
#7889=DIRECTION('ref_axis',(0.866025403784435,-6.81437383295693E-31,0.500000000000007));
#7890=DIRECTION('center_axis',(-0.500000000000004,1.96383789733224E-16,
0.866025403784436));
#7891=DIRECTION('ref_axis',(0.866025403784436,-5.83267376229116E-31,0.500000000000004));
#7892=DIRECTION('center_axis',(-0.500000000000004,0.,0.866025403784436));
#7893=DIRECTION('ref_axis',(0.866025403784436,0.,0.500000000000004));
#7894=DIRECTION('center_axis',(9.81918948666125E-17,1.,-1.70073350800433E-16));
#7895=DIRECTION('ref_axis',(0.,0.,1.));
#7896=DIRECTION('center_axis',(-0.636172414174605,5.51791610818759E-16,
0.771546926274258));
#7897=DIRECTION('ref_axis',(0.771546926274258,-2.75521141229581E-31,0.636172414174605));
#7898=DIRECTION('center_axis',(0.636172414174592,2.75895805409376E-16,0.771546926274269));
#7899=DIRECTION('ref_axis',(0.771546926274269,-8.00143989047643E-32,-0.636172414174592));
#7900=DIRECTION('center_axis',(9.81918948666102E-17,1.,1.70073350800434E-16));
#7901=DIRECTION('ref_axis',(0.,0.,1.));
#7902=DIRECTION('center_axis',(0.49999999999999,-2.78778876297724E-15,0.866025403784444));
#7903=DIRECTION('ref_axis',(0.866025403784444,1.07195328581195E-30,-0.49999999999999));
#7904=DIRECTION('center_axis',(0.499999999999992,-1.96383789733223E-16,
0.866025403784443));
#7905=DIRECTION('ref_axis',(0.866025403784443,-2.82965419628534E-32,-0.499999999999992));
#7906=DIRECTION('center_axis',(-0.866025403784443,1.23259516440783E-32,
0.499999999999992));
#7907=DIRECTION('ref_axis',(0.499999999999992,1.98035884533862E-47,0.866025403784443));
#7908=DIRECTION('center_axis',(0.866025403784442,0.,-0.499999999999993));
#7909=DIRECTION('ref_axis',(-0.499999999999993,0.,-0.866025403784443));
#7910=DIRECTION('center_axis',(9.81918948666102E-17,1.,1.70073350800434E-16));
#7911=DIRECTION('ref_axis',(0.,0.,1.));
#7912=DIRECTION('center_axis',(-0.499999999999993,0.,-0.866025403784443));
#7913=DIRECTION('ref_axis',(-0.866025403784443,0.,0.499999999999993));
#7914=DIRECTION('center_axis',(-0.499999999999992,1.96383789733223E-16,
-0.866025403784443));
#7915=DIRECTION('ref_axis',(-0.866025403784443,3.11793429776653E-31,0.499999999999992));
#7916=DIRECTION('center_axis',(-0.499999999999992,2.32408877239612E-16,
-0.866025403784443));
#7917=DIRECTION('ref_axis',(-0.866025403784443,-4.65759760521399E-33,0.499999999999992));
#7918=DIRECTION('center_axis',(9.81918948666102E-17,1.,1.70073350800434E-16));
#7919=DIRECTION('ref_axis',(0.,0.,1.));
#7920=DIRECTION('center_axis',(-0.350093031278002,3.65204128232947E-15,
-0.936714934999213));
#7921=DIRECTION('ref_axis',(-0.936714934999213,-9.98642723764943E-32,0.350093031278002));
#9084=CARTESIAN_POINT('',(0.,0.,0.));
#9085=CARTESIAN_POINT('Origin',(0.,-25.4,0.));
#9086=CARTESIAN_POINT('',(-8.53327934765894E-14,19.7627746953453,-8.326));
#9087=CARTESIAN_POINT('',(1.31190385833674E-13,20.1637230794129,-8.326));
#9088=CARTESIAN_POINT('',(-1.01964092497009E-15,-25.4,-8.326));
#9089=CARTESIAN_POINT('',(1.15457232288591,22.22,-8.24555872886889));
#9090=CARTESIAN_POINT('Ctrl Pts',(2.9393154576951E-13,20.1637230794129,
-8.326));
#9091=CARTESIAN_POINT('Ctrl Pts',(-0.708200717931855,20.1895051998125,-8.326));
#9092=CARTESIAN_POINT('Ctrl Pts',(-1.41494612036022,20.2171332728378,-8.23565416784787));
#9093=CARTESIAN_POINT('Ctrl Pts',(-3.16729826485032,20.2905430311874,-7.77819055474686));
#9094=CARTESIAN_POINT('Ctrl Pts',(-4.16596846789998,20.3371138773749,-7.29223028439277));
#9095=CARTESIAN_POINT('Ctrl Pts',(-5.88380050089614,20.4271213329289,-5.98530507331128));
#9096=CARTESIAN_POINT('Ctrl Pts',(-6.59647033054524,20.4697946579353,-5.1894105472544));
#9097=CARTESIAN_POINT('Ctrl Pts',(-7.70794823763998,20.5492238742483,-3.33553158228336));
#9098=CARTESIAN_POINT('Ctrl Pts',(-8.08157861678374,20.5926134393248,-2.28631103821033));
#9099=CARTESIAN_POINT('Ctrl Pts',(-8.39575024460199,20.6837076506364,-0.119309885693965));
#9100=CARTESIAN_POINT('Ctrl Pts',(-8.33966207607041,20.7297596899249,0.976202340350647));
#9101=CARTESIAN_POINT('Ctrl Pts',(-7.81768239149004,20.8170405939904,3.05249036106223));
#9102=CARTESIAN_POINT('Ctrl Pts',(-7.36879696098183,20.8548878518499,4.01677584313272));
#9103=CARTESIAN_POINT('Ctrl Pts',(-6.10637108416454,20.9376219601132,5.76644257170316));
#9104=CARTESIAN_POINT('Ctrl Pts',(-5.28937860377834,20.9832860564796,6.52393732253735));
#9105=CARTESIAN_POINT('Ctrl Pts',(-3.43256215082987,21.0747868850767,7.66118487941332));
#9106=CARTESIAN_POINT('Ctrl Pts',(-2.41646683206916,21.1197342681174,8.03972422596952));
#9107=CARTESIAN_POINT('Ctrl Pts',(-0.30103886964946,21.2040887303464,8.38903981540581));
#9108=CARTESIAN_POINT('Ctrl Pts',(0.77805047538717,21.2413690487989,8.35830671932943));
#9109=CARTESIAN_POINT('Ctrl Pts',(2.89883696890837,21.3285727435666,7.88271403447874));
#9110=CARTESIAN_POINT('Ctrl Pts',(3.91705889205637,21.3751678727251,7.42946302233154));
#9111=CARTESIAN_POINT('Ctrl Pts',(5.68342520927749,21.4658085523941,6.17647466325817));
#9112=CARTESIAN_POINT('Ctrl Pts',(6.42420250024152,21.5090577158337,5.40186694088489));
#9113=CARTESIAN_POINT('Ctrl Pts',(7.59864239252401,21.5901331939427,3.57871690055576));
#9114=CARTESIAN_POINT('Ctrl Pts',(8.00651613636646,21.6320216270508,2.53827512105294));
#9115=CARTESIAN_POINT('Ctrl Pts',(8.38863518496435,21.722950323466,0.375211331472238));
#9116=CARTESIAN_POINT('Ctrl Pts',(8.36567998459492,21.7691937855692,-0.724854569873513));
#9117=CARTESIAN_POINT('Ctrl Pts',(7.90507099774516,21.8571908196599,-2.81817830084023));
#9118=CARTESIAN_POINT('Ctrl Pts',(7.48545823607019,21.8959733497179,-3.79471255741776));
#9119=CARTESIAN_POINT('Ctrl Pts',(6.27658819709621,21.9775203773607,-5.58066281390651));
#9120=CARTESIAN_POINT('Ctrl Pts',(5.48278798673984,22.0228461833929,-6.36223286723487));
#9121=CARTESIAN_POINT('Ctrl Pts',(4.04328783254457,22.0950557765146,-7.30447159027245));
#9122=CARTESIAN_POINT('Ctrl Pts',(3.49067741606164,22.1210511178399,-7.58410633998801));
#9123=CARTESIAN_POINT('Ctrl Pts',(2.34434684189784,22.1717792313269,-8.01210224550795));
#9124=CARTESIAN_POINT('Ctrl Pts',(1.75496663665873,22.1963755718445,-8.16148939163003));
#9125=CARTESIAN_POINT('Ctrl Pts',(1.15457232288581,22.22,-8.2455587288689));
#9126=CARTESIAN_POINT('',(-7.30706743901566,22.22,-3.99112032412919));
#9127=CARTESIAN_POINT('Origin',(0.,22.22,0.));
#9128=CARTESIAN_POINT('',(2.02140576001126E-13,21.8627746953453,-8.326));
#9129=CARTESIAN_POINT('Ctrl Pts',(-7.30706743901566,22.22,-3.99112032412919));
#9130=CARTESIAN_POINT('Ctrl Pts',(-6.80957791613765,22.1817118950886,-4.90193964267893));
#9131=CARTESIAN_POINT('Ctrl Pts',(-6.14607950438177,22.141467826149,-5.71189907139109));
#9132=CARTESIAN_POINT('Ctrl Pts',(-4.52911708821652,22.0540951363203,-7.06818095845697));
#9133=CARTESIAN_POINT('Ctrl Pts',(-3.58212247816543,22.0086069804025,-7.59213467174586));
#9134=CARTESIAN_POINT('Ctrl Pts',(-1.73288189728967,21.9287159657206,-8.19014224877633));
#9135=CARTESIAN_POINT('Ctrl Pts',(-0.868435929643723,21.8943901952037,-8.32600000000001));
#9136=CARTESIAN_POINT('Ctrl Pts',(3.16691117774326E-13,21.8627746953453,
-8.326));
#9137=CARTESIAN_POINT('',(-1.01964092497009E-15,24.9,-8.326));
#9138=CARTESIAN_POINT('',(-1.01964092497009E-15,-25.4,-8.326));
#9139=CARTESIAN_POINT('Origin',(0.,24.9,0.));
#9140=CARTESIAN_POINT('Ctrl Pts',(2.73392419813945E-13,21.8627746953453,
-8.326));
#9141=CARTESIAN_POINT('Ctrl Pts',(0.222420275737213,21.8546774621977,-8.326));
#9142=CARTESIAN_POINT('Ctrl Pts',(0.445088669140307,21.8463838731545,-8.31708769992091));
#9143=CARTESIAN_POINT('Ctrl Pts',(1.72956012537363,21.7974512311123,-8.21378222217217));
#9144=CARTESIAN_POINT('Ctrl Pts',(2.76535295574494,21.7536792163472,-7.92528063087028));
#9145=CARTESIAN_POINT('Ctrl Pts',(4.70935917599653,21.6625113677188,-6.9548924164029));
#9146=CARTESIAN_POINT('Ctrl Pts',(5.59165784984499,21.6159442735309,-6.26754925433765));
#9147=CARTESIAN_POINT('Ctrl Pts',(7.00684017904237,21.529824526478,-4.62138544212288));
#9148=CARTESIAN_POINT('Ctrl Pts',(7.53914569966282,21.4928809496688,-3.68975621000039));
#9149=CARTESIAN_POINT('Ctrl Pts',(8.2291331827155,21.4076770804388,-1.66287788083303));
#9150=CARTESIAN_POINT('Ctrl Pts',(8.37505267279169,21.3623615337414,-0.584885761396712));
#9151=CARTESIAN_POINT('Ctrl Pts',(8.24648416511102,21.2708521782396,1.59199107833957));
#9152=CARTESIAN_POINT('Ctrl Pts',(7.96327969214975,21.2255626695136,2.66936379163521));
#9153=CARTESIAN_POINT('Ctrl Pts',(7.0152084419188,21.144136245221,4.60638210209414));
#9154=CARTESIAN_POINT('Ctrl Pts',(6.37675301190161,21.1052415183809,5.45612438337728));
#9155=CARTESIAN_POINT('Ctrl Pts',(4.78959810321677,21.0171730787018,6.89713617786851));
#9156=CARTESIAN_POINT('Ctrl Pts',(3.84635314660346,20.9709125093812,7.46433370424951));
#9157=CARTESIAN_POINT('Ctrl Pts',(1.78044218858592,20.8800677193668,8.20820651339556));
#9158=CARTESIAN_POINT('Ctrl Pts',(0.676127188089457,20.8383517093461,8.37179460683603));
#9159=CARTESIAN_POINT('Ctrl Pts',(-1.48885324123266,20.7571943549324,8.26041566296981));
#9160=CARTESIAN_POINT('Ctrl Pts',(-2.52964769301862,20.7138984210511,8.00322770229722));
#9161=CARTESIAN_POINT('Ctrl Pts',(-4.49594281807084,20.6232085649402,7.09418652168197));
#9162=CARTESIAN_POINT('Ctrl Pts',(-5.39595620582177,20.5766138261025,6.43621089068518));
#9163=CARTESIAN_POINT('Ctrl Pts',(-6.86332004775605,20.4895022029757,4.83323748008094));
#9164=CARTESIAN_POINT('Ctrl Pts',(-7.4265465602687,20.4522662415181,3.9130188955332));
#9165=CARTESIAN_POINT('Ctrl Pts',(-8.17616169136161,20.3678381340514,1.9045948304856));
#9166=CARTESIAN_POINT('Ctrl Pts',(-8.35346386919154,20.3228574715675,0.834569128080672));
#9167=CARTESIAN_POINT('Ctrl Pts',(-8.29082102121212,20.2313519706046,-1.3422160176817));
#9168=CARTESIAN_POINT('Ctrl Pts',(-8.04024058237028,20.1857179501071,-2.42778417386124));
#9169=CARTESIAN_POINT('Ctrl Pts',(-7.15070000077872,20.1030946136455,-4.39327531494625));
#9170=CARTESIAN_POINT('Ctrl Pts',(-6.53768510268979,20.0651732446934,-5.26234377960467));
#9171=CARTESIAN_POINT('Ctrl Pts',(-4.99629403922793,19.9778244858738,-6.7483805201122));
#9172=CARTESIAN_POINT('Ctrl Pts',(-4.07364773146887,19.9317528080013,-7.34226903746486));
#9173=CARTESIAN_POINT('Ctrl Pts',(-2.0873033090925,19.8429221520908,-8.12812838292694));
#9174=CARTESIAN_POINT('Ctrl Pts',(-1.04801299029565,19.8009277166739,-8.32599999999998));
#9175=CARTESIAN_POINT('Ctrl Pts',(-1.4432899320127E-13,19.7627746953453,
-8.326));
#9176=CARTESIAN_POINT('Origin',(0.,-25.4,0.));
#9177=CARTESIAN_POINT('',(-5.25515247417893E-14,17.6627746953453,-8.326));
#9178=CARTESIAN_POINT('',(2.16625517025532E-13,18.0637230794129,-8.326));
#9179=CARTESIAN_POINT('',(-1.01964092497009E-15,-25.4,-8.326));
#9180=CARTESIAN_POINT('Ctrl Pts',(2.52020626589911E-13,18.0637230794129,
-8.326));
#9181=CARTESIAN_POINT('Ctrl Pts',(-0.890419891838311,18.0961389076892,-8.326));
#9182=CARTESIAN_POINT('Ctrl Pts',(-1.77639189334566,18.1313947631273,-8.1831756499706));
#9183=CARTESIAN_POINT('Ctrl Pts',(-3.66112836545653,18.2131638963057,-7.55729324801004));
#9184=CARTESIAN_POINT('Ctrl Pts',(-4.62037689809789,18.2595459254736,-7.01203601590485));
#9185=CARTESIAN_POINT('Ctrl Pts',(-6.24408054969564,18.3481770243168,-5.60755878566216));
#9186=CARTESIAN_POINT('Ctrl Pts',(-6.90299349539498,18.3880811030606,-4.77298598603335));
#9187=CARTESIAN_POINT('Ctrl Pts',(-7.89718765749648,18.46854217343,-2.85893206632874));
#9188=CARTESIAN_POINT('Ctrl Pts',(-8.20603261947695,18.5135288767537,-1.78876266097571));
#9189=CARTESIAN_POINT('Ctrl Pts',(-8.38685799405134,18.604981436681,0.386763093180027));
#9190=CARTESIAN_POINT('Ctrl Pts',(-8.26601443080375,18.6505352226678,1.47042258496924));
#9191=CARTESIAN_POINT('Ctrl Pts',(-7.62326100457352,18.7363397578568,3.51158989920655));
#9192=CARTESIAN_POINT('Ctrl Pts',(-7.11494212544351,18.7732834184323,4.45229486945681));
#9193=CARTESIAN_POINT('Ctrl Pts',(-5.7408036723115,18.8586081423939,6.13172383316992));
#9194=CARTESIAN_POINT('Ctrl Pts',(-4.87297955135116,18.9051237215524,6.84168671833937));
#9195=CARTESIAN_POINT('Ctrl Pts',(-2.94767213755927,18.9966100831954,7.85961615483011));
#9196=CARTESIAN_POINT('Ctrl Pts',(-1.91643098526058,19.0407291195881,8.17251178137013));
#9197=CARTESIAN_POINT('Ctrl Pts',(0.226566935638505,19.1233906949082,8.39353207965677));
#9198=CARTESIAN_POINT('Ctrl Pts',(1.31869908885409,19.1624366089017,8.29240327023542));
#9199=CARTESIAN_POINT('Ctrl Pts',(3.41208572998068,19.2516557666824,7.67346267722576));
#9200=CARTESIAN_POINT('Ctrl Pts',(4.39178998104064,19.2981569649045,7.15796606561161));
#9201=CARTESIAN_POINT('Ctrl Pts',(6.06368536035962,19.387512273397,5.80250353034279));
#9202=CARTESIAN_POINT('Ctrl Pts',(6.74982179139679,19.4290584529639,4.98762194233357));
#9203=CARTESIAN_POINT('Ctrl Pts',(7.8040409043102,19.5082348491522,3.10412858614996));
#9204=CARTESIAN_POINT('Ctrl Pts',(8.14610250630801,19.5527862684777,2.04431396528135));
#9205=CARTESIAN_POINT('Ctrl Pts',(8.39522393183261,19.6440847731824,-0.127547035208562));
#9206=CARTESIAN_POINT('Ctrl Pts',(8.30742204212602,19.6899135850502,-1.21774899981201));
#9207=CARTESIAN_POINT('Ctrl Pts',(7.72647180284449,19.7764844822775,-3.27714697213884));
#9208=CARTESIAN_POINT('Ctrl Pts',(7.24888972111259,19.8137313904644,-4.22984071149828));
#9209=CARTESIAN_POINT('Ctrl Pts',(5.92803207045448,19.898005531026,-5.9515709756581));
#9210=CARTESIAN_POINT('Ctrl Pts',(5.079672161943,19.9444159902647,-6.69024556027974));
#9211=CARTESIAN_POINT('Ctrl Pts',(3.1801110567652,20.0362414234368,-7.7689009659777));
#9212=CARTESIAN_POINT('Ctrl Pts',(2.15556595890407,20.0807750999972,-8.11312189350259));
#9213=CARTESIAN_POINT('Ctrl Pts',(0.730483570767718,20.1366251233243,-8.30199133068642));
#9214=CARTESIAN_POINT('Ctrl Pts',(0.365066982180118,20.1504327781605,-8.326));
#9215=CARTESIAN_POINT('Ctrl Pts',(2.43693953905222E-13,20.1637230794129,
-8.326));
#9216=CARTESIAN_POINT('Ctrl Pts',(-1.69645946028209E-13,19.7627746953453,
-8.326));
#9217=CARTESIAN_POINT('Ctrl Pts',(0.0537760328361958,19.7608169733068,-8.32600000000001));
#9218=CARTESIAN_POINT('Ctrl Pts',(0.107574246419283,19.7588474932951,-8.32547900742368));
#9219=CARTESIAN_POINT('Ctrl Pts',(1.22032386865729,19.717884294939,-8.30390594916758));
#9220=CARTESIAN_POINT('Ctrl Pts',(2.26557642210438,19.675157325493,-8.08150934929497));
#9221=CARTESIAN_POINT('Ctrl Pts',(4.25439689276674,19.5850888690087,-7.24104763054406));
#9222=CARTESIAN_POINT('Ctrl Pts',(5.17296265458766,19.5385136547805,-6.61613457917031));
#9223=CARTESIAN_POINT('Ctrl Pts',(6.69769916516932,19.4503382758645,-5.06192308448468));
#9224=CARTESIAN_POINT('Ctrl Pts',(7.29556680177744,19.4124020752022,-4.15413589911575));
#9225=CARTESIAN_POINT('Ctrl Pts',(8.11027653410421,19.3288434821876,-2.16639634071711));
#9226=CARTESIAN_POINT('Ctrl Pts',(8.32142803602603,19.2842710064197,-1.10608081716402));
#9227=CARTESIAN_POINT('Ctrl Pts',(8.33060510978089,19.1924165715265,1.07900496832259));
#9228=CARTESIAN_POINT('Ctrl Pts',(8.11166964648995,19.1460188118018,2.18274138966102));
#9229=CARTESIAN_POINT('Ctrl Pts',(7.27482662402643,19.0618495981043,4.18500674179216));
#9230=CARTESIAN_POINT('Ctrl Pts',(6.68601371437469,19.0245541532904,5.07293964281488));
#9231=CARTESIAN_POINT('Ctrl Pts',(5.18838404047147,18.9379083407741,6.60132915675086));
#9232=CARTESIAN_POINT('Ctrl Pts',(4.28597903871517,18.8920544918981,7.21991296322557));
#9233=CARTESIAN_POINT('Ctrl Pts',(2.27756009335754,18.8007762125735,8.08398904216306));
#9234=CARTESIAN_POINT('Ctrl Pts',(1.18800422662706,18.7562704237527,8.3142811960007));
#9235=CARTESIAN_POINT('Ctrl Pts',(-0.970574421465393,18.6772229603539,8.33636576399424));
#9236=CARTESIAN_POINT('Ctrl Pts',(-2.01903107640799,18.6354936260255,8.14625193122687));
#9237=CARTESIAN_POINT('Ctrl Pts',(-4.02696397192928,18.5460671966126,7.36943971707767));
#9238=CARTESIAN_POINT('Ctrl Pts',(-4.96163230319053,18.4995567041815,6.77549641229619));
#9239=CARTESIAN_POINT('Ctrl Pts',(-6.53890596645596,18.4104340420465,5.26721290630533));
#9240=CARTESIAN_POINT('Ctrl Pts',(-7.16916082099009,18.3715093575615,4.37078513603769));
#9241=CARTESIAN_POINT('Ctrl Pts',(-8.04313227967416,18.2887628323817,2.40236351133255));
#9242=CARTESIAN_POINT('Ctrl Pts',(-8.28466633463081,18.2445995564128,1.35178226642655));
#9243=CARTESIAN_POINT('Ctrl Pts',(-8.35906795948745,18.1530746958544,-0.825463416455813));
#9244=CARTESIAN_POINT('Ctrl Pts',(-8.17458512402766,18.1065678943966,-1.93179378485013));
#9245=CARTESIAN_POINT('Ctrl Pts',(-7.40071930074816,18.0213496277566,-3.95901460783598));
#9246=CARTESIAN_POINT('Ctrl Pts',(-6.83757202508643,17.9843906714201,-4.86745290900539));
#9247=CARTESIAN_POINT('Ctrl Pts',(-5.38647179191651,17.898507096619,-6.44016868567395));
#9248=CARTESIAN_POINT('Ctrl Pts',(-4.50612444658721,17.8529234024623,-7.0841042841063));
#9249=CARTESIAN_POINT('Ctrl Pts',(-2.52840988388469,17.7614823987188,-8.00910387674011));
#9250=CARTESIAN_POINT('Ctrl Pts',(-1.44636514008738,17.7165379978424,-8.27327358554525));
#9251=CARTESIAN_POINT('Ctrl Pts',(-0.229460356638047,17.6711780304915,-8.32363031929139));
#9252=CARTESIAN_POINT('Ctrl Pts',(-0.114688347109808,17.6669499364864,-8.326));
#9253=CARTESIAN_POINT('Ctrl Pts',(-9.72832925327793E-14,17.6627746953453,
-8.326));
#9254=CARTESIAN_POINT('Origin',(0.,-25.4,0.));
#9255=CARTESIAN_POINT('',(-1.73496445486892E-13,15.5627746953453,-8.326));
#9256=CARTESIAN_POINT('',(-8.53327934765894E-14,15.9637230794129,-8.326));
#9257=CARTESIAN_POINT('',(-1.01964092497009E-15,-25.4,-8.326));
#9258=CARTESIAN_POINT('Ctrl Pts',(-1.01030295240889E-13,15.9637230794129,
-8.326));
#9259=CARTESIAN_POINT('Ctrl Pts',(-1.06766019611996,16.0025913593021,-8.32599999999998));
#9260=CARTESIAN_POINT('Ctrl Pts',(-2.12593713442031,16.0454344607786,-8.12063706622244));
#9261=CARTESIAN_POINT('Ctrl Pts',(-4.12404446198688,16.1351306644149,-7.31397138239622));
#9262=CARTESIAN_POINT('Ctrl Pts',(-5.04197560981409,16.1811543292689,-6.7142002907157));
#9263=CARTESIAN_POINT('Ctrl Pts',(-6.57307250804579,16.268338992533,-5.21814073069542));
#9264=CARTESIAN_POINT('Ctrl Pts',(-7.18038549971979,16.3060862262824,-4.34466982618623));
#9265=CARTESIAN_POINT('Ctrl Pts',(-8.05663598620786,16.3889768494034,-2.37282031731172));
#9266=CARTESIAN_POINT('Ctrl Pts',(-8.29980195235844,16.4346829044047,-1.28553856319385));
#9267=CARTESIAN_POINT('Ctrl Pts',(-8.34754816142187,16.5261758537262,0.89094799695044));
#9268=CARTESIAN_POINT('Ctrl Pts',(-8.16319350057409,16.5710755391503,1.95904737078116));
#9269=CARTESIAN_POINT('Ctrl Pts',(-7.40008811787804,16.6553253882446,3.96323092380682));
#9270=CARTESIAN_POINT('Ctrl Pts',(-6.82976049081476,16.6926735547414,4.88087307410312));
#9271=CARTESIAN_POINT('Ctrl Pts',(-5.35053928533847,16.7800074091779,6.47388205937465));
#9272=CARTESIAN_POINT('Ctrl Pts',(-4.4466108738051,16.8266024358327,7.12509036378162));
#9273=CARTESIAN_POINT('Ctrl Pts',(-2.47548792401173,16.9171721477538,8.02005338937477));
#9274=CARTESIAN_POINT('Ctrl Pts',(-1.43368173786436,16.9603544152598,8.27008105335408));
#9275=CARTESIAN_POINT('Ctrl Pts',(0.734035591731605,17.0413133397641,8.36727881874682));
#9276=CARTESIAN_POINT('Ctrl Pts',(1.83997710111426,17.0834518014106,8.19544045616635));
#9277=CARTESIAN_POINT('Ctrl Pts',(3.90203516139383,17.1744991125026,7.43525885814066));
#9278=CARTESIAN_POINT('Ctrl Pts',(4.84033335378641,17.220717531209,6.86149869059172));
#9279=CARTESIAN_POINT('Ctrl Pts',(6.41637397647712,17.3086126976293,5.40948023465566));
#9280=CARTESIAN_POINT('Ctrl Pts',(7.0486350625867,17.3472412213165,4.55507985860513));
#9281=CARTESIAN_POINT('Ctrl Pts',(7.98257278257802,17.428959582952,2.6111167758123));
#9282=CARTESIAN_POINT('Ctrl Pts',(8.25790602060779,17.4743363547778,1.5316681980353));
#9283=CARTESIAN_POINT('Ctrl Pts',(8.37051137781878,17.5658525086914,-0.645370366206906));
#9284=CARTESIAN_POINT('Ctrl Pts',(8.21696717253769,17.6110904807199,-1.7215170950898));
#9285=CARTESIAN_POINT('Ctrl Pts',(7.51254948138263,17.6961083691393,-3.74397120645815));
#9286=CARTESIAN_POINT('Ctrl Pts',(6.97282744523094,17.7330925721754,-4.67283653177338));
#9287=CARTESIAN_POINT('Ctrl Pts',(5.54505326333423,17.8194536431009,-6.3086721157136));
#9288=CARTESIAN_POINT('Ctrl Pts',(4.65840815242837,17.8660313162708,-6.98899034570502));
#9289=CARTESIAN_POINT('Ctrl Pts',(2.70886925636158,17.95709134306,-7.94466582950618));
#9290=CARTESIAN_POINT('Ctrl Pts',(1.67178820401725,18.000752057619,-8.22564080909474));
#9291=CARTESIAN_POINT('Ctrl Pts',(0.40662470803591,18.0487635135138,-8.31856125006016));
#9292=CARTESIAN_POINT('Ctrl Pts',(0.203202195754393,18.0563254824552,-8.326));
#9293=CARTESIAN_POINT('Ctrl Pts',(2.88657986402541E-13,18.0637230794129,
-8.326));
#9294=CARTESIAN_POINT('Ctrl Pts',(-1.62647673107585E-13,17.6627746953453,
-8.32600000000001));
#9295=CARTESIAN_POINT('Ctrl Pts',(0.937428171083856,17.6286475258,-8.32600000000003));
#9296=CARTESIAN_POINT('Ctrl Pts',(1.86902802054237,17.5914051457875,-8.16769223739126));
#9297=CARTESIAN_POINT('Ctrl Pts',(3.78693416571463,17.5074465822747,-7.49509455465147));
#9298=CARTESIAN_POINT('Ctrl Pts',(4.7372426102813,17.4610503279071,-6.93367584142013));
#9299=CARTESIAN_POINT('Ctrl Pts',(6.36854294282441,17.3709826643249,-5.47400880272639));
#9300=CARTESIAN_POINT('Ctrl Pts',(7.03283715715672,17.3306964041795,-4.58933185072455));
#9301=CARTESIAN_POINT('Ctrl Pts',(7.96749087277855,17.2488016572187,-2.64117281302412));
#9302=CARTESIAN_POINT('Ctrl Pts',(8.23964999089758,17.2050932528527,-1.60141231373512));
#9303=CARTESIAN_POINT('Ctrl Pts',(8.38017383007285,17.1139867134581,0.565882106262566));
#9304=CARTESIAN_POINT('Ctrl Pts',(8.23080475600197,17.067413244654,1.67379839558519));
#9305=CARTESIAN_POINT('Ctrl Pts',(7.52151860508346,16.9811548538322,3.72576228696615));
#9306=CARTESIAN_POINT('Ctrl Pts',(6.98435774174966,16.9441902237068,4.65545852901487));
#9307=CARTESIAN_POINT('Ctrl Pts',(5.58036455598891,16.8590930472698,6.27235151787872));
#9308=CARTESIAN_POINT('Ctrl Pts',(4.72285823283805,16.8138217755528,6.94098476017238));
#9309=CARTESIAN_POINT('Ctrl Pts',(2.77783410889142,16.7223079121988,7.92607230575084));
#9310=CARTESIAN_POINT('Ctrl Pts',(1.70442017914298,16.6769679903503,8.22400878079362));
#9311=CARTESIAN_POINT('Ctrl Pts',(-0.446522969877771,16.5953737458763,8.38048698816194));
#9312=CARTESIAN_POINT('Ctrl Pts',(-1.50218431899096,16.5566342895529,8.25685945638442));
#9313=CARTESIAN_POINT('Ctrl Pts',(-3.54600325216184,16.4686652785713,7.61154348763457));
#9314=CARTESIAN_POINT('Ctrl Pts',(-4.51068510061488,16.4224286312543,7.08261388765972));
#9315=CARTESIAN_POINT('Ctrl Pts',(-6.19486653546212,16.3314671777391,5.67201563359183));
#9316=CARTESIAN_POINT('Ctrl Pts',(-6.89326576259661,16.2895104354326,4.79900506276053));
#9317=CARTESIAN_POINT('Ctrl Pts',(-7.88714772594216,16.2084670496717,2.87109869177676));
#9318=CARTESIAN_POINT('Ctrl Pts',(-8.18867382432303,16.1652362687781,1.84270017257802));
#9319=CARTESIAN_POINT('Ctrl Pts',(-8.39297278532252,16.0746150173042,-0.313049941056341));
#9320=CARTESIAN_POINT('Ctrl Pts',(-8.27765322129032,16.0280198395401,-1.42148265552545));
#9321=CARTESIAN_POINT('Ctrl Pts',(-7.631489900257,15.9407801999068,-3.49678905434423));
#9322=CARTESIAN_POINT('Ctrl Pts',(-7.11949600278651,15.9034817484166,-4.44746066470012));
#9323=CARTESIAN_POINT('Ctrl Pts',(-5.76095076674326,15.8191561169798,-6.10636390487672));
#9324=CARTESIAN_POINT('Ctrl Pts',(-4.92591855586582,15.774221829667,-6.79789069632792));
#9325=CARTESIAN_POINT('Ctrl Pts',(-3.01387150876772,15.6827230275315,-7.83937964475539));
#9326=CARTESIAN_POINT('Ctrl Pts',(-1.9497251141762,15.6370472783281,-8.16934566758503));
#9327=CARTESIAN_POINT('Ctrl Pts',(-0.568555311775885,15.5837786856521,-8.31145683949874));
#9328=CARTESIAN_POINT('Ctrl Pts',(-0.284127003756134,15.57311836831,-8.326));
#9329=CARTESIAN_POINT('Ctrl Pts',(-1.89154247820511E-13,15.5627746953453,
-8.326));
#9330=CARTESIAN_POINT('Origin',(0.,-25.4,0.));
#9331=CARTESIAN_POINT('',(-1.11957170745022E-14,13.4627746953453,-8.326));
#9332=CARTESIAN_POINT('',(-5.82414177429932E-14,13.863723079413,-8.32600000000001));
#9333=CARTESIAN_POINT('',(-1.01964092497009E-15,-25.4,-8.326));
#9334=CARTESIAN_POINT('Ctrl Pts',(-1.4582085539061E-13,13.863723079413,
-8.326));
#9335=CARTESIAN_POINT('Ctrl Pts',(-0.135836828135204,13.8686682331935,-8.326));
#9336=CARTESIAN_POINT('Ctrl Pts',(-0.271785053719794,13.8736873117228,-8.32267581772396));
#9337=CARTESIAN_POINT('Ctrl Pts',(-1.50950589218815,13.9200221532606,-8.26199182042639));
#9338=CARTESIAN_POINT('Ctrl Pts',(-2.58954375088037,13.9650672888594,-7.98955341437777));
#9339=CARTESIAN_POINT('Ctrl Pts',(-4.55944747076069,14.0565344481263,-7.0497806400479));
#9340=CARTESIAN_POINT('Ctrl Pts',(-5.43428128731425,14.1020456522445,-6.39974419856835));
#9341=CARTESIAN_POINT('Ctrl Pts',(-6.87391755623469,14.1877391807443,-4.81621411339271));
#9342=CARTESIAN_POINT('Ctrl Pts',(-7.43074385164979,14.2246674325236,-3.90264947429375));
#9343=CARTESIAN_POINT('Ctrl Pts',(-8.1889707434789,14.3101409425543,-1.8693567756763));
#9344=CARTESIAN_POINT('Ctrl Pts',(-8.36492764659033,14.3566680587784,-0.762543148013781));
#9345=CARTESIAN_POINT('Ctrl Pts',(-8.27443805711982,14.4480989999331,1.41246832642682));
#9346=CARTESIAN_POINT('Ctrl Pts',(-8.02543631461458,14.4921553401998,2.46050572374258));
#9347=CARTESIAN_POINT('Ctrl Pts',(-7.1367614153721,14.5746973638872,4.42406255008773));
#9348=CARTESIAN_POINT('Ctrl Pts',(-6.49834127821936,14.6139194508751,5.31765719475317));
#9349=CARTESIAN_POINT('Ctrl Pts',(-4.90799537658902,14.7032735693802,6.81431095251126));
#9350=CARTESIAN_POINT('Ctrl Pts',(-3.96945604358268,14.7497608912359,7.40044709581961));
#9351=CARTESIAN_POINT('Ctrl Pts',(-1.95701469491134,14.8390158062621,8.16129027556823));
#9352=CARTESIAN_POINT('Ctrl Pts',(-0.907781491932131,14.8803102780559,8.34336195724052));
#9353=CARTESIAN_POINT('Ctrl Pts',(1.25002532406152,14.959667796113,8.30518902206611));
#9354=CARTESIAN_POINT('Ctrl Pts',(2.33788033733056,15.0042827301164,8.06675808767319));
#9355=CARTESIAN_POINT('Ctrl Pts',(4.33911191421371,15.0956082046261,7.18798770930206));
#9356=CARTESIAN_POINT('Ctrl Pts',(5.23629522702819,15.141401066234,6.56326127224253));
#9357=CARTESIAN_POINT('Ctrl Pts',(6.72280797819924,15.2278661186725,5.02421673135485));
#9358=CARTESIAN_POINT('Ctrl Pts',(7.30548506957144,15.2650502817789,4.13142775172451));
#9359=CARTESIAN_POINT('Ctrl Pts',(8.12735299824442,15.3494719846849,2.12315604202303));
#9360=CARTESIAN_POINT('Ctrl Pts',(8.33808083599502,15.3958996429541,1.01870837702462));
#9361=CARTESIAN_POINT('Ctrl Pts',(8.31333421448786,15.4876828292901,-1.16468250707291));
#9362=CARTESIAN_POINT('Ctrl Pts',(8.09491472867419,15.5321611558964,-2.22275835656821));
#9363=CARTESIAN_POINT('Ctrl Pts',(7.26610606428713,15.6155283161931,-4.20594400408292));
#9364=CARTESIAN_POINT('Ctrl Pts',(6.66060813053494,15.6536692230037,-5.11103507158764));
#9365=CARTESIAN_POINT('Ctrl Pts',(5.12339638574204,15.7420719450369,-6.6544551627523));
#9366=CARTESIAN_POINT('Ctrl Pts',(4.2009289386824,15.7886358811958,-7.27207371873985));
#9367=CARTESIAN_POINT('Ctrl Pts',(2.20749238849329,15.8785557742899,-8.09747193158456));
#9368=CARTESIAN_POINT('Ctrl Pts',(1.16141776831797,15.9211526735467,-8.31225630215715));
#9369=CARTESIAN_POINT('Ctrl Pts',(0.0687215117795646,15.9612167961274,-8.32578735205743));
#9370=CARTESIAN_POINT('Ctrl Pts',(0.0343560586356681,15.9624723435442,-8.326));
#9371=CARTESIAN_POINT('Ctrl Pts',(-1.69645946028209E-13,15.9637230794129,
-8.326));
#9372=CARTESIAN_POINT('Ctrl Pts',(-1.55153667691366E-13,15.5627746953453,
-8.326));
#9373=CARTESIAN_POINT('Ctrl Pts',(0.766473007452974,15.5348711662173,-8.32600000000002));
#9374=CARTESIAN_POINT('Ctrl Pts',(1.53059056240928,15.5048290963712,-8.22017457936218));
#9375=CARTESIAN_POINT('Ctrl Pts',(3.315932973231,15.4291964951735,-7.71409527197532));
#9376=CARTESIAN_POINT('Ctrl Pts',(4.29316118863751,15.3831522201064,-7.21604913902925));
#9377=CARTESIAN_POINT('Ctrl Pts',(6.01417786317076,15.2920486182911,-5.86248838162399));
#9378=CARTESIAN_POINT('Ctrl Pts',(6.73696230357398,15.2485957082345,-5.01513072376378));
#9379=CARTESIAN_POINT('Ctrl Pts',(7.78880263202565,15.169221526306,-3.12693232737676));
#9380=CARTESIAN_POINT('Ctrl Pts',(8.12286538336693,15.1265692379339,-2.11229531884364));
#9381=CARTESIAN_POINT('Ctrl Pts',(8.39826316592157,15.036585808248,0.0282819256256184));
#9382=CARTESIAN_POINT('Ctrl Pts',(8.3211193271742,14.9900167842913,1.13609247837785));
#9383=CARTESIAN_POINT('Ctrl Pts',(7.74647417120216,14.9017102095279,3.23677973975202));
#9384=CARTESIAN_POINT('Ctrl Pts',(7.2627833257141,14.8636583216416,4.21146930995301));
#9385=CARTESIAN_POINT('Ctrl Pts',(5.9550395739323,14.7802099460948,5.91662597317146));
#9386=CARTESIAN_POINT('Ctrl Pts',(5.14556445242495,14.7356914964966,6.6326345715706));
#9387=CARTESIAN_POINT('Ctrl Pts',(3.26313744592203,14.643877584444,7.74041896476706));
#9388=CARTESIAN_POINT('Ctrl Pts',(2.19981065428884,14.5974622874687,8.10699015155958));
#9389=CARTESIAN_POINT('Ctrl Pts',(0.0486893857144464,14.5131473062414,8.39260472799874));
#9390=CARTESIAN_POINT('Ctrl Pts',(-1.01534262136813,14.4759184106797,8.33110828659527));
#9391=CARTESIAN_POINT('Ctrl Pts',(-3.08990218717426,14.3893767506368,7.80694593494561));
#9392=CARTESIAN_POINT('Ctrl Pts',(-4.07838391792978,14.3435578020054,7.33911185036683));
#9393=CARTESIAN_POINT('Ctrl Pts',(-5.83618716670347,14.2522516602417,6.0396310365248));
#9394=CARTESIAN_POINT('Ctrl Pts',(-6.58398529979185,14.2076825850543,5.21438613963775));
#9395=CARTESIAN_POINT('Ctrl Pts',(-7.69022007882209,14.1284560366258,3.36106816935293));
#9396=CARTESIAN_POINT('Ctrl Pts',(-8.05404936263119,14.0869802088156,2.35995744330347));
#9397=CARTESIAN_POINT('Ctrl Pts',(-8.39456826427114,13.9976526424611,0.234982250540276));
#9398=CARTESIAN_POINT('Ctrl Pts',(-8.35255602044774,13.9511551906314,-0.871125703558243));
#9399=CARTESIAN_POINT('Ctrl Pts',(-7.84456729604378,13.8618985928561,-2.9944126552092));
#9400=CARTESIAN_POINT('Ctrl Pts',(-7.38713856607453,13.8228045832374,-3.99170590989937));
#9401=CARTESIAN_POINT('Ctrl Pts',(-6.12610103946332,13.7401760861308,-5.73875265446514));
#9402=CARTESIAN_POINT('Ctrl Pts',(-5.34046520368155,13.6960743460471,-6.47622625885644));
#9403=CARTESIAN_POINT('Ctrl Pts',(-3.49787283183606,13.6046031740294,-7.63669967157466));
#9404=CARTESIAN_POINT('Ctrl Pts',(-2.44973670994727,13.5580843076334,-8.03450940729452));
#9405=CARTESIAN_POINT('Ctrl Pts',(-0.905737253757057,13.4965243087677,-8.28907276263488));
#9406=CARTESIAN_POINT('Ctrl Pts',(-0.452759042309395,13.4792574351185,-8.32599999999999));
#9407=CARTESIAN_POINT('Ctrl Pts',(-1.12271303365219E-13,13.4627746953453,
-8.326));
#9408=CARTESIAN_POINT('Origin',(0.,-25.4,0.));
#9409=CARTESIAN_POINT('',(1.23965221987824E-14,11.3627746953453,-8.326));
#9410=CARTESIAN_POINT('',(-1.7738222607308E-13,11.763723079413,-8.32600000000001));
#9411=CARTESIAN_POINT('',(-1.01964092497009E-15,-25.4,-8.326));
#9412=CARTESIAN_POINT('Ctrl Pts',(-2.02754479872169E-13,11.763723079413,
-8.326));
#9413=CARTESIAN_POINT('Ctrl Pts',(-0.303252472074516,11.7747630170303,-8.326));
#9414=CARTESIAN_POINT('Ctrl Pts',(-0.606820499119774,11.7861626527411,-8.30943314966895));
#9415=CARTESIAN_POINT('Ctrl Pts',(-2.006123196559,11.8403360153408,-8.15568270533984));
#9416=CARTESIAN_POINT('Ctrl Pts',(-3.0679903265585,11.8860833591555,-7.81836261337937));
#9417=CARTESIAN_POINT('Ctrl Pts',(-4.97219018423794,11.9775669309886,-6.76400654845765));
#9418=CARTESIAN_POINT('Ctrl Pts',(-5.80194903063939,12.0224181649271,-6.06729746404484));
#9419=CARTESIAN_POINT('Ctrl Pts',(-7.14994139612737,12.1065628343985,-4.39872576918177));
#9420=CARTESIAN_POINT('Ctrl Pts',(-7.65607384812685,12.1439849020982,-3.44311446949431));
#9421=CARTESIAN_POINT('Ctrl Pts',(-8.28746475539839,12.2314488778649,-1.36247143454109));
#9422=CARTESIAN_POINT('Ctrl Pts',(-8.39486154416642,12.2780430273218,-0.254063182030855));
#9423=CARTESIAN_POINT('Ctrl Pts',(-8.17577182323232,12.3685400772549,1.89873235437619));
#9424=CARTESIAN_POINT('Ctrl Pts',(-7.86745931090753,12.4116545474063,2.92436400717674));
#9425=CARTESIAN_POINT('Ctrl Pts',(-6.85972962789788,12.4924959910119,4.84746646277679));
#9426=CARTESIAN_POINT('Ctrl Pts',(-6.1532288151958,12.5348918593769,5.71771214982715));
#9427=CARTESIAN_POINT('Ctrl Pts',(-4.45667115926648,12.6260577404462,7.11660023911833));
#9428=CARTESIAN_POINT('Ctrl Pts',(-3.48876230026754,12.6722501006202,7.63783343714226));
#9429=CARTESIAN_POINT('Ctrl Pts',(-1.44092546537248,12.7600423327032,8.26777956105381));
#9430=CARTESIAN_POINT('Ctrl Pts',(-0.384296819897299,12.7985224076212,8.38358291612028));
#9431=CARTESIAN_POINT('Ctrl Pts',(1.76555131698124,12.8804130475961,8.21110644099873));
#9432=CARTESIAN_POINT('Ctrl Pts',(2.83675341664969,12.9258403501148,7.90518164125101));
#9433=CARTESIAN_POINT('Ctrl Pts',(4.77373411316413,13.0173582017968,6.90597271744218));
#9434=CARTESIAN_POINT('Ctrl Pts',(5.62570972681814,13.0625491659331,6.23158081053345));
#9435=CARTESIAN_POINT('Ctrl Pts',(7.01844275423167,13.1474563783671,4.60422259982182));
#9436=CARTESIAN_POINT('Ctrl Pts',(7.54937778889659,13.1844736122372,3.66937446773204));
#9437=CARTESIAN_POINT('Ctrl Pts',(8.24309946706272,13.2709773220947,1.61157478694954));
#9438=CARTESIAN_POINT('Ctrl Pts',(8.38404516506843,13.3175601021255,0.503436996845469));
#9439=CARTESIAN_POINT('Ctrl Pts',(8.22771272001427,13.408553899823,-1.66117545923843));
#9440=CARTESIAN_POINT('Ctrl Pts',(7.94825830436621,13.4521475008907,-2.69820495206495));
#9441=CARTESIAN_POINT('Ctrl Pts',(6.9989919870918,13.5338340516951,-4.6414113006288));
#9442=CARTESIAN_POINT('Ctrl Pts',(6.32636525605991,13.5745011148047,-5.52323132314027));
#9443=CARTESIAN_POINT('Ctrl Pts',(4.68202887376216,13.6647920808336,-6.97094335373384));
#9444=CARTESIAN_POINT('Ctrl Pts',(3.728089952798,13.7111534209451,-7.52441277683913));
#9445=CARTESIAN_POINT('Ctrl Pts',(1.82619866592454,13.7940649276322,-8.17493303565393));
#9446=CARTESIAN_POINT('Ctrl Pts',(0.915744931208586,13.8303852904585,-8.32600000000003));
#9447=CARTESIAN_POINT('Ctrl Pts',(-1.52655665885959E-13,13.863723079413,
-8.32600000000001));
#9448=CARTESIAN_POINT('Ctrl Pts',(-1.28785870856518E-13,13.4627746953453,
-8.326));
#9449=CARTESIAN_POINT('Ctrl Pts',(0.602475208085855,13.4408415230689,-8.32600000000002));
#9450=CARTESIAN_POINT('Ctrl Pts',(1.20446106602682,13.4175518737411,-8.26061511824214));
#9451=CARTESIAN_POINT('Ctrl Pts',(2.85005435699202,13.3500058164016,-7.89721788731316));
#9452=CARTESIAN_POINT('Ctrl Pts',(3.84936152349472,13.3044637551861,-7.46130751960217));
#9453=CARTESIAN_POINT('Ctrl Pts',(5.64444722471778,13.2130069623409,-6.21923425961092));
#9454=CARTESIAN_POINT('Ctrl Pts',(6.41781466084013,13.1680039634893,-5.41763184652892));
#9455=CARTESIAN_POINT('Ctrl Pts',(7.58056217918825,13.087492624649,-3.60107015505294));
#9456=CARTESIAN_POINT('Ctrl Pts',(7.97507616633824,13.0476459325469,-2.61367977412177));
#9457=CARTESIAN_POINT('Ctrl Pts',(8.38213775996806,12.9590437430625,-0.505960260844928));
#9458=CARTESIAN_POINT('Ctrl Pts',(8.37612732733517,12.9126673606885,0.597267623858461));
#9459=CARTESIAN_POINT('Ctrl Pts',(7.93743142281672,12.8224701255431,2.74293099477509));
#9460=CARTESIAN_POINT('Ctrl Pts',(7.50726802011452,12.7819657713616,3.76391307165841));
#9461=CARTESIAN_POINT('Ctrl Pts',(6.2941538258584,12.700191484644,5.55332457302669));
#9462=CARTESIAN_POINT('Ctrl Pts',(5.53325443955575,12.6565493400172,6.31177672600054));
#9463=CARTESIAN_POINT('Ctrl Pts',(3.7325000233972,12.56550754908,7.52428687864775));
#9464=CARTESIAN_POINT('Ctrl Pts',(2.70065483388178,12.5189283691453,7.95318288278388));
#9465=CARTESIAN_POINT('Ctrl Pts',(0.570533848588451,12.4325276141087,8.37440617533124));
#9466=CARTESIAN_POINT('Ctrl Pts',(-0.503966248242079,12.3955349082409,8.37867533336922));
#9467=CARTESIAN_POINT('Ctrl Pts',(-2.6082270937139,12.3105477467568,7.97991570715822));
#9468=CARTESIAN_POINT('Ctrl Pts',(-3.61732900654454,12.2653227648794,7.57605606670174));
#9469=CARTESIAN_POINT('Ctrl Pts',(-5.44772472808909,12.1738059650236,6.39228659380338));
#9470=CARTESIAN_POINT('Ctrl Pts',(-6.24582818079019,12.1284150581469,5.61507266269158));
#9471=CARTESIAN_POINT('Ctrl Pts',(-7.4645333267061,12.0466487516106,3.83572464787945));
#9472=CARTESIAN_POINT('Ctrl Pts',(-7.88950950913947,12.0080621878062,2.86146760637413));
#9473=CARTESIAN_POINT('Ctrl Pts',(-8.36145215618212,11.9201956169881,0.771247410285937));
#9474=CARTESIAN_POINT('Ctrl Pts',(-8.39053311634181,11.8739843619691,-0.328052330537919));
#9475=CARTESIAN_POINT('Ctrl Pts',(-8.02048208966464,11.7829039823986,-2.49472444569266));
#9476=CARTESIAN_POINT('Ctrl Pts',(-7.61737029272528,11.7406944885028,-3.53932837946436));
#9477=CARTESIAN_POINT('Ctrl Pts',(-6.45112885884589,11.6597682299118,-5.36957912797074));
#9478=CARTESIAN_POINT('Ctrl Pts',(-5.71463194672094,11.6166047768032,-6.14752283130325));
#9479=CARTESIAN_POINT('Ctrl Pts',(-3.95561993247836,11.5260551556824,-7.40891691123526));
#9480=CARTESIAN_POINT('Ctrl Pts',(-2.94033701199002,11.4794602953578,-7.86724563496573));
#9481=CARTESIAN_POINT('Ctrl Pts',(-1.25207829660374,11.409842157908,-8.25532783449594));
#9482=CARTESIAN_POINT('Ctrl Pts',(-0.626361873301063,11.38557746414,-8.326));
#9483=CARTESIAN_POINT('Ctrl Pts',(2.84772205816353E-13,11.3627746953453,
-8.326));
#9484=CARTESIAN_POINT('Origin',(0.,-25.4,0.));
#9485=CARTESIAN_POINT('',(1.94473098237308E-13,9.26277469534531,-8.326));
#9486=CARTESIAN_POINT('',(1.71062558676527E-15,9.66372307941294,-8.326));
#9487=CARTESIAN_POINT('',(-1.01964092497009E-15,-25.4,-8.326));
#9488=CARTESIAN_POINT('Ctrl Pts',(-1.72223346694977E-13,9.66372307941295,
-8.326));
#9489=CARTESIAN_POINT('Ctrl Pts',(-0.474199948109406,9.68098637757983,-8.326));
#9490=CARTESIAN_POINT('Ctrl Pts',(-0.948564287601614,9.69910706346753,-8.28549267616555));
#9491=CARTESIAN_POINT('Ctrl Pts',(-2.51093903145465,9.76166088539588,-8.01547299083435));
#9492=CARTESIAN_POINT('Ctrl Pts',(-3.55519873590362,9.80819853902353,-7.61005526035746));
#9493=CARTESIAN_POINT('Ctrl Pts',(-5.3877587457154,9.8995729445105,-6.43680916193083));
#9494=CARTESIAN_POINT('Ctrl Pts',(-6.16743606182152,9.94356643510009,-5.6941653003555));
#9495=CARTESIAN_POINT('Ctrl Pts',(-7.41688487727091,10.0259895644163,-3.93681713196663));
#9496=CARTESIAN_POINT('Ctrl Pts',(-7.86775284239254,10.0653932510665,-2.93384043089224));
#9497=CARTESIAN_POINT('Ctrl Pts',(-8.35906861457206,10.1548806124347,-0.805063943029334));
#9498=CARTESIAN_POINT('Ctrl Pts',(-8.39236780364888,10.2013532156509,0.300452898050963));
#9499=CARTESIAN_POINT('Ctrl Pts',(-8.03573869924169,10.2905079433405,2.42131650589003));
#9500=CARTESIAN_POINT('Ctrl Pts',(-7.66452791394732,10.331559107744,3.41908188803614));
#9501=CARTESIAN_POINT('Ctrl Pts',(-6.54469345955934,10.4110963696274,5.26362738806832));
#9502=CARTESIAN_POINT('Ctrl Pts',(-5.79069118709908,10.4557736515338,6.0832745668736));
#9503=CARTESIAN_POINT('Ctrl Pts',(-4.02377198376237,10.5471242117649,7.36907938802327));
#9504=CARTESIAN_POINT('Ctrl Pts',(-3.03260117434181,10.5928804912406,7.82927423235415));
#9505=CARTESIAN_POINT('Ctrl Pts',(-0.954371183257477,10.6792397998651,8.33840346145337));
#9506=CARTESIAN_POINT('Ctrl Pts',(0.110819689456831,10.7163680467929,8.39210534172936));
#9507=CARTESIAN_POINT('Ctrl Pts',(2.25961469410576,10.8009363753522,8.09040801577519));
#9508=CARTESIAN_POINT('Ctrl Pts',(3.31939921095577,10.8473803507535,7.71633699151253));
#9509=CARTESIAN_POINT('Ctrl Pts',(5.19245858238359,10.9391198505578,6.5958677005875));
#9510=CARTESIAN_POINT('Ctrl Pts',(5.99630069783449,10.983542260661,5.87467173427252));
#9511=CARTESIAN_POINT('Ctrl Pts',(7.2929547143924,11.0667971103334,4.15951449438082));
#9512=CARTESIAN_POINT('Ctrl Pts',(7.77043385499936,11.1050663529639,3.17950258404369));
#9513=CARTESIAN_POINT('Ctrl Pts',(8.32933089730255,11.1936012981371,1.07338271686461));
#9514=CARTESIAN_POINT('Ctrl Pts',(8.39813326278913,11.2401574660181,-0.0341220082125714));
#9515=CARTESIAN_POINT('Ctrl Pts',(8.10725762469965,11.3299882681282,-2.17106846069599));
#9516=CARTESIAN_POINT('Ctrl Pts',(7.76614069422855,11.3725080725837,-3.18255386611217));
#9517=CARTESIAN_POINT('Ctrl Pts',(6.70139780907636,11.4515366532656,-5.06253090256127));
#9518=CARTESIAN_POINT('Ctrl Pts',(5.97271674059568,11.4953938433415,-5.90471045661073));
#9519=CARTESIAN_POINT('Ctrl Pts',(4.24285960338634,11.5865535444329,-7.24562812676891));
#9520=CARTESIAN_POINT('Ctrl Pts',(3.2628970493093,11.6325481260211,-7.73657397246758));
#9521=CARTESIAN_POINT('Ctrl Pts',(1.49306607867275,11.7072519314285,-8.22533043235189));
#9522=CARTESIAN_POINT('Ctrl Pts',(0.747569406382801,11.7365077378375,-8.32600000000001));
#9523=CARTESIAN_POINT('Ctrl Pts',(-1.68060010352633E-13,11.763723079413,
-8.326));
#9524=CARTESIAN_POINT('Ctrl Pts',(3.17246229286638E-13,11.3627746953453,
-8.326));
#9525=CARTESIAN_POINT('Ctrl Pts',(0.43974300939449,11.3467658055969,-8.326));
#9526=CARTESIAN_POINT('Ctrl Pts',(0.879750206370908,11.330015125447,-8.29116531842167));
#9527=CARTESIAN_POINT('Ctrl Pts',(2.37622328087344,11.270501412391,-8.05164028759308));
#9528=CARTESIAN_POINT('Ctrl Pts',(3.39370126759801,11.2256151617867,-7.67840429886385));
#9529=CARTESIAN_POINT('Ctrl Pts',(5.25588865827407,11.1341246763999,-6.55095157941137));
#9530=CARTESIAN_POINT('Ctrl Pts',(6.07676516332524,11.0884070404113,-5.79763689437981));
#9531=CARTESIAN_POINT('Ctrl Pts',(7.34829876630346,11.0054727971358,-4.05422335819444));
#9532=CARTESIAN_POINT('Ctrl Pts',(7.8021809619017,10.9677524572588,-3.09198527340771));
#9533=CARTESIAN_POINT('Ctrl Pts',(8.33451523277333,10.88059469251,-1.01862656112783));
#9534=CARTESIAN_POINT('Ctrl Pts',(8.39618247397769,10.834579066331,0.0760194490623026));
#9535=CARTESIAN_POINT('Ctrl Pts',(8.09341281379174,10.7434423052017,2.24403280095633));
#9536=CARTESIAN_POINT('Ctrl Pts',(7.72529352344289,10.6997560888879,3.2951318423501));
#9537=CARTESIAN_POINT('Ctrl Pts',(6.62387520353467,10.6205825087671,5.15427208379822));
#9538=CARTESIAN_POINT('Ctrl Pts',(5.91584121845181,10.5780070403487,5.95354039130136));
#9539=CARTESIAN_POINT('Ctrl Pts',(4.20606760973629,10.4881118368888,7.2690825687462));
#9540=CARTESIAN_POINT('Ctrl Pts',(3.21067803326855,10.4415499806909,7.76029733300199));
#9541=CARTESIAN_POINT('Ctrl Pts',(1.10594381595948,10.3531103177683,8.32249720930198));
#9542=CARTESIAN_POINT('Ctrl Pts',(0.0191197917106355,10.3149342484212,8.39562891452947));
#9543=CARTESIAN_POINT('Ctrl Pts',(-2.1132777072148,10.2315983927577,8.12416781458325));
#9544=CARTESIAN_POINT('Ctrl Pts',(-3.13907909322553,10.1871356018457,7.7854953785785));
#9545=CARTESIAN_POINT('Ctrl Pts',(-5.04334369665254,10.0953644533491,6.71756938058307));
#9546=CARTESIAN_POINT('Ctrl Pts',(-5.89522363595378,10.0489321566374,5.9839527035621));
#9547=CARTESIAN_POINT('Ctrl Pts',(-7.22556881879485,9.96446947296532,4.26968498468107));
#9548=CARTESIAN_POINT('Ctrl Pts',(-7.70859384852291,9.92730158568948,3.31914539716159));
#9549=CARTESIAN_POINT('Ctrl Pts',(-8.30059192471654,9.84086603030577,1.26296701394893));
#9550=CARTESIAN_POINT('Ctrl Pts',(-8.39431687163808,9.79508330663404,0.173861421689487));
#9551=CARTESIAN_POINT('Ctrl Pts',(-8.15739166509317,9.70375064862286,-1.99881203717135));
#9552=CARTESIAN_POINT('Ctrl Pts',(-7.82123735923041,9.65911821207469,-3.06055394202927));
#9553=CARTESIAN_POINT('Ctrl Pts',(-6.77772150535337,9.57971043425691,-4.94955153663381));
#9554=CARTESIAN_POINT('Ctrl Pts',(-6.0964918257955,9.53848464817047,-5.76794177750132));
#9555=CARTESIAN_POINT('Ctrl Pts',(-4.43324056799386,9.44925769153702,-7.13226975569284));
#9556=CARTESIAN_POINT('Ctrl Pts',(-3.45714963380328,9.40277439015981,-7.65317333496234));
#9557=CARTESIAN_POINT('Ctrl Pts',(-1.62582185353653,9.32447410626235,-8.20652436697391));
#9558=CARTESIAN_POINT('Ctrl Pts',(-0.814402088748981,9.29242308763611,-8.32600000000001));
#9559=CARTESIAN_POINT('Ctrl Pts',(2.66453525910038E-13,9.26277469534532,
-8.32600000000001));
#9560=CARTESIAN_POINT('Origin',(0.,-25.4,0.));
#9561=CARTESIAN_POINT('',(1.6837414297283E-14,7.16277469534533,-8.326));
#9562=CARTESIAN_POINT('',(5.38911077441476E-14,7.56372307941295,-8.326));
#9563=CARTESIAN_POINT('',(-1.01964092497009E-15,-25.4,-8.326));
#9564=CARTESIAN_POINT('Ctrl Pts',(2.52159404467989E-13,7.56372307941294,
-8.326));
#9565=CARTESIAN_POINT('Ctrl Pts',(-0.646166079188242,7.58724682237162,-8.326));
#9566=CARTESIAN_POINT('Ctrl Pts',(-1.29151752362468,7.61232174378504,-8.25078837229487));
#9567=CARTESIAN_POINT('Ctrl Pts',(-2.99553195348629,7.68285860964985,-7.84628539769874));
#9568=CARTESIAN_POINT('Ctrl Pts',(-4.00685913034017,7.7294511525345,-7.38121538218405));
#9569=CARTESIAN_POINT('Ctrl Pts',(-5.7560065685614,7.81987582713428,-6.10867995386882));
#9570=CARTESIAN_POINT('Ctrl Pts',(-6.48677428614185,7.86292342757756,-5.32632493330393));
#9571=CARTESIAN_POINT('Ctrl Pts',(-7.64205544266831,7.94364960845092,-3.48660955371491));
#9572=CARTESIAN_POINT('Ctrl Pts',(-8.03877974932396,7.98630322303686,-2.43642206911082));
#9573=CARTESIAN_POINT('Ctrl Pts',(-8.39265713520717,8.07758446765967,-0.264971661311598));
#9574=CARTESIAN_POINT('Ctrl Pts',(-8.35539629462834,8.12375047093282,0.833251605123153));
#9575=CARTESIAN_POINT('Ctrl Pts',(-7.86831170863093,8.21144146718116,2.91929513301856));
#9576=CARTESIAN_POINT('Ctrl Pts',(-7.43614052398183,8.24978250879786,3.89052068008099));
#9577=CARTESIAN_POINT('Ctrl Pts',(-6.20425617670594,8.33184176118451,5.66097917510394));
#9578=CARTESIAN_POINT('Ctrl Pts',(-5.40041701443523,8.37731781705428,6.43230971163402));
#9579=CARTESIAN_POINT('Ctrl Pts',(-3.56194700431721,8.46883564977609,7.60214324730046));
#9580=CARTESIAN_POINT('Ctrl Pts',(-2.55067534908799,8.51397971436136,7.99839497011445));
#9581=CARTESIAN_POINT('Ctrl Pts',(-0.443025731472404,8.59877788690376,8.38229351692315));
#9582=CARTESIAN_POINT('Ctrl Pts',(0.632825873132995,8.63583414320664,8.37010532378516));
#9583=CARTESIAN_POINT('Ctrl Pts',(2.76020839296628,8.72247757178746,7.93259315604519));
#9584=CARTESIAN_POINT('Ctrl Pts',(3.78803083251719,8.76906451810793,7.49636004213978));
#9585=CARTESIAN_POINT('Ctrl Pts',(5.57857788868775,8.85999159475243,6.27162800167303));
#9586=CARTESIAN_POINT('Ctrl Pts',(6.33348554769889,8.90351846461245,5.50828231665004));
#9587=CARTESIAN_POINT('Ctrl Pts',(7.53505857253065,8.98508509467007,3.70876063403948));
#9588=CARTESIAN_POINT('Ctrl Pts',(7.95859913789034,9.02597976931485,2.68200228536735));
#9589=CARTESIAN_POINT('Ctrl Pts',(8.38047241067967,9.11639797448044,0.531082353341697));
#9590=CARTESIAN_POINT('Ctrl Pts',(8.37782841188649,9.16273798161244,-0.571280216318487));
#9591=CARTESIAN_POINT('Ctrl Pts',(7.95477284015797,9.25116138123764,-2.67474657425873));
#9592=CARTESIAN_POINT('Ctrl Pts',(7.55280247544499,9.29066662359165,-3.65887733459845));
#9593=CARTESIAN_POINT('Ctrl Pts',(6.37633864427922,9.37148720986523,-5.46639478469158));
#9594=CARTESIAN_POINT('Ctrl Pts',(5.59685221872653,9.41658919703079,-6.26210837834233));
#9595=CARTESIAN_POINT('Ctrl Pts',(3.79296005377837,9.50806897776786,-7.49002209394443));
#9596=CARTESIAN_POINT('Ctrl Pts',(2.79116570028853,9.5535372772894,-7.91811515677167));
#9597=CARTESIAN_POINT('Ctrl Pts',(1.1637569824839,9.62007369357247,-8.26497315555356));
#9598=CARTESIAN_POINT('Ctrl Pts',(0.582049594485062,9.64253350371268,-8.32600000000002));
#9599=CARTESIAN_POINT('Ctrl Pts',(-2.13024042849952E-13,9.66372307941295,
-8.326));
#9600=CARTESIAN_POINT('Ctrl Pts',(2.65829025458686E-13,9.26277469534532,
-8.326));
#9601=CARTESIAN_POINT('Ctrl Pts',(0.270011332909717,9.25294490483806,-8.326));
#9602=CARTESIAN_POINT('Ctrl Pts',(0.540330328713359,9.24282785542697,-8.31286592986294));
#9603=CARTESIAN_POINT('Ctrl Pts',(1.8722686141496,9.19160195337279,-8.18266865276879));
#9604=CARTESIAN_POINT('Ctrl Pts',(2.90463882928701,9.14756312398022,-7.8755446403364));
#9605=CARTESIAN_POINT('Ctrl Pts',(4.83447661738027,9.05614783747807,-6.86884359444069));
#9606=CARTESIAN_POINT('Ctrl Pts',(5.70577910102292,9.00961768353316,-6.16421198346843));
#9607=CARTESIAN_POINT('Ctrl Pts',(7.08966225860657,8.92410304413962,-4.49262570933537));
#9608=CARTESIAN_POINT('Ctrl Pts',(7.60365014163406,8.88717781687242,-3.55408682810106));
#9609=CARTESIAN_POINT('Ctrl Pts',(8.25764608625664,8.80151508631727,-1.51629284352452));
#9610=CARTESIAN_POINT('Ctrl Pts',(8.38447345847686,8.75601581466154,-0.43393016979451));
#9611=CARTESIAN_POINT('Ctrl Pts',(8.21608442769125,8.66454493988926,1.74203126836012));
#9612=CARTESIAN_POINT('Ctrl Pts',(7.91332388916238,8.61948379405422,2.8139715547111));
#9613=CARTESIAN_POINT('Ctrl Pts',(6.93008815760916,8.53879162550238,4.73352297003514));
#9614=CARTESIAN_POINT('Ctrl Pts',(6.27607052332773,8.49914701973004,5.5716960307008));
#9615=CARTESIAN_POINT('Ctrl Pts',(4.66108897497509,8.41064917972435,6.98494031216529));
#9616=CARTESIAN_POINT('Ctrl Pts',(3.70562210090701,8.36429372470061,7.53548324720289));
#9617=CARTESIAN_POINT('Ctrl Pts',(1.63032274656187,8.27396701813399,8.23844594669925));
#9618=CARTESIAN_POINT('Ctrl Pts',(0.530057311503819,8.23323680801519,8.38144266320653));
#9619=CARTESIAN_POINT('Ctrl Pts',(-1.62792472637798,8.15158384599891,8.23436255608475));
#9620=CARTESIAN_POINT('Ctrl Pts',(-2.66594668201158,8.10800889182977,7.95909750311635));
#9621=CARTESIAN_POINT('Ctrl Pts',(-4.61960871021218,8.01703365213557,7.01459742138488));
#9622=CARTESIAN_POINT('Ctrl Pts',(-5.50951373087223,7.97044961766743,6.33962286832511));
#9623=CARTESIAN_POINT('Ctrl Pts',(-6.94681990713011,7.88390665710639,4.7116433937412));
#9624=CARTESIAN_POINT('Ctrl Pts',(-7.49217320594941,7.84687913003538,3.78486720922831));
#9625=CARTESIAN_POINT('Ctrl Pts',(-8.20749596222921,7.76200248643653,1.76577311036096));
#9626=CARTESIAN_POINT('Ctrl Pts',(-8.36678981857217,7.716824612001,0.691056017360496));
#9627=CARTESIAN_POINT('Ctrl Pts',(-8.26624484813637,7.62530659708561,-1.48602681745564));
#9628=CARTESIAN_POINT('Ctrl Pts',(-7.99687043893497,7.57986552404543,-2.56700502926336));
#9629=CARTESIAN_POINT('Ctrl Pts',(-7.07362642223966,7.497927502703,-4.51619350268564));
#9630=CARTESIAN_POINT('Ctrl Pts',(-6.44602993909129,7.45948712400998,-5.37412175554442));
#9631=CARTESIAN_POINT('Ctrl Pts',(-4.87837176501689,7.3717232907501,-6.83441058184061));
#9632=CARTESIAN_POINT('Ctrl Pts',(-3.94382848183897,7.3255382517794,-7.4130863304762));
#9633=CARTESIAN_POINT('Ctrl Pts',(-1.98841059853127,7.2389325423352,-8.14665541703044));
#9634=CARTESIAN_POINT('Ctrl Pts',(-0.997760808690797,7.19909828080406,-8.32600000000001));
#9635=CARTESIAN_POINT('Ctrl Pts',(2.78110867668602E-13,7.16277469534532,
-8.32600000000001));
#9636=CARTESIAN_POINT('Origin',(0.,-25.4,0.));
#9637=CARTESIAN_POINT('',(-1.48126560903206E-15,5.06277469534534,-8.32600000000001));
#9638=CARTESIAN_POINT('',(2.12097888753232E-13,5.46372307941294,-8.326));
#9639=CARTESIAN_POINT('',(-1.01964092497009E-15,-25.4,-8.326));
#9640=CARTESIAN_POINT('Ctrl Pts',(2.66869859544272E-13,5.46372307941295,
-8.32600000000001));
#9641=CARTESIAN_POINT('Ctrl Pts',(-0.836238710997287,5.49416643619563,-8.32600000000001));
#9642=CARTESIAN_POINT('Ctrl Pts',(-1.6691076352286,5.52713480092555,-8.20003069430066));
#9643=CARTESIAN_POINT('Ctrl Pts',(-3.51605227828332,5.60643469280897,-7.6261703701439));
#9644=CARTESIAN_POINT('Ctrl Pts',(-4.48736206739596,5.65289217823176,-7.09821385403226));
#9645=CARTESIAN_POINT('Ctrl Pts',(-6.13926504489025,5.74194958478934,-5.72229678595137));
#9646=CARTESIAN_POINT('Ctrl Pts',(-6.81406939673126,5.78277185299237,-4.89928546051299));
#9647=CARTESIAN_POINT('Ctrl Pts',(-7.8434923195373,5.86248277281707,-3.0030765506242));
#9648=CARTESIAN_POINT('Ctrl Pts',(-8.1718573836664,5.90721963796853,-1.93885043847795));
#9649=CARTESIAN_POINT('Ctrl Pts',(-8.39273444303584,5.99859283259092,0.234787328453905));
#9650=CARTESIAN_POINT('Ctrl Pts',(-8.29123071882295,6.0443129058275,1.32240255636142));
#9651=CARTESIAN_POINT('Ctrl Pts',(-7.68470419092934,6.13056937921356,3.37432083468098));
#9652=CARTESIAN_POINT('Ctrl Pts',(-7.19448788927728,6.16764968623736,4.3220352924857));
#9653=CARTESIAN_POINT('Ctrl Pts',(-5.8516413287853,6.25235984893773,6.02642433519535));
#9654=CARTESIAN_POINT('Ctrl Pts',(-4.99515856122614,6.29881886716971,6.75334001340205));
#9655=CARTESIAN_POINT('Ctrl Pts',(-3.08477432069922,6.39051447046153,7.80707226401682));
#9656=CARTESIAN_POINT('Ctrl Pts',(-2.05735958893951,6.43488191143801,8.13841382570729));
#9657=CARTESIAN_POINT('Ctrl Pts',(0.0780813666116063,6.51802730695115,8.39554195436847));
#9658=CARTESIAN_POINT('Ctrl Pts',(1.16639161912466,6.55642742029657,8.31449901901567));
#9659=CARTESIAN_POINT('Ctrl Pts',(3.26797984233654,6.64509040181786,7.73622526022656));
#9660=CARTESIAN_POINT('Ctrl Pts',(4.25898323384728,6.69163818482159,7.23808296314459));
#9661=CARTESIAN_POINT('Ctrl Pts',(5.95801836496231,6.7813807989042,5.91120096349971));
#9662=CARTESIAN_POINT('Ctrl Pts',(6.65988782344491,6.82382491694228,5.10750465853079));
#9663=CARTESIAN_POINT('Ctrl Pts',(7.74794429048108,6.90265681557172,3.2414772381525));
#9664=CARTESIAN_POINT('Ctrl Pts',(8.10874982004316,6.94674901219425,2.18793166761265));
#9665=CARTESIAN_POINT('Ctrl Pts',(8.39641154396656,7.03793848012301,0.0186644962552045));
#9666=CARTESIAN_POINT('Ctrl Pts',(8.32736417643051,7.08390407115339,-1.07479124922758));
#9667=CARTESIAN_POINT('Ctrl Pts',(7.78132089306779,7.17089779552674,-3.14424767531945));
#9668=CARTESIAN_POINT('Ctrl Pts',(7.32079618340722,7.20846408878987,-4.10378319334718));
#9669=CARTESIAN_POINT('Ctrl Pts',(6.03717307551937,7.2916631814244,-5.83885786857691));
#9670=CARTESIAN_POINT('Ctrl Pts',(5.21116882224519,7.33745006928877,-6.58658583954571));
#9671=CARTESIAN_POINT('Ctrl Pts',(3.34192411406301,7.42892306594443,-7.70098286265292));
#9672=CARTESIAN_POINT('Ctrl Pts',(2.32265069959541,7.47372640841552,-8.06716454721469));
#9673=CARTESIAN_POINT('Ctrl Pts',(0.843407827322808,7.53234586696614,-8.29398708937408));
#9674=CARTESIAN_POINT('Ctrl Pts',(0.421555332686322,7.54837631391661,-8.326));
#9675=CARTESIAN_POINT('Ctrl Pts',(3.47361028829596E-13,7.56372307941294,
-8.326));
#9676=CARTESIAN_POINT('Ctrl Pts',(3.17176840347599E-13,7.16277469534532,
-8.326));
#9677=CARTESIAN_POINT('Ctrl Pts',(0.110531407005316,7.15875078803883,-8.326));
#9678=CARTESIAN_POINT('Ctrl Pts',(0.221146764566538,7.15467756251844,-8.32379898692281));
#9679=CARTESIAN_POINT('Ctrl Pts',(1.39221484264702,7.11106308580878,-8.27709620822705));
#9680=CARTESIAN_POINT('Ctrl Pts',(2.43474869707119,7.0679673551769,-8.03244607989538));
#9681=CARTESIAN_POINT('Ctrl Pts',(4.40943191700961,6.97749051763201,-7.14806832054697));
#9682=CARTESIAN_POINT('Ctrl Pts',(5.31626753571269,6.9308967450319,-6.50195511100492));
#9683=CARTESIAN_POINT('Ctrl Pts',(6.80437648512559,6.84339711469949,-4.91645300631127));
#9684=CARTESIAN_POINT('Ctrl Pts',(7.38004618128376,6.80595372948799,-4.00073896649165));
#9685=CARTESIAN_POINT('Ctrl Pts',(8.15325004613083,6.72183798589981,-1.99974559187804));
#9686=CARTESIAN_POINT('Ctrl Pts',(8.34287163849979,6.67700016300087,-0.933117839145429));
#9687=CARTESIAN_POINT('Ctrl Pts',(8.30627021956783,6.58551942388972,1.24307825753891));
#9688=CARTESIAN_POINT('Ctrl Pts',(8.06866161818484,6.5397608817083,2.33160860668945));
#9689=CARTESIAN_POINT('Ctrl Pts',(7.20237143688086,6.45667104581957,4.30819710271847));
#9690=CARTESIAN_POINT('Ctrl Pts',(6.59931472806746,6.41904313295165,5.18497119551834));
#9691=CARTESIAN_POINT('Ctrl Pts',(5.07590919889841,6.33198158776267,6.68849499128344));
#9692=CARTESIAN_POINT('Ctrl Pts',(4.16151989849957,6.28599510059205,7.29263193471018));
#9693=CARTESIAN_POINT('Ctrl Pts',(2.1363687615072,6.19482687975152,8.12249073939595));
#9694=CARTESIAN_POINT('Ctrl Pts',(1.04292815878845,6.15090401440863,8.33367950045313));
#9695=CARTESIAN_POINT('Ctrl Pts',(-1.11743517016165,6.07193069835686,8.31821380931037));
#9696=CARTESIAN_POINT('Ctrl Pts',(-2.16408733753655,6.02943213951944,8.10910853602593));
#9697=CARTESIAN_POINT('Ctrl Pts',(-4.16089487781268,5.93962602065705,7.2949621021605));
#9698=CARTESIAN_POINT('Ctrl Pts',(-5.08623646770629,5.89307213146327,6.68279971348423));
#9699=CARTESIAN_POINT('Ctrl Pts',(-6.63273819124001,5.80450107051947,5.14746125310297));
#9700=CARTESIAN_POINT('Ctrl Pts',(-7.24394210984032,5.76619557337075,4.24437780125603));
#9701=CARTESIAN_POINT('Ctrl Pts',(-8.08323842736825,5.68297152755918,2.26459664289444));
#9702=CARTESIAN_POINT('Ctrl Pts',(-8.30704860044801,5.63856454044485,1.208217857998));
#9703=CARTESIAN_POINT('Ctrl Pts',(-8.3433565962951,5.54683726336699,-0.97384302471674));
#9704=CARTESIAN_POINT('Ctrl Pts',(-8.13873009131252,5.50038896906575,-2.07878159143743));
#9705=CARTESIAN_POINT('Ctrl Pts',(-7.32800466069326,5.41578061817603,-4.09149339003265));
#9706=CARTESIAN_POINT('Ctrl Pts',(-6.74987920718193,5.37866651333336,-4.98790357997048));
#9707=CARTESIAN_POINT('Ctrl Pts',(-5.27161683067499,5.29233616772912,-6.53482922266064));
#9708=CARTESIAN_POINT('Ctrl Pts',(-4.37832878617842,5.24659002303265,-7.16407980518596));
#9709=CARTESIAN_POINT('Ctrl Pts',(-2.38249229096588,5.15523291310326,-8.05369986200487));
#9710=CARTESIAN_POINT('Ctrl Pts',(-1.29593786950077,5.11053874562274,-8.29815318994175));
#9711=CARTESIAN_POINT('Ctrl Pts',(-0.128827677076796,5.06748038441164,-8.32525284116874));
#9712=CARTESIAN_POINT('Ctrl Pts',(-0.0643990695313742,5.06511915013371,
-8.326));
#9713=CARTESIAN_POINT('Ctrl Pts',(2.80624040585213E-13,5.06277469534533,
-8.326));
#9714=CARTESIAN_POINT('Origin',(0.,-25.4,0.));
#9715=CARTESIAN_POINT('',(-1.87582400111824E-13,2.96277469534536,-8.326));
#9716=CARTESIAN_POINT('',(-8.53327934765894E-14,3.36372307941297,-8.326));
#9717=CARTESIAN_POINT('',(-1.01964092497009E-15,-25.4,-8.326));
#9718=CARTESIAN_POINT('Ctrl Pts',(-1.18793863634892E-13,3.36372307941297,
-8.32599999999999));
#9719=CARTESIAN_POINT('Ctrl Pts',(-1.01836376702856,3.40079671770132,-8.32599999999997));
#9720=CARTESIAN_POINT('Ctrl Pts',(-2.02901965751839,3.44151663238114,-8.13917015344795));
#9721=CARTESIAN_POINT('Ctrl Pts',(-3.99734367168246,3.52904090918155,-7.38425233093585));
#9722=CARTESIAN_POINT('Ctrl Pts',(-4.92702575069337,3.57518100252677,-6.79929511414191));
#9723=CARTESIAN_POINT('Ctrl Pts',(-6.48389859140411,3.66277504659142,-5.3284036272797));
#9724=CARTESIAN_POINT('Ctrl Pts',(-7.10550172745547,3.70098935641988,-4.46591707897539));
#9725=CARTESIAN_POINT('Ctrl Pts',(-8.01494287944838,3.78320932991601,-2.51002136660578));
#9726=CARTESIAN_POINT('Ctrl Pts',(-8.27662251212905,3.82873120460592,-1.42712099898192));
#9727=CARTESIAN_POINT('Ctrl Pts',(-8.36162443406572,3.92024745868604,0.749919948078396));
#9728=CARTESIAN_POINT('Ctrl Pts',(-8.19493445769682,3.96534599110138,1.82274960776392));
#9729=CARTESIAN_POINT('Ctrl Pts',(-7.46555349515448,4.05003955738955,3.83748855894897));
#9730=CARTESIAN_POINT('Ctrl Pts',(-6.91290358877263,4.08713924640636,4.76157456578563));
#9731=CARTESIAN_POINT('Ctrl Pts',(-5.46329019484257,4.17391595682806,6.37935846457562));
#9732=CARTESIAN_POINT('Ctrl Pts',(-4.56921462651943,4.22050609686749,7.04739990282447));
#9733=CARTESIAN_POINT('Ctrl Pts',(-2.61031192483623,4.311367800571,7.97742115377031));
#9734=CARTESIAN_POINT('Ctrl Pts',(-1.57111891415557,4.35483008732094,8.24529748599969));
#9735=CARTESIAN_POINT('Ctrl Pts',(0.589739027879327,4.43628138737034,8.37780188080297));
#9736=CARTESIAN_POINT('Ctrl Pts',(1.69164942547461,4.47740058732764,8.22642886267737));
#9737=CARTESIAN_POINT('Ctrl Pts',(3.76316894793577,4.56794020341399,7.50678967567851));
#9738=CARTESIAN_POINT('Ctrl Pts',(4.71368626587519,4.61425885797127,6.94942471900162));
#9739=CARTESIAN_POINT('Ctrl Pts',(6.31733377238988,4.70258257366624,5.52483363842384));
#9740=CARTESIAN_POINT('Ctrl Pts',(6.96500296712227,4.74190739602998,4.6819639424229));
#9741=CARTESIAN_POINT('Ctrl Pts',(7.93395357776352,4.82289919832966,2.75528466828652));
#9742=CARTESIAN_POINT('Ctrl Pts',(8.22877510544623,4.86805504852651,1.68109150046035));
#9743=CARTESIAN_POINT('Ctrl Pts',(8.38097082524413,4.95954527861263,-0.49533037295973));
#9744=CARTESIAN_POINT('Ctrl Pts',(8.2463670677231,5.00497152327706,-1.57595583889112));
#9745=CARTESIAN_POINT('Ctrl Pts',(7.57773447837673,5.090448545739,-3.60933209322709));
#9746=CARTESIAN_POINT('Ctrl Pts',(7.05632880145078,5.12736695766995,-4.54505674397575));
#9747=CARTESIAN_POINT('Ctrl Pts',(5.6597358437157,5.21312822444436,-6.20636282462398));
#9748=CARTESIAN_POINT('Ctrl Pts',(4.78393547707342,5.25967520081863,-6.90400423683939));
#9749=CARTESIAN_POINT('Ctrl Pts',(2.84827344830574,5.35099353959103,-7.89600490598302));
#9750=CARTESIAN_POINT('Ctrl Pts',(1.81447574080089,5.39492571590364,-8.19558218028575));
#9751=CARTESIAN_POINT('Ctrl Pts',(0.501719643319216,5.44521990738753,-8.31467585461312));
#9752=CARTESIAN_POINT('Ctrl Pts',(0.250717041383125,5.45459569958473,-8.326));
#9753=CARTESIAN_POINT('Ctrl Pts',(2.86368151414251E-13,5.46372307941295,
-8.326));
#9754=CARTESIAN_POINT('Ctrl Pts',(2.80886425230165E-13,5.06277469534533,
-8.326));
#9755=CARTESIAN_POINT('Ctrl Pts',(0.98938994559301,5.02675585202358,-8.326));
#9756=CARTESIAN_POINT('Ctrl Pts',(1.97154206318376,4.98729387796089,-8.14964939102314));
#9757=CARTESIAN_POINT('Ctrl Pts',(3.92683794662508,4.90083922264985,-7.42305571857651));
#9758=CARTESIAN_POINT('Ctrl Pts',(4.86819512279073,4.85437079776511,-6.84269928667721));
#9759=CARTESIAN_POINT('Ctrl Pts',(6.46817564592858,4.76484721600004,-5.35467060515037));
#9760=CARTESIAN_POINT('Ctrl Pts',(7.112642278346,4.72539283222041,-4.46316745034782));
#9761=CARTESIAN_POINT('Ctrl Pts',(8.01214487047178,4.6430021741349,-2.50321139543531));
#9762=CARTESIAN_POINT('Ctrl Pts',(8.26662695749645,4.59902593358394,-1.45707945592931));
#9763=CARTESIAN_POINT('Ctrl Pts',(8.3689375242085,4.50766721207635,0.716214016276809));
#9764=CARTESIAN_POINT('Ctrl Pts',(8.19925236532742,4.46112684145986,1.82334294699955));
#9765=CARTESIAN_POINT('Ctrl Pts',(7.45254564987965,4.37546667437354,3.86107595031696));
#9766=CARTESIAN_POINT('Ctrl Pts',(6.90036360677415,4.33854782460159,4.77842564798735));
#9767=CARTESIAN_POINT('Ctrl Pts',(5.46914904938857,4.25299445984832,6.3698739748369));
#9768=CARTESIAN_POINT('Ctrl Pts',(4.5983844945359,4.20753797265641,7.02435530931477));
#9769=CARTESIAN_POINT('Ctrl Pts',(2.63427890012778,4.11605506929538,7.97491979056402));
#9770=CARTESIAN_POINT('Ctrl Pts',(1.55575398765627,4.07093777131744,8.25341197616064));
#9771=CARTESIAN_POINT('Ctrl Pts',(-0.597677104968653,3.9900687341678,8.37107764632682));
#9772=CARTESIAN_POINT('Ctrl Pts',(-1.65108899359419,3.95061517335544,8.22839756708033));
#9773=CARTESIAN_POINT('Ctrl Pts',(-3.68494463374718,3.86221993194998,7.54554584284826));
#9774=CARTESIAN_POINT('Ctrl Pts',(-4.64149569507564,3.81588587958301,6.9978990524894));
#9775=CARTESIAN_POINT('Ctrl Pts',(-6.29534005757804,3.72543324975436,5.55896382499089));
#9776=CARTESIAN_POINT('Ctrl Pts',(-6.9740746221251,3.68447564688011,4.67923463565191));
#9777=CARTESIAN_POINT('Ctrl Pts',(-7.933993206594,3.60294162668782,2.73965677245104));
#9778=CARTESIAN_POINT('Ctrl Pts',(-8.21874543774091,3.55943297781633,1.7046481710116));
#9779=CARTESIAN_POINT('Ctrl Pts',(-8.38657213518008,3.46852426640382,-0.457940203903986));
#9780=CARTESIAN_POINT('Ctrl Pts',(-8.25175791078302,3.42193633662906,-1.56620049906026));
#9781=CARTESIAN_POINT('Ctrl Pts',(-7.56938605684569,3.33525511430828,-3.62822294775514));
#9782=CARTESIAN_POINT('Ctrl Pts',(-7.0429821529524,3.29818716034735,-4.5668361622465));
#9783=CARTESIAN_POINT('Ctrl Pts',(-5.65843785820305,3.21341859132525,-6.20178141656848));
#9784=CARTESIAN_POINT('Ctrl Pts',(-4.81050026118659,3.16828735903497,-6.88032550288151));
#9785=CARTESIAN_POINT('Ctrl Pts',(-2.87942229464534,3.07676981877775,-7.8897434382078));
#9786=CARTESIAN_POINT('Ctrl Pts',(-1.8098638956802,3.03128070198162,-8.20145615779368));
#9787=CARTESIAN_POINT('Ctrl Pts',(-0.473919123104029,2.98024015797251,-8.31589518941546));
#9788=CARTESIAN_POINT('Ctrl Pts',(-0.236834098017002,2.97139666518413,-8.326));
#9789=CARTESIAN_POINT('Ctrl Pts',(-1.73680514414798E-13,2.96277469534536,
-8.326));
#9790=CARTESIAN_POINT('Origin',(0.,-25.4,0.));
#9791=CARTESIAN_POINT('',(-1.6746832197628E-14,0.862774695345363,-8.32600000000001));
#9792=CARTESIAN_POINT('',(-5.1302523839086E-14,1.26372307941298,-8.326));
#9793=CARTESIAN_POINT('',(-1.01964092497009E-15,-25.4,-8.326));
#9794=CARTESIAN_POINT('Ctrl Pts',(-1.69645946028209E-13,1.26372307941299,
-8.326));
#9795=CARTESIAN_POINT('Ctrl Pts',(-0.0837768214034725,1.26677298326288,
-8.326));
#9796=CARTESIAN_POINT('Ctrl Pts',(-0.167601579300017,1.26985120902554,-8.32473555275498));
#9797=CARTESIAN_POINT('Ctrl Pts',(-1.3539457410103,1.31379357929034,-8.28889148852802));
#9798=CARTESIAN_POINT('Ctrl Pts',(-2.43880631725384,1.35858594554283,-8.03683231760474));
#9799=CARTESIAN_POINT('Ctrl Pts',(-4.42773562785666,1.44997899855494,-7.13353859692295));
#9800=CARTESIAN_POINT('Ctrl Pts',(-5.31606588894694,1.49566420549788,-6.49860012585041));
#9801=CARTESIAN_POINT('Ctrl Pts',(-6.78387820388031,1.58182325722266,-4.94172411894643));
#9802=CARTESIAN_POINT('Ctrl Pts',(-7.35624026525427,1.61886395956457,-4.04070580530918));
#9803=CARTESIAN_POINT('Ctrl Pts',(-8.15281686088358,1.70370780369458,-2.02239195894645));
#9804=CARTESIAN_POINT('Ctrl Pts',(-8.34970350508474,1.75018032569696,-0.916877049826637));
#9805=CARTESIAN_POINT('Ctrl Pts',(-8.29874479024791,1.84183306570532,1.26341070248638));
#9806=CARTESIAN_POINT('Ctrl Pts',(-8.06811115217157,1.88614789682518,2.31759722792569));
#9807=CARTESIAN_POINT('Ctrl Pts',(-7.21550118058259,1.96918938584951,4.29303562111409));
#9808=CARTESIAN_POINT('Ctrl Pts',(-6.59701641921928,2.00771898813145,5.19356725068109));
#9809=CARTESIAN_POINT('Ctrl Pts',(-5.03870961518502,2.09650276267898,6.71857901736009));
#9810=CARTESIAN_POINT('Ctrl Pts',(-4.10975467197251,2.14304184596436,7.32377847168283));
#9811=CARTESIAN_POINT('Ctrl Pts',(-2.10874593485223,2.23269950506558,8.12358492789594));
#9812=CARTESIAN_POINT('Ctrl Pts',(-1.0614027300489,2.27507127258183,8.32546092044366));
#9813=CARTESIAN_POINT('Ctrl Pts',(1.09821997672844,2.35371566105738,8.32655997253554));
#9814=CARTESIAN_POINT('Ctrl Pts',(2.19016207354498,2.39803518065504,8.1081431028105));
#9815=CARTESIAN_POINT('Ctrl Pts',(4.20907432661105,2.48925161014868,7.26518460420603));
#9816=CARTESIAN_POINT('Ctrl Pts',(5.11892502241012,2.53518909188473,6.65551810557873));
#9817=CARTESIAN_POINT('Ctrl Pts',(6.63252465185689,2.62209304366012,5.14250783763209));
#9818=CARTESIAN_POINT('Ctrl Pts',(7.23015926129918,2.65958222891784,4.26150491778023));
#9819=CARTESIAN_POINT('Ctrl Pts',(8.08371261568657,2.74292541938276,2.27888947831906));
#9820=CARTESIAN_POINT('Ctrl Pts',(8.31421456842586,2.7887492107285,1.18880694476285));
#9821=CARTESIAN_POINT('Ctrl Pts',(8.33658991899218,2.88021085400004,-0.986934889176645));
#9822=CARTESIAN_POINT('Ctrl Pts',(8.14025679028578,2.92496811769043,-2.05164625342269));
#9823=CARTESIAN_POINT('Ctrl Pts',(7.35415411630031,3.00891174121332,-4.04854513756839));
#9824=CARTESIAN_POINT('Ctrl Pts',(6.77162781890511,3.04649077030201,-4.96179654281381));
#9825=CARTESIAN_POINT('Ctrl Pts',(5.27215257541828,3.13420139337505,-6.53765008044056));
#9826=CARTESIAN_POINT('Ctrl Pts',(4.36163341616348,3.18079171921284,-7.17721922349229));
#9827=CARTESIAN_POINT('Ctrl Pts',(2.3824705566221,3.27114625086254,-8.04801905440062));
#9828=CARTESIAN_POINT('Ctrl Pts',(1.33904462603134,3.3141296388214,-8.285779118084));
#9829=CARTESIAN_POINT('Ctrl Pts',(0.185981993360484,3.35691966319102,-8.32444315628126));
#9830=CARTESIAN_POINT('Ctrl Pts',(0.0929600549114514,3.36033885899719,-8.326));
#9831=CARTESIAN_POINT('Ctrl Pts',(-1.69645946028209E-13,3.36372307941297,
-8.326));
#9832=CARTESIAN_POINT('Ctrl Pts',(-1.82076576038526E-13,2.96277469534536,
-8.326));
#9833=CARTESIAN_POINT('Ctrl Pts',(0.813556815714888,2.93315707530678,-8.32600000000002));
#9834=CARTESIAN_POINT('Ctrl Pts',(1.62397012934317,2.90114791058247,-8.20677243150924));
#9835=CARTESIAN_POINT('Ctrl Pts',(3.44723056130226,2.82320780122122,-7.65658441771259));
#9836=CARTESIAN_POINT('Ctrl Pts',(4.41743669168115,2.77704906892423,-7.14093012874506));
#9837=CARTESIAN_POINT('Ctrl Pts',(6.12293048574269,2.685736751059,-5.75055284036092));
#9838=CARTESIAN_POINT('Ctrl Pts',(6.83531027266515,2.643012464414,-4.88231332932904));
#9839=CARTESIAN_POINT('Ctrl Pts',(7.85303680208091,2.56231749481875,-2.96269528118814));
#9840=CARTESIAN_POINT('Ctrl Pts',(8.1662290676751,2.51928806067112,-1.9390865134368));
#9841=CARTESIAN_POINT('Ctrl Pts',(8.3959665744779,2.42888316692028,0.211516759046871));
#9842=CARTESIAN_POINT('Ctrl Pts',(8.29427947588552,2.38229118501643,1.31987344856551));
#9843=CARTESIAN_POINT('Ctrl Pts',(7.67355633196759,2.29466647743399,3.404340063799));
#9844=CARTESIAN_POINT('Ctrl Pts',(7.17165113038443,2.2571446505772,4.36352557621024));
#9845=CARTESIAN_POINT('Ctrl Pts',(5.83126000942862,2.17313074369003,6.03904170265549));
#9846=CARTESIAN_POINT('Ctrl Pts',(5.00531155999211,2.12834042858072,6.73945224437031));
#9847=CARTESIAN_POINT('Ctrl Pts',(3.10680679284471,2.03687052649224,7.80302212805181));
#9848=CARTESIAN_POINT('Ctrl Pts',(2.04661048153777,1.99107309342936,8.14561926619544));
#9849=CARTESIAN_POINT('Ctrl Pts',(-0.0976340101182796,1.90783304287678,
8.39200263937633));
#9850=CARTESIAN_POINT('Ctrl Pts',(-1.15903231784563,1.87028914896897,8.31216195281203));
#9851=CARTESIAN_POINT('Ctrl Pts',(-3.22479127438158,1.78332090368117,7.75246079163234));
#9852=CARTESIAN_POINT('Ctrl Pts',(-4.2066826292331,1.73736323871729,7.2666121143808));
#9853=CARTESIAN_POINT('Ctrl Pts',(-5.94282182088796,1.64616598469532,5.93478862055471));
#9854=CARTESIAN_POINT('Ctrl Pts',(-6.67570707028367,1.60200963702447,5.09634321262818));
#9855=CARTESIAN_POINT('Ctrl Pts',(-7.74965742290837,1.5232309206312,3.22231009065765));
#9856=CARTESIAN_POINT('Ctrl Pts',(-8.09581206121049,1.48080730375074,2.21311285023932));
#9857=CARTESIAN_POINT('Ctrl Pts',(-8.39775521983311,1.39108869823119,0.0788353943661968));
#9858=CARTESIAN_POINT('Ctrl Pts',(-8.33492431754466,1.34454331319512,-1.02841282223466));
#9859=CARTESIAN_POINT('Ctrl Pts',(-7.78733004158013,1.25584594677796,-3.13839645877649));
#9860=CARTESIAN_POINT('Ctrl Pts',(-7.31430595671989,1.21740957143647,-4.12223537722999));
#9861=CARTESIAN_POINT('Ctrl Pts',(-6.02559014343174,1.13429368963372,-5.84453029432095));
#9862=CARTESIAN_POINT('Ctrl Pts',(-5.22579107191315,1.08994115003569,-6.56940477934618));
#9863=CARTESIAN_POINT('Ctrl Pts',(-3.39229921268728,0.999870221400379,-7.67902116285679));
#9864=CARTESIAN_POINT('Ctrl Pts',(-2.37477190565768,0.954986193959591,-8.05206595434195));
#9865=CARTESIAN_POINT('Ctrl Pts',(-0.878764722238898,0.895496747091505,
-8.29124341631015));
#9866=CARTESIAN_POINT('Ctrl Pts',(-0.43924976329083,0.878765628418327,-8.32599999999999));
#9867=CARTESIAN_POINT('Ctrl Pts',(-2.1163626406917E-13,0.862774695345371,
-8.326));
#9868=CARTESIAN_POINT('Origin',(0.,-25.4,0.));
#9869=CARTESIAN_POINT('',(1.71843589924784E-14,-1.23722530465463,-8.326));
#9870=CARTESIAN_POINT('',(-1.91468180698012E-13,-0.836276920586999,-8.326));
#9871=CARTESIAN_POINT('',(-1.01964092497009E-15,-25.4,-8.326));
#9872=CARTESIAN_POINT('Ctrl Pts',(-2.39808173319034E-13,-0.836276920587004,
-8.326));
#9873=CARTESIAN_POINT('Ctrl Pts',(-0.255368949442104,-0.826980187564671,
-8.326));
#9874=CARTESIAN_POINT('Ctrl Pts',(-0.511010728906746,-0.817426591330658,
-8.31425173774534));
#9875=CARTESIAN_POINT('Ctrl Pts',(-1.86474347872633,-0.765514493499206,
-8.1891563457596));
#9876=CARTESIAN_POINT('Ctrl Pts',(-2.93221896013381,-0.719950607316501,
-7.87027859334921));
#9877=CARTESIAN_POINT('Ctrl Pts',(-4.85590214026335,-0.628437197390175,
-6.84824902158977));
#9878=CARTESIAN_POINT('Ctrl Pts',(-5.69880496181663,-0.583381716280099,
-6.16458847309249));
#9879=CARTESIAN_POINT('Ctrl Pts',(-7.07317588236123,-0.498785972970789,
-4.52024497139059));
#9880=CARTESIAN_POINT('Ctrl Pts',(-7.59394586307286,-0.46164039435956,-3.57693223608604));
#9881=CARTESIAN_POINT('Ctrl Pts',(-8.26218083383954,-0.37473971366601,-1.50968918621494));
#9882=CARTESIAN_POINT('Ctrl Pts',(-8.38937147905276,-0.328147295434776,
-0.401322117091165));
#9883=CARTESIAN_POINT('Ctrl Pts',(-8.20726869881849,-0.237347928498029,
1.75866510895241));
#9884=CARTESIAN_POINT('Ctrl Pts',(-7.91594414736932,-0.193946534618926,
2.79112226734456));
#9885=CARTESIAN_POINT('Ctrl Pts',(-6.94276165816964,-0.112603341226765,
4.72616063358038));
#9886=CARTESIAN_POINT('Ctrl Pts',(-6.25638197848218,-0.0712687203542418,
5.60327588765145));
#9887=CARTESIAN_POINT('Ctrl Pts',(-4.59069347327753,0.0193838465750226,
7.03120889421505));
#9888=CARTESIAN_POINT('Ctrl Pts',(-3.63093094664952,0.0656817477729541,
7.57157329417422));
#9889=CARTESIAN_POINT('Ctrl Pts',(-1.59316574834101,0.153911777804031,8.23979317988505));
#9890=CARTESIAN_POINT('Ctrl Pts',(-0.538895882621613,0.193073454439265,
8.37505510863373));
#9891=CARTESIAN_POINT('Ctrl Pts',(1.61359623483333,0.27422539722241,8.242303244025));
#9892=CARTESIAN_POINT('Ctrl Pts',(2.69017757877837,0.31943101084386,7.95624289300489));
#9893=CARTESIAN_POINT('Ctrl Pts',(4.64693956999572,0.4109295297381,6.99221597546405));
#9894=CARTESIAN_POINT('Ctrl Pts',(5.51257792110755,0.456315648234544,6.33220373713382));
#9895=CARTESIAN_POINT('Ctrl Pts',(6.93322897944752,0.541692550568771,4.73085447095174));
#9896=CARTESIAN_POINT('Ctrl Pts',(7.47958407163772,0.578615355971894,3.80873401534467));
#9897=CARTESIAN_POINT('Ctrl Pts',(8.21180291906934,0.664508608103169,1.76545625178619));
#9898=CARTESIAN_POINT('Ctrl Pts',(8.37361188370897,0.711063595039071,0.657979619704897));
#9899=CARTESIAN_POINT('Ctrl Pts',(8.25647245025157,0.802327859707633,-1.51306685923906));
#9900=CARTESIAN_POINT('Ctrl Pts',(7.99512358570411,0.846201783309242,-2.55676482468719));
#9901=CARTESIAN_POINT('Ctrl Pts',(7.08200810399254,0.928401211867213,-4.5121718023247));
#9902=CARTESIAN_POINT('Ctrl Pts',(6.42989899223848,0.968163647926906,-5.40103844750506));
#9903=CARTESIAN_POINT('Ctrl Pts',(4.81779649078895,1.0578990590066,-6.87814948027013));
#9904=CARTESIAN_POINT('Ctrl Pts',(3.87293675512195,1.10434150518562,-7.45120330856285));
#9905=CARTESIAN_POINT('Ctrl Pts',(1.93192930928717,1.18983341635668,-8.15674066542193));
#9906=CARTESIAN_POINT('Ctrl Pts',(0.969300700853793,1.22843558712422,-8.32600000000001));
#9907=CARTESIAN_POINT('Ctrl Pts',(-2.25375273998907E-13,1.26372307941299,
-8.326));
#9908=CARTESIAN_POINT('Ctrl Pts',(-1.974809205052E-13,0.86277469534537,
-8.32600000000001));
#9909=CARTESIAN_POINT('Ctrl Pts',(0.626897877395358,0.839952413266184,-8.32600000000002));
#9910=CARTESIAN_POINT('Ctrl Pts',(1.25314594048656,0.815665821847271,-8.2552068339659));
#9911=CARTESIAN_POINT('Ctrl Pts',(2.94183309963131,0.74602281149041,-7.86668333894596));
#9912=CARTESIAN_POINT('Ctrl Pts',(3.95700950465341,0.69942798442542,-7.40817170741499));
#9913=CARTESIAN_POINT('Ctrl Pts',(5.71575539196035,0.608881692148581,-6.14647505899301));
#9914=CARTESIAN_POINT('Ctrl Pts',(6.45209755885893,0.565721351262088,-5.36841139969592));
#9915=CARTESIAN_POINT('Ctrl Pts',(7.61804276313728,0.484800491399616,-3.53790442254404));
#9916=CARTESIAN_POINT('Ctrl Pts',(8.02098224619923,0.442579217743075,-2.49314986709691));
#9917=CARTESIAN_POINT('Ctrl Pts',(8.39059674336028,0.351493380304156,-0.326347917050532));
#9918=CARTESIAN_POINT('Ctrl Pts',(8.36129455522583,0.305283315324501,0.772923514436969));
#9919=CARTESIAN_POINT('Ctrl Pts',(7.8889425125532,0.217421472437857,2.86303123979268));
#9920=CARTESIAN_POINT('Ctrl Pts',(7.4637722429967,0.178841792696816,3.83720615500331));
#9921=CARTESIAN_POINT('Ctrl Pts',(6.24471135935666,0.0970675653949035,5.61631486139091));
#9922=CARTESIAN_POINT('Ctrl Pts',(5.44645262225463,0.0516743286916036,6.39337067852439));
#9923=CARTESIAN_POINT('Ctrl Pts',(3.61583772491597,-0.0398425650265737,
7.5767649935127));
#9924=CARTESIAN_POINT('Ctrl Pts',(2.60667655209084,-0.0850653940335428,
7.98041956522313));
#9925=CARTESIAN_POINT('Ctrl Pts',(0.502323978040994,-0.170047473770475,
8.37877853787446));
#9926=CARTESIAN_POINT('Ctrl Pts',(-0.572212235113425,-0.207041635407368,
8.37429626480301));
#9927=CARTESIAN_POINT('Ctrl Pts',(-2.70226013375954,-0.293448947391339,
7.95263442165316));
#9928=CARTESIAN_POINT('Ctrl Pts',(-3.73399768157828,-0.340028369924945,
7.52354043446785));
#9929=CARTESIAN_POINT('Ctrl Pts',(-5.53447836288067,-0.431067133719925,
6.31070018191802));
#9930=CARTESIAN_POINT('Ctrl Pts',(-6.29521685254581,-0.474706202518919,
5.55211568688792));
#9931=CARTESIAN_POINT('Ctrl Pts',(-7.5080208242872,-0.556474917320835,3.76243196018632));
#9932=CARTESIAN_POINT('Ctrl Pts',(-7.93800651383442,-0.596989508342807,
2.7412949716939));
#9933=CARTESIAN_POINT('Ctrl Pts',(-8.37625091447417,-0.687192712219641,
0.595489613184537));
#9934=CARTESIAN_POINT('Ctrl Pts',(-8.38202861856108,-0.733568153513214,
-0.507715884559157));
#9935=CARTESIAN_POINT('Ctrl Pts',(-7.97453695305073,-0.82216555754434,-2.61532155874035));
#9936=CARTESIAN_POINT('Ctrl Pts',(-7.5798228992792,-0.86200280905928,-3.60262409777236));
#9937=CARTESIAN_POINT('Ctrl Pts',(-6.41670722618219,-0.942522461806419,
-5.41894367844299));
#9938=CARTESIAN_POINT('Ctrl Pts',(-5.64317509392435,-0.987528150287472,
-6.22038879433125));
#9939=CARTESIAN_POINT('Ctrl Pts',(-3.84785176083109,-1.07898562990653,-7.46208313858954));
#9940=CARTESIAN_POINT('Ctrl Pts',(-2.84847711250222,-1.12452574484206,-7.89778402590663));
#9941=CARTESIAN_POINT('Ctrl Pts',(-1.20336946459652,-1.19204472116218,-8.26073397776654));
#9942=CARTESIAN_POINT('Ctrl Pts',(-0.601927322205734,-1.21531207822038,
-8.32599999999999));
#9943=CARTESIAN_POINT('Ctrl Pts',(-1.81243908770057E-13,-1.23722530465462,
-8.326));
#9944=CARTESIAN_POINT('Origin',(0.,-25.4,0.));
#9945=CARTESIAN_POINT('',(1.68035912463422E-13,-3.33722530465466,-8.326));
#9946=CARTESIAN_POINT('',(-4.60289644721165E-14,-2.93627692058703,-8.326));
#9947=CARTESIAN_POINT('',(-1.01964092497009E-15,-25.4,-8.326));
#9948=CARTESIAN_POINT('Ctrl Pts',(-1.52516888007881E-13,-2.93627692058703,
-8.326));
#9949=CARTESIAN_POINT('Ctrl Pts',(-0.419347816656509,-2.92101051994014,
-8.326));
#9950=CARTESIAN_POINT('Ctrl Pts',(-0.838976472693165,-2.90506806032965,
-8.29432147418403));
#9951=CARTESIAN_POINT('Ctrl Pts',(-2.35405396764038,-2.84505473469001,-8.06325010554558));
#9952=CARTESIAN_POINT('Ctrl Pts',(-3.40812639263809,-2.79857044827765,-7.67736756524498));
#9953=CARTESIAN_POINT('Ctrl Pts',(-5.26618315455172,-2.70695816396692,-6.53696554210616));
#9954=CARTESIAN_POINT('Ctrl Pts',(-6.06103874368431,-2.66269210570163,-5.80764322935427));
#9955=CARTESIAN_POINT('Ctrl Pts',(-7.34007153167069,-2.5797462304383,-4.07666524588282));
#9956=CARTESIAN_POINT('Ctrl Pts',(-7.80765100377409,-2.54109299157087,-3.08813887717487));
#9957=CARTESIAN_POINT('Ctrl Pts',(-8.34142423238497,-2.45219871426703,-0.97347101194023));
#9958=CARTESIAN_POINT('Ctrl Pts',(-8.39697114654256,-2.40566826989119,0.133421787697617));
#9959=CARTESIAN_POINT('Ctrl Pts',(-8.08149228983829,-2.31607566197319,2.26470194062641));
#9960=CARTESIAN_POINT('Ctrl Pts',(-7.72908041097248,-2.27390250326293,3.27104224553266));
#9961=CARTESIAN_POINT('Ctrl Pts',(-6.64387894148651,-2.19515835887964,5.13783957042563));
#9962=CARTESIAN_POINT('Ctrl Pts',(-5.9057366629076,-2.15076126886918,5.97162633458237));
#9963=CARTESIAN_POINT('Ctrl Pts',(-4.16220688676714,-2.05953390545653,7.29208147936309));
#9964=CARTESIAN_POINT('Ctrl Pts',(-3.17798706527946,-2.01362295991409,7.77167435750885));
#9965=CARTESIAN_POINT('Ctrl Pts',(-1.10914838475207,-1.92680230808719,8.31901920508821));
#9966=CARTESIAN_POINT('Ctrl Pts',(-0.0468512596586299,-1.8893801589713,
8.39249445380201));
#9967=CARTESIAN_POINT('Ctrl Pts',(2.09630088469165,-1.80590378948209,8.13297569977981));
#9968=CARTESIAN_POINT('Ctrl Pts',(3.15440692553243,-1.76004638159588,7.78390467624997));
#9969=CARTESIAN_POINT('Ctrl Pts',(5.04585127685949,-1.66859639437445,6.70905328611966));
#9970=CARTESIAN_POINT('Ctrl Pts',(5.86709482506276,-1.62388233158846,6.00412148410425));
#9971=CARTESIAN_POINT('Ctrl Pts',(7.19812694415682,-1.54002990006924,4.32007762757575));
#9972=CARTESIAN_POINT('Ctrl Pts',(7.69482077893012,-1.50237294510652,3.35647285756903));
#9973=CARTESIAN_POINT('Ctrl Pts',(8.30237793912328,-1.41455134371416,1.26732241987429));
#9974=CARTESIAN_POINT('Ctrl Pts',(8.39703215218012,-1.36796367610518,0.159068361267252));
#9975=CARTESIAN_POINT('Ctrl Pts',(8.15419247908559,-1.27767534839152,-1.98876197171501));
#9976=CARTESIAN_POINT('Ctrl Pts',(7.83500228377835,-1.2347520572277,-3.00984574951449));
#9977=CARTESIAN_POINT('Ctrl Pts',(6.80494146750566,-1.15423861122331,-4.92514561074857));
#9978=CARTESIAN_POINT('Ctrl Pts',(6.08527294656668,-1.11109595639874,-5.79089739470389));
#9979=CARTESIAN_POINT('Ctrl Pts',(4.36875245723809,-1.01960431883729,-7.17070740544971));
#9980=CARTESIAN_POINT('Ctrl Pts',(3.39574973309031,-0.973488997974973,-7.67945245989225));
#9981=CARTESIAN_POINT('Ctrl Pts',(1.58727304806974,-0.896454993343481,-8.21213680034134));
#9982=CARTESIAN_POINT('Ctrl Pts',(0.795046098036533,-0.865220656033569,
-8.32600000000002));
#9983=CARTESIAN_POINT('Ctrl Pts',(-1.76803016671556E-13,-0.836276920587007,
-8.326));
#9984=CARTESIAN_POINT('Ctrl Pts',(-1.64313007644523E-13,-1.23722530465462,
-8.326));
#9985=CARTESIAN_POINT('Ctrl Pts',(0.45333287016887,-1.25372893469042,-8.32600000000001));
#9986=CARTESIAN_POINT('Ctrl Pts',(0.906883604181015,-1.27101861962826,-8.2889791048775));
#9987=CARTESIAN_POINT('Ctrl Pts',(2.45137675289882,-1.33260520473156,-8.03400595285804));
#9988=CARTESIAN_POINT('Ctrl Pts',(3.4994098080405,-1.37912460857061,-7.63599213029627));
#9989=CARTESIAN_POINT('Ctrl Pts',(5.3417347790895,-1.47059325393864,-6.47517577658188));
#9990=CARTESIAN_POINT('Ctrl Pts',(6.12721156907266,-1.51469212536274,-5.73756317941479));
#9991=CARTESIAN_POINT('Ctrl Pts',(7.38793936163156,-1.59731514352563,-3.99024063221344));
#9992=CARTESIAN_POINT('Ctrl Pts',(7.84519299083219,-1.6364171675431,-2.99279585597472));
#9993=CARTESIAN_POINT('Ctrl Pts',(8.35273678667891,-1.72567995947416,-0.869361554209782));
#9994=CARTESIAN_POINT('Ctrl Pts',(8.39451611548493,-1.77217678388878,0.236731474578972));
#9995=CARTESIAN_POINT('Ctrl Pts',(8.05356647674601,-1.86149975252815,2.36159729426944));
#9996=CARTESIAN_POINT('Ctrl Pts',(7.68954020709712,-1.90296397982766,3.36261837976914));
#9997=CARTESIAN_POINT('Ctrl Pts',(6.58294250017045,-1.98219883243943,5.21570282980361));
#9998=CARTESIAN_POINT('Ctrl Pts',(5.83497839553806,-2.02677082600436,6.04079910360755));
#9999=CARTESIAN_POINT('Ctrl Pts',(4.07693071225599,-2.11807821982965,7.33991611397237));
#10000=CARTESIAN_POINT('Ctrl Pts',(3.08837653689269,-2.16389552857394,7.80754669966619));
#10001=CARTESIAN_POINT('Ctrl Pts',(1.01371873022242,-2.25043234230026,8.33130831925508));
#10002=CARTESIAN_POINT('Ctrl Pts',(-0.0503438229743022,-2.2876583024077,
8.39259726328537));
#10003=CARTESIAN_POINT('Ctrl Pts',(-2.20140372280025,-2.37198004742297,
8.10655459135599));
#10004=CARTESIAN_POINT('Ctrl Pts',(-3.26463690440948,-2.41839613987866,
7.73978342056256));
#10005=CARTESIAN_POINT('Ctrl Pts',(-5.14681570295621,-2.51020813123452,
6.63166049983803));
#10006=CARTESIAN_POINT('Ctrl Pts',(-5.95614134912819,-2.55472405224028,
5.91551330576726));
#10007=CARTESIAN_POINT('Ctrl Pts',(-7.26359036630716,-2.63816729368409,
4.21009041318948));
#10008=CARTESIAN_POINT('Ctrl Pts',(-7.74711629613665,-2.67622471447422,
3.23525975383656));
#10009=CARTESIAN_POINT('Ctrl Pts',(-8.32134354280608,-2.76453738050967,
1.13442758980562));
#10010=CARTESIAN_POINT('Ctrl Pts',(-8.39826570590334,-2.81110609603825,
0.026624374117372));
#10011=CARTESIAN_POINT('Ctrl Pts',(-8.12245633024576,-2.90108553134084,
-2.11385784968141));
#10012=CARTESIAN_POINT('Ctrl Pts',(-7.7882058564614,-2.9437343272369,-3.12841177719816));
#10013=CARTESIAN_POINT('Ctrl Pts',(-6.73602202434712,-3.02309937664837,
-5.01639292405682));
#10014=CARTESIAN_POINT('Ctrl Pts',(-6.01308051593968,-3.06656282599005,
-5.86361355011189));
#10015=CARTESIAN_POINT('Ctrl Pts',(-4.29182791602042,-3.15766797377071,
-7.216839225372));
#10016=CARTESIAN_POINT('Ctrl Pts',(-3.31452643198635,-3.20371095642881,
-7.71469696420591));
#10017=CARTESIAN_POINT('Ctrl Pts',(-1.52959397443031,-3.2793189003798,-8.22031321013249));
#10018=CARTESIAN_POINT('Ctrl Pts',(-0.765970835835665,-3.30934005713638,
-8.32600000000001));
#10019=CARTESIAN_POINT('Ctrl Pts',(2.7602919949743E-13,-3.33722530465466,
-8.32600000000001));
#10020=CARTESIAN_POINT('Origin',(0.,-25.4,0.));
#10021=CARTESIAN_POINT('',(6.90525909241849E-14,-5.43722530465464,-8.326));
#10022=CARTESIAN_POINT('',(2.10354451091469E-14,-5.03627692058703,-8.326));
#10023=CARTESIAN_POINT('',(-1.01964092497009E-15,-25.4,-8.326));
#10024=CARTESIAN_POINT('Ctrl Pts',(-1.93317584162855E-13,-5.03627692058702,
-8.32600000000001));
#10025=CARTESIAN_POINT('Ctrl Pts',(-0.627541089026963,-5.01343122232191,
-8.326));
#10026=CARTESIAN_POINT('Ctrl Pts',(-1.25438846567005,-4.98911976048114,
-8.25506161187213));
#10027=CARTESIAN_POINT('Ctrl Pts',(-2.92207237103168,-4.9203349052019,-7.87098798089334));
#10028=CARTESIAN_POINT('Ctrl Pts',(-3.91824713956257,-4.87470570623752,
-7.42550637562141));
#10029=CARTESIAN_POINT('Ctrl Pts',(-5.70237834616604,-4.78328446629484,
-6.16615087989869));
#10030=CARTESIAN_POINT('Ctrl Pts',(-6.46817800278721,-4.73840654091963,
-5.35739132687811));
#10031=CARTESIAN_POINT('Ctrl Pts',(-7.61406835007107,-4.65827666942867,
-3.52978128523068));
#10032=CARTESIAN_POINT('Ctrl Pts',(-7.99942490620298,-4.61798142540627,
-2.5383477346419));
#10033=CARTESIAN_POINT('Ctrl Pts',(-8.38674744177094,-4.52916092693061,
-0.425434962331447));
#10034=CARTESIAN_POINT('Ctrl Pts',(-8.37005524029738,-4.48274354844585,
0.678768161280285));
#10035=CARTESIAN_POINT('Ctrl Pts',(-7.91068720079588,-4.39282183208492,
2.81787733391118));
#10036=CARTESIAN_POINT('Ctrl Pts',(-7.47238878950199,-4.35277187807424,
3.8317740885327));
#10037=CARTESIAN_POINT('Ctrl Pts',(-6.24504309267525,-4.27074256311847,
5.60866941930545));
#10038=CARTESIAN_POINT('Ctrl Pts',(-5.47677251068441,-4.22696068286926,
6.36100250850893));
#10039=CARTESIAN_POINT('Ctrl Pts',(-3.6634992643114,-4.13578340203622,7.55827563330548));
#10040=CARTESIAN_POINT('Ctrl Pts',(-2.62674553517158,-4.089217376626,7.97804394272964));
#10041=CARTESIAN_POINT('Ctrl Pts',(-0.493299661123184,-4.00311931726632,
8.37910696355535));
#10042=CARTESIAN_POINT('Ctrl Pts',(0.579550680952056,-3.96617845848151,
8.37358382216603));
#10043=CARTESIAN_POINT('Ctrl Pts',(2.67956787801854,-3.8809579531506,7.95637214776438));
#10044=CARTESIAN_POINT('Ctrl Pts',(3.68589481875409,-3.83563555477465,7.54307131598211));
#10045=CARTESIAN_POINT('Ctrl Pts',(5.50610740935759,-3.74412705080919,6.34205883767688));
#10046=CARTESIAN_POINT('Ctrl Pts',(6.29702077858317,-3.69884549288094,5.55759382721559));
#10047=CARTESIAN_POINT('Ctrl Pts',(7.49931750586196,-3.61744533361428,3.7672458386162));
#10048=CARTESIAN_POINT('Ctrl Pts',(7.91534818506142,-3.57852575872554,2.78918236097401));
#10049=CARTESIAN_POINT('Ctrl Pts',(8.36836596637517,-3.49044180108196,0.693790842857477));
#10050=CARTESIAN_POINT('Ctrl Pts',(8.38721689004991,-3.44417756367676,-0.406769286183216));
#10051=CARTESIAN_POINT('Ctrl Pts',(8.00606656997257,-3.35545392974148,-2.51737778980474));
#10052=CARTESIAN_POINT('Ctrl Pts',(7.6232516134654,-3.3150284961571,-3.50994129513667));
#10053=CARTESIAN_POINT('Ctrl Pts',(6.48204165644963,-3.23500481003877,-5.34060601389237));
#10054=CARTESIAN_POINT('Ctrl Pts',(5.71835232030774,-3.19016227447647,-6.15133700302137));
#10055=CARTESIAN_POINT('Ctrl Pts',(3.93728803867132,-3.09875232751809,-7.41546728068426));
#10056=CARTESIAN_POINT('Ctrl Pts',(2.9419976746152,-3.05309962121162,-7.86359913161293));
#10057=CARTESIAN_POINT('Ctrl Pts',(1.26823149266639,-2.98397125555753,-8.25348119269115));
#10058=CARTESIAN_POINT('Ctrl Pts',(0.634493343967036,-2.9593757164125,-8.32600000000003));
#10059=CARTESIAN_POINT('Ctrl Pts',(-1.35863542638504E-13,-2.93627692058703,
-8.32600000000001));
#10060=CARTESIAN_POINT('Ctrl Pts',(2.68188249386014E-13,-3.33722530465466,
-8.326));
#10061=CARTESIAN_POINT('Ctrl Pts',(0.284634040473044,-3.34758743634347,
-8.326));
#10062=CARTESIAN_POINT('Ctrl Pts',(0.5695698157431,-3.35826731999166,-8.31140488963583));
#10063=CARTESIAN_POINT('Ctrl Pts',(1.95122153822608,-3.41155987284974,-8.16898847079264));
#10064=CARTESIAN_POINT('Ctrl Pts',(3.01530817863659,-3.4572375489945,-7.8388272723186));
#10065=CARTESIAN_POINT('Ctrl Pts',(4.9271483037556,-3.54873600418471,-6.7969964311812));
#10066=CARTESIAN_POINT('Ctrl Pts',(5.76204111184506,-3.59366811490462,-6.10533174307115));
#10067=CARTESIAN_POINT('Ctrl Pts',(7.12030687096346,-3.67798896252267,-4.44617203508329));
#10068=CARTESIAN_POINT('Ctrl Pts',(7.63214563950504,-3.71529046447498,-3.49536994096109));
#10069=CARTESIAN_POINT('Ctrl Pts',(8.27791829973826,-3.80253606293005,-1.41992179028542));
#10070=CARTESIAN_POINT('Ctrl Pts',(8.3930281071515,-3.84913124309678,-0.31148901866247));
#10071=CARTESIAN_POINT('Ctrl Pts',(8.18833732112736,-3.93974926131201,1.84418418036667));
#10072=CARTESIAN_POINT('Ctrl Pts',(7.88663132312279,-3.98297698808641,2.87251004643474));
#10073=CARTESIAN_POINT('Ctrl Pts',(6.89238308755243,-4.06401504670441,4.80028969230388));
#10074=CARTESIAN_POINT('Ctrl Pts',(6.19377020061474,-4.10598316736002,5.6732273343516));
#10075=CARTESIAN_POINT('Ctrl Pts',(4.50926145560161,-4.1969500512168,7.08351703071612));
#10076=CARTESIAN_POINT('Ctrl Pts',(3.54449358779289,-4.24318556136984,7.61224353778558));
#10077=CARTESIAN_POINT('Ctrl Pts',(1.50056805248625,-4.3311499187908,8.25715346310258));
#10078=CARTESIAN_POINT('Ctrl Pts',(0.44488149708526,-4.36988227433181,8.38057447494808));
#10079=CARTESIAN_POINT('Ctrl Pts',(-1.70603330412962,-4.45148435351502,
8.22367441466779));
#10080=CARTESIAN_POINT('Ctrl Pts',(-2.7793896961637,-4.4968266124313,7.92552709037528));
#10081=CARTESIAN_POINT('Ctrl Pts',(-4.72420305139443,-4.58834064668239,
6.94006635187627));
#10082=CARTESIAN_POINT('Ctrl Pts',(-5.581564023546,-4.633609830387,6.27128069592846));
#10083=CARTESIAN_POINT('Ctrl Pts',(-6.98526054098617,-4.71870200902734,
4.6541116433428));
#10084=CARTESIAN_POINT('Ctrl Pts',(-7.52225758131639,-4.75566777851888,
3.72427989316282));
#10085=CARTESIAN_POINT('Ctrl Pts',(-8.23113434903166,-4.84193264488188,
1.6721619579118));
#10086=CARTESIAN_POINT('Ctrl Pts',(-8.38028167058735,-4.88850639197476,
0.564239048497007));
#10087=CARTESIAN_POINT('Ctrl Pts',(-8.23934139144515,-4.97961002486669,
-1.60298622995543));
#10088=CARTESIAN_POINT('Ctrl Pts',(-7.96698996357564,-5.02331543516025,
-2.64267550453953));
#10089=CARTESIAN_POINT('Ctrl Pts',(-7.03195186438206,-5.10520472094139,
-4.59070462858071));
#10090=CARTESIAN_POINT('Ctrl Pts',(-6.36743914444412,-5.14550073499438,
-5.47530658661011));
#10091=CARTESIAN_POINT('Ctrl Pts',(-4.73579600884035,-5.23557429482982,
-6.9346603998634));
#10092=CARTESIAN_POINT('Ctrl Pts',(-3.7853913736369,-5.28196966790777,-7.49587057678226));
#10093=CARTESIAN_POINT('Ctrl Pts',(-1.86790297413526,-5.36590075728786,
-8.16788467551488));
#10094=CARTESIAN_POINT('Ctrl Pts',(-0.936858401587628,-5.40311887762686,
-8.32600000000001));
#10095=CARTESIAN_POINT('Ctrl Pts',(2.76167977375508E-13,-5.43722530465465,
-8.32600000000001));
#10096=CARTESIAN_POINT('Origin',(0.,-25.4,0.));
#10097=CARTESIAN_POINT('',(1.3923078857642E-14,-7.53722530465463,-8.32600000000001));
#10098=CARTESIAN_POINT('',(1.79415698465829E-13,-7.13627692058703,-8.326));
#10099=CARTESIAN_POINT('',(-1.01964092497009E-15,-25.4,-8.326));
#10100=CARTESIAN_POINT('Ctrl Pts',(2.82274204010946E-13,-7.13627692058702,
-8.32600000000001));
#10101=CARTESIAN_POINT('Ctrl Pts',(-0.789165471781706,-7.10754726994771,
-8.32600000000001));
#10102=CARTESIAN_POINT('Ctrl Pts',(-1.57561086339154,-7.076558686669,-8.21381512205618));
#10103=CARTESIAN_POINT('Ctrl Pts',(-3.3793572552361,-6.9998128428404,-7.68664754117325));
#10104=CARTESIAN_POINT('Ctrl Pts',(-4.35323870101583,-6.95371174366766,
-7.18010110459946));
#10105=CARTESIAN_POINT('Ctrl Pts',(-6.06353261638026,-6.86268119196448,
-5.8114434991415));
#10106=CARTESIAN_POINT('Ctrl Pts',(-6.77919512355584,-6.81969313260729,
-4.95792394651815));
#10107=CARTESIAN_POINT('Ctrl Pts',(-7.81547082758754,-6.73990905249919,
-3.05997465800181));
#10108=CARTESIAN_POINT('Ctrl Pts',(-8.14103231066469,-6.69710048598408,
-2.04162001570176));
#10109=CARTESIAN_POINT('Ctrl Pts',(-8.39780737308328,-6.60693999020395,
0.103169378199973));
#10110=CARTESIAN_POINT('Ctrl Pts',(-8.31064190933164,-6.56035891466547,
1.2112666208665));
#10111=CARTESIAN_POINT('Ctrl Pts',(-7.71713685090388,-6.4723289820834,3.30537295994639));
#10112=CARTESIAN_POINT('Ctrl Pts',(-7.22599867976158,-6.43451331818395,
4.27370401224569));
#10113=CARTESIAN_POINT('Ctrl Pts',(-5.90492838340159,-6.35083333427368,
5.96679768736565));
#10114=CARTESIAN_POINT('Ctrl Pts',(-5.08870848526377,-6.30620192994361,
6.67649805336952));
#10115=CARTESIAN_POINT('Ctrl Pts',(-3.1951027538352,-6.21430444864484,7.76889631299521));
#10116=CARTESIAN_POINT('Ctrl Pts',(-2.12757422265706,-6.16792702929897,
8.12638776402861));
#10117=CARTESIAN_POINT('Ctrl Pts',(0.0262958920409874,-6.08391961518951,
8.39260803460962));
#10118=CARTESIAN_POINT('Ctrl Pts',(1.08896143852785,-6.04654298732901,8.32170952011937));
#10119=CARTESIAN_POINT('Ctrl Pts',(3.15903894726869,-5.95978221498718,7.77935928075863));
#10120=CARTESIAN_POINT('Ctrl Pts',(4.14418876263519,-5.91389061189867,7.30229745795536));
#10121=CARTESIAN_POINT('Ctrl Pts',(5.89081572379785,-5.82264522114307,5.98634910552458));
#10122=CARTESIAN_POINT('Ctrl Pts',(6.63104730371181,-5.77821055380764,5.15439329567684));
#10123=CARTESIAN_POINT('Ctrl Pts',(7.72078661688588,-5.69936214463135,3.2904951256647));
#10124=CARTESIAN_POINT('Ctrl Pts',(8.0756620491109,-5.65734359062175,2.28528884202502));
#10125=CARTESIAN_POINT('Ctrl Pts',(8.3965560385927,-5.56780792566576,0.155363280813972));
#10126=CARTESIAN_POINT('Ctrl Pts',(8.34393513110765,-5.52128403700471,-0.951373567734187));
#10127=CARTESIAN_POINT('Ctrl Pts',(7.81572462935436,-5.43231103653743,-3.06791414456359));
#10128=CARTESIAN_POINT('Ctrl Pts',(7.35033571627815,-5.39356666948127,-4.05832948874711));
#10129=CARTESIAN_POINT('Ctrl Pts',(6.07519282028708,-5.31068924186536,-5.79278841929773));
#10130=CARTESIAN_POINT('Ctrl Pts',(5.28232667201742,-5.26645830908955,-6.52388537427337));
#10131=CARTESIAN_POINT('Ctrl Pts',(3.42760068430076,-5.17487557640673,-7.66865048552837));
#10132=CARTESIAN_POINT('Ctrl Pts',(2.37480276131679,-5.12838325423159,-8.05712284670339));
#10133=CARTESIAN_POINT('Ctrl Pts',(0.853433947479236,-5.06803527645898,
-8.29321912371142));
#10134=CARTESIAN_POINT('Ctrl Pts',(0.426582072994635,-5.05180668508432,
-8.32600000000001));
#10135=CARTESIAN_POINT('Ctrl Pts',(-1.83880688453542E-13,-5.03627692058702,
-8.326));
#10136=CARTESIAN_POINT('Ctrl Pts',(3.22658566531686E-13,-5.43722530465465,
-8.326));
#10137=CARTESIAN_POINT('Ctrl Pts',(0.115242825540931,-5.44142073164033,
-8.326));
#10138=CARTESIAN_POINT('Ctrl Pts',(0.230570012134633,-5.44566951968454,
-8.32360735092844));
#10139=CARTESIAN_POINT('Ctrl Pts',(1.44802154484938,-5.49105499582223,-8.27298397950286));
#10140=CARTESIAN_POINT('Ctrl Pts',(2.53001450434268,-5.53600207189707,-8.00859729935472));
#10141=CARTESIAN_POINT('Ctrl Pts',(4.50752570799239,-5.62744383038148,-7.08320957009196));
#10142=CARTESIAN_POINT('Ctrl Pts',(5.38772903319495,-5.67302565544003,-6.43911344783354));
#10143=CARTESIAN_POINT('Ctrl Pts',(6.83852901515565,-5.75890426387314,-4.86611390641289));
#10144=CARTESIAN_POINT('Ctrl Pts',(7.40151074496943,-5.79586215273628,-3.95754172249426));
#10145=CARTESIAN_POINT('Ctrl Pts',(8.17496759702204,-5.88108712121583,-1.93016147232249));
#10146=CARTESIAN_POINT('Ctrl Pts',(8.35922730506451,-5.927594488038,-0.823817654718859));
#10147=CARTESIAN_POINT('Ctrl Pts',(8.28440438257484,-6.01911695318644,1.35337104478397));
#10148=CARTESIAN_POINT('Ctrl Pts',(8.04267463665364,-6.06327745927948,2.40388639830039));
#10149=CARTESIAN_POINT('Ctrl Pts',(7.16831860410432,-6.14601865095975,4.37218114667342));
#10150=CARTESIAN_POINT('Ctrl Pts',(6.53785084847891,-6.18495084955976,5.26853490975192));
#10151=CARTESIAN_POINT('Ctrl Pts',(4.96023544643382,-6.27407958464587,6.77651544047292));
#10152=CARTESIAN_POINT('Ctrl Pts',(4.02546522173726,-6.32058950742719,7.37025515833655));
#10153=CARTESIAN_POINT('Ctrl Pts',(2.01741401214559,-6.41001147690843,8.14665025570088));
#10154=CARTESIAN_POINT('Ctrl Pts',(0.96893740319249,-6.45172920697687,8.33655409840725));
#10155=CARTESIAN_POINT('Ctrl Pts',(-1.18962159763602,-6.53078477097846,
8.31405009682517));
#10156=CARTESIAN_POINT('Ctrl Pts',(-2.27913392655953,-6.5752934368299,8.08354565240009));
#10157=CARTESIAN_POINT('Ctrl Pts',(-4.28736690734935,-6.66657301189691,
7.21908582566198));
#10158=CARTESIAN_POINT('Ctrl Pts',(-5.1896363256036,-6.7124253012663,6.60034137853915));
#10159=CARTESIAN_POINT('Ctrl Pts',(-6.6869764967138,-6.79906641750539,5.07167386650422));
#10160=CARTESIAN_POINT('Ctrl Pts',(-7.27562957264802,-6.83635871872085,
4.18361484138809));
#10161=CARTESIAN_POINT('Ctrl Pts',(-8.11208318058106,-6.92053452190012,
2.18119273490226));
#10162=CARTESIAN_POINT('Ctrl Pts',(-8.33080510686291,-6.96693309058429,
1.07743706957574));
#10163=CARTESIAN_POINT('Ctrl Pts',(-8.32122271503474,-7.05878572940046,
-1.10760598980569));
#10164=CARTESIAN_POINT('Ctrl Pts',(-8.10988188534875,-7.10335578212811,
-2.16786387269312));
#10165=CARTESIAN_POINT('Ctrl Pts',(-7.29480546599385,-7.18690941030035,
-4.15548532458625));
#10166=CARTESIAN_POINT('Ctrl Pts',(-6.69673996384445,-7.22485069476321,
-5.06320242269887));
#10167=CARTESIAN_POINT('Ctrl Pts',(-5.17167919968289,-7.31303200118316,
-6.61713430741024));
#10168=CARTESIAN_POINT('Ctrl Pts',(-4.25301141865439,-7.35960695430917,
-7.24185823383286));
#10169=CARTESIAN_POINT('Ctrl Pts',(-2.26406967797738,-7.44967161048689,
-8.08192909903374));
#10170=CARTESIAN_POINT('Ctrl Pts',(-1.21879508517463,-7.49239522799274,
-8.30412804988923));
#10171=CARTESIAN_POINT('Ctrl Pts',(-0.106565493398858,-7.53333503073361,
-8.32548873079942));
#10172=CARTESIAN_POINT('Ctrl Pts',(-0.0532718526244207,-7.53528593734887,
-8.326));
#10173=CARTESIAN_POINT('Ctrl Pts',(-1.69645946028209E-13,-7.53722530465462,
-8.326));
#10174=CARTESIAN_POINT('Origin',(0.,-25.4,0.));
#10175=CARTESIAN_POINT('',(-2.09648082726249E-13,-9.63722530465461,-8.32599999999999));
#10176=CARTESIAN_POINT('',(-8.53327934765894E-14,-9.23627692058699,-8.326));
#10177=CARTESIAN_POINT('',(-1.01964092497009E-15,-25.4,-8.326));
#10178=CARTESIAN_POINT('Ctrl Pts',(-1.5931700403371E-13,-9.236276920587,
-8.32600000000001));
#10179=CARTESIAN_POINT('Ctrl Pts',(-0.962827742290914,-9.20122507702443,
-8.32599999999999));
#10180=CARTESIAN_POINT('Ctrl Pts',(-1.91916005087542,-9.16289949585406,
-8.15899449696305));
#10181=CARTESIAN_POINT('Ctrl Pts',(-3.85551855683091,-9.07771841623852,
-7.46019341735059));
#10182=CARTESIAN_POINT('Ctrl Pts',(-4.80149563487271,-9.03128485713617,
-6.88949770453631));
#10183=CARTESIAN_POINT('Ctrl Pts',(-6.41750042506982,-8.94148158700807,
-5.41591709451043));
#10184=CARTESIAN_POINT('Ctrl Pts',(-7.0720782020427,-8.90161624283425,-4.52790056294519));
#10185=CARTESIAN_POINT('Ctrl Pts',(-7.98957366844959,-8.81947856321835,
-2.5739625044236));
#10186=CARTESIAN_POINT('Ctrl Pts',(-8.25312633563117,-8.77563794010715,
-1.53105671006943));
#10187=CARTESIAN_POINT('Ctrl Pts',(-8.37502902429166,-8.6844049307812,0.63924624892485));
#10188=CARTESIAN_POINT('Ctrl Pts',(-8.21575204543581,-8.63784572502947,
1.74682324060707));
#10189=CARTESIAN_POINT('Ctrl Pts',(-7.4881957532555,-8.55187785526042,3.79187605116871));
#10190=CARTESIAN_POINT('Ctrl Pts',(-6.94371280324449,-8.51495006180625,
4.71553437529232));
#10191=CARTESIAN_POINT('Ctrl Pts',(-5.52645478157601,-8.42962999276952,
6.32005658747283));
#10192=CARTESIAN_POINT('Ctrl Pts',(-4.66246809746165,-8.38426688399616,
6.98183486007834));
#10193=CARTESIAN_POINT('Ctrl Pts',(-2.70808146161542,-8.29276432099371,
7.950168420921));
#10194=CARTESIAN_POINT('Ctrl Pts',(-1.63213515306542,-8.24753085845283,
8.23865365752571));
#10195=CARTESIAN_POINT('Ctrl Pts',(0.520048250783737,-8.16628844384065,
8.37624462091184));
#10196=CARTESIAN_POINT('Ctrl Pts',(1.57459773525679,-8.12721653133655,8.24335870237829));
#10197=CARTESIAN_POINT('Ctrl Pts',(3.61360696238517,-8.03903962169354,7.57982085407758));
#10198=CARTESIAN_POINT('Ctrl Pts',(4.57438581497659,-7.99275377962882,7.04179052142734));
#10199=CARTESIAN_POINT('Ctrl Pts',(6.24385941608477,-7.90203766145591,5.61738990668474));
#10200=CARTESIAN_POINT('Ctrl Pts',(6.93269095124139,-7.86057902586403,4.74111236724755));
#10201=CARTESIAN_POINT('Ctrl Pts',(7.91011108858901,-7.7792970103382,2.80752933505153));
#10202=CARTESIAN_POINT('Ctrl Pts',(8.20352963955394,-7.73593022547473,1.77589547569885));
#10203=CARTESIAN_POINT('Ctrl Pts',(8.39018480114286,-7.64516658335104,-0.383241908078162));
#10204=CARTESIAN_POINT('Ctrl Pts',(8.26542708644195,-7.59857317969374,-1.49163241907991));
#10205=CARTESIAN_POINT('Ctrl Pts',(7.60170970248472,-7.51160275538163,-3.56053457000042));
#10206=CARTESIAN_POINT('Ctrl Pts',(7.08273791404664,-7.47442901591286,-4.50535137706311));
#10207=CARTESIAN_POINT('Ctrl Pts',(5.71161189305219,-7.38988853142366,-6.15268615287862));
#10208=CARTESIAN_POINT('Ctrl Pts',(4.87031909218055,-7.34485756864492,-6.83796882684674));
#10209=CARTESIAN_POINT('Ctrl Pts',(2.94900870780505,-7.25334634450483,-7.86400420794327));
#10210=CARTESIAN_POINT('Ctrl Pts',(1.88220704353294,-7.20775908119327,-8.18516126286428));
#10211=CARTESIAN_POINT('Ctrl Pts',(0.522825152156074,-7.15556890449744,
-8.31370225250549));
#10212=CARTESIAN_POINT('Ctrl Pts',(0.261272938417734,-7.14578858893879,
-8.326));
#10213=CARTESIAN_POINT('Ctrl Pts',(2.80955814169204E-13,-7.13627692058702,
-8.326));
#10214=CARTESIAN_POINT('Ctrl Pts',(-1.90125692967058E-13,-7.53722530465462,
-8.326));
#10215=CARTESIAN_POINT('Ctrl Pts',(1.04852291534761,-7.57539688985758,-8.32600000000002));
#10216=CARTESIAN_POINT('Ctrl Pts',(2.08830637447319,-7.61741332770767,-8.12793571414206));
#10217=CARTESIAN_POINT('Ctrl Pts',(4.07495867046306,-7.70626649247324,-7.34153871441035));
#10218=CARTESIAN_POINT('Ctrl Pts',(4.99748301714605,-7.75233695005276,-6.7474970123295));
#10219=CARTESIAN_POINT('Ctrl Pts',(6.53860700822734,-7.83968146158204,-5.26119976282755));
#10220=CARTESIAN_POINT('Ctrl Pts',(7.15147389388194,-7.87759810417472,-4.39201734627695));
#10221=CARTESIAN_POINT('Ctrl Pts',(8.04067026318169,-7.96022838452596,-2.42636101998051));
#10222=CARTESIAN_POINT('Ctrl Pts',(8.29105868446047,-8.00586429958108,-1.3407477949843));
#10223=CARTESIAN_POINT('Ctrl Pts',(8.3533153449621,-8.09736952956764,0.836030904638805));
#10224=CARTESIAN_POINT('Ctrl Pts',(8.17583015512162,-8.14234811747502,1.90600725582994));
#10225=CARTESIAN_POINT('Ctrl Pts',(7.42586539952756,-8.22677161790711,3.91432172611022));
#10226=CARTESIAN_POINT('Ctrl Pts',(6.86245535308907,-8.26401027132523,4.8344735219243));
#10227=CARTESIAN_POINT('Ctrl Pts',(5.39478443440082,-8.3511276649061,6.43718960170184));
#10228=CARTESIAN_POINT('Ctrl Pts',(4.4946691345482,-8.39772243939458,7.0949904119213));
#10229=CARTESIAN_POINT('Ctrl Pts',(2.5282478613329,-8.4884092382017,8.00366763973184));
#10230=CARTESIAN_POINT('Ctrl Pts',(1.48742661994211,-8.53170225410734,8.2606703705065));
#10231=CARTESIAN_POINT('Ctrl Pts',(-0.677624860631812,-8.61285449078688,
8.37168276283262));
#10232=CARTESIAN_POINT('Ctrl Pts',(-1.78198178346068,-8.65458119998758,
8.20788193260203));
#10233=CARTESIAN_POINT('Ctrl Pts',(-3.84779404884213,-8.74543124868007,
7.46358798992179));
#10234=CARTESIAN_POINT('Ctrl Pts',(-4.79091179709949,-8.79169076047985,
6.89622044602366));
#10235=CARTESIAN_POINT('Ctrl Pts',(-6.37777986034509,-8.87975474067345,
5.45492399023233));
#10236=CARTESIAN_POINT('Ctrl Pts',(-7.01607527868148,-8.91864235756438,
4.60506176421419));
#10237=CARTESIAN_POINT('Ctrl Pts',(-7.96378240360662,-9.00007632614148,
2.66786398600753));
#10238=CARTESIAN_POINT('Ctrl Pts',(-8.24678415772775,-9.04536811559753,
1.59043701740506));
#10239=CARTESIAN_POINT('Ctrl Pts',(-8.37494108319709,-9.13687770840444,
-0.586445467481097));
#10240=CARTESIAN_POINT('Ctrl Pts',(-8.22882479580037,-9.18219128317005,
-1.66439067747666));
#10241=CARTESIAN_POINT('Ctrl Pts',(-7.53846529710902,-9.26739037080332,
-3.69115525929112));
#10242=CARTESIAN_POINT('Ctrl Pts',(-7.00596906938306,-9.3043347570921,-4.62271324724077));
#10243=CARTESIAN_POINT('Ctrl Pts',(-5.5904624310613,-9.39046073420771,-6.26861174815476));
#10244=CARTESIAN_POINT('Ctrl Pts',(-4.70805124321643,-9.43702813184697,
-6.95577446760812));
#10245=CARTESIAN_POINT('Ctrl Pts',(-2.76390130338,-9.52819326307102,-7.92578446611702));
#10246=CARTESIAN_POINT('Ctrl Pts',(-1.72807464976882,-9.57196243961983,
-8.21409243963136));
#10247=CARTESIAN_POINT('Ctrl Pts',(-0.444099013686395,-9.62087134292898,
-8.31712728198367));
#10248=CARTESIAN_POINT('Ctrl Pts',(-0.221925795915121,-9.62914607309612,
-8.32599999999999));
#10249=CARTESIAN_POINT('Ctrl Pts',(-5.92095816820404E-13,-9.6372253046546,
-8.326));
#10250=CARTESIAN_POINT('Origin',(0.,-25.4,0.));
#10251=CARTESIAN_POINT('',(-9.90421138979677E-14,-11.7372253046546,-8.326));
#10252=CARTESIAN_POINT('',(-4.00615157147562E-14,-11.336276920587,-8.32600000000001));
#10253=CARTESIAN_POINT('',(-1.01964092497009E-15,-25.4,-8.326));
#10254=CARTESIAN_POINT('Ctrl Pts',(-1.69645946028209E-13,-11.336276920587,
-8.326));
#10255=CARTESIAN_POINT('Ctrl Pts',(-0.0871960257465394,-11.3331025402493,
-8.326));
#10256=CARTESIAN_POINT('Ctrl Pts',(-0.174447220291238,-11.3298973610918,
-8.32463023531683));
#10257=CARTESIAN_POINT('Ctrl Pts',(-1.32159335929085,-11.2873770915746,
-8.28855269462512));
#10258=CARTESIAN_POINT('Ctrl Pts',(-2.3653020782673,-11.2444309137276,-8.05305278559879));
#10259=CARTESIAN_POINT('Ctrl Pts',(-4.34591435243672,-11.1541173109236,
-7.1867106920077));
#10260=CARTESIAN_POINT('Ctrl Pts',(-5.25763171742414,-11.1075285653815,
-6.54929208811676));
#10261=CARTESIAN_POINT('Ctrl Pts',(-6.76083033989904,-11.0197490755468,
-4.97661114831729));
#10262=CARTESIAN_POINT('Ctrl Pts',(-7.3456088754959,-10.9821222281375,-4.06416580190189));
#10263=CARTESIAN_POINT('Ctrl Pts',(-8.13593319278081,-10.8982351388597,
-2.06861178668239));
#10264=CARTESIAN_POINT('Ctrl Pts',(-8.33445896658462,-10.8535046155213,
-1.00453653720931));
#10265=CARTESIAN_POINT('Ctrl Pts',(-8.31673721429141,-10.7620500738183,
1.17103636056043));
#10266=CARTESIAN_POINT('Ctrl Pts',(-8.08856308821634,-10.7162053646745,
2.26161649865052));
#10267=CARTESIAN_POINT('Ctrl Pts',(-7.23918189662006,-10.6327795247358,
4.2461980510198));
#10268=CARTESIAN_POINT('Ctrl Pts',(-6.64331845503563,-10.5953324209896,
5.12858740153929));
#10269=CARTESIAN_POINT('Ctrl Pts',(-5.13292371355345,-10.5084801268576,
6.6446909752));
#10270=CARTESIAN_POINT('Ctrl Pts',(-4.22456190574248,-10.462559050157,7.25615579875248));
#10271=CARTESIAN_POINT('Ctrl Pts',(-2.20800795669339,-10.3713414629086,
8.10325408239908));
#10272=CARTESIAN_POINT('Ctrl Pts',(-1.11657276023476,-10.3269643782068,
8.32416776740145));
#10273=CARTESIAN_POINT('Ctrl Pts',(1.04284823483265,-10.2482754933851,8.3277332034444));
#10274=CARTESIAN_POINT('Ctrl Pts',(2.09043928045532,-10.2060195316864,8.12832978682023));
#10275=CARTESIAN_POINT('Ctrl Pts',(4.09310626916356,-10.1163968212246,7.33305826301642));
#10276=CARTESIAN_POINT('Ctrl Pts',(5.0232235754974,-10.0698630308749,6.73012390343341));
#10277=CARTESIAN_POINT('Ctrl Pts',(6.58535863862057,-9.98101056785104,5.20847487455484));
#10278=CARTESIAN_POINT('Ctrl Pts',(7.20621183314151,-9.94240469857657,4.3087710844042));
#10279=CARTESIAN_POINT('Ctrl Pts',(8.06313620508689,-9.8594225795479,2.33474501859507));
#10280=CARTESIAN_POINT('Ctrl Pts',(8.29597620131348,-9.81513799275605,1.28127796251173));
#10281=CARTESIAN_POINT('Ctrl Pts',(8.35167616643896,-9.72351025955491,-0.898414913581594));
#10282=CARTESIAN_POINT('Ctrl Pts',(8.1572962509068,-9.67703035837541,-2.00410536278288));
#10283=CARTESIAN_POINT('Ctrl Pts',(7.36530564639993,-9.5921105506584,-4.02422627435801));
#10284=CARTESIAN_POINT('Ctrl Pts',(6.79480785101672,-9.55508992471361,-4.92674058358165));
#10285=CARTESIAN_POINT('Ctrl Pts',(5.33037633488831,-9.46898644920149,-6.4868281483814));
#10286=CARTESIAN_POINT('Ctrl Pts',(4.44365565862945,-9.4233213765627,-7.12359656949709));
#10287=CARTESIAN_POINT('Ctrl Pts',(2.45697842123912,-9.33191767918727,-8.03129742379779));
#10288=CARTESIAN_POINT('Ctrl Pts',(1.37267689681404,-9.28709405993964,-8.2858118290869));
#10289=CARTESIAN_POINT('Ctrl Pts',(0.180130366492069,-9.24286528284347,
-8.32453949447813));
#10290=CARTESIAN_POINT('Ctrl Pts',(0.0900378828094111,-9.2395547590251,
-8.32600000000001));
#10291=CARTESIAN_POINT('Ctrl Pts',(-1.69645946028209E-13,-9.23627692058699,
-8.326));
#10292=CARTESIAN_POINT('Ctrl Pts',(-5.87307980026708E-13,-9.6372253046546,
-8.326));
#10293=CARTESIAN_POINT('Ctrl Pts',(0.869000389542001,-9.66886135373401,
-8.32600000000007));
#10294=CARTESIAN_POINT('Ctrl Pts',(1.73399941374016,-9.70321097215906,-8.18996555552375));
#10295=CARTESIAN_POINT('Ctrl Pts',(3.60396064025448,-9.78400592166834,-7.58484055309296));
#10296=CARTESIAN_POINT('Ctrl Pts',(4.56801084048846,-9.83041971757347,-7.04638868262423));
#10297=CARTESIAN_POINT('Ctrl Pts',(6.20286970073507,-9.91922029391959,-5.65316958515805));
#10298=CARTESIAN_POINT('Ctrl Pts',(6.8680568557066,-9.95947314318247,-4.82318427548233));
#10299=CARTESIAN_POINT('Ctrl Pts',(7.87622322720337,-10.0396380060417,-2.91617670929505));
#10300=CARTESIAN_POINT('Ctrl Pts',(8.1928178586592,-10.084527539032,-1.84831884736067));
#10301=CARTESIAN_POINT('Ctrl Pts',(8.38951602297935,-10.175952367871,0.326547223819863));
#10302=CARTESIAN_POINT('Ctrl Pts',(8.27632441033917,-10.221573749385,1.41181471663556));
#10303=CARTESIAN_POINT('Ctrl Pts',(7.64792358066077,-10.3075582523984,3.45726320832134));
#10304=CARTESIAN_POINT('Ctrl Pts',(7.14680640941996,-10.3445420065178,4.40073958274844));
#10305=CARTESIAN_POINT('Ctrl Pts',(5.78508544492922,-10.4296237060143,6.09011385799029));
#10306=CARTESIAN_POINT('Ctrl Pts',(4.92173077957157,-10.4761186151316,6.80683464583901));
#10307=CARTESIAN_POINT('Ctrl Pts',(3.0022771914387,-10.567691467586,7.83901819148436));
#10308=CARTESIAN_POINT('Ctrl Pts',(1.97251798521658,-10.6119107462533,8.15924986493847));
#10309=CARTESIAN_POINT('Ctrl Pts',(-0.16749159896407,-10.6947655384569,
8.39463882152912));
#10310=CARTESIAN_POINT('Ctrl Pts',(-1.25808996118376,-10.7335405198673,
8.30153012264513));
#10311=CARTESIAN_POINT('Ctrl Pts',(-3.35478832608991,-10.8225394833933,
7.69880181699771));
#10312=CARTESIAN_POINT('Ctrl Pts',(-4.33903155554408,-10.8690611361328,
7.1901937790795));
#10313=CARTESIAN_POINT('Ctrl Pts',(-6.02187123199346,-10.9585779435994,
5.84600366272615));
#10314=CARTESIAN_POINT('Ctrl Pts',(-6.71423630389552,-11.0005458801513,
5.03555110976292));
#10315=CARTESIAN_POINT('Ctrl Pts',(-7.78196847488304,-11.0794287420123,
3.15904051589254));
#10316=CARTESIAN_POINT('Ctrl Pts',(-8.13147695047584,-11.12387577742,2.10170903930992));
#10317=CARTESIAN_POINT('Ctrl Pts',(-8.39600473501651,-11.2151270044095,
-0.0690272918744915));
#10318=CARTESIAN_POINT('Ctrl Pts',(-8.31569897347412,-11.261012150754,-1.16056937320085));
#10319=CARTESIAN_POINT('Ctrl Pts',(-7.74871382918034,-11.3477530860962,
-3.22401230937071));
#10320=CARTESIAN_POINT('Ctrl Pts',(-7.27798106075176,-11.3851151234394,
-4.17943658060089));
#10321=CARTESIAN_POINT('Ctrl Pts',(-5.96909251183774,-11.4691505252429,
-5.91053942909384));
#10322=CARTESIAN_POINT('Ctrl Pts',(-5.12520597859944,-11.5155315283573,
-6.65556068873632));
#10323=CARTESIAN_POINT('Ctrl Pts',(-3.23165076425933,-11.6074217081022,
-7.74769905945298));
#10324=CARTESIAN_POINT('Ctrl Pts',(-2.20872951052089,-11.6520429968389,
-8.09890090453043));
#10325=CARTESIAN_POINT('Ctrl Pts',(-0.766347204124753,-11.7087709278027,
-8.29957434137255));
#10326=CARTESIAN_POINT('Ctrl Pts',(-0.383003348969663,-11.7232820281137,
-8.326));
#10327=CARTESIAN_POINT('Ctrl Pts',(-1.91097138113605E-13,-11.7372253046546,
-8.32600000000001));
#10328=CARTESIAN_POINT('Origin',(0.,-25.4,0.));
#10329=CARTESIAN_POINT('',(-3.00001195540908E-14,-13.8372253046546,-8.326));
#10330=CARTESIAN_POINT('',(-2.20333979338266E-13,-13.436276920587,-8.326));
#10331=CARTESIAN_POINT('',(-1.01964092497009E-15,-25.4,-8.326));
#10332=CARTESIAN_POINT('Ctrl Pts',(-6.35810848415019E-13,-13.436276920587,
-8.326));
#10333=CARTESIAN_POINT('Ctrl Pts',(-0.244293380369658,-13.4273833948025,
-8.32599999999998));
#10334=CARTESIAN_POINT('Ctrl Pts',(-0.488864284435648,-13.4182537891015,
-8.31524867723662));
#10335=CARTESIAN_POINT('Ctrl Pts',(-1.7952150574658,-13.3682692059687,-8.19979093626448));
#10336=CARTESIAN_POINT('Ctrl Pts',(-2.82947595083118,-13.3243729980939,
-7.90272719891034));
#10337=CARTESIAN_POINT('Ctrl Pts',(-4.76705283660299,-13.2330879564291,
-6.91562734063026));
#10338=CARTESIAN_POINT('Ctrl Pts',(-5.6443386572485,-13.1865359381765,-6.2203189320574));
#10339=CARTESIAN_POINT('Ctrl Pts',(-7.04515688427244,-13.1006929553017,
-4.56244341391435));
#10340=CARTESIAN_POINT('Ctrl Pts',(-7.56903468065117,-13.0637724887533,
-3.62765171586709));
#10341=CARTESIAN_POINT('Ctrl Pts',(-8.2425265460097,-12.9783573924836,-1.59574859717597));
#10342=CARTESIAN_POINT('Ctrl Pts',(-8.37970838905144,-12.9329559048327,
-0.515712065229338));
#10343=CARTESIAN_POINT('Ctrl Pts',(-8.23288905208651,-12.8414603721068,
1.66083595041613));
#10344=CARTESIAN_POINT('Ctrl Pts',(-7.94070750201063,-12.7962736361084,
2.73576384733817));
#10345=CARTESIAN_POINT('Ctrl Pts',(-6.97650406028944,-12.7151826690141,
4.66480211027158));
#10346=CARTESIAN_POINT('Ctrl Pts',(-6.33093644428556,-12.6759595128334,
5.5092335064573));
#10347=CARTESIAN_POINT('Ctrl Pts',(-4.73104640127706,-12.587693759401,6.93757502589118));
#10348=CARTESIAN_POINT('Ctrl Pts',(-3.78217867448249,-12.5413878669107,
7.49718997555689));
#10349=CARTESIAN_POINT('Ctrl Pts',(-1.71192558243361,-12.4507782382054,
8.2223536847459));
#10350=CARTESIAN_POINT('Ctrl Pts',(-0.609468416702,-12.40952625874,8.37650681930984));
#10351=CARTESIAN_POINT('Ctrl Pts',(1.55233521257709,-12.3281418750017,8.24882408974617));
#10352=CARTESIAN_POINT('Ctrl Pts',(2.5919037050054,-12.2847172399287,7.98338947018905));
#10353=CARTESIAN_POINT('Ctrl Pts',(4.55251481294434,-12.1938940018742,7.05815735135888));
#10354=CARTESIAN_POINT('Ctrl Pts',(5.44795676229049,-12.1473023705306,6.39241160247143));
#10355=CARTESIAN_POINT('Ctrl Pts',(6.90163061743603,-12.0604488147846,4.77800454784065));
#10356=CARTESIAN_POINT('Ctrl Pts',(7.45669437328654,-12.0233213068294,3.85480445672747));
#10357=CARTESIAN_POINT('Ctrl Pts',(8.19070822572816,-11.9386883178769,1.84150655381739));
#10358=CARTESIAN_POINT('Ctrl Pts',(8.35983152585037,-11.8936163918223,0.769309821443966));
#10359=CARTESIAN_POINT('Ctrl Pts',(8.27995043713631,-11.8021017440288,-1.40769291435304));
#10360=CARTESIAN_POINT('Ctrl Pts',(8.02080968950356,-11.7565537587041,-2.49121441667634));
#10361=CARTESIAN_POINT('Ctrl Pts',(7.11592151099839,-11.6742411722816,-4.44931325825822));
#10362=CARTESIAN_POINT('Ctrl Pts',(6.49628867115953,-11.6360973086953,-5.3133046025694));
#10363=CARTESIAN_POINT('Ctrl Pts',(4.94296495827753,-11.5485593337285,-6.78767575167891));
#10364=CARTESIAN_POINT('Ctrl Pts',(4.01488982970492,-11.5024345196705,-7.37468934344307));
#10365=CARTESIAN_POINT('Ctrl Pts',(2.04236887930033,-11.4146088993274,-8.13667492393123));
#10366=CARTESIAN_POINT('Ctrl Pts',(1.02513969015335,-11.3735972370578,-8.32600000000002));
#10367=CARTESIAN_POINT('Ctrl Pts',(-1.49047441055927E-13,-11.336276920587,
-8.326));
#10368=CARTESIAN_POINT('Ctrl Pts',(-1.70974345792274E-13,-11.7372253046546,
-8.326));
#10369=CARTESIAN_POINT('Ctrl Pts',(0.688416805123358,-11.7622871896619,
-8.32600000000001));
#10370=CARTESIAN_POINT('Ctrl Pts',(1.37560149155916,-11.7890985396939,-8.24063136044071));
#10371=CARTESIAN_POINT('Ctrl Pts',(3.11270832515499,-11.8615930580718,-7.80030659717876));
#10372=CARTESIAN_POINT('Ctrl Pts',(4.11545846611232,-11.908173194906,-7.32097096414827));
#10373=CARTESIAN_POINT('Ctrl Pts',(5.84334509313178,-11.9983179442442,-6.02492877478023));
#10374=CARTESIAN_POINT('Ctrl Pts',(6.56181117057933,-12.0411124930625,-5.23330616179504));
#10375=CARTESIAN_POINT('Ctrl Pts',(7.68588015961778,-12.1208597058931,-3.38610622472077));
#10376=CARTESIAN_POINT('Ctrl Pts',(8.06641453193172,-12.1638889131946,-2.33928227228454));
#10377=CARTESIAN_POINT('Ctrl Pts',(8.39489220525927,-12.2549263330369,-0.17363210769324));
#10378=CARTESIAN_POINT('Ctrl Pts',(8.34581543744271,-12.301022417095,0.922927880507992));
#10379=CARTESIAN_POINT('Ctrl Pts',(7.83683890332679,-12.388457021665,3.00287221665176));
#10380=CARTESIAN_POINT('Ctrl Pts',(7.39420399893262,-12.4264764337694,3.96973644201845));
#10381=CARTESIAN_POINT('Ctrl Pts',(6.14318644496827,-12.5089591261339,5.72720131525916));
#10382=CARTESIAN_POINT('Ctrl Pts',(5.33108418628558,-12.5545545097282,6.48989702116947));
#10383=CARTESIAN_POINT('Ctrl Pts',(3.48106058093707,-12.6460648708137,7.6393636637798));
#10384=CARTESIAN_POINT('Ctrl Pts',(2.46673345852369,-12.6910872200773,8.02453229494171));
#10385=CARTESIAN_POINT('Ctrl Pts',(0.354198819465129,-12.7756083676375,
8.38678967926924));
#10386=CARTESIAN_POINT('Ctrl Pts',(-0.723663939789811,-12.8127923416359,
8.36301614042901));
#10387=CARTESIAN_POINT('Ctrl Pts',(-2.84695595370087,-12.8997871229495,
7.90170264944797));
#10388=CARTESIAN_POINT('Ctrl Pts',(-3.86880978107385,-12.9463808201591,
7.45481040798338));
#10389=CARTESIAN_POINT('Ctrl Pts',(-5.64429487073648,-13.0371318739719,
6.21236493967363));
#10390=CARTESIAN_POINT('Ctrl Pts',(-6.39039052642516,-13.0804865120355,
5.44195071395798));
#10391=CARTESIAN_POINT('Ctrl Pts',(-7.57502979177055,-13.1617471005116,
3.62765948359466));
#10392=CARTESIAN_POINT('Ctrl Pts',(-7.98880913892081,-13.2032495293137,
2.59237801568459));
#10393=CARTESIAN_POINT('Ctrl Pts',(-8.38590534881367,-13.2939878427895,
0.433843164257152));
#10394=CARTESIAN_POINT('Ctrl Pts',(-8.37057874153018,-13.3402694076479,
-0.667129147202364));
#10395=CARTESIAN_POINT('Ctrl Pts',(-7.9240781663077,-13.4284276948276,-2.76428885879811));
#10396=CARTESIAN_POINT('Ctrl Pts',(-7.51111629860612,-13.4674686056598,
-3.74366776027912));
#10397=CARTESIAN_POINT('Ctrl Pts',(-6.31445379093895,-13.5487426811493,
-5.53777579763203));
#10398=CARTESIAN_POINT('Ctrl Pts',(-5.52602162297095,-13.5939858440471,
-6.3247116488873));
#10399=CARTESIAN_POINT('Ctrl Pts',(-3.70933867906954,-13.6854897128754,
-7.53161712802861));
#10400=CARTESIAN_POINT('Ctrl Pts',(-2.7039832981551,-13.7308447110542,-7.94815175625943));
#10401=CARTESIAN_POINT('Ctrl Pts',(-1.10368897537432,-13.7958920421356,
-8.27112684548052));
#10402=CARTESIAN_POINT('Ctrl Pts',(-0.551922163868698,-13.8171325211826,
-8.32599999999999));
#10403=CARTESIAN_POINT('Ctrl Pts',(-1.69447789133415E-13,-13.8372253046546,
-8.326));
#10404=CARTESIAN_POINT('Origin',(0.,-25.4,0.));
#10405=CARTESIAN_POINT('',(1.31710802876467E-13,-15.9372253046546,-8.326));
#10406=CARTESIAN_POINT('',(-5.24127468637111E-14,-15.536276920587,-8.32600000000001));
#10407=CARTESIAN_POINT('',(-1.01964092497009E-15,-25.4,-8.326));
#10408=CARTESIAN_POINT('Ctrl Pts',(-1.9824419883463E-13,-15.536276920587,
-8.326));
#10409=CARTESIAN_POINT('Ctrl Pts',(-0.415423225689894,-15.5211533950802,
-8.32599999999999));
#10410=CARTESIAN_POINT('Ctrl Pts',(-0.831152842721723,-15.5053652841283,
-8.29491160871503));
#10411=CARTESIAN_POINT('Ctrl Pts',(-2.30456298631406,-15.4470470746465,
-8.07231905411615));
#10412=CARTESIAN_POINT('Ctrl Pts',(-3.32443099059752,-15.4022721166688,
-7.70851768241614));
#10413=CARTESIAN_POINT('Ctrl Pts',(-5.19603470084908,-15.3108059798038,
-6.59853293999313));
#10414=CARTESIAN_POINT('Ctrl Pts',(-6.02375926394927,-15.2649962294663,
-5.85269690189743));
#10415=CARTESIAN_POINT('Ctrl Pts',(-7.31145534060758,-15.1817081186679,
-4.12044158562378));
#10416=CARTESIAN_POINT('Ctrl Pts',(-7.77422058168194,-15.1441900200468,
-3.16181276029789));
#10417=CARTESIAN_POINT('Ctrl Pts',(-8.32487343007585,-15.0572517101063,
-1.09367456439759));
#10418=CARTESIAN_POINT('Ctrl Pts',(-8.39640058252918,-15.0113034100589,
-0.000630146698329115));
#10419=CARTESIAN_POINT('Ctrl Pts',(-8.11382169386083,-14.9200971440347,
2.16903662735235));
#10420=CARTESIAN_POINT('Ctrl Pts',(-7.75547962811613,-14.8758650529199,
3.22339452550135));
#10421=CARTESIAN_POINT('Ctrl Pts',(-6.67192674647674,-14.7971488574488,
5.09171755891762));
#10422=CARTESIAN_POINT('Ctrl Pts',(-5.97213680740976,-14.7547493610765,
5.89689272580657));
#10423=CARTESIAN_POINT('Ctrl Pts',(-4.27672996110017,-14.6650590678691,
7.22756982132451));
#10424=CARTESIAN_POINT('Ctrl Pts',(-3.28721224745853,-14.6185165723781,
7.72803382321316));
#10425=CARTESIAN_POINT('Ctrl Pts',(-1.18669435827851,-14.5297789102049,
8.31171454696549));
#10426=CARTESIAN_POINT('Ctrl Pts',(-0.0978809398525554,-14.4912994342431,
8.39542208880966));
#10427=CARTESIAN_POINT('Ctrl Pts',(2.03857652379367,-14.4082182045706,8.14310743117581));
#10428=CARTESIAN_POINT('Ctrl Pts',(3.06652100905073,-14.3638832033155,7.81422681871336));
#10429=CARTESIAN_POINT('Ctrl Pts',(4.9789354556467,-14.2722139334238,6.76526385610018));
#10430=CARTESIAN_POINT('Ctrl Pts',(5.83695116708594,-14.2257464873203,6.04060234053506));
#10431=CARTESIAN_POINT('Ctrl Pts',(7.18398591264743,-14.1409536612427,4.33953455985475));
#10432=CARTESIAN_POINT('Ctrl Pts',(7.67661647837247,-14.1038984858139,3.39276329165898));
#10433=CARTESIAN_POINT('Ctrl Pts',(8.28800307877674,-14.017702196901,1.34227671597481));
#10434=CARTESIAN_POINT('Ctrl Pts',(8.39210620743553,-13.9720035985342,0.255172344540094));
#10435=CARTESIAN_POINT('Ctrl Pts',(8.17659970973539,-13.8806179549867,-1.91876156453496));
#10436=CARTESIAN_POINT('Ctrl Pts',(7.85084545688346,-13.8358466947024,-2.9838058877545));
#10437=CARTESIAN_POINT('Ctrl Pts',(6.82614140066146,-13.756034658513,-4.88242021150409));
#10438=CARTESIAN_POINT('Ctrl Pts',(6.15347965511124,-13.7153428614236,-5.70697927224458));
#10439=CARTESIAN_POINT('Ctrl Pts',(4.50536797928717,-13.6263423599158,-7.0867556877632));
#10440=CARTESIAN_POINT('Ctrl Pts',(3.53566489294802,-13.5798940837778,-7.61705694325303));
#10441=CARTESIAN_POINT('Ctrl Pts',(1.68355465962175,-13.500260965082,-8.19782418226262));
#10442=CARTESIAN_POINT('Ctrl Pts',(0.843529862891192,-13.4669857125087,
-8.32600000000006));
#10443=CARTESIAN_POINT('Ctrl Pts',(-6.21447338033931E-13,-13.436276920587,
-8.326));
#10444=CARTESIAN_POINT('Ctrl Pts',(-1.22263310586845E-13,-13.8372253046546,
-8.326));
#10445=CARTESIAN_POINT('Ctrl Pts',(0.506006521673632,-13.8556465244225,
-8.32600000000001));
#10446=CARTESIAN_POINT('Ctrl Pts',(1.01207216474324,-13.8750393390131,-8.2798766955888));
#10447=CARTESIAN_POINT('Ctrl Pts',(2.60142913319411,-13.9390688051404,-7.98638465930482));
#10448=CARTESIAN_POINT('Ctrl Pts',(3.63984296492492,-13.9856294345243,-7.56974845942933));
#10449=CARTESIAN_POINT('Ctrl Pts',(5.45736661377731,-14.0768513846503,-6.37771201034996));
#10450=CARTESIAN_POINT('Ctrl Pts',(6.22814566591867,-14.1206802871203,-5.62748653598145));
#10451=CARTESIAN_POINT('Ctrl Pts',(7.46034339023599,-14.202796288597,-3.85487086634778));
#10452=CARTESIAN_POINT('Ctrl Pts',(7.90140763876149,-14.2426981553964,-2.84338012778482));
#10453=CARTESIAN_POINT('Ctrl Pts',(8.36780531265433,-14.332525185874,-0.706523397054396));
#10454=CARTESIAN_POINT('Ctrl Pts',(8.38814146698981,-14.3789555675698,0.397989054372284));
#10455=CARTESIAN_POINT('Ctrl Pts',(8.00755289703476,-14.4678499428711,2.51265925082595));
#10456=CARTESIAN_POINT('Ctrl Pts',(7.62530940326286,-14.5083049882139,3.5054772831053));
#10457=CARTESIAN_POINT('Ctrl Pts',(6.48515189101122,-14.5883047810943,5.33682811766344));
#10458=CARTESIAN_POINT('Ctrl Pts',(5.72193762573087,-14.6331393193333,6.14800146386527));
#10459=CARTESIAN_POINT('Ctrl Pts',(3.94156448946698,-14.724546642076,7.41320398774386));
#10460=CARTESIAN_POINT('Ctrl Pts',(2.9464738700826,-14.770204593253,7.86193134254663));
#10461=CARTESIAN_POINT('Ctrl Pts',(0.86280018710557,-14.8562885270598,8.34853027366915));
#10462=CARTESIAN_POINT('Ctrl Pts',(-0.20417723742401,-14.893302526408,8.39050850143965));
#10463=CARTESIAN_POINT('Ctrl Pts',(-2.34939178007754,-14.978248993173,8.06461889796505));
#10464=CARTESIAN_POINT('Ctrl Pts',(-3.40374961079458,-15.0247314331787,
7.67931854162733));
#10465=CARTESIAN_POINT('Ctrl Pts',(-5.26255306531183,-15.1163502780165,
6.53989769688107));
#10466=CARTESIAN_POINT('Ctrl Pts',(-6.05785492677433,-15.1606241903758,
5.81097467512499));
#10467=CARTESIAN_POINT('Ctrl Pts',(-7.33776083397924,-15.2435854173261,
4.08077858908891));
#10468=CARTESIAN_POINT('Ctrl Pts',(-7.805831728621,-15.282218517097,3.09267575201798));
#10469=CARTESIAN_POINT('Ctrl Pts',(-8.34085273165634,-15.3710950941658,
0.978428950091469));
#10470=CARTESIAN_POINT('Ctrl Pts',(-8.39705642800904,-15.4176269663975,
-0.128497816196545));
#10471=CARTESIAN_POINT('Ctrl Pts',(-8.08279322671259,-15.5072323289714,
-2.26008138417037));
#10472=CARTESIAN_POINT('Ctrl Pts',(-7.73093398441479,-15.5494404810598,
-3.26667650095998));
#10473=CARTESIAN_POINT('Ctrl Pts',(-6.64675040664428,-15.6281612235212,
-5.13412346942883));
#10474=CARTESIAN_POINT('Ctrl Pts',(-5.90907723633758,-15.6725498490239,
-5.96832003585186));
#10475=CARTESIAN_POINT('Ctrl Pts',(-4.16624352443,-15.7637730910409,-7.28978471501692));
#10476=CARTESIAN_POINT('Ctrl Pts',(-3.18223310098026,-15.8096883371853,
-7.76994489155944));
#10477=CARTESIAN_POINT('Ctrl Pts',(-1.43620030413394,-15.8829833267367,
-8.23289356433938));
#10478=CARTESIAN_POINT('Ctrl Pts',(-0.718940118465088,-15.9110522152675,
-8.326));
#10479=CARTESIAN_POINT('Ctrl Pts',(2.76445533131664E-13,-15.9372253046546,
-8.32600000000001));
#10480=CARTESIAN_POINT('Origin',(0.,-25.4,0.));
#10481=CARTESIAN_POINT('',(1.72372721153364E-13,-18.0372253046546,-8.326));
#10482=CARTESIAN_POINT('',(-1.03630498060333E-14,-17.636276920587,-8.326));
#10483=CARTESIAN_POINT('',(-1.01964092497009E-15,-25.4,-8.326));
#10484=CARTESIAN_POINT('Ctrl Pts',(-2.12052597703405E-13,-17.636276920587,
-8.326));
#10485=CARTESIAN_POINT('Ctrl Pts',(-0.575058079507399,-17.6153418717128,
-8.32599999999999));
#10486=CARTESIAN_POINT('Ctrl Pts',(-1.14982045747753,-17.5931655233299,
-8.26643034587313));
#10487=CARTESIAN_POINT('Ctrl Pts',(-2.77096762089726,-17.5269746993386,
-7.92516931059649));
#10488=CARTESIAN_POINT('Ctrl Pts',(-3.77359980056906,-17.4815322151829,
-7.49975562662993));
#10489=CARTESIAN_POINT('Ctrl Pts',(-5.58048141429174,-17.3900458012541,
-6.27670419988311));
#10490=CARTESIAN_POINT('Ctrl Pts',(-6.3620523412699,-17.3449105381877,-5.48301789632078));
#10491=CARTESIAN_POINT('Ctrl Pts',(-7.54320702466148,-17.2639844312338,
-3.67860486814112));
#10492=CARTESIAN_POINT('Ctrl Pts',(-7.94772870978091,-17.2245911121536,
-2.69558273995902));
#10493=CARTESIAN_POINT('Ctrl Pts',(-8.37624041010279,-17.1362290890949,
-0.593576442852489));
#10494=CARTESIAN_POINT('Ctrl Pts',(-8.38183638881273,-17.0899021394706,
0.508475507353455));
#10495=CARTESIAN_POINT('Ctrl Pts',(-7.96571678629875,-16.9994090296343,
2.66117731448738));
#10496=CARTESIAN_POINT('Ctrl Pts',(-7.54444213160671,-16.9583766883461,
3.68991327890768));
#10497=CARTESIAN_POINT('Ctrl Pts',(-6.34680823611166,-16.8768811055922,
5.49287750595405));
#10498=CARTESIAN_POINT('Ctrl Pts',(-5.5939483096094,-16.833393974563,6.2578793076948));
#10499=CARTESIAN_POINT('Ctrl Pts',(-3.80689607512934,-16.7425070311971,
7.48675513016755));
#10500=CARTESIAN_POINT('Ctrl Pts',(-2.78045510064503,-16.6959180237583,
7.9254790738769));
#10501=CARTESIAN_POINT('Ctrl Pts',(-0.654016405705544,-16.6091923630911,
8.36853836200114));
#10502=CARTESIAN_POINT('Ctrl Pts',(0.422300111506851,-16.5721100296044,
8.38342505306291));
#10503=CARTESIAN_POINT('Ctrl Pts',(2.53109525486195,-16.4873763282887,8.0045779717921));
#10504=CARTESIAN_POINT('Ctrl Pts',(3.54309116781857,-16.4422602642142,7.6109128844606));
#10505=CARTESIAN_POINT('Ctrl Pts',(5.38427974268193,-16.350743224854,6.44582578693569));
#10506=CARTESIAN_POINT('Ctrl Pts',(6.19005720279719,-16.3052388201027,5.67650372197135));
#10507=CARTESIAN_POINT('Ctrl Pts',(7.42641387110462,-16.2230803922604,3.90907302938784));
#10508=CARTESIAN_POINT('Ctrl Pts',(7.8610288922322,-16.1848182227143,2.93887109003904));
#10509=CARTESIAN_POINT('Ctrl Pts',(8.35324018828346,-16.0971869998293,0.854249485064087));
#10510=CARTESIAN_POINT('Ctrl Pts',(8.39326929677321,-16.0510368938999,-0.243595606274021));
#10511=CARTESIAN_POINT('Ctrl Pts',(8.04488101332369,-15.9596881118743,-2.41665263240238));
#10512=CARTESIAN_POINT('Ctrl Pts',(7.65032609785298,-15.9168802102447,-3.46873641199449));
#10513=CARTESIAN_POINT('Ctrl Pts',(6.49875765868641,-15.8362219575584,-5.31165057763646));
#10514=CARTESIAN_POINT('Ctrl Pts',(5.76993233127877,-15.7932139260652,-6.09548733907829));
#10515=CARTESIAN_POINT('Ctrl Pts',(4.02413471964635,-15.7028324013838,-7.37177188741203));
#10516=CARTESIAN_POINT('Ctrl Pts',(3.01415431952855,-15.6562411476875,-7.83911325276364));
#10517=CARTESIAN_POINT('Ctrl Pts',(1.3048478767382,-15.5853938080833,-8.24922164553926));
#10518=CARTESIAN_POINT('Ctrl Pts',(0.652861729446362,-15.560044419386,-8.32600000000001));
#10519=CARTESIAN_POINT('Ctrl Pts',(-1.69170233377258E-13,-15.536276920587,
-8.326));
#10520=CARTESIAN_POINT('Ctrl Pts',(2.71588307398929E-13,-15.9372253046546,
-8.326));
#10521=CARTESIAN_POINT('Ctrl Pts',(0.332370296269366,-15.949325279674,-8.326));
#10522=CARTESIAN_POINT('Ctrl Pts',(0.665068926132207,-15.9618554937788,
-8.30609914404716));
#10523=CARTESIAN_POINT('Ctrl Pts',(2.09179478361076,-16.0174100114443,-8.13413559434496));
#10524=CARTESIAN_POINT('Ctrl Pts',(3.15009218418154,-16.063262048947,-7.78565152309358));
#10525=CARTESIAN_POINT('Ctrl Pts',(5.04218002261011,-16.1547139850303,-6.71182196403841));
#10526=CARTESIAN_POINT('Ctrl Pts',(5.86385151991641,-16.1994350303207,-6.00729918400101));
#10527=CARTESIAN_POINT('Ctrl Pts',(7.19573372747264,-16.2833021503588,-4.32402888611314));
#10528=CARTESIAN_POINT('Ctrl Pts',(7.69290123095891,-16.320946271798,-3.36082636447661));
#10529=CARTESIAN_POINT('Ctrl Pts',(8.30165570219128,-16.4087500355188,-1.27210025950698));
#10530=CARTESIAN_POINT('Ctrl Pts',(8.39694883678225,-16.4553381700915,-0.163835092499947));
#10531=CARTESIAN_POINT('Ctrl Pts',(8.15529886321142,-16.5456372268563,1.984250469281));
#10532=CARTESIAN_POINT('Ctrl Pts',(7.83665298720733,-16.5885702247514,3.00556515635138));
#10533=CARTESIAN_POINT('Ctrl Pts',(6.8077136801888,-16.6691002127173,4.92125852722286));
#10534=CARTESIAN_POINT('Ctrl Pts',(6.08870950300239,-16.7122042267477,5.78723709941025));
#10535=CARTESIAN_POINT('Ctrl Pts',(4.37319166116847,-16.8036796223934,7.16801100261096));
#10536=CARTESIAN_POINT('Ctrl Pts',(3.40044148216312,-16.849798978357,7.67738545666204));
#10537=CARTESIAN_POINT('Ctrl Pts',(1.34649982119402,-16.9373171129223,8.2837169348852));
#10538=CARTESIAN_POINT('Ctrl Pts',(0.288331930262472,-16.97543654558,8.3874699219568));
#10539=CARTESIAN_POINT('Ctrl Pts',(-1.85974418193972,-17.0577818452421,
8.1902928011815));
#10540=CARTESIAN_POINT('Ctrl Pts',(-2.92741157807384,-17.1033390022504,
7.8720676097236));
#10541=CARTESIAN_POINT('Ctrl Pts',(-4.85177226945907,-17.1948529603484,
6.85118544144144));
#10542=CARTESIAN_POINT('Ctrl Pts',(-5.6951352910351,-17.2399154235644,6.16798979411118));
#10543=CARTESIAN_POINT('Ctrl Pts',(-7.0704344504019,-17.3245269623444,4.52450254583816));
#10544=CARTESIAN_POINT('Ctrl Pts',(-7.59171871260332,-17.3616647877063,
3.5816196117483));
#10545=CARTESIAN_POINT('Ctrl Pts',(-8.26124523219371,-17.4485454946569,
1.51485170868987));
#10546=CARTESIAN_POINT('Ctrl Pts',(-8.38913173063085,-17.4951375912553,
0.406492290752532));
#10547=CARTESIAN_POINT('Ctrl Pts',(-8.20833131569507,-17.5859471021696,
-1.75373624602508));
#10548=CARTESIAN_POINT('Ctrl Pts',(-7.91760598460155,-17.6293583608581,
-2.78642807414316));
#10549=CARTESIAN_POINT('Ctrl Pts',(-6.94563509800759,-17.7107190270286,
-4.72188209281742));
#10550=CARTESIAN_POINT('Ctrl Pts',(-6.25995560544519,-17.7520185073925,
-5.59923662458799));
#10551=CARTESIAN_POINT('Ctrl Pts',(-4.59534922424053,-17.842652874823,-7.02817804474219));
#10552=CARTESIAN_POINT('Ctrl Pts',(-3.63587814624271,-17.8889541784923,
-7.56920912840256));
#10553=CARTESIAN_POINT('Ctrl Pts',(-1.75941205318623,-17.9702285311227,
-8.18587600226779));
#10554=CARTESIAN_POINT('Ctrl Pts',(-0.881962201508673,-18.0051173794697,
-8.32600000000001));
#10555=CARTESIAN_POINT('Ctrl Pts',(2.67563748934663E-13,-18.0372253046546,
-8.32600000000001));
#10556=CARTESIAN_POINT('Origin',(0.,-25.4,0.));
#10557=CARTESIAN_POINT('',(3.96816528613292E-9,-20.1372253049435,-8.326));
#10558=CARTESIAN_POINT('',(1.34659832785628E-13,-19.736276920587,-8.326));
#10559=CARTESIAN_POINT('',(-1.01964092497009E-15,-25.4,-8.326));
#10560=CARTESIAN_POINT('Ctrl Pts',(3.03784775113058E-13,-19.736276920587,
-8.326));
#10561=CARTESIAN_POINT('Ctrl Pts',(-0.741011693602677,-19.7093003132238,
-8.326));
#10562=CARTESIAN_POINT('Ctrl Pts',(-1.48004434879021,-19.68031679053,-8.22708890753572));
#10563=CARTESIAN_POINT('Ctrl Pts',(-3.2444565536996,-19.6059354644762,-7.74428951636322));
#10564=CARTESIAN_POINT('Ctrl Pts',(-4.22535623213429,-19.5599586218775,
-7.25581078810072));
#10565=CARTESIAN_POINT('Ctrl Pts',(-5.95826066548303,-19.4687804626706,
-5.91929300528484));
#10566=CARTESIAN_POINT('Ctrl Pts',(-6.6889796239238,-19.4247794053195,-5.07891910823867));
#10567=CARTESIAN_POINT('Ctrl Pts',(-7.75818481398095,-19.3458715811982,
-3.20181469785529));
#10568=CARTESIAN_POINT('Ctrl Pts',(-8.10174283459321,-19.3033982210791,
-2.19143413684825));
#10569=CARTESIAN_POINT('Ctrl Pts',(-8.39797991796542,-19.2136214509322,
-0.0557730275832109));
#10570=CARTESIAN_POINT('Ctrl Pts',(-8.3320695963325,-19.1670703405566,1.05161138666675));
#10571=CARTESIAN_POINT('Ctrl Pts',(-7.77864352391814,-19.078456621778,3.15960516538214));
#10572=CARTESIAN_POINT('Ctrl Pts',(-7.30332110660647,-19.040107635104,4.14146876881184));
#10573=CARTESIAN_POINT('Ctrl Pts',(-6.01051168074491,-18.9569200440293,
5.86008506322163));
#10574=CARTESIAN_POINT('Ctrl Pts',(-5.2086265645188,-18.9125313569302,6.58306620743989));
#10575=CARTESIAN_POINT('Ctrl Pts',(-3.3388282817735,-18.8208186777339,7.70790782175316));
#10576=CARTESIAN_POINT('Ctrl Pts',(-2.28028135621384,-18.7743653587606,
8.08456695747027));
#10577=CARTESIAN_POINT('Ctrl Pts',(-0.132301086442923,-18.6897097506465,
8.39182795746986));
#10578=CARTESIAN_POINT('Ctrl Pts',(0.933296066553777,-18.652611722947,8.34082228835986));
#10579=CARTESIAN_POINT('Ctrl Pts',(3.01278616610347,-18.5663156313633,7.83688331731904));
#10580=CARTESIAN_POINT('Ctrl Pts',(4.0048717208109,-18.5205815362637,7.37932832753217));
#10581=CARTESIAN_POINT('Ctrl Pts',(5.77491249608914,-18.4292168573335,6.09825850022494));
#10582=CARTESIAN_POINT('Ctrl Pts',(6.53104614376202,-18.3845028252529,5.28055450329049));
#10583=CARTESIAN_POINT('Ctrl Pts',(7.65556865793812,-18.3048586762036,3.43904357504579));
#10584=CARTESIAN_POINT('Ctrl Pts',(8.02932411892815,-18.2639491185334,2.4424249145819));
#10585=CARTESIAN_POINT('Ctrl Pts',(8.39149230014016,-18.1748542313203,0.322984826192618));
#10586=CARTESIAN_POINT('Ctrl Pts',(8.36118956244984,-18.1283908287504,-0.78231314465672));
#10587=CARTESIAN_POINT('Ctrl Pts',(7.87562154473628,-18.038824561216,-2.91296669748745));
#10588=CARTESIAN_POINT('Ctrl Pts',(7.42701502102502,-17.9993096945417,-3.91790521670791));
#10589=CARTESIAN_POINT('Ctrl Pts',(6.18155268726809,-17.9169573879563,-5.67878863076229));
#10590=CARTESIAN_POINT('Ctrl Pts',(5.40392870253753,-17.8730015678831,-6.4231967110492));
#10591=CARTESIAN_POINT('Ctrl Pts',(3.5748326958408,-17.7816615041576,-7.60080875598084));
#10592=CARTESIAN_POINT('Ctrl Pts',(2.5319159568273,-17.7351180128823,-8.00883030942075));
#10593=CARTESIAN_POINT('Ctrl Pts',(0.963266230846582,-17.6722227700236,
-8.28422523926223));
#10594=CARTESIAN_POINT('Ctrl Pts',(0.481561790093202,-17.6538082273729,
-8.32600000000001));
#10595=CARTESIAN_POINT('Ctrl Pts',(-1.88044024795886E-13,-17.636276920587,
-8.326));
#10596=CARTESIAN_POINT('Ctrl Pts',(2.95805047123565E-13,-18.0372253046546,
-8.326));
#10597=CARTESIAN_POINT('Ctrl Pts',(0.168981087311088,-18.0433770786193,
-8.326));
#10598=CARTESIAN_POINT('Ctrl Pts',(0.338120011567569,-18.0496427233294,
-8.3208557368868));
#10599=CARTESIAN_POINT('Ctrl Pts',(1.60830093220243,-18.0975131031637,-8.24333772622879));
#10600=CARTESIAN_POINT('Ctrl Pts',(2.68506258215882,-18.1427107214706,-7.9579700686103));
#10601=CARTESIAN_POINT('Ctrl Pts',(4.642501116715,-18.2342079995147,-6.99517399461026));
#10602=CARTESIAN_POINT('Ctrl Pts',(5.5086104621158,-18.2796006496375,-6.33566678619455));
#10603=CARTESIAN_POINT('Ctrl Pts',(6.93023001768936,-18.3649937606886,-4.73522384198799));
#10604=CARTESIAN_POINT('Ctrl Pts',(7.47711943818315,-18.4019154738673,-3.813541860389));
#10605=CARTESIAN_POINT('Ctrl Pts',(8.21066834594864,-18.4877874049101,-1.77077129506958));
#10606=CARTESIAN_POINT('Ctrl Pts',(8.37319984712582,-18.534341145119,-0.663324320842134));
#10607=CARTESIAN_POINT('Ctrl Pts',(8.25742001501766,-18.6256142494957,1.50793244212956));
#10608=CARTESIAN_POINT('Ctrl Pts',(7.9967003642083,-18.6694976394034,2.55185559747756));
#10609=CARTESIAN_POINT('Ctrl Pts',(7.08483442339588,-18.7517146642827,4.50768116646479));
#10610=CARTESIAN_POINT('Ctrl Pts',(6.43342871760873,-18.7914480807177,5.39679016863165));
#10611=CARTESIAN_POINT('Ctrl Pts',(4.82243930383149,-18.8811641058222,6.87490679647979));
#10612=CARTESIAN_POINT('Ctrl Pts',(3.87789919103356,-18.9276090400981,7.44863260436268));
#10613=CARTESIAN_POINT('Ctrl Pts',(1.85840928867414,-19.0165892949646,8.18419978535578));
#10614=CARTESIAN_POINT('Ctrl Pts',(0.807893080887373,-19.0572352662045,
8.35352848045677));
#10615=CARTESIAN_POINT('Ctrl Pts',(-1.3486079894212,-19.1370832046557,8.28976112626951));
#10616=CARTESIAN_POINT('Ctrl Pts',(-2.43362679443577,-19.1818666240449,
8.03840168180975));
#10617=CARTESIAN_POINT('Ctrl Pts',(-4.42319592982404,-19.2732565577242,
7.13636457911092));
#10618=CARTESIAN_POINT('Ctrl Pts',(-5.31198409205434,-19.3189474613863,
6.50194818245679));
#10619=CARTESIAN_POINT('Ctrl Pts',(-6.78075924333669,-19.4051223267751,
4.94598748806984));
#10620=CARTESIAN_POINT('Ctrl Pts',(-7.3536522617107,-19.442169075152,4.04539476239995));
#10621=CARTESIAN_POINT('Ctrl Pts',(-8.15153415864958,-19.5269912651094,
2.02759603787036));
#10622=CARTESIAN_POINT('Ctrl Pts',(-8.3491344671574,-19.5734616444342,0.922132099992329));
#10623=CARTESIAN_POINT('Ctrl Pts',(-8.29952591628968,-19.6651214263525,
-1.25832316929844));
#10624=CARTESIAN_POINT('Ctrl Pts',(-8.06952074714483,-19.7094448324464,
-2.31271368112304));
#10625=CARTESIAN_POINT('Ctrl Pts',(-7.21813885438952,-19.7925032020478,
-4.28855363912642));
#10626=CARTESIAN_POINT('Ctrl Pts',(-6.60032745014865,-19.8310114214651,
-5.18932082489098));
#10627=CARTESIAN_POINT('Ctrl Pts',(-5.04311010714147,-19.9197756220679,
-6.71528832105067));
#10628=CARTESIAN_POINT('Ctrl Pts',(-4.11448679814829,-19.9663161675756,
-7.32113175104967));
#10629=CARTESIAN_POINT('Ctrl Pts',(-2.11386189931371,-20.0559877100324,
-8.12226356506916));
#10630=CARTESIAN_POINT('Ctrl Pts',(-1.06658045254075,-20.0983712645419,
-8.32480731712692));
#10631=CARTESIAN_POINT('Ctrl Pts',(-0.00623416757088782,-20.1369983123485,
-8.32599824958923));
#10632=CARTESIAN_POINT('Ctrl Pts',(-0.00311703891250096,-20.1371118285306,
-8.32600000000297));
#10633=CARTESIAN_POINT('Ctrl Pts',(7.93618616483201E-9,-20.1372253049435,
-8.326));
#10634=CARTESIAN_POINT('Origin',(0.,-25.4,0.));
#10635=CARTESIAN_POINT('',(-1.37067252491379E-13,-22.2372253046546,-8.32600000000001));
#10636=CARTESIAN_POINT('',(1.39802199830121E-13,-21.836276920587,-8.326));
#10637=CARTESIAN_POINT('',(-1.01964092497009E-15,-25.4,-8.326));
#10638=CARTESIAN_POINT('Ctrl Pts',(3.3056890558214E-13,-21.836276920587,
-8.32600000000001));
#10639=CARTESIAN_POINT('Ctrl Pts',(-0.908108585131477,-21.8032171336015,
-8.326));
#10640=CARTESIAN_POINT('Ctrl Pts',(-1.81110815181515,-21.7672208890341,
-8.17744265861093));
#10641=CARTESIAN_POINT('Ctrl Pts',(-3.70730244560357,-21.6846788454566,
-7.53463291746772));
#10642=CARTESIAN_POINT('Ctrl Pts',(-4.66250514039434,-21.6383304747457,
-6.98396946186045));
#10643=CARTESIAN_POINT('Ctrl Pts',(-6.31142773900649,-21.5479614016373,
-5.54048487926333));
#10644=CARTESIAN_POINT('Ctrl Pts',(-6.98699738054398,-21.5071555424562,
-4.65967258766987));
#10645=CARTESIAN_POINT('Ctrl Pts',(-7.94140241989562,-21.4255424931981,
-2.7182147358875));
#10646=CARTESIAN_POINT('Ctrl Pts',(-8.22341469315457,-21.3819897412754,
-1.68215698586221));
#10647=CARTESIAN_POINT('Ctrl Pts',(-8.3852952316952,-21.2910366853893,0.481486280730521));
#10648=CARTESIAN_POINT('Ctrl Pts',(-8.24730836793455,-21.2444512489582,
1.58968726280175));
#10649=CARTESIAN_POINT('Ctrl Pts',(-7.55906152604825,-21.1578617658357,
3.64952736702381));
#10650=CARTESIAN_POINT('Ctrl Pts',(-7.03031309405226,-21.1208213621961,
4.58619078151074));
#10651=CARTESIAN_POINT('Ctrl Pts',(-5.64153242231531,-21.0359810148221,
6.21721342455858));
#10652=CARTESIAN_POINT('Ctrl Pts',(-4.79150414422494,-20.990818741746,6.89361317693311));
#10653=CARTESIAN_POINT('Ctrl Pts',(-2.85736689459058,-20.8993007037906,
7.89775595756132));
#10654=CARTESIAN_POINT('Ctrl Pts',(-1.78695446083802,-20.8538433842544,
8.20647662272373));
#10655=CARTESIAN_POINT('Ctrl Pts',(0.362500134543461,-20.7718492172337,
8.38456025275674));
#10656=CARTESIAN_POINT('Ctrl Pts',(1.4194733277575,-20.7334552437087,8.27149545687334));
#10657=CARTESIAN_POINT('Ctrl Pts',(3.46870639771315,-20.6457251120916,7.64692224576267));
#10658=CARTESIAN_POINT('Ctrl Pts',(4.43772923043642,-20.5995488348411,7.12838368637743));
#10659=CARTESIAN_POINT('Ctrl Pts',(6.13860673557218,-20.508312040779,5.73360395780598));
#10660=CARTESIAN_POINT('Ctrl Pts',(6.84794643020952,-20.4657585990833,4.86432701474728));
#10661=CARTESIAN_POINT('Ctrl Pts',(7.86050887218106,-20.3849878927729,2.94290729834406));
#10662=CARTESIAN_POINT('Ctrl Pts',(8.17118244694402,-20.3419144199962,1.91825091451713));
#10663=CARTESIAN_POINT('Ctrl Pts',(8.39542277107465,-20.2514616608006,-0.233491008519554));
#10664=CARTESIAN_POINT('Ctrl Pts',(8.2907872614984,-20.2048684103033,-1.34187787606265));
#10665=CARTESIAN_POINT('Ctrl Pts',(7.66455310005366,-20.1173266040453,-3.42437238721642));
#10666=CARTESIAN_POINT('Ctrl Pts',(7.16046463414603,-20.0798574060706,-4.38171071135767));
#10667=CARTESIAN_POINT('Ctrl Pts',(5.8161487017165,-19.9957759382129,-6.05364322287303));
#10668=CARTESIAN_POINT('Ctrl Pts',(4.98823156595436,-19.9509540545005,-6.75214584378655));
#10669=CARTESIAN_POINT('Ctrl Pts',(3.0867817751318,-19.8594768129244,-7.81096398868598));
#10670=CARTESIAN_POINT('Ctrl Pts',(2.02571973403472,-19.8137050882996,-8.15083850481592));
#10671=CARTESIAN_POINT('Ctrl Pts',(0.620131098081054,-19.7592165139285,
-8.30869825973521));
#10672=CARTESIAN_POINT('Ctrl Pts',(0.309905806485666,-19.7475590735318,
-8.326));
#10673=CARTESIAN_POINT('Ctrl Pts',(3.26197402422679E-13,-19.736276920587,
-8.326));
#10674=CARTESIAN_POINT('Ctrl Pts',(7.93620114070137E-9,-20.1372253049435,
-8.32599999999999));
#10675=CARTESIAN_POINT('Ctrl Pts',(1.09929152081772,-20.1772451262137,-8.32599999895217));
#10676=CARTESIAN_POINT('Ctrl Pts',(2.18807547233758,-20.2214584908025,-8.10828355822521));
#10677=CARTESIAN_POINT('Ctrl Pts',(4.20468880037571,-20.3125406121911,-7.2677332005755));
#10678=CARTESIAN_POINT('Ctrl Pts',(5.11496013298754,-20.3584826994036,-6.65857615086658));
#10679=CARTESIAN_POINT('Ctrl Pts',(6.62946625597013,-20.4454012489607,-5.1464414550283));
#10680=CARTESIAN_POINT('Ctrl Pts',(7.22760191635294,-20.4829026282789,-4.26583029573217));
#10681=CARTESIAN_POINT('Ctrl Pts',(8.08233451684404,-20.566222427601,-2.28377129814597));
#10682=CARTESIAN_POINT('Ctrl Pts',(8.31349443187262,-20.6120402658695,-1.19383037979337));
#10683=CARTESIAN_POINT('Ctrl Pts',(8.33718568320761,-20.7035038407883,0.981957405275777));
#10684=CARTESIAN_POINT('Ctrl Pts',(8.14147282185833,-20.7482686311639,2.04684781861082));
#10685=CARTESIAN_POINT('Ctrl Pts',(7.35656369922082,-20.8322282201805,4.04412649904621));
#10686=CARTESIAN_POINT('Ctrl Pts',(6.77467342822941,-20.8697940363974,4.95760578517001));
#10687=CARTESIAN_POINT('Ctrl Pts',(5.27625057320422,-20.9574851722186,6.53435496530883));
#10688=CARTESIAN_POINT('Ctrl Pts',(4.36607083693896,-21.0040759043001,7.17453133414064));
#10689=CARTESIAN_POINT('Ctrl Pts',(2.38731926118937,-21.0944419268729,8.04659023476296));
#10690=CARTESIAN_POINT('Ctrl Pts',(1.34397410464132,-21.1374357954337,8.28498884029207));
#10691=CARTESIAN_POINT('Ctrl Pts',(-0.828146017691834,-21.2180697833976,
8.3591011927717));
#10692=CARTESIAN_POINT('Ctrl Pts',(-1.93675392260759,-21.260933224618,8.173743957929));
#10693=CARTESIAN_POINT('Ctrl Pts',(-3.99238573558019,-21.3523060506757,
7.38694470104383));
#10694=CARTESIAN_POINT('Ctrl Pts',(-4.92252070723055,-21.3984504126804,
6.80256882669288));
#10695=CARTESIAN_POINT('Ctrl Pts',(-6.48039524342482,-21.486060263998,5.33266026336641));
#10696=CARTESIAN_POINT('Ctrl Pts',(-7.10255463824954,-21.5242948102021,
4.47059799089661));
#10697=CARTESIAN_POINT('Ctrl Pts',(-8.01327983054783,-21.606488629631,2.51532444642886));
#10698=CARTESIAN_POINT('Ctrl Pts',(-8.27567542750925,-21.6520030919063,
1.43260040955898));
#10699=CARTESIAN_POINT('Ctrl Pts',(-8.36212210043179,-21.7435197071686,
-0.744449129507846));
#10700=CARTESIAN_POINT('Ctrl Pts',(-8.1961189482673,-21.7886257042918,-1.81745636394051));
#10701=CARTESIAN_POINT('Ctrl Pts',(-7.46804495038655,-21.8733363379352,
-3.83260132312565));
#10702=CARTESIAN_POINT('Ctrl Pts',(-6.916075171964,-21.910428541569,-4.75693730423157));
#10703=CARTESIAN_POINT('Ctrl Pts',(-5.46760684795329,-21.997183556465,-6.37567231116854));
#10704=CARTESIAN_POINT('Ctrl Pts',(-4.57391746847598,-22.043773228963,-7.04436040383322));
#10705=CARTESIAN_POINT('Ctrl Pts',(-2.61549840024866,-22.1346456897299,
-7.97573112283634));
#10706=CARTESIAN_POINT('Ctrl Pts',(-1.57641225491258,-22.1781185513746,
-8.24429567455344));
#10707=CARTESIAN_POINT('Ctrl Pts',(-0.343231816087832,-22.2246185042882,
-8.32069940223016));
#10708=CARTESIAN_POINT('Ctrl Pts',(-0.17152966831258,-22.2309807493349,
-8.326));
#10709=CARTESIAN_POINT('Ctrl Pts',(-1.23893950654264E-13,-22.2372253046546,
-8.326));
#10710=CARTESIAN_POINT('Origin',(0.,-25.4,0.));
#10711=CARTESIAN_POINT('',(-1.64753439167969E-13,-24.3372253046546,-8.326));
#10712=CARTESIAN_POINT('',(-1.89759924326649E-15,-23.936276920587,-8.326));
#10713=CARTESIAN_POINT('',(-1.01964092497009E-15,-25.4,-8.326));
#10714=CARTESIAN_POINT('',(8.27736571547526,-24.9,0.898606038414384));
#10715=CARTESIAN_POINT('Ctrl Pts',(-1.50296441958631E-13,-24.3372253046546,
-8.326));
#10716=CARTESIAN_POINT('Ctrl Pts',(0.742893768952232,-24.3642704291657,
-8.32600000000001));
#10717=CARTESIAN_POINT('Ctrl Pts',(1.48389594827494,-24.3933362330634,-8.22658551882158));
#10718=CARTESIAN_POINT('Ctrl Pts',(3.262585844936,-24.4683481831947,-7.73851252336228));
#10719=CARTESIAN_POINT('Ctrl Pts',(4.25400469153752,-24.51489739812,-7.24102168886792));
#10720=CARTESIAN_POINT('Ctrl Pts',(5.95405524569837,-24.6046545861794,-5.91520506535258));
#10721=CARTESIAN_POINT('Ctrl Pts',(6.65650698446997,-24.6471111704798,-5.11192419028058));
#10722=CARTESIAN_POINT('Ctrl Pts',(7.62856775351797,-24.7174862679998,-3.44733676201697));
#10723=CARTESIAN_POINT('Ctrl Pts',(7.94693649975717,-24.7515948625903,-2.63174017322248));
#10724=CARTESIAN_POINT('Ctrl Pts',(8.32586411060715,-24.8243159404673,-0.901809617782638));
#10725=CARTESIAN_POINT('Ctrl Pts',(8.37455760848785,-24.8623656438899,0.00333846992109366));
#10726=CARTESIAN_POINT('Ctrl Pts',(8.27736571547527,-24.9,0.898606038414273));
#10727=CARTESIAN_POINT('',(2.19919404320626,-24.9,8.03030644249185));
#10728=CARTESIAN_POINT('Origin',(0.,-24.9,0.));
#10729=CARTESIAN_POINT('Ctrl Pts',(2.19919404320625,-24.9,8.03030644249185));
#10730=CARTESIAN_POINT('Ctrl Pts',(2.94095280141566,-24.8687265114472,7.82716706615144));
#10731=CARTESIAN_POINT('Ctrl Pts',(3.65097101877844,-24.8364691142525,7.52223989839009));
#10732=CARTESIAN_POINT('Ctrl Pts',(4.96518040040976,-24.7719179658425,6.7273581096632));
#10733=CARTESIAN_POINT('Ctrl Pts',(5.56341734142977,-24.7399313157154,6.24170146387279));
#10734=CARTESIAN_POINT('Ctrl Pts',(6.81761446664068,-24.666028411966,4.89794559820416));
#10735=CARTESIAN_POINT('Ctrl Pts',(7.39050128363734,-24.6286357804595,3.98122819228775));
#10736=CARTESIAN_POINT('Ctrl Pts',(8.1584498305441,-24.5444501764425,1.97857293787148));
#10737=CARTESIAN_POINT('Ctrl Pts',(8.34533182165618,-24.4995800271944,0.911176187470449));
#10738=CARTESIAN_POINT('Ctrl Pts',(8.30293131992899,-24.4080926332995,-1.26517821701211));
#10739=CARTESIAN_POINT('Ctrl Pts',(8.06242989867319,-24.3623612521532,-2.3530624439374));
#10740=CARTESIAN_POINT('Ctrl Pts',(7.19095506233322,-24.2793749941559,-4.32718696989518));
#10741=CARTESIAN_POINT('Ctrl Pts',(6.58568461817839,-24.2416861622831,-5.2022412392326));
#10742=CARTESIAN_POINT('Ctrl Pts',(5.0582780140935,-24.1545605163226,-6.70188470152501));
#10743=CARTESIAN_POINT('Ctrl Pts',(4.1420442351946,-24.1085545504541,-7.30375365526574));
#10744=CARTESIAN_POINT('Ctrl Pts',(2.13977222107689,-24.0185490972115,-8.11791910308778));
#10745=CARTESIAN_POINT('Ctrl Pts',(1.07469957386274,-23.9754014697511,-8.32600000000002));
#10746=CARTESIAN_POINT('Ctrl Pts',(-1.75692793646931E-13,-23.936276920587,
-8.326));
#10747=CARTESIAN_POINT('Origin',(0.,-24.4,0.));
#10748=CARTESIAN_POINT('',(2.33295215237571E-15,-24.4,19.05));
#10749=CARTESIAN_POINT('',(-2.33295215237571E-15,-24.4,-19.05));
#10750=CARTESIAN_POINT('Origin',(0.,-24.4,0.));
#10751=CARTESIAN_POINT('Origin',(0.,-24.4,0.));
#10752=CARTESIAN_POINT('',(-2.21048747246097E-15,-25.4,-18.05));
#10753=CARTESIAN_POINT('Origin',(-2.21048747246097E-15,-24.4,-18.05));
#10754=CARTESIAN_POINT('Origin',(0.,-25.4,0.));
#10755=CARTESIAN_POINT('Origin',(0.,14.4,0.));
#10756=CARTESIAN_POINT('',(-2.21048747246097E-15,15.4,-18.05));
#10757=CARTESIAN_POINT('Origin',(0.,15.4,0.));
#10758=CARTESIAN_POINT('',(-2.33295215237571E-15,14.4,-19.05));
#10759=CARTESIAN_POINT('Origin',(-2.21048747246097E-15,14.4,-18.05));
#10760=CARTESIAN_POINT('',(2.33295215237571E-15,14.4,19.05));
#10761=CARTESIAN_POINT('Origin',(0.,14.4,0.));
#10762=CARTESIAN_POINT('Origin',(0.,14.4,0.));
#10763=CARTESIAN_POINT('Origin',(17.3316043908594,-21.9,45.4192193816532));
#10764=CARTESIAN_POINT('',(19.3316043908594,-22.9,48.883320996791));
#10765=CARTESIAN_POINT('',(13.8675027757216,-22.9,47.4192193816532));
#10766=CARTESIAN_POINT('Origin',(17.3316043908594,-22.9,45.4192193816532));
#10767=CARTESIAN_POINT('',(19.8316043908594,-21.9,49.7493464005754));
#10768=CARTESIAN_POINT('Origin',(19.3316043908594,-21.9,48.883320996791));
#10769=CARTESIAN_POINT('',(13.0014773719372,-21.9,47.9192193816532));
#10770=CARTESIAN_POINT('Origin',(17.3316043908594,-21.9,45.4192193816532));
#10771=CARTESIAN_POINT('Origin',(13.8675027757216,-21.9,47.4192193816532));
#10772=CARTESIAN_POINT('Origin',(17.3316043908594,-7.90000000000001,45.4192193816532));
#10773=CARTESIAN_POINT('',(13.0014773719372,-7.9,47.9192193816532));
#10774=CARTESIAN_POINT('',(19.1957890247756,-4.56844441699029,48.6480818822852));
#10775=CARTESIAN_POINT('Origin',(17.3316043908594,-7.90000000000001,45.4192193816532));
#10776=CARTESIAN_POINT('',(11.9501151712092,11.6489333498058,36.0982066328347));
#10777=CARTESIAN_POINT('',(19.1957890247756,-4.56844441699029,48.6480818822853));
#10778=CARTESIAN_POINT('',(10.1102324883161,11.3230083161312,36.8657033664312));
#10779=CARTESIAN_POINT('Origin',(10.384104613565,7.6499999999371,33.3857967817714));
#10780=CARTESIAN_POINT('',(6.05397759465256,7.65,35.8857967818225));
#10781=CARTESIAN_POINT('Ctrl Pts',(6.05397759465256,7.65,35.8857967818225));
#10782=CARTESIAN_POINT('Ctrl Pts',(6.08928976743534,7.74017246065655,35.9469592592079));
#10783=CARTESIAN_POINT('Ctrl Pts',(6.12832838012931,7.83131579263958,36.006848308931));
#10784=CARTESIAN_POINT('Ctrl Pts',(6.17111895326201,7.92309626160611,36.0651473231755));
#10785=CARTESIAN_POINT('Ctrl Pts',(6.21435423570126,8.01583057684584,36.1240522211999));
#10786=CARTESIAN_POINT('Ctrl Pts',(6.26141987741726,8.10921506410549,36.1813336075092));
#10787=CARTESIAN_POINT('Ctrl Pts',(6.3122944546444,8.2028829922255,36.2366721483555));
#10788=CARTESIAN_POINT('Ctrl Pts',(6.36402406580603,8.29812516943968,36.2929407476491));
#10789=CARTESIAN_POINT('Ctrl Pts',(6.41969173269722,8.39366006533703,36.3472003412477));
#10790=CARTESIAN_POINT('Ctrl Pts',(6.47922558198133,8.48908360809998,36.3991269669764));
#10791=CARTESIAN_POINT('Ctrl Pts',(6.53926650009729,8.5853199036908,36.4514958683812));
#10792=CARTESIAN_POINT('Ctrl Pts',(6.60323963772497,8.68144252076869,36.5014915701947));
#10793=CARTESIAN_POINT('Ctrl Pts',(6.67102226579008,8.77702401761752,36.5487983543273));
#10794=CARTESIAN_POINT('Ctrl Pts',(6.73940230767439,8.87344793838393,36.5965220849163));
#10795=CARTESIAN_POINT('Ctrl Pts',(6.81165913893223,8.96932067908334,36.6415089425318));
#10796=CARTESIAN_POINT('Ctrl Pts',(6.88761899106763,9.06419708738261,36.6834566789221));
#10797=CARTESIAN_POINT('Ctrl Pts',(6.91875332268202,9.1030849139822,36.7006501659884));
#10798=CARTESIAN_POINT('Ctrl Pts',(6.95050922415029,9.14180532432651,36.7173333620187));
#10799=CARTESIAN_POINT('Ctrl Pts',(6.98287254062646,9.18032765868938,36.7334867131329));
#10800=CARTESIAN_POINT('Ctrl Pts',(7.06065466533108,9.27291239170125,36.7723097420302));
#10801=CARTESIAN_POINT('Ctrl Pts',(7.14193522550449,9.36433490372364,36.8080617552191));
#10802=CARTESIAN_POINT('Ctrl Pts',(7.22639353034653,9.45421392953755,36.8405831329111));
#10803=CARTESIAN_POINT('Ctrl Pts',(7.31498815818374,9.54849475671312,36.8746972364177));
#10804=CARTESIAN_POINT('Ctrl Pts',(7.40707923745252,9.64107659815097,36.9052560617205));
#10805=CARTESIAN_POINT('Ctrl Pts',(7.5022523237989,9.73153397866236,36.9321141600708));
#10806=CARTESIAN_POINT('Ctrl Pts',(7.59398106932454,9.81871768107638,36.9580002562715));
#10807=CARTESIAN_POINT('Ctrl Pts',(7.68857206543916,9.90392756518674,36.9804487410977));
#10808=CARTESIAN_POINT('Ctrl Pts',(7.78562171747329,9.98680273224879,36.9993663118177));
#10809=CARTESIAN_POINT('Ctrl Pts',(7.88226230101848,10.0693285768903,37.0182041441574));
#10810=CARTESIAN_POINT('Ctrl Pts',(7.98134035104027,10.1495389355592,37.0335406880032));
#10811=CARTESIAN_POINT('Ctrl Pts',(8.08243321548938,10.2271033948173,37.0453212245668));
#10812=CARTESIAN_POINT('Ctrl Pts',(8.18238435349759,10.3037918536328,37.0569687136581));
#10813=CARTESIAN_POINT('Ctrl Pts',(8.28430455192637,10.37789350802,37.0651400528604));
#10814=CARTESIAN_POINT('Ctrl Pts',(8.3877691935037,10.4491198811129,37.0698195899984));
#10815=CARTESIAN_POINT('Ctrl Pts',(8.40167504206957,10.4586928438471,37.0704485288688));
#10816=CARTESIAN_POINT('Ctrl Pts',(8.41560877166897,10.4682139182184,37.071014447974));
#10817=CARTESIAN_POINT('Ctrl Pts',(8.429569336418,10.4776824519197,37.0715173614424));
#10818=CARTESIAN_POINT('Ctrl Pts',(8.53515074276735,10.549291381947,37.0753208115335));
#10819=CARTESIAN_POINT('Ctrl Pts',(8.64225116327287,10.6178811928978,37.0755170775839));
#10820=CARTESIAN_POINT('Ctrl Pts',(8.75036064416503,10.683271528406,37.072237567608));
#10821=CARTESIAN_POINT('Ctrl Pts',(8.86231822477556,10.7509893982765,37.0688413252113));
#10822=CARTESIAN_POINT('Ctrl Pts',(8.97535731700236,10.815275468209,37.0617173928374));
#10823=CARTESIAN_POINT('Ctrl Pts',(9.08891450935123,10.8759743328058,37.0510506189197));
#10824=CARTESIAN_POINT('Ctrl Pts',(9.19619874745181,10.933320162754,37.0409730827542));
#10825=CARTESIAN_POINT('Ctrl Pts',(9.30394500151563,10.9874643718571,37.0277337487462));
#10826=CARTESIAN_POINT('Ctrl Pts',(9.41168854166736,11.0383162475296,37.0115189784436));
#10827=CARTESIAN_POINT('Ctrl Pts',(9.51841693092522,11.0886890009553,36.9954569823913));
#10828=CARTESIAN_POINT('Ctrl Pts',(9.62514225220611,11.1358311057241,36.9764755314245));
#10829=CARTESIAN_POINT('Ctrl Pts',(9.73142938425917,11.1796944882328,36.9547824460045));
#10830=CARTESIAN_POINT('Ctrl Pts',(9.83642685367666,11.2230256429507,36.9333525792938));
#10831=CARTESIAN_POINT('Ctrl Pts',(9.94099637984397,11.2631571549113,36.9092766665018));
#10832=CARTESIAN_POINT('Ctrl Pts',(10.0447401308685,11.3000824629291,36.8827785309424));
#10833=CARTESIAN_POINT('Ctrl Pts',(10.0666087164109,11.3078661053085,36.877192876496));
#10834=CARTESIAN_POINT('Ctrl Pts',(10.0884406962602,11.3155074248239,36.8714996709178));
#10835=CARTESIAN_POINT('Ctrl Pts',(10.1102324887055,11.3230065889554,36.8657011341632));
#10836=CARTESIAN_POINT('',(5.75580351837084,8.31737776679611,35.3693441322026));
#10837=CARTESIAN_POINT('Origin',(17.3316043908594,-22.9,45.4192193816532));
#10838=CARTESIAN_POINT('',(19.8316043908594,-7.90000000000001,49.7493464005754));
#10839=CARTESIAN_POINT('',(19.8316043908594,-22.9,49.7493464005754));
#10840=CARTESIAN_POINT('Origin',(17.3316043908594,-7.90000000000001,45.4192193816532));
#10841=CARTESIAN_POINT('',(13.0014773719372,-7.90000000000001,47.9192193816532));
#10842=CARTESIAN_POINT('Origin',(17.33160439086,-7.90000000000001,-45.419219381653));
#10843=CARTESIAN_POINT('',(13.0014773719379,-7.90000000000001,-47.919219381653));
#10844=CARTESIAN_POINT('',(19.8316043908601,-7.90000000000001,-49.7493464005752));
#10845=CARTESIAN_POINT('Origin',(17.33160439086,-7.90000000000001,-45.419219381653));
#10846=CARTESIAN_POINT('',(19.8316043908601,-21.9,-49.7493464005752));
#10847=CARTESIAN_POINT('',(19.8316043908601,-22.9,-49.7493464005752));
#10848=CARTESIAN_POINT('',(13.0014773719379,-21.9,-47.919219381653));
#10849=CARTESIAN_POINT('Origin',(17.33160439086,-21.9,-45.419219381653));
#10850=CARTESIAN_POINT('',(13.0014773719379,-7.90000000000001,-47.919219381653));
#10851=CARTESIAN_POINT('Origin',(17.33160439086,-7.90000000000001,-45.419219381653));
#10852=CARTESIAN_POINT('',(6.05397759465306,7.65,-35.8857967818224));
#10853=CARTESIAN_POINT('',(10.1102324887059,11.3230065889554,-36.865701134163));
#10854=CARTESIAN_POINT('Ctrl Pts',(6.05397759465306,7.65,-35.8857967818224));
#10855=CARTESIAN_POINT('Ctrl Pts',(6.08928976743518,7.74017246065474,-35.9469592592067));
#10856=CARTESIAN_POINT('Ctrl Pts',(6.12832838012837,7.83131579263597,-36.0068483089287));
#10857=CARTESIAN_POINT('Ctrl Pts',(6.17111895326016,7.92309626160072,-36.0651473231721));
#10858=CARTESIAN_POINT('Ctrl Pts',(6.21435423569857,8.01583057683878,-36.1240522211956));
#10859=CARTESIAN_POINT('Ctrl Pts',(6.26141987741361,8.10921506409678,-36.1813336075041));
#10860=CARTESIAN_POINT('Ctrl Pts',(6.31229445463966,8.20288299221516,-36.2366721483496));
#10861=CARTESIAN_POINT('Ctrl Pts',(6.36402406580065,8.29812516942855,-36.292940747643));
#10862=CARTESIAN_POINT('Ctrl Pts',(6.41969173269114,8.39366006532512,-36.3472003412414));
#10863=CARTESIAN_POINT('Ctrl Pts',(6.47922558197449,8.48908360808729,-36.3991269669699));
#10864=CARTESIAN_POINT('Ctrl Pts',(6.53926650008992,8.58531990367772,-36.4514958683748));
#10865=CARTESIAN_POINT('Ctrl Pts',(6.60323963771704,8.68144252075522,-36.5014915701884));
#10866=CARTESIAN_POINT('Ctrl Pts',(6.67102226578152,8.77702401760362,-36.5487983543211));
#10867=CARTESIAN_POINT('Ctrl Pts',(6.73940230766558,8.87344793837014,-36.5965220849105));
#10868=CARTESIAN_POINT('Ctrl Pts',(6.81165913892316,8.96932067906961,-36.6415089425263));
#10869=CARTESIAN_POINT('Ctrl Pts',(6.88761899105827,9.06419708736885,-36.6834566789171));
#10870=CARTESIAN_POINT('Ctrl Pts',(6.91875332267609,9.10308491397287,-36.7006501659855));
#10871=CARTESIAN_POINT('Ctrl Pts',(6.95050922414792,9.14180532432155,-36.7173333620177));
#10872=CARTESIAN_POINT('Ctrl Pts',(6.9828725406278,9.18032765868873,-36.7334867131338));
#10873=CARTESIAN_POINT('Ctrl Pts',(7.0606546653326,9.2729123917006,-36.7723097420312));
#10874=CARTESIAN_POINT('Ctrl Pts',(7.14193522550624,9.36433490372311,-36.8080617552203));
#10875=CARTESIAN_POINT('Ctrl Pts',(7.22639353034854,9.45421392953721,-36.8405831329123));
#10876=CARTESIAN_POINT('Ctrl Pts',(7.31498815818571,9.54849475671266,-36.8746972364189));
#10877=CARTESIAN_POINT('Ctrl Pts',(7.40707923745448,9.6410765981505,-36.9052560617216));
#10878=CARTESIAN_POINT('Ctrl Pts',(7.50225232380081,9.73153397866191,-36.9321141600718));
#10879=CARTESIAN_POINT('Ctrl Pts',(7.59398106932713,9.81871768107662,-36.9580002562726));
#10880=CARTESIAN_POINT('Ctrl Pts',(7.68857206544245,9.90392756518769,-36.9804487410988));
#10881=CARTESIAN_POINT('Ctrl Pts',(7.78562171747729,9.9868027322504,-36.9993663118188));
#10882=CARTESIAN_POINT('Ctrl Pts',(7.8822623010229,10.0693285768923,-37.0182041441584));
#10883=CARTESIAN_POINT('Ctrl Pts',(7.9813403510451,10.1495389355616,-37.0335406880041));
#10884=CARTESIAN_POINT('Ctrl Pts',(8.08243321549461,10.22710339482,-37.0453212245677));
#10885=CARTESIAN_POINT('Ctrl Pts',(8.18238435350325,10.3037918536358,-37.0569687136589));
#10886=CARTESIAN_POINT('Ctrl Pts',(8.28430455193243,10.3778935080232,-37.0651400528611));
#10887=CARTESIAN_POINT('Ctrl Pts',(8.38776919351014,10.4491198811163,-37.069819589999));
#10888=CARTESIAN_POINT('Ctrl Pts',(8.40167504207419,10.4586928438492,-37.0704485288693));
#10889=CARTESIAN_POINT('Ctrl Pts',(8.41560877167175,10.4682139182192,-37.0710144479744));
#10890=CARTESIAN_POINT('Ctrl Pts',(8.42956933641895,10.4776824519193,-37.0715173614427));
#10891=CARTESIAN_POINT('Ctrl Pts',(8.53515074276891,10.5492913819469,-37.0753208115339));
#10892=CARTESIAN_POINT('Ctrl Pts',(8.64225116327509,10.6178811928981,-37.0755170775842));
#10893=CARTESIAN_POINT('Ctrl Pts',(8.75036064416794,10.6832715284068,-37.0722375676082));
#10894=CARTESIAN_POINT('Ctrl Pts',(8.86231822477821,10.750989398277,-37.0688413252115));
#10895=CARTESIAN_POINT('Ctrl Pts',(8.97535731700476,10.8152754682094,-37.0617173928375));
#10896=CARTESIAN_POINT('Ctrl Pts',(9.08891450935341,10.8759743328061,-37.0510506189198));
#10897=CARTESIAN_POINT('Ctrl Pts',(9.19619874745444,10.9333201627546,-37.0409730827541));
#10898=CARTESIAN_POINT('Ctrl Pts',(9.30394500151872,10.987464371858,-37.027733748746));
#10899=CARTESIAN_POINT('Ctrl Pts',(9.41168854167092,11.0383162475307,-37.0115189784432));
#10900=CARTESIAN_POINT('Ctrl Pts',(9.51841693092913,11.0886890009566,-36.9954569823907));
#10901=CARTESIAN_POINT('Ctrl Pts',(9.62514225221039,11.1358311057255,-36.9764755314237));
#10902=CARTESIAN_POINT('Ctrl Pts',(9.73142938426382,11.1796944882344,-36.9547824460035));
#10903=CARTESIAN_POINT('Ctrl Pts',(9.83642685368137,11.2230256429523,-36.9333525792928));
#10904=CARTESIAN_POINT('Ctrl Pts',(9.94099637984871,11.2631571549129,-36.9092766665007));
#10905=CARTESIAN_POINT('Ctrl Pts',(10.0447401308733,11.3000824629307,-36.8827785309411));
#10906=CARTESIAN_POINT('Ctrl Pts',(10.0666087164143,11.3078661053095,-36.8771928764951));
#10907=CARTESIAN_POINT('Ctrl Pts',(10.0884406962621,11.3155074248244,-36.8714996709173));
#10908=CARTESIAN_POINT('Ctrl Pts',(10.1102324887059,11.3230065889554,-36.865701134163));
#10909=CARTESIAN_POINT('',(11.9501151712097,11.6489333498058,-36.0982066328345));
#10910=CARTESIAN_POINT('Origin',(10.3841046135622,7.6499999999151,-33.3857967817529));
#10911=CARTESIAN_POINT('',(19.1957890247762,-4.56844441699029,-48.648081882285));
#10912=CARTESIAN_POINT('',(19.1957890247762,-4.56844441699029,-48.648081882285));
#10913=CARTESIAN_POINT('Origin',(17.33160439086,-7.90000000000001,-45.419219381653));
#10914=CARTESIAN_POINT('',(13.0014773719379,-7.90000000000001,-47.919219381653));
#10915=CARTESIAN_POINT('Origin',(0.,24.9,0.));
#10916=CARTESIAN_POINT('',(-1.08087326492746E-15,25.4,-8.82600000000003));
#10917=CARTESIAN_POINT('',(-1.01964092497009E-15,24.9,-8.326));
#10918=CARTESIAN_POINT('Origin',(0.,25.4,0.));
#10919=CARTESIAN_POINT('Origin',(0.,13.15,0.));
#10920=CARTESIAN_POINT('',(1.82293408768471,12.6595351585866,-19.3672161093864));
#10921=CARTESIAN_POINT('',(-7.41942469371926E-7,12.7590298799455,-19.2383203234121));
#10922=CARTESIAN_POINT('Ctrl Pts',(1.82293408768471,12.6595351585866,-19.3672161093864));
#10923=CARTESIAN_POINT('Ctrl Pts',(1.78888997792411,12.6607896844181,-19.3640610554799));
#10924=CARTESIAN_POINT('Ctrl Pts',(1.75461498816483,12.6621343910058,-19.361044358231));
#10925=CARTESIAN_POINT('Ctrl Pts',(1.72025845212816,12.6635474656982,-19.358140139342));
#10926=CARTESIAN_POINT('Ctrl Pts',(1.68456107776077,12.6650156886952,-19.3551225770122));
#10927=CARTESIAN_POINT('Ctrl Pts',(1.6487753668818,12.6665577514038,-19.3522264959792));
#10928=CARTESIAN_POINT('Ctrl Pts',(1.61301220996673,12.6681551150688,-19.3494277462689));
#10929=CARTESIAN_POINT('Ctrl Pts',(1.57497663282431,12.669853976527,-19.3464511617138));
#10930=CARTESIAN_POINT('Ctrl Pts',(1.53696644084721,12.6716154025952,-19.3435847123621));
#10931=CARTESIAN_POINT('Ctrl Pts',(1.49905533094398,12.6734233512426,-19.3408040316618));
#10932=CARTESIAN_POINT('Ctrl Pts',(1.45973281213481,12.6752986087826,-19.3379198278117));
#10933=CARTESIAN_POINT('Ctrl Pts',(1.42051649491172,12.6772239582494,-19.3351279625462));
#10934=CARTESIAN_POINT('Ctrl Pts',(1.38143082867857,12.6791875669107,-19.3324052587621));
#10935=CARTESIAN_POINT('Ctrl Pts',(1.34004990580164,12.6812664860236,-19.3295226676189));
#10936=CARTESIAN_POINT('Ctrl Pts',(1.29881519384669,12.683388313637,-19.3267176591772));
#10937=CARTESIAN_POINT('Ctrl Pts',(1.25769687566335,12.6855451971966,-19.3239661713634));
#10938=CARTESIAN_POINT('Ctrl Pts',(1.23647135280047,12.6866585934474,-19.3225458368245));
#10939=CARTESIAN_POINT('Ctrl Pts',(1.2152759371352,12.6877814266293,-19.3211398124163));
#10940=CARTESIAN_POINT('Ctrl Pts',(1.19410123994597,12.6889131739459,-19.3197450375488));
#10941=CARTESIAN_POINT('Ctrl Pts',(1.14719948359475,12.6914199836738,-19.3166556242542));
#10942=CARTESIAN_POINT('Ctrl Pts',(1.10043265364891,12.6939663244445,-19.3136179280417));
#10943=CARTESIAN_POINT('Ctrl Pts',(1.05358207653531,12.6965557025242,-19.3105915433049));
#10944=CARTESIAN_POINT('Ctrl Pts',(1.02728833978127,12.6980089274316,-19.3088930591348));
#10945=CARTESIAN_POINT('Ctrl Pts',(1.00096726291399,12.699475822638,-19.3071982112495));
#10946=CARTESIAN_POINT('Ctrl Pts',(0.974573185146914,12.7009578120448,-19.3055001747126));
#10947=CARTESIAN_POINT('Ctrl Pts',(0.956266388874189,12.7019857122574,-19.3043224253243));
#10948=CARTESIAN_POINT('Ctrl Pts',(0.937924370736718,12.7030208856048,-19.30314314581));
#10949=CARTESIAN_POINT('Ctrl Pts',(0.91953055081917,12.7040639541404,-19.30196006824));
#10950=CARTESIAN_POINT('Ctrl Pts',(0.910862311987517,12.7045555087618,-19.3014025332104));
#10951=CARTESIAN_POINT('Ctrl Pts',(0.902182660540566,12.7050488136889,-19.3008441612167));
#10952=CARTESIAN_POINT('Ctrl Pts',(0.893505909217807,12.705543019972,-19.3002857525201));
#10953=CARTESIAN_POINT('Ctrl Pts',(0.822076183406764,12.7096114803876,-19.2956887577922));
#10954=CARTESIAN_POINT('Ctrl Pts',(0.750602616626036,12.7137542634669,-19.2910724211421));
#10955=CARTESIAN_POINT('Ctrl Pts',(0.679155770279492,12.717948730176,-19.2863841545952));
#10956=CARTESIAN_POINT('Ctrl Pts',(0.605333316726877,12.7222826628776,-19.2815400032141));
#10957=CARTESIAN_POINT('Ctrl Pts',(0.53153928875299,12.7266718216052,-19.2766193209322));
#10958=CARTESIAN_POINT('Ctrl Pts',(0.457798195777434,12.7310987618933,-19.2715763930781));
#10959=CARTESIAN_POINT('Ctrl Pts',(0.444313844229887,12.7319082755134,-19.2706542395099));
#10960=CARTESIAN_POINT('Ctrl Pts',(0.430831125913135,12.7327190709993,-19.2697280242799));
#10961=CARTESIAN_POINT('Ctrl Pts',(0.417350010399558,12.733531065795,-19.268797499997));
#10962=CARTESIAN_POINT('Ctrl Pts',(0.343529011221796,12.7379774535652,-19.2637020587293));
#10963=CARTESIAN_POINT('Ctrl Pts',(0.26971644232983,12.7424626536921,-19.2584731521507));
#10964=CARTESIAN_POINT('Ctrl Pts',(0.195920274301196,12.7469772849337,-19.2530745663503));
#10965=CARTESIAN_POINT('Ctrl Pts',(0.13061107197285,12.7509727087215,-19.2482968476456));
#10966=CARTESIAN_POINT('Ctrl Pts',(0.0653136611866498,12.7549912939957,
-19.2433864290818));
#10967=CARTESIAN_POINT('Ctrl Pts',(-1.16478701239764E-7,12.7590298412712,
-19.2383203719261));
#10968=CARTESIAN_POINT('',(-6.07314264709754,13.15,-18.0560083736136));
#10969=CARTESIAN_POINT('Ctrl Pts',(-1.36740623685183E-6,12.7590299186198,
-19.238320274898));
#10970=CARTESIAN_POINT('Ctrl Pts',(-0.0976846971834283,12.7650699730032,
-19.2307434734679));
#10971=CARTESIAN_POINT('Ctrl Pts',(-0.195826602486313,12.7711799956073,
-19.2227859628905));
#10972=CARTESIAN_POINT('Ctrl Pts',(-0.294252134116968,12.7773367444421,
-19.2143959580921));
#10973=CARTESIAN_POINT('Ctrl Pts',(-0.359553588796595,12.7814215042431,
-19.2088295211217));
#10974=CARTESIAN_POINT('Ctrl Pts',(-0.424981033355307,12.7855269574494,
-19.2030729859267));
#10975=CARTESIAN_POINT('Ctrl Pts',(-0.490495587159556,12.7896476277827,
-19.1971137495186));
#10976=CARTESIAN_POINT('Ctrl Pts',(-0.602712929565564,12.7967057644391,
-19.1869064042244));
#10977=CARTESIAN_POINT('Ctrl Pts',(-0.714605986300817,12.8037719382783,
-19.1761531494054));
#10978=CARTESIAN_POINT('Ctrl Pts',(-0.82612323045651,12.8108347372977,-19.1648175733631));
#10979=CARTESIAN_POINT('Ctrl Pts',(-0.943193195446338,12.8182492106394,
-19.1529175708078));
#10980=CARTESIAN_POINT('Ctrl Pts',(-1.0598491202423,12.8256599893232,-19.1403761143674));
#10981=CARTESIAN_POINT('Ctrl Pts',(-1.17609035809504,12.8330594679584,-19.1271552243471));
#10982=CARTESIAN_POINT('Ctrl Pts',(-1.2847832692999,12.8399784485982,-19.11479285578));
#10983=CARTESIAN_POINT('Ctrl Pts',(-1.39311451381811,12.8468876427769,-19.1018366670684));
#10984=CARTESIAN_POINT('Ctrl Pts',(-1.50112450746874,12.8537845810569,-19.08825515445));
#10985=CARTESIAN_POINT('Ctrl Pts',(-1.62066135458927,12.8614175623108,-19.0732242194165));
#10986=CARTESIAN_POINT('Ctrl Pts',(-1.73981679586176,12.869034758093,-19.0574096075086));
#10987=CARTESIAN_POINT('Ctrl Pts',(-1.85866951308033,12.8766408833612,-19.0407937879716));
#10988=CARTESIAN_POINT('Ctrl Pts',(-1.9837153295282,12.884643343603,-19.023312162237));
#10989=CARTESIAN_POINT('Ctrl Pts',(-2.10842629293182,12.8926335674546,-19.0049439848625));
#10990=CARTESIAN_POINT('Ctrl Pts',(-2.23294928564757,12.9006206698086,-18.9856519958004));
#10991=CARTESIAN_POINT('Ctrl Pts',(-2.36105802888851,12.9088377678914,-18.9658044767241));
#10992=CARTESIAN_POINT('Ctrl Pts',(-2.48896829721021,12.9170515954563,-18.9449794918307));
#10993=CARTESIAN_POINT('Ctrl Pts',(-2.61689111717973,12.9252753964184,-18.9231141413901));
#10994=CARTESIAN_POINT('Ctrl Pts',(-2.74926523716585,12.9337853590314,-18.9004879475377));
#10995=CARTESIAN_POINT('Ctrl Pts',(-2.8816532683033,12.9423060343459,-18.8767481373003));
#10996=CARTESIAN_POINT('Ctrl Pts',(-3.01433566154705,12.9508550880408,-18.8517957698283));
#10997=CARTESIAN_POINT('Ctrl Pts',(-3.03374933409837,12.9521059588233,-18.8481448175079));
#10998=CARTESIAN_POINT('Ctrl Pts',(-3.05316937993749,12.953357441682,-18.8444678500867));
#10999=CARTESIAN_POINT('Ctrl Pts',(-3.07259674806375,12.9546095964169,-18.8407644990186));
#11000=CARTESIAN_POINT('Ctrl Pts',(-3.23684149935945,12.9651956851594,-18.8094552670537));
#11001=CARTESIAN_POINT('Ctrl Pts',(-3.40082753073851,12.9757755153363,-18.7764116206451));
#11002=CARTESIAN_POINT('Ctrl Pts',(-3.56454054604347,12.9863481136657,-18.7415646366649));
#11003=CARTESIAN_POINT('Ctrl Pts',(-3.6174038037455,12.9897620266586,-18.7303124763473));
#11004=CARTESIAN_POINT('Ctrl Pts',(-3.67023898229499,12.9931752118673,-18.7188721447255));
#11005=CARTESIAN_POINT('Ctrl Pts',(-3.72304664363111,12.9965877069929,-18.7072408831335));
#11006=CARTESIAN_POINT('Ctrl Pts',(-3.88049171455976,13.0067619984406,-18.6725624906427));
#11007=CARTESIAN_POINT('Ctrl Pts',(-4.0376742623794,13.0169318588212,-18.6361554750793));
#11008=CARTESIAN_POINT('Ctrl Pts',(-4.19448641334882,13.0270950616618,-18.5980827891145));
#11009=CARTESIAN_POINT('Ctrl Pts',(-4.36539686099497,13.0381719937508,-18.5565871539797));
#11010=CARTESIAN_POINT('Ctrl Pts',(-4.53586787392932,13.0492410451786,-18.5131132431364));
#11011=CARTESIAN_POINT('Ctrl Pts',(-4.70580770848692,13.060302140562,-18.4677001278632));
#11012=CARTESIAN_POINT('Ctrl Pts',(-4.88444462846006,13.071929314473,-18.4199628856803));
#11013=CARTESIAN_POINT('Ctrl Pts',(-5.06249585260001,13.0835477606057,-18.3700830167689));
#11014=CARTESIAN_POINT('Ctrl Pts',(-5.23989080423082,13.0951596114433,-18.3180572321707));
#11015=CARTESIAN_POINT('Ctrl Pts',(-5.42489221768705,13.1072693631474,-18.2638006504677));
#11016=CARTESIAN_POINT('Ctrl Pts',(-5.60918160043135,13.1193720281311,-18.2072102845129));
#11017=CARTESIAN_POINT('Ctrl Pts',(-5.79269367431625,13.1314711984988,-18.1482289026053));
#11018=CARTESIAN_POINT('Ctrl Pts',(-5.88638240479708,13.1376482084777,-18.118117037615));
#11019=CARTESIAN_POINT('Ctrl Pts',(-5.97986860207494,13.1438243177559,-18.0873811205117));
#11020=CARTESIAN_POINT('Ctrl Pts',(-6.07314264709754,13.15,-18.0560083736136));
#11021=CARTESIAN_POINT('',(18.6735332660427,13.15,-3.76850837361349));
#11022=CARTESIAN_POINT('Origin',(0.,13.15,0.));
#11023=CARTESIAN_POINT('',(15.8610341074696,12.6595351585866,-11.2623152840526));
#11024=CARTESIAN_POINT('Ctrl Pts',(18.6735332660427,13.15,-3.76850837361349));
#11025=CARTESIAN_POINT('Ctrl Pts',(18.635609003944,13.1379692270563,-3.95642887150844));
#11026=CARTESIAN_POINT('Ctrl Pts',(18.595290610597,13.1259554920877,-4.14350652629558));
#11027=CARTESIAN_POINT('Ctrl Pts',(18.5526294017364,13.1139455297031,-4.32990938943143));
#11028=CARTESIAN_POINT('Ctrl Pts',(18.5107522750365,13.10215630174,-4.51288630277349));
#11029=CARTESIAN_POINT('Ctrl Pts',(18.4666170044181,13.0903706662367,-4.69521392858484));
#11030=CARTESIAN_POINT('Ctrl Pts',(18.4202313065065,13.0785760987623,-4.87702411982452));
#11031=CARTESIAN_POINT('Ctrl Pts',(18.3751916837961,13.0671238000367,-5.0535583272856));
#11032=CARTESIAN_POINT('Ctrl Pts',(18.3280297551566,13.0556630399901,-5.22960544275274));
#11033=CARTESIAN_POINT('Ctrl Pts',(18.2787228864419,13.0441829769088,-5.4052483437446));
#11034=CARTESIAN_POINT('Ctrl Pts',(18.2319440507293,13.0332915129232,-5.57188578440453));
#11035=CARTESIAN_POINT('Ctrl Pts',(18.1832340569148,13.0223826439743,-5.73815981936693));
#11036=CARTESIAN_POINT('Ctrl Pts',(18.132554518669,13.0114481775998,-5.90409869240932));
#11037=CARTESIAN_POINT('Ctrl Pts',(18.1097293612668,13.0065234895551,-5.97883459228983));
#11038=CARTESIAN_POINT('Ctrl Pts',(18.0865044745234,13.0015936267203,-6.0535018781925));
#11039=CARTESIAN_POINT('Ctrl Pts',(18.0628754032633,12.9966579427863,-6.12809973553589));
#11040=CARTESIAN_POINT('Ctrl Pts',(18.0183561237835,12.9873586736755,-6.26864875767551));
#11041=CARTESIAN_POINT('Ctrl Pts',(17.972373035958,12.9780292666563,-6.40910769298485));
#11042=CARTESIAN_POINT('Ctrl Pts',(17.9250244537378,12.9686821009643,-6.54928034556807));
#11043=CARTESIAN_POINT('Ctrl Pts',(17.8807222934487,12.9599363347065,-6.68043424779068));
#11044=CARTESIAN_POINT('Ctrl Pts',(17.8352244399587,12.9511750020392,-6.81133765846827));
#11045=CARTESIAN_POINT('Ctrl Pts',(17.7886209010951,12.9424107435037,-6.94178628068565));
#11046=CARTESIAN_POINT('Ctrl Pts',(17.7539427147616,12.9358891660017,-7.03885448062299));
#11047=CARTESIAN_POINT('Ctrl Pts',(17.7186524670563,12.9293660137816,-7.13567005199129));
#11048=CARTESIAN_POINT('Ctrl Pts',(17.6827922878973,12.9228475964183,-7.23213062593721));
#11049=CARTESIAN_POINT('Ctrl Pts',(17.6352878328313,12.9142125624615,-7.35991322792396));
#11050=CARTESIAN_POINT('Ctrl Pts',(17.5867942563818,12.9055857664759,-7.48707423642674));
#11051=CARTESIAN_POINT('Ctrl Pts',(17.5373852100854,12.8969734463818,-7.61356929829063));
#11052=CARTESIAN_POINT('Ctrl Pts',(17.4919426291,12.8890525071474,-7.72990957449293));
#11053=CARTESIAN_POINT('Ctrl Pts',(17.4456790187502,12.8811371827701,-7.84580544759027));
#11054=CARTESIAN_POINT('Ctrl Pts',(17.3985927372716,12.8732239828729,-7.96135319383724));
#11055=CARTESIAN_POINT('Ctrl Pts',(17.3588829295431,12.8665504542662,-8.05879938501738));
#11056=CARTESIAN_POINT('Ctrl Pts',(17.3185880217668,12.8598784744127,-8.15599735052392));
#11057=CARTESIAN_POINT('Ctrl Pts',(17.2777163855609,12.8532079839213,-8.25297752920841));
#11058=CARTESIAN_POINT('Ctrl Pts',(17.2313167512056,12.845635291744,-8.36307453653147));
#11059=CARTESIAN_POINT('Ctrl Pts',(17.1841737380798,12.8380640091309,-8.47289269012394));
#11060=CARTESIAN_POINT('Ctrl Pts',(17.1363234461559,12.8305004633246,-8.5824610079591));
#11061=CARTESIAN_POINT('Ctrl Pts',(17.0906598957075,12.8232825688958,-8.68702209228785));
#11062=CARTESIAN_POINT('Ctrl Pts',(17.0443519564341,12.8160717028972,-8.7913556001471));
#11063=CARTESIAN_POINT('Ctrl Pts',(16.997455397443,12.8088775452789,-8.89544771685909));
#11064=CARTESIAN_POINT('Ctrl Pts',(16.9549407548744,12.8023555947072,-8.98981368381757));
#11065=CARTESIAN_POINT('Ctrl Pts',(16.9119423673544,12.7958473962748,-9.08398094533463));
#11066=CARTESIAN_POINT('Ctrl Pts',(16.8685236708355,12.7893635951273,-9.17790944158495));
#11067=CARTESIAN_POINT('Ctrl Pts',(16.831166098439,12.7837849138173,-9.25872579214598));
#11068=CARTESIAN_POINT('Ctrl Pts',(16.7934219290083,12.7782136874733,-9.33951840434077));
#11069=CARTESIAN_POINT('Ctrl Pts',(16.7554251187229,12.7726724740285,-9.42009967844722));
#11070=CARTESIAN_POINT('Ctrl Pts',(16.7500131624358,12.771883228702,-9.43157701903831));
#11071=CARTESIAN_POINT('Ctrl Pts',(16.7445961295867,12.7710945998699,-9.44305000107886));
#11072=CARTESIAN_POINT('Ctrl Pts',(16.7391744571789,12.7703066605067,-9.45451800992888));
#11073=CARTESIAN_POINT('Ctrl Pts',(16.7095471419653,12.7660008806425,-9.51718618452878));
#11074=CARTESIAN_POINT('Ctrl Pts',(16.6797728051853,12.7617151304109,-9.57972202319642));
#11075=CARTESIAN_POINT('Ctrl Pts',(16.6498373535122,12.757449305424,-9.64220564374232));
#11076=CARTESIAN_POINT('Ctrl Pts',(16.6211714013588,12.7533643850993,-9.70203946540951));
#11077=CARTESIAN_POINT('Ctrl Pts',(16.5923573963794,12.7492976981851,-9.76182568605953));
#11078=CARTESIAN_POINT('Ctrl Pts',(16.5634043886492,12.7452532521653,-9.82159229151741));
#11079=CARTESIAN_POINT('Ctrl Pts',(16.5359798968833,12.7414223245601,-9.87820363893009));
#11080=CARTESIAN_POINT('Ctrl Pts',(16.5084304766136,12.7376113278547,-9.93479754780587));
#11081=CARTESIAN_POINT('Ctrl Pts',(16.4807870976986,12.7338278436748,-9.9913559826116));
#11082=CARTESIAN_POINT('Ctrl Pts',(16.479246381964,12.7336169695401,-9.99450829154966));
#11083=CARTESIAN_POINT('Ctrl Pts',(16.4777053811798,12.7334061820622,-9.99766047853941));
#11084=CARTESIAN_POINT('Ctrl Pts',(16.4761641031983,12.7331954829858,-10.0008125362049));
#11085=CARTESIAN_POINT('Ctrl Pts',(16.4461689478205,12.7290950211555,-10.0621554351298));
#11086=CARTESIAN_POINT('Ctrl Pts',(16.4160888758792,12.725029433906,-10.1234195935806));
#11087=CARTESIAN_POINT('Ctrl Pts',(16.3859390142828,12.7210081247693,-10.1846516877651));
#11088=CARTESIAN_POINT('Ctrl Pts',(16.3574486213335,12.7172081511904,-10.2425135263293));
#11089=CARTESIAN_POINT('Ctrl Pts',(16.3288958340789,12.7134477064406,-10.3003465245089));
#11090=CARTESIAN_POINT('Ctrl Pts',(16.3003198960741,12.7097399996136,-10.358156854131));
#11091=CARTESIAN_POINT('Ctrl Pts',(16.2762833586279,12.7066212766527,-10.4067837846802));
#11092=CARTESIAN_POINT('Ctrl Pts',(16.2523127582846,12.7035507329856,-10.4552276437463));
#11093=CARTESIAN_POINT('Ctrl Pts',(16.2283644290953,12.7005283628054,-10.5036422639959));
#11094=CARTESIAN_POINT('Ctrl Pts',(16.2050726155633,12.6975888473968,-10.5507296536072));
#11095=CARTESIAN_POINT('Ctrl Pts',(16.1818016507761,12.6946948638812,-10.5977893480704));
#11096=CARTESIAN_POINT('Ctrl Pts',(16.1585395211624,12.6918520765314,-10.6449228641774));
#11097=CARTESIAN_POINT('Ctrl Pts',(16.1500867003578,12.690819085466,-10.6620498930506));
#11098=CARTESIAN_POINT('Ctrl Pts',(16.1416353373009,12.6897929124041,-10.6791862812815));
#11099=CARTESIAN_POINT('Ctrl Pts',(16.133185909691,12.6887740383049,-10.6963355459743));
#11100=CARTESIAN_POINT('Ctrl Pts',(16.1101815887034,12.68600006261,-10.7430259500949));
#11101=CARTESIAN_POINT('Ctrl Pts',(16.0871876783737,12.6832787578847,-10.7898158379825));
#11102=CARTESIAN_POINT('Ctrl Pts',(16.064233957608,12.6806283209993,-10.8367452553848));
#11103=CARTESIAN_POINT('Ctrl Pts',(16.0426664098205,12.6781379437413,-10.8808406098069));
#11104=CARTESIAN_POINT('Ctrl Pts',(16.0211342964406,12.675710111483,-10.9250589443984));
#11105=CARTESIAN_POINT('Ctrl Pts',(15.9996942678004,12.6733674903699,-10.9693973797136));
#11106=CARTESIAN_POINT('Ctrl Pts',(15.9787445551771,12.6710784430964,-11.0127218310757));
#11107=CARTESIAN_POINT('Ctrl Pts',(15.9578825024016,12.6688706813128,-11.0561609810969));
#11108=CARTESIAN_POINT('Ctrl Pts',(15.9371949671836,12.6667735640339,-11.0996774884489));
#11109=CARTESIAN_POINT('Ctrl Pts',(15.917184796503,12.6647451119131,-11.1417691504261));
#11110=CARTESIAN_POINT('Ctrl Pts',(15.8973376991438,12.6628201182914,-11.1839331484321));
#11111=CARTESIAN_POINT('Ctrl Pts',(15.8777677308615,12.6610338566175,-11.2261030546386));
#11112=CARTESIAN_POINT('Ctrl Pts',(15.8721658177008,12.6605225383244,-11.2381742112781));
#11113=CARTESIAN_POINT('Ctrl Pts',(15.8665868518027,12.6600226469234,-11.250245643483));
#11114=CARTESIAN_POINT('Ctrl Pts',(15.8610341074696,12.6595351585866,-11.2623152840526));
#11115=CARTESIAN_POINT('',(15.6532787469445,12.65,-11.7122740947458));
#11116=CARTESIAN_POINT('Ctrl Pts',(15.8610341074696,12.6595351585866,-11.2623152840526));
#11117=CARTESIAN_POINT('Ctrl Pts',(15.8165145702369,12.655626684734,-11.3590845188816));
#11118=CARTESIAN_POINT('Ctrl Pts',(15.7718505903917,12.6527974939087,-11.4558489811135));
#11119=CARTESIAN_POINT('Ctrl Pts',(15.7271279180831,12.6512766915384,-11.5525992725652));
#11120=CARTESIAN_POINT('Ctrl Pts',(15.7025232501934,12.6504400054614,-11.6058275048357));
#11121=CARTESIAN_POINT('Ctrl Pts',(15.6779011866278,12.65,-11.6590517667082));
#11122=CARTESIAN_POINT('Ctrl Pts',(15.6532787469445,12.65,-11.7122740947458));
#11123=CARTESIAN_POINT('',(2.31648752866421,12.65,-19.4122740947459));
#11124=CARTESIAN_POINT('Origin',(0.,12.65,0.));
#11125=CARTESIAN_POINT('Ctrl Pts',(2.31648752866421,12.65,-19.4122740947459));
#11126=CARTESIAN_POINT('Ctrl Pts',(2.2103311248206,12.65,-19.4026632604047));
#11127=CARTESIAN_POINT('Ctrl Pts',(2.10416883388078,12.6514513272156,-19.3930461613134));
#11128=CARTESIAN_POINT('Ctrl Pts',(1.99804499033973,12.6541030519185,-19.3833359160023));
#11129=CARTESIAN_POINT('Ctrl Pts',(1.93965979583085,12.6555619272985,-19.3779937182238));
#11130=CARTESIAN_POINT('Ctrl Pts',(1.881286570062,12.6573848689003,-19.3726239534149));
#11131=CARTESIAN_POINT('Ctrl Pts',(1.82293408768471,12.6595351585866,-19.3672161093864));
#11132=CARTESIAN_POINT('Origin',(0.,-23.4,0.));
#11133=CARTESIAN_POINT('',(-2.42665362134782,-22.9,19.3988105873015));
#11134=CARTESIAN_POINT('',(18.0131895824794,-22.9,7.59786161137834));
#11135=CARTESIAN_POINT('Origin',(4.90959474333048E-17,-22.9,8.50366754002165E-17));
#11136=CARTESIAN_POINT('',(-6.07314264709777,-23.4,18.0560083736135));
#11137=CARTESIAN_POINT('Ctrl Pts',(-2.42665362134782,-22.9,19.3988105873015));
#11138=CARTESIAN_POINT('Ctrl Pts',(-2.49483230883249,-22.9,19.3675892623714));
#11139=CARTESIAN_POINT('Ctrl Pts',(-2.56318139468448,-22.9014413252167,
19.3371168853022));
#11140=CARTESIAN_POINT('Ctrl Pts',(-2.63168706866709,-22.9040302787143,
19.3072597052728));
#11141=CARTESIAN_POINT('Ctrl Pts',(-2.70103054707964,-22.9066508943588,
19.2770373806321));
#11142=CARTESIAN_POINT('Ctrl Pts',(-2.77053455038377,-22.9104479219792,
19.2474455750134));
#11143=CARTESIAN_POINT('Ctrl Pts',(-2.8402082733943,-22.9151689742963,19.2183597505841));
#11144=CARTESIAN_POINT('Ctrl Pts',(-2.91389838884986,-22.9201621751085,
19.187597252648));
#11145=CARTESIAN_POINT('Ctrl Pts',(-2.98777825664906,-22.9261892251367,
19.1574008581504));
#11146=CARTESIAN_POINT('Ctrl Pts',(-3.06188524730074,-22.9330040852335,
19.1276368660924));
#11147=CARTESIAN_POINT('Ctrl Pts',(-3.12537434075582,-22.9388425261926,
19.1021373975976));
#11148=CARTESIAN_POINT('Ctrl Pts',(-3.1890306252501,-22.9452603057855,19.0769556044239));
#11149=CARTESIAN_POINT('Ctrl Pts',(-3.2528923076016,-22.9521283804573,19.0520136663235));
#11150=CARTESIAN_POINT('Ctrl Pts',(-3.27850056656131,-22.9548824487541,
19.0420120568089));
#11151=CARTESIAN_POINT('Ctrl Pts',(-3.30407836463786,-22.957705512208,19.0320737013011));
#11152=CARTESIAN_POINT('Ctrl Pts',(-3.32962845656234,-22.960593031896,19.0221941700939));
#11153=CARTESIAN_POINT('Ctrl Pts',(-3.43797011955961,-22.9728371633792,
18.9803013720646));
#11154=CARTESIAN_POINT('Ctrl Pts',(-3.54647772773345,-22.9863118482884,
18.9392088437263));
#11155=CARTESIAN_POINT('Ctrl Pts',(-3.65506054302364,-23.000712480614,18.8987487638366));
#11156=CARTESIAN_POINT('Ctrl Pts',(-3.77015005916127,-23.0159760543387,
18.855864159998));
#11157=CARTESIAN_POINT('Ctrl Pts',(-3.8853241639595,-23.0322800742794,18.8136901601118));
#11158=CARTESIAN_POINT('Ctrl Pts',(-4.00050877634662,-23.0493077902531,
18.772042864334));
#11159=CARTESIAN_POINT('Ctrl Pts',(-4.0530285423963,-23.0570717757436,18.7530532945857));
#11160=CARTESIAN_POINT('Ctrl Pts',(-4.10555093233817,-23.0649868063103,
18.734173429334));
#11161=CARTESIAN_POINT('Ctrl Pts',(-4.15807096335396,-23.0730255541293,
18.715386756417));
#11162=CARTESIAN_POINT('Ctrl Pts',(-4.18604852539236,-23.0773078167531,
18.705379045133));
#11163=CARTESIAN_POINT('Ctrl Pts',(-4.21404153215336,-23.0816279527546,
18.6953900829876));
#11164=CARTESIAN_POINT('Ctrl Pts',(-4.24204848892154,-23.0859836968891,
18.6854192437152));
#11165=CARTESIAN_POINT('Ctrl Pts',(-4.36416486299477,-23.104975681077,18.6419442332563));
#11166=CARTESIAN_POINT('Ctrl Pts',(-4.48640499350052,-23.1246111362377,
18.598870351077));
#11167=CARTESIAN_POINT('Ctrl Pts',(-4.60869052279136,-23.1447278442301,
18.556125457237));
#11168=CARTESIAN_POINT('Ctrl Pts',(-4.74760212112971,-23.1675796409777,
18.5075689227186));
#11169=CARTESIAN_POINT('Ctrl Pts',(-4.886572286895,-23.1910529746397,18.4594369686117));
#11170=CARTESIAN_POINT('Ctrl Pts',(-5.02554817388977,-23.2149438103717,
18.4116315716704));
#11171=CARTESIAN_POINT('Ctrl Pts',(-5.18078521662232,-23.2416300418297,
18.3582326072292));
#11172=CARTESIAN_POINT('Ctrl Pts',(-5.33603027633239,-23.2688383566178,
18.3052415157176));
#11173=CARTESIAN_POINT('Ctrl Pts',(-5.49127574609483,-23.2963096837761,
18.2525271420218));
#11174=CARTESIAN_POINT('Ctrl Pts',(-5.68520897685116,-23.3306269700528,
18.1866761460876));
#11175=CARTESIAN_POINT('Ctrl Pts',(-5.87914576531621,-23.3653575842081,
18.1212592702554));
#11176=CARTESIAN_POINT('Ctrl Pts',(-6.07314264709777,-23.4,18.0560083736135));
#11177=CARTESIAN_POINT('',(-2.33295215237571E-15,-23.4,19.05));
#11178=CARTESIAN_POINT('Origin',(0.,-23.4,0.));
#11179=CARTESIAN_POINT('',(18.6735332660427,-23.4,3.76850837361377));
#11180=CARTESIAN_POINT('Origin',(0.,-23.4,0.));
#11181=CARTESIAN_POINT('Ctrl Pts',(18.6735332660427,-23.4,3.76850837361377));
#11182=CARTESIAN_POINT('Ctrl Pts',(18.6350144631045,-23.3670436986399,3.95937491196879));
#11183=CARTESIAN_POINT('Ctrl Pts',(18.5966676676154,-23.3340202715025,4.15019613839664));
#11184=CARTESIAN_POINT('Ctrl Pts',(18.5586614537198,-23.3013555121996,4.34116274406092));
#11185=CARTESIAN_POINT('Ctrl Pts',(18.5277984165564,-23.2748300160513,4.49623763428238));
#11186=CARTESIAN_POINT('Ctrl Pts',(18.4971580439715,-23.2485394308233,4.65140928850101));
#11187=CARTESIAN_POINT('Ctrl Pts',(18.4668399407577,-23.2227118267817,4.80675183465115));
#11188=CARTESIAN_POINT('Ctrl Pts',(18.4388540307315,-23.1988709882634,4.95014479327899));
#11189=CARTESIAN_POINT('Ctrl Pts',(18.4111419439031,-23.1754236716161,5.09368400762515));
#11190=CARTESIAN_POINT('Ctrl Pts',(18.3838068036978,-23.1525653654293,5.23739146952049));
#11191=CARTESIAN_POINT('Ctrl Pts',(18.359835246298,-23.1325197686369,5.36341576080758));
#11192=CARTESIAN_POINT('Ctrl Pts',(18.3361535391227,-23.1129267586639,5.48956941598828));
#11193=CARTESIAN_POINT('Ctrl Pts',(18.3128553330328,-23.0939393205251,5.61583514399125));
#11194=CARTESIAN_POINT('Ctrl Pts',(18.309586231902,-23.0912750872682,5.63355219193056));
#11195=CARTESIAN_POINT('Ctrl Pts',(18.3063247250108,-23.0886228202051,5.6512713887974));
#11196=CARTESIAN_POINT('Ctrl Pts',(18.3030711156135,-23.0859829876023,5.66899262803536));
#11197=CARTESIAN_POINT('Ctrl Pts',(18.2977029311688,-23.0816274837341,5.69823119640761));
#11198=CARTESIAN_POINT('Ctrl Pts',(18.2923574142506,-23.0773075842935,5.72746674517875));
#11199=CARTESIAN_POINT('Ctrl Pts',(18.2870358543619,-23.0730255541509,5.75669829321656));
#11200=CARTESIAN_POINT('Ctrl Pts',(18.2649583928884,-23.055260771366,5.877970700012));
#11201=CARTESIAN_POINT('Ctrl Pts',(18.2432675843708,-23.0380976121135,5.9994818912581));
#11202=CARTESIAN_POINT('Ctrl Pts',(18.2221517586248,-23.0218415529585,6.12126924644107));
#11203=CARTESIAN_POINT('Ctrl Pts',(18.2022839003277,-23.0065462439498,6.23585884119596));
#11204=CARTESIAN_POINT('Ctrl Pts',(18.1829249568717,-22.9920537993276,6.35069295735908));
#11205=CARTESIAN_POINT('Ctrl Pts',(18.1642557197366,-22.9786542883935,6.46578579604177));
#11206=CARTESIAN_POINT('Ctrl Pts',(18.1555179094392,-22.9723828813846,6.51965298856382));
#11207=CARTESIAN_POINT('Ctrl Pts',(18.1469315449829,-22.9663514277283,6.57357660250184));
#11208=CARTESIAN_POINT('Ctrl Pts',(18.1385172401805,-22.960592775276,6.62755666242319));
#11209=CARTESIAN_POINT('Ctrl Pts',(18.1342982464804,-22.9577053450025,6.65462265754528));
#11210=CARTESIAN_POINT('Ctrl Pts',(18.1301163408571,-22.9548823672323,6.68174205639669));
#11211=CARTESIAN_POINT('Ctrl Pts',(18.1259739819792,-22.9521283805007,6.70891945903846));
#11212=CARTESIAN_POINT('Ctrl Pts',(18.113919279733,-22.9441139879726,6.78800857379809));
#11213=CARTESIAN_POINT('Ctrl Pts',(18.1022868108286,-22.9367118504463,6.86701914290839));
#11214=CARTESIAN_POINT('Ctrl Pts',(18.0911547751198,-22.9301299080703,6.94606439194116));
#11215=CARTESIAN_POINT('Ctrl Pts',(18.0804160048456,-22.923780488343,7.02231718099403));
#11216=CARTESIAN_POINT('Ctrl Pts',(18.0701428237499,-22.9181939831416,7.09860216030664));
#11217=CARTESIAN_POINT('Ctrl Pts',(18.0604250099349,-22.9135965970109,7.17500646404394));
#11218=CARTESIAN_POINT('Ctrl Pts',(18.0512249388187,-22.9092441490059,7.24734012276077));
#11219=CARTESIAN_POINT('Ctrl Pts',(18.0425226047623,-22.9057780702216,7.31978062515643));
#11220=CARTESIAN_POINT('Ctrl Pts',(18.0344129323305,-22.9034297890292,7.39239005519619));
#11221=CARTESIAN_POINT('Ctrl Pts',(18.0267815700159,-22.9012200099356,7.46071696639418));
#11222=CARTESIAN_POINT('Ctrl Pts',(18.0196750266457,-22.9,7.52919337317792));
#11223=CARTESIAN_POINT('Ctrl Pts',(18.0131895824794,-22.9,7.59786161137834));
#11224=CARTESIAN_POINT('Origin',(0.,-23.4,0.));
#11225=CARTESIAN_POINT('',(-15.5865359611318,-22.9,-11.8009489759233));
#11226=CARTESIAN_POINT('',(-15.5865359611318,-22.9,11.8009489759233));
#11227=CARTESIAN_POINT('Origin',(-9.81918948666111E-17,-22.9,0.));
#11228=CARTESIAN_POINT('',(-12.6003906189451,-23.4,-14.2875));
#11229=CARTESIAN_POINT('Ctrl Pts',(-15.5865359611318,-22.9,-11.8009489759233));
#11230=CARTESIAN_POINT('Ctrl Pts',(-15.5254081568604,-22.9,-11.8443827888175));
#11231=CARTESIAN_POINT('Ctrl Pts',(-15.4648437612788,-22.9014413252167,
-11.8883386449565));
#11232=CARTESIAN_POINT('Ctrl Pts',(-15.4047338478967,-22.9040302787143,
-11.9327377089142));
#11233=CARTESIAN_POINT('Ctrl Pts',(-15.3438888077885,-22.9066508943588,
-11.9776797604873));
#11234=CARTESIAN_POINT('Ctrl Pts',(-15.2835095507252,-22.9104479219794,
-12.0230760902052));
#11235=CARTESIAN_POINT('Ctrl Pts',(-15.2234836263725,-22.9151689742967,
-12.068872392095));
#11236=CARTESIAN_POINT('Ctrl Pts',(-15.1599974639465,-22.920162175109,-12.1173086551203));
#11237=CARTESIAN_POINT('Ctrl Pts',(-15.0969066853077,-22.9261892251374,
-12.1661923002148));
#11238=CARTESIAN_POINT('Ctrl Pts',(-15.03407681674,-22.9330040852346,-12.2154888406893));
#11239=CARTESIAN_POINT('Ctrl Pts',(-14.9802490825162,-22.9388425261934,
-12.2577222742345));
#11240=CARTESIAN_POINT('Ctrl Pts',(-14.9266128676709,-22.9452603057859,
-12.3002593371276));
#11241=CARTESIAN_POINT('Ctrl Pts',(-14.8730816744838,-22.9521283804573,
-12.3430942073196));
#11242=CARTESIAN_POINT('Ctrl Pts',(-14.8516158970855,-22.9548824487541,
-12.3602708053681));
#11243=CARTESIAN_POINT('Ctrl Pts',(-14.8302201297056,-22.957705512208,-12.3774526505213));
#11244=CARTESIAN_POINT('Ctrl Pts',(-14.8088891587405,-22.960593031896,-12.3946399135934));
#11245=CARTESIAN_POINT('Ctrl Pts',(-14.7184380998966,-22.9728371633814,
-12.4675201470358));
#11246=CARTESIAN_POINT('Ctrl Pts',(-14.6285971223469,-22.9863118482931,
-12.5409442280624));
#11247=CARTESIAN_POINT('Ctrl Pts',(-14.5392662576623,-23.0007124806216,
-12.6147496645868));
#11248=CARTESIAN_POINT('Ctrl Pts',(-14.4445823432294,-23.015976054348,-12.6929778073595));
#11249=CARTESIAN_POINT('Ctrl Pts',(-14.350471535541,-23.0322800742906,-12.7716345080375));
#11250=CARTESIAN_POINT('Ctrl Pts',(-14.2568116131964,-23.0493077902663,
-12.8505636606085));
#11251=CARTESIAN_POINT('Ctrl Pts',(-14.2141062803874,-23.0570717757524,
-12.8865523273134));
#11252=CARTESIAN_POINT('Ctrl Pts',(-14.1714946425131,-23.0649868063146,
-12.9225981186239));
#11253=CARTESIAN_POINT('Ctrl Pts',(-14.1289648910311,-23.073025554129,-12.9586884632117));
#11254=CARTESIAN_POINT('Ctrl Pts',(-14.1063091778062,-23.0773078167528,
-12.9779138870309));
#11255=CARTESIAN_POINT('Ctrl Pts',(-14.0836619794504,-23.0816279527543,
-12.9971620609415));
#11256=CARTESIAN_POINT('Ctrl Pts',(-14.0610235009594,-23.0859836968888,
-13.0164313773492));
#11257=CARTESIAN_POINT('Ctrl Pts',(-13.9623148504585,-23.1049756810725,
-13.1004497542657));
#11258=CARTESIAN_POINT('Ctrl Pts',(-13.8638917090216,-23.1246111362285,
-13.1847758715363));
#11259=CARTESIAN_POINT('Ctrl Pts',(-13.7657307804515,-23.144727844216,-13.2693057994777));
#11260=CARTESIAN_POINT('Ctrl Pts',(-13.6542237888969,-23.1675796409578,
-13.3653285052362));
#11261=CARTESIAN_POINT('Ctrl Pts',(-13.5430552110511,-23.1910529746138,
-13.4616142220801));
#11262=CARTESIAN_POINT('Ctrl Pts',(-13.4321665793915,-23.2149438103394,
-13.5580681722366));
#11263=CARTESIAN_POINT('Ctrl Pts',(-13.3083031983276,-23.2416300417875,
-13.6658079125919));
#11264=CARTESIAN_POINT('Ctrl Pts',(-13.1847890370931,-23.2688383565652,
-13.7737585323181));
#11265=CARTESIAN_POINT('Ctrl Pts',(-13.0615143154905,-23.2963096837132,
-13.8818478660677));
#11266=CARTESIAN_POINT('Ctrl Pts',(-12.9075190646744,-23.3306269700103,
-14.0168734726555));
#11267=CARTESIAN_POINT('Ctrl Pts',(-12.753897994041,-23.3653575841868,-14.1521192203606));
#11268=CARTESIAN_POINT('Ctrl Pts',(-12.6003906189451,-23.4,-14.2875));
#11269=CARTESIAN_POINT('',(-12.6003906189451,-23.4,14.2875));
#11270=CARTESIAN_POINT('Origin',(0.,-23.4,0.));
#11271=CARTESIAN_POINT('Ctrl Pts',(-12.6003906189451,-23.4,14.2875));
#11272=CARTESIAN_POINT('Ctrl Pts',(-12.7464264885013,-23.3670436986217,
14.1587084688864));
#11273=CARTESIAN_POINT('Ctrl Pts',(-12.8925091205016,-23.3340202714665,
14.0300885565564));
#11274=CARTESIAN_POINT('Ctrl Pts',(-13.0388879454113,-23.3013555121465,
13.9016909069208));
#11275=CARTESIAN_POINT('Ctrl Pts',(-13.1577552213119,-23.2748300159846,
13.7974252875346));
#11276=CARTESIAN_POINT('Ctrl Pts',(-13.2768176295818,-23.2485394307436,
13.6933041193317));
#11277=CARTESIAN_POINT('Ctrl Pts',(-13.396189169292,-23.22271182669,13.5893765986257));
#11278=CARTESIAN_POINT('Ctrl Pts',(-13.5063781591052,-23.1988709881879,
13.4934436103423));
#11279=CARTESIAN_POINT('Ctrl Pts',(-13.6168307216849,-23.1754236715566,
13.3976746320453));
#11280=CARTESIAN_POINT('Ctrl Pts',(-13.7276174642274,-23.1525653653853,
13.3021479753249));
#11281=CARTESIAN_POINT('Ctrl Pts',(-13.8247719233332,-23.1325197685822,
13.2183758519566));
#11282=CARTESIAN_POINT('Ctrl Pts',(-13.9221833399697,-23.112926758599,13.1347900642995));
#11283=CARTESIAN_POINT('Ctrl Pts',(-14.0198835650604,-23.093939320451,13.0514803619139));
#11284=CARTESIAN_POINT('Ctrl Pts',(-14.0335924279632,-23.0912750872191,
13.0397907134262));
#11285=CARTESIAN_POINT('Ctrl Pts',(-14.0473069490115,-23.0886228201808,
13.0281065672791));
#11286=CARTESIAN_POINT('Ctrl Pts',(-14.0610271875519,-23.0859829876025,
13.0164282393766));
#11287=CARTESIAN_POINT('Ctrl Pts',(-14.0836644383102,-23.0816274837344,
12.9971599710891));
#11288=CARTESIAN_POINT('Ctrl Pts',(-14.1063104077805,-23.0773075842938,
12.9779128432561));
#11289=CARTESIAN_POINT('Ctrl Pts',(-14.1289648910289,-23.0730255541512,
12.9586884631858));
#11290=CARTESIAN_POINT('Ctrl Pts',(-14.2229511453529,-23.0552607713666,
12.8789326173029));
#11291=CARTESIAN_POINT('Ctrl Pts',(-14.317337519555,-23.0380976121144,12.7993922304769));
#11292=CARTESIAN_POINT('Ctrl Pts',(-14.412250550128,-23.0218415529598,12.7202117113694));
#11293=CARTESIAN_POINT('Ctrl Pts',(-14.5015541210375,-23.0065462439525,
12.6457108439954));
#11294=CARTESIAN_POINT('Ctrl Pts',(-14.5913239111188,-22.9920537993316,
12.5715284490981));
#11295=CARTESIAN_POINT('Ctrl Pts',(-14.6816626146348,-22.9786542883986,
12.4978139961358));
#11296=CARTESIAN_POINT('Ctrl Pts',(-14.7239440666521,-22.9723828813878,
12.4633132341744));
#11297=CARTESIAN_POINT('Ctrl Pts',(-14.7663501039695,-22.9663514277299,
12.4289154174509));
#11298=CARTESIAN_POINT('Ctrl Pts',(-14.8088910547694,-22.960592775276,12.3946383857669));
#11299=CARTESIAN_POINT('Ctrl Pts',(-14.8302213972738,-22.9577053450025,
12.3774516324831));
#11300=CARTESIAN_POINT('Ctrl Pts',(-14.8516165328029,-22.9548823672323,
12.3602702965515));
#11301=CARTESIAN_POINT('Ctrl Pts',(-14.8730816744606,-22.9521283805007,
12.3430942072107));
#11302=CARTESIAN_POINT('Ctrl Pts',(-14.9355475058829,-22.9441139879725,
12.2931099714499));
#11303=CARTESIAN_POINT('Ctrl Pts',(-14.9981564314485,-22.9367118504461,
12.2435306733137));
#11304=CARTESIAN_POINT('Ctrl Pts',(-15.0610456073057,-22.93012990807,12.1943674230766));
#11305=CARTESIAN_POINT('Ctrl Pts',(-15.1217130745985,-22.9237804883426,
12.1469409806861));
#11306=CARTESIAN_POINT('Ctrl Pts',(-15.1826412140633,-22.9181939831412,
12.099901655222));
#11307=CARTESIAN_POINT('Ctrl Pts',(-15.2439503751515,-22.9135965970105,
12.0532836297194));
#11308=CARTESIAN_POINT('Ctrl Pts',(-15.301993125592,-22.9092441490055,12.0091493050565));
#11309=CARTESIAN_POINT('Ctrl Pts',(-15.3603772739025,-22.9057780702211,
11.9653926114926));
#11310=CARTESIAN_POINT('Ctrl Pts',(-15.4192040486566,-22.9034297890288,
11.92206471413));
#11311=CARTESIAN_POINT('Ctrl Pts',(-15.4745612083561,-22.9012200099355,
11.8812923049035));
#11312=CARTESIAN_POINT('Ctrl Pts',(-15.5303102445029,-22.9,11.8408996544229));
#11313=CARTESIAN_POINT('Ctrl Pts',(-15.5865359611318,-22.9,11.8009489759233));
#11314=CARTESIAN_POINT('Origin',(0.,-25.4,0.));
#11315=CARTESIAN_POINT('Ctrl Pts',(-1.69645946028209E-13,-23.936276920587,
-8.326));
#11316=CARTESIAN_POINT('Ctrl Pts',(-0.0274010994650395,-23.9352793807263,
-8.326));
#11317=CARTESIAN_POINT('Ctrl Pts',(-0.0548082522194444,-23.9342787773939,
-8.32586473338683));
#11318=CARTESIAN_POINT('Ctrl Pts',(-1.14031167491963,-23.8945355941156,
-8.31514470485895));
#11319=CARTESIAN_POINT('Ctrl Pts',(-2.18666730607269,-23.8519857556232,
-8.10308607630245));
#11320=CARTESIAN_POINT('Ctrl Pts',(-4.18172956133545,-23.7621201564241,
-7.28308681563853));
#11321=CARTESIAN_POINT('Ctrl Pts',(-5.10558039539358,-23.7155608683631,
-6.66808549943798));
#11322=CARTESIAN_POINT('Ctrl Pts',(-6.64725277062572,-23.6270772146309,
-5.12854094782683));
#11323=CARTESIAN_POINT('Ctrl Pts',(-7.25548788820093,-23.5888585730357,
-4.22441382368631));
#11324=CARTESIAN_POINT('Ctrl Pts',(-8.08933343975371,-23.5055600699609,
-2.24286143339713));
#11325=CARTESIAN_POINT('Ctrl Pts',(-8.31034359466962,-23.4611158669201,
-1.18559733477432));
#11326=CARTESIAN_POINT('Ctrl Pts',(-8.34064497983556,-23.3693592227615,
0.997162148839258));
#11327=CARTESIAN_POINT('Ctrl Pts',(-8.13284787200331,-23.3229214829502,
2.10184963932125));
#11328=CARTESIAN_POINT('Ctrl Pts',(-7.3163309983539,-23.2384100139353,4.1122567565138));
#11329=CARTESIAN_POINT('Ctrl Pts',(-6.7358412207762,-23.2012608476925,5.00678392849045));
#11330=CARTESIAN_POINT('Ctrl Pts',(-5.25329289484859,-23.1148604650577,
6.54961825083766));
#11331=CARTESIAN_POINT('Ctrl Pts',(-4.35797920905201,-23.0690898974778,
7.17652229072915));
#11332=CARTESIAN_POINT('Ctrl Pts',(-2.35933360070256,-22.9777488620224,
8.06051204332207));
#11333=CARTESIAN_POINT('Ctrl Pts',(-1.27209948259276,-22.9330956672779,
8.3018387364197));
#11334=CARTESIAN_POINT('Ctrl Pts',(0.885423436170803,-22.8536280810239,
8.34574012634027));
#11335=CARTESIAN_POINT('Ctrl Pts',(1.93493869722947,-22.812483370607,8.1665258638054));
#11336=CARTESIAN_POINT('Ctrl Pts',(3.94897071169433,-22.7232897406262,7.41135356538661));
#11337=CARTESIAN_POINT('Ctrl Pts',(4.88886987738679,-22.6768113197837,6.82799620615969));
#11338=CARTESIAN_POINT('Ctrl Pts',(6.48385244888632,-22.587375526442,5.33548754082332));
#11339=CARTESIAN_POINT('Ctrl Pts',(7.12517942377867,-22.5480430338092,4.44289902482894));
#11340=CARTESIAN_POINT('Ctrl Pts',(8.01906609183926,-22.4655737864135,2.48107344249377));
#11341=CARTESIAN_POINT('Ctrl Pts',(8.27070775145324,-22.421555858589,1.43394982230191));
#11342=CARTESIAN_POINT('Ctrl Pts',(8.36689005008122,-22.3301593565971,-0.740242393655139));
#11343=CARTESIAN_POINT('Ctrl Pts',(8.19395271794373,-22.2836256801925,-1.84721207863885));
#11344=CARTESIAN_POINT('Ctrl Pts',(7.44127053091648,-22.1980621863545,-3.8826453634813));
#11345=CARTESIAN_POINT('Ctrl Pts',(6.88668076886145,-22.1611398532551,-4.79803083062937));
#11346=CARTESIAN_POINT('Ctrl Pts',(5.4511003404151,-22.0755137687582,-6.38537704461722));
#11347=CARTESIAN_POINT('Ctrl Pts',(4.57822428142744,-22.0300287619124,-7.03755803030118));
#11348=CARTESIAN_POINT('Ctrl Pts',(2.61110659379847,-21.9385536544961,-7.98253450427656));
#11349=CARTESIAN_POINT('Ctrl Pts',(1.53179329320156,-21.8934735716324,-8.25789057277571));
#11350=CARTESIAN_POINT('Ctrl Pts',(0.286737659835875,-21.8467934011162,
-8.32230009878138));
#11351=CARTESIAN_POINT('Ctrl Pts',(0.143308012216421,-21.8414940635969,
-8.326));
#11352=CARTESIAN_POINT('Ctrl Pts',(3.32268934588598E-13,-21.836276920587,
-8.326));
#11353=CARTESIAN_POINT('Ctrl Pts',(-2.01505478969466E-13,-22.2372253046546,
-8.32600000000001));
#11354=CARTESIAN_POINT('Ctrl Pts',(0.926857554021544,-22.2709676497922,
-8.32600000000003));
#11355=CARTESIAN_POINT('Ctrl Pts',(1.84844442910887,-22.3077708387169,-8.17124471417512));
#11356=CARTESIAN_POINT('Ctrl Pts',(3.75781019274245,-22.3911906936277,-7.50948487280907));
#11357=CARTESIAN_POINT('Ctrl Pts',(4.7087912106428,-22.437512891261,-6.95275449859051));
#11358=CARTESIAN_POINT('Ctrl Pts',(6.31349671328978,-22.5258529063643,-5.52922044179108));
#11359=CARTESIAN_POINT('Ctrl Pts',(6.96175792246993,-22.5652067461283,-4.68679005226099));
#11360=CARTESIAN_POINT('Ctrl Pts',(7.93204417654554,-22.6461706110426,-2.76077536861622));
#11361=CARTESIAN_POINT('Ctrl Pts',(8.22760832882724,-22.6913177186374,-1.68679017480437));
#11362=CARTESIAN_POINT('Ctrl Pts',(8.38131717801809,-22.7828063553502,0.489593794539997));
#11363=CARTESIAN_POINT('Ctrl Pts',(8.24743933582676,-22.8282395216875,1.57038391718162));
#11364=CARTESIAN_POINT('Ctrl Pts',(7.58017435530881,-22.9137339484021,3.60417419382718));
#11365=CARTESIAN_POINT('Ctrl Pts',(7.05946358391859,-22.950652170909,4.54016153542568));
#11366=CARTESIAN_POINT('Ctrl Pts',(5.66405929039187,-23.0363904243803,6.2024315356574));
#11367=CARTESIAN_POINT('Ctrl Pts',(4.78867770309699,-23.0829359327552,6.9007284517633));
#11368=CARTESIAN_POINT('Ctrl Pts',(2.8535562941473,-23.1742635426255,7.89410659424699));
#11369=CARTESIAN_POINT('Ctrl Pts',(1.81988991642697,-23.2182057915544,8.19439056473317));
#11370=CARTESIAN_POINT('Ctrl Pts',(-0.328193483426126,-23.3005326623219,
8.39067826878061));
#11371=CARTESIAN_POINT('Ctrl Pts',(-1.42300337566758,-23.3400880033768,
8.27565797708005));
#11372=CARTESIAN_POINT('Ctrl Pts',(-3.51053754999324,-23.4296825252423,
7.62872186353711));
#11373=CARTESIAN_POINT('Ctrl Pts',(-4.48229778555067,-23.476142544793,7.1014249769915));
#11374=CARTESIAN_POINT('Ctrl Pts',(-6.13526565951377,-23.56521591143,5.72659302872137));
#11375=CARTESIAN_POINT('Ctrl Pts',(-6.81067217932797,-23.6060752175234,
4.90401607272714));
#11376=CARTESIAN_POINT('Ctrl Pts',(-7.8414195696069,-23.6857577215008,3.00848313525754));
#11377=CARTESIAN_POINT('Ctrl Pts',(-8.17051718871768,-23.7304848812186,
1.9444879015138));
#11378=CARTESIAN_POINT('Ctrl Pts',(-8.39290191134532,-23.8218544804352,
-0.229064335848684));
#11379=CARTESIAN_POINT('Ctrl Pts',(-8.29212825200708,-23.8675805364092,
-1.31682188453286));
#11380=CARTESIAN_POINT('Ctrl Pts',(-7.6869662415816,-23.9538538822449,-3.36914153432897));
#11381=CARTESIAN_POINT('Ctrl Pts',(-7.1974269872857,-23.9909416216189,-4.3171209688485));
#11382=CARTESIAN_POINT('Ctrl Pts',(-5.85575574791044,-24.0756285643245,
-6.02244098643312));
#11383=CARTESIAN_POINT('Ctrl Pts',(-4.99970398980033,-24.122085170087,-6.74998841649908));
#11384=CARTESIAN_POINT('Ctrl Pts',(-3.08989128939176,-24.2137880707544,
-7.80505779191651));
#11385=CARTESIAN_POINT('Ctrl Pts',(-2.06262619271256,-24.2581645704731,
-8.13708951824372));
#11386=CARTESIAN_POINT('Ctrl Pts',(-0.667929305579545,-24.3124874043931,
-8.30592887838815));
#11387=CARTESIAN_POINT('Ctrl Pts',(-0.333789202319721,-24.3250736742137,
-8.326));
#11388=CARTESIAN_POINT('Ctrl Pts',(-1.72639680329212E-13,-24.3372253046546,
-8.32600000000001));
#11389=CARTESIAN_POINT('Origin',(8.05147737193781,-7.025,-39.3455678841871));
#11390=CARTESIAN_POINT('',(6.45147737193779,-7.025,-36.5742865920769));
#11391=CARTESIAN_POINT('Origin',(8.05147737193781,-7.025,-39.3455678841871));
#11392=CARTESIAN_POINT('',(28.4485226280625,-7.025,-23.8742865920768));
#11393=CARTESIAN_POINT('',(6.4514773719378,-7.025,-36.5742865920769));
#11394=CARTESIAN_POINT('Origin',(30.0485226280625,-7.025,-26.645567884187));
#11395=CARTESIAN_POINT('Origin',(30.0485226280621,-7.025,26.6455678841874));
#11396=CARTESIAN_POINT('',(28.4485226280621,-7.025,23.8742865920772));
#11397=CARTESIAN_POINT('Origin',(30.0485226280621,-7.025,26.6455678841874));
#11398=CARTESIAN_POINT('',(6.45147737193728,-7.025,36.574286592077));
#11399=CARTESIAN_POINT('',(28.4485226280621,-7.025,23.8742865920772));
#11400=CARTESIAN_POINT('Origin',(8.05147737193726,-7.025,39.3455678841872));
#11401=CARTESIAN_POINT('Origin',(-38.1,-7.025,12.7));
#11402=CARTESIAN_POINT('',(-34.9,-7.025,12.7));
#11403=CARTESIAN_POINT('Origin',(-38.1,-7.025,12.7));
#11404=CARTESIAN_POINT('',(-34.9,-7.025,-12.7));
#11405=CARTESIAN_POINT('',(-34.9,-7.025,12.7));
#11406=CARTESIAN_POINT('Origin',(-38.1,-7.025,-12.7));
#11407=CARTESIAN_POINT('Origin',(0.,25.4,0.));
#11408=CARTESIAN_POINT('',(-2.33295215237571E-15,25.4,19.05));
#11409=CARTESIAN_POINT('',(-6.07314264709777,13.15,18.0560083736135));
#11410=CARTESIAN_POINT('',(-6.07314264709777,25.4,18.0560083736135));
#11411=CARTESIAN_POINT('',(-2.33295215237571E-15,13.15,19.05));
#11412=CARTESIAN_POINT('Origin',(0.,13.15,0.));
#11413=CARTESIAN_POINT('',(-2.33295215237571E-15,25.4,19.05));
#11414=CARTESIAN_POINT('',(18.6735332660427,13.15,3.76850837361377));
#11415=CARTESIAN_POINT('Origin',(0.,13.15,0.));
#11416=CARTESIAN_POINT('',(18.6735332660427,25.4,3.76850837361377));
#11417=CARTESIAN_POINT('',(-6.07314264709753,-23.4,-18.0560083736136));
#11418=CARTESIAN_POINT('',(-6.07314264709754,25.4,-18.0560083736136));
#11419=CARTESIAN_POINT('',(18.6735332660427,-23.4,-3.76850837361349));
#11420=CARTESIAN_POINT('Origin',(0.,-23.4,0.));
#11421=CARTESIAN_POINT('',(18.6735332660427,25.4,-3.76850837361349));
#11422=CARTESIAN_POINT('',(-12.6003906189451,13.15,14.2875));
#11423=CARTESIAN_POINT('',(-12.6003906189451,25.4,14.2875));
#11424=CARTESIAN_POINT('',(-12.6003906189451,13.15,-14.2875));
#11425=CARTESIAN_POINT('',(-12.6003906189451,25.4,-14.2875));
#11426=CARTESIAN_POINT('Origin',(0.,13.15,0.));
#11427=CARTESIAN_POINT('Origin',(0.,25.4,0.));
#11428=CARTESIAN_POINT('',(-9.525,25.4,5.49926131403119));
#11429=CARTESIAN_POINT('',(-1.73472347597681E-15,25.4,10.9985226280624));
#11430=CARTESIAN_POINT('Origin',(0.,25.4,0.));
#11431=CARTESIAN_POINT('',(9.525,25.4,5.49926131403118));
#11432=CARTESIAN_POINT('Origin',(0.,25.4,0.));
#11433=CARTESIAN_POINT('',(9.525,25.4,-5.49926131403119));
#11434=CARTESIAN_POINT('Origin',(0.,25.4,0.));
#11435=CARTESIAN_POINT('',(0.,25.4,-10.9985226280624));
#11436=CARTESIAN_POINT('Origin',(0.,25.4,0.));
#11437=CARTESIAN_POINT('',(-9.525,25.4,-5.49926131403119));
#11438=CARTESIAN_POINT('Origin',(0.,25.4,0.));
#11439=CARTESIAN_POINT('Origin',(0.,25.4,0.));
#11440=CARTESIAN_POINT('Origin',(-6.35,15.4,10.9985226280624));
#11441=CARTESIAN_POINT('',(-5.19529946162075,24.727212412536,10.9985226280624));
#11442=CARTESIAN_POINT('',(-5.19529946162075,16.4,10.9985226280624));
#11443=CARTESIAN_POINT('',(-5.19529946162075,15.4,10.9985226280624));
#11444=CARTESIAN_POINT('',(5.19529946162075,16.4,10.9985226280624));
#11445=CARTESIAN_POINT('',(5.19529946162075,16.4,10.9985226280624));
#11446=CARTESIAN_POINT('',(5.19529946162075,24.727212412536,10.9985226280624));
#11447=CARTESIAN_POINT('',(5.19529946162075,15.4,10.9985226280624));
#11448=CARTESIAN_POINT('Ctrl Pts',(5.19529946162091,24.7272124125359,10.9985226280624));
#11449=CARTESIAN_POINT('Ctrl Pts',(2.46696145927109,25.4,10.9985226280624));
#11450=CARTESIAN_POINT('Ctrl Pts',(-5.96292472080612E-15,25.4,10.9985226280624));
#11451=CARTESIAN_POINT('Ctrl Pts',(-5.96292472080612E-15,25.4,10.9985226280624));
#11452=CARTESIAN_POINT('Ctrl Pts',(-2.4669614592711,25.4,10.9985226280624));
#11453=CARTESIAN_POINT('Ctrl Pts',(-5.19529946162091,24.7272124125359,10.9985226280624));
#11454=CARTESIAN_POINT('Origin',(-12.7,15.4,3.66198162423638E-16));
#11455=CARTESIAN_POINT('',(-12.1226497308104,24.727212412536,0.999999999999998));
#11456=CARTESIAN_POINT('',(-12.1226497308104,16.4,0.999999999999999));
#11457=CARTESIAN_POINT('',(-12.1226497308104,15.4,0.999999999999999));
#11458=CARTESIAN_POINT('',(-6.92735026918963,16.4,9.99852262806237));
#11459=CARTESIAN_POINT('',(-6.92735026918962,16.4,9.99852262806237));
#11460=CARTESIAN_POINT('',(-6.92735026918963,24.727212412536,9.99852262806237));
#11461=CARTESIAN_POINT('',(-6.92735026918963,15.4,9.99852262806237));
#11462=CARTESIAN_POINT('Ctrl Pts',(-6.92735026918955,24.7272124125359,9.99852262806251));
#11463=CARTESIAN_POINT('Ctrl Pts',(-8.29151927036445,25.4,7.63571260791709));
#11464=CARTESIAN_POINT('Ctrl Pts',(-9.525,25.4,5.4992613140312));
#11465=CARTESIAN_POINT('Ctrl Pts',(-9.525,25.4,5.4992613140312));
#11466=CARTESIAN_POINT('Ctrl Pts',(-10.7584807296355,25.4,3.36281002014529));
#11467=CARTESIAN_POINT('Ctrl Pts',(-12.1226497308105,24.7272124125359,0.999999999999857));
#11468=CARTESIAN_POINT('Origin',(-6.35,15.4,-10.9985226280624));
#11469=CARTESIAN_POINT('',(-6.92735026918963,24.727212412536,-9.99852262806237));
#11470=CARTESIAN_POINT('',(-6.92735026918963,16.4,-9.99852262806237));
#11471=CARTESIAN_POINT('',(-6.92735026918963,15.4,-9.99852262806237));
#11472=CARTESIAN_POINT('',(-12.1226497308104,16.4,-1.));
#11473=CARTESIAN_POINT('',(-12.1226497308104,16.4,-0.999999999999998));
#11474=CARTESIAN_POINT('',(-12.1226497308104,24.727212412536,-1.));
#11475=CARTESIAN_POINT('',(-12.1226497308104,15.4,-1.));
#11476=CARTESIAN_POINT('Ctrl Pts',(-12.1226497308105,24.7272124125359,-0.99999999999986));
#11477=CARTESIAN_POINT('Ctrl Pts',(-10.7584807296355,25.4,-3.36281002014529));
#11478=CARTESIAN_POINT('Ctrl Pts',(-9.525,25.4,-5.4992613140312));
#11479=CARTESIAN_POINT('Ctrl Pts',(-9.525,25.4,-5.4992613140312));
#11480=CARTESIAN_POINT('Ctrl Pts',(-8.29151927036445,25.4,-7.63571260791709));
#11481=CARTESIAN_POINT('Ctrl Pts',(-6.92735026918955,24.7272124125359,-9.9985226280625));
#11482=CARTESIAN_POINT('Origin',(6.35,15.4,-10.9985226280624));
#11483=CARTESIAN_POINT('',(5.19529946162075,24.727212412536,-10.9985226280624));
#11484=CARTESIAN_POINT('',(5.19529946162075,16.4,-10.9985226280624));
#11485=CARTESIAN_POINT('',(5.19529946162075,15.4,-10.9985226280624));
#11486=CARTESIAN_POINT('',(-5.19529946162075,16.4,-10.9985226280624));
#11487=CARTESIAN_POINT('',(-5.19529946162075,16.4,-10.9985226280624));
#11488=CARTESIAN_POINT('',(-5.19529946162075,24.727212412536,-10.9985226280624));
#11489=CARTESIAN_POINT('',(-5.19529946162075,15.4,-10.9985226280624));
#11490=CARTESIAN_POINT('Ctrl Pts',(-5.19529946162091,24.7272124125359,-10.9985226280624));
#11491=CARTESIAN_POINT('Ctrl Pts',(-2.4669614592711,25.4,-10.9985226280624));
#11492=CARTESIAN_POINT('Ctrl Pts',(-5.96292472080612E-15,25.4,-10.9985226280624));
#11493=CARTESIAN_POINT('Ctrl Pts',(-5.96292472080612E-15,25.4,-10.9985226280624));
#11494=CARTESIAN_POINT('Ctrl Pts',(2.4669614592711,25.4,-10.9985226280624));
#11495=CARTESIAN_POINT('Ctrl Pts',(5.19529946162093,24.7272124125359,-10.9985226280624));
#11496=CARTESIAN_POINT('Origin',(12.7,15.4,-6.93499540769888E-15));
#11497=CARTESIAN_POINT('',(12.1226497308104,24.727212412536,-1.));
#11498=CARTESIAN_POINT('',(12.1226497308104,16.4,-1.00000000000001));
#11499=CARTESIAN_POINT('',(12.1226497308104,15.4,-1.00000000000001));
#11500=CARTESIAN_POINT('',(6.92735026918963,16.4,-9.99852262806237));
#11501=CARTESIAN_POINT('',(6.92735026918962,16.4,-9.99852262806237));
#11502=CARTESIAN_POINT('',(6.92735026918963,24.727212412536,-9.99852262806237));
#11503=CARTESIAN_POINT('',(6.92735026918963,15.4,-9.99852262806237));
#11504=CARTESIAN_POINT('Ctrl Pts',(6.92735026918955,24.7272124125359,-9.99852262806251));
#11505=CARTESIAN_POINT('Ctrl Pts',(8.29151927036445,25.4,-7.6357126079171));
#11506=CARTESIAN_POINT('Ctrl Pts',(9.52499999999999,25.4,-5.49926131403121));
#11507=CARTESIAN_POINT('Ctrl Pts',(9.52499999999999,25.4,-5.49926131403121));
#11508=CARTESIAN_POINT('Ctrl Pts',(10.7584807296355,25.4,-3.36281002014531));
#11509=CARTESIAN_POINT('Ctrl Pts',(12.1226497308104,24.7272124125359,-0.999999999999882));
#11510=CARTESIAN_POINT('Origin',(6.35,15.4,10.9985226280624));
#11511=CARTESIAN_POINT('',(6.92735026918962,24.727212412536,9.99852262806237));
#11512=CARTESIAN_POINT('',(6.92735026918962,16.4,9.99852262806237));
#11513=CARTESIAN_POINT('',(6.92735026918962,15.4,9.99852262806237));
#11514=CARTESIAN_POINT('',(12.1226497308104,16.4,0.999999999999996));
#11515=CARTESIAN_POINT('',(12.1226497308104,16.4,0.999999999999996));
#11516=CARTESIAN_POINT('',(12.1226497308104,24.727212412536,0.999999999999994));
#11517=CARTESIAN_POINT('',(12.1226497308104,15.4,0.999999999999996));
#11518=CARTESIAN_POINT('Ctrl Pts',(12.1226497308105,24.7272124125359,0.999999999999861));
#11519=CARTESIAN_POINT('Ctrl Pts',(10.7584807296355,25.4,3.36281002014528));
#11520=CARTESIAN_POINT('Ctrl Pts',(9.525,25.4,5.49926131403118));
#11521=CARTESIAN_POINT('Ctrl Pts',(9.525,25.4,5.49926131403118));
#11522=CARTESIAN_POINT('Ctrl Pts',(8.29151927036445,25.4,7.63571260791708));
#11523=CARTESIAN_POINT('Ctrl Pts',(6.92735026918955,24.7272124125359,9.9985226280625));
#11524=CARTESIAN_POINT('Origin',(0.,-25.4,0.));
#11525=CARTESIAN_POINT('',(5.8718173029053,-25.4,-8.00113003034161));
#11526=CARTESIAN_POINT('',(6.22809017016564,-25.4,6.25373239212283));
#11527=CARTESIAN_POINT('Ctrl Pts',(5.87181730290515,-25.4,-8.00113003034174));
#11528=CARTESIAN_POINT('Ctrl Pts',(6.41997597897823,-25.4,-7.53910516553241));
#11529=CARTESIAN_POINT('Ctrl Pts',(6.91671183935199,-25.4,-7.01935260004522));
#11530=CARTESIAN_POINT('Ctrl Pts',(7.8176532996952,-25.4,-5.84670254590401));
#11531=CARTESIAN_POINT('Ctrl Pts',(8.21489293449085,-25.3999999996063,-5.18646211216675));
#11532=CARTESIAN_POINT('Ctrl Pts',(9.03044928377891,-25.3999999996063,-3.37939524432784));
#11533=CARTESIAN_POINT('Ctrl Pts',(9.30940044368467,-25.4,-2.17127523394385));
#11534=CARTESIAN_POINT('Ctrl Pts',(9.38117787326285,-25.4,0.257055530030207));
#11535=CARTESIAN_POINT('Ctrl Pts',(9.1837385826432,-25.4,1.45330461325936));
#11536=CARTESIAN_POINT('Ctrl Pts',(8.43719385355252,-25.4,3.45684341944329));
#11537=CARTESIAN_POINT('Ctrl Pts',(8.03460625325573,-25.4,4.1345974411627));
#11538=CARTESIAN_POINT('Ctrl Pts',(7.28968847710234,-25.4,5.21524977190067));
#11539=CARTESIAN_POINT('Ctrl Pts',(6.7912859412746,-25.4,5.76979234178763));
#11540=CARTESIAN_POINT('Ctrl Pts',(6.22809017016566,-25.4,6.25373239212283));
#11541=CARTESIAN_POINT('',(-7.7648517191704,-25.4,-4.1958734226972));
#11542=CARTESIAN_POINT('Ctrl Pts',(-7.76485171917045,-25.4,-4.19587342269709));
#11543=CARTESIAN_POINT('Ctrl Pts',(-7.5153669902019,-25.4,-4.74202422930472));
#11544=CARTESIAN_POINT('Ctrl Pts',(-7.11824932711354,-25.4,-5.46216308143309));
#11545=CARTESIAN_POINT('Ctrl Pts',(-6.02425805366761,-25.4,-6.78618608402815));
#11546=CARTESIAN_POINT('Ctrl Pts',(-5.47681493420003,-25.4,-7.30383758510192));
#11547=CARTESIAN_POINT('Ctrl Pts',(-3.95926137314159,-25.4,-8.42099215986769));
#11548=CARTESIAN_POINT('Ctrl Pts',(-2.92934762161546,-25.4000000000001,
-8.91762230918457));
#11549=CARTESIAN_POINT('Ctrl Pts',(-0.398296561048911,-25.4000000000001,
-9.60246458995361));
#11550=CARTESIAN_POINT('Ctrl Pts',(0.902188672117903,-25.4,-9.57961545600489));
#11551=CARTESIAN_POINT('Ctrl Pts',(2.60403764477334,-25.4,-9.3536353399083));
#11552=CARTESIAN_POINT('Ctrl Pts',(3.2999578043234,-25.4,-9.18265881085097));
#11553=CARTESIAN_POINT('Ctrl Pts',(4.63664497571866,-25.4,-8.69493921576204));
#11554=CARTESIAN_POINT('Ctrl Pts',(5.27387123787004,-25.4,-8.38091270986061));
#11555=CARTESIAN_POINT('Ctrl Pts',(5.87181730290536,-25.4,-8.00113003034165));
#11556=CARTESIAN_POINT('Origin',(0.,-25.4,0.));
#11557=CARTESIAN_POINT('Origin',(0.,-25.4,0.));
#11558=CARTESIAN_POINT('',(8.29083424217445,-24.9756402675196,1.3600098358447));
#11559=CARTESIAN_POINT('Ctrl Pts',(8.27736571547514,-24.8999999999998,0.898606038414263));
#11560=CARTESIAN_POINT('Ctrl Pts',(8.27792777712598,-24.9005058876881,0.898115980561187));
#11561=CARTESIAN_POINT('Ctrl Pts',(8.27851833941179,-24.9010467821481,0.897687233867645));
#11562=CARTESIAN_POINT('Ctrl Pts',(8.27968811062583,-24.9021422632964,0.897061021095975));
#11563=CARTESIAN_POINT('Ctrl Pts',(8.28025936483844,-24.9026872898312,0.896848287015314));
#11564=CARTESIAN_POINT('Ctrl Pts',(8.28167137333571,-24.9040642904923,0.896599354755583));
#11565=CARTESIAN_POINT('Ctrl Pts',(8.28247701078594,-24.9048744754402,0.896685085175965));
#11566=CARTESIAN_POINT('Ctrl Pts',(8.28424370644011,-24.9067065626039,0.897387848768569));
#11567=CARTESIAN_POINT('Ctrl Pts',(8.28512484299656,-24.9076604489329,0.898111048931224));
#11568=CARTESIAN_POINT('Ctrl Pts',(8.28727633454631,-24.9100640801295,0.900564978387333));
#11569=CARTESIAN_POINT('Ctrl Pts',(8.28841257360746,-24.9114278355422,0.902731407094527));
#11570=CARTESIAN_POINT('Ctrl Pts',(8.29319510537141,-24.9174019317703,0.913972293170574));
#11571=CARTESIAN_POINT('Ctrl Pts',(8.29589583640989,-24.9217968036879,0.929557055849718));
#11572=CARTESIAN_POINT('Ctrl Pts',(8.30405884437143,-24.9378851382505,1.00000457409689));
#11573=CARTESIAN_POINT('Ctrl Pts',(8.30347691095396,-24.947772881011,1.08337191045941));
#11574=CARTESIAN_POINT('Ctrl Pts',(8.30147063765394,-24.96111035307,1.19797632784268));
#11575=CARTESIAN_POINT('Ctrl Pts',(8.29692634943919,-24.9688790701265,1.28110320078678));
#11576=CARTESIAN_POINT('Ctrl Pts',(8.29083424217439,-24.9756402675196,1.36000983584488));
#11577=CARTESIAN_POINT('Ctrl Pts',(8.29083424217443,-24.9756402675196,1.36000983584492));
#11578=CARTESIAN_POINT('Ctrl Pts',(8.22153300492422,-25.0525527912602,2.25761836423918));
#11579=CARTESIAN_POINT('Ctrl Pts',(8.00586925271954,-25.1258907620308,3.13818145654568));
#11580=CARTESIAN_POINT('Ctrl Pts',(7.35437567063969,-25.2503896474066,4.66543782159151));
#11581=CARTESIAN_POINT('Ctrl Pts',(6.89843763491226,-25.3178303686065,5.47016614476703));
#11582=CARTESIAN_POINT('Ctrl Pts',(6.22809017016576,-25.4,6.25373239212268));
#11583=CARTESIAN_POINT('',(-1.22646583495775,-24.9756402675196,8.31163887211714));
#11584=CARTESIAN_POINT('Ctrl Pts',(-7.76485171917038,-25.4,-4.19587342269725));
#11585=CARTESIAN_POINT('Ctrl Pts',(-8.1625641051082,-25.3799542890918,-3.41770382146533));
#11586=CARTESIAN_POINT('Ctrl Pts',(-8.44096609023593,-25.3583447746017,
-2.58416658384216));
#11587=CARTESIAN_POINT('Ctrl Pts',(-8.73067322640372,-25.3148141240392,
-0.918583409896716));
#11588=CARTESIAN_POINT('Ctrl Pts',(-8.75681063341049,-25.2932206376699,
-0.0982451433149351));
#11589=CARTESIAN_POINT('Ctrl Pts',(-8.55253607540217,-25.2434905757203,
1.7768193962029));
#11590=CARTESIAN_POINT('Ctrl Pts',(-8.24197358540638,-25.2158150895935,
2.80962671360843));
#11591=CARTESIAN_POINT('Ctrl Pts',(-7.49207553268971,-25.1764653617559,
4.26541248529107));
#11592=CARTESIAN_POINT('Ctrl Pts',(-7.18187287266752,-25.1634972947921,
4.7463215114945));
#11593=CARTESIAN_POINT('Ctrl Pts',(-6.17167919809883,-25.1235000651364,
6.0077427917133));
#11594=CARTESIAN_POINT('Ctrl Pts',(-5.3745473042224,-25.0957922580711,6.69504056537595));
#11595=CARTESIAN_POINT('Ctrl Pts',(-3.98322276197756,-25.0521915511955,
7.5056283585964));
#11596=CARTESIAN_POINT('Ctrl Pts',(-3.46631461954251,-25.0367984221239,
7.74108627138892));
#11597=CARTESIAN_POINT('Ctrl Pts',(-2.37691369428902,-25.0059102608247,
8.11098499338516));
#11598=CARTESIAN_POINT('Ctrl Pts',(-1.80610835590355,-24.9905087719593,
8.2411362995407));
#11599=CARTESIAN_POINT('Ctrl Pts',(-1.22646583495779,-24.9756402675196,
8.31163887211713));
#11600=CARTESIAN_POINT('Ctrl Pts',(-1.22646583495773,-24.9756402675196,
8.31163887211714));
#11601=CARTESIAN_POINT('Ctrl Pts',(-0.655124605969128,-24.9609847008681,
8.38113174920447));
#11602=CARTESIAN_POINT('Ctrl Pts',(-0.0736308671996442,-24.9483146439235,
8.39393002745997));
#11603=CARTESIAN_POINT('Ctrl Pts',(1.0776057392628,-24.9235712832695,8.29979327199434));
#11604=CARTESIAN_POINT('Ctrl Pts',(1.64605625058501,-24.911464890879,8.19367679821349));
#11605=CARTESIAN_POINT('Ctrl Pts',(2.19919404320639,-24.9,8.03030644249182));
#11606=CARTESIAN_POINT('Origin',(-48.,-7.90000000000001,12.7));
#11607=CARTESIAN_POINT('',(-48.,-7.90000000000001,12.7));
#11608=CARTESIAN_POINT('',(-48.,-21.9,12.7));
#11609=CARTESIAN_POINT('',(-48.,-7.90000000000001,12.7));
#11610=CARTESIAN_POINT('',(-16.8005208252602,-21.9,12.7));
#11611=CARTESIAN_POINT('',(-48.,-21.9,12.7));
#11612=CARTESIAN_POINT('',(-16.8005208252602,7.75488674445212,12.7));
#11613=CARTESIAN_POINT('',(-16.8005208252602,12.65,12.7));
#11614=CARTESIAN_POINT('',(-17.9697662756086,7.65,12.7));
#11615=CARTESIAN_POINT('Origin',(-24.2765469920838,163.404688042985,12.7));
#11616=CARTESIAN_POINT('',(-34.1050004454305,7.65,12.7));
#11617=CARTESIAN_POINT('',(-48.,7.65,12.7));
#11618=CARTESIAN_POINT('',(-48.,-7.90000000000001,12.7));
#11619=CARTESIAN_POINT('Origin',(-48.,-7.90000000000001,-12.7));
#11620=CARTESIAN_POINT('',(-16.8005208252602,7.75488674445212,-12.7));
#11621=CARTESIAN_POINT('',(-16.8005208252602,-21.9,-12.7));
#11622=CARTESIAN_POINT('',(-16.8005208252602,-7.90000000000001,-12.7));
#11623=CARTESIAN_POINT('',(-48.,-21.9,-12.7));
#11624=CARTESIAN_POINT('',(-48.,-21.9,-12.7));
#11625=CARTESIAN_POINT('',(-48.,-7.90000000000001,-12.7));
#11626=CARTESIAN_POINT('',(-48.,-7.90000000000001,-12.7));
#11627=CARTESIAN_POINT('',(-34.1050004454305,7.65,-12.7));
#11628=CARTESIAN_POINT('',(-33.5086522928671,8.31737776679611,-12.7));
#11629=CARTESIAN_POINT('',(-17.9697662756086,7.65,-12.7));
#11630=CARTESIAN_POINT('',(-16.8005208252602,7.65,-12.7));
#11631=CARTESIAN_POINT('Origin',(-24.2765469720169,163.404687367871,-12.7));
#11632=CARTESIAN_POINT('Origin',(-35.,12.65,12.7));
#11633=CARTESIAN_POINT('',(-35.,12.65,7.7));
#11634=CARTESIAN_POINT('',(-35.,12.65,-7.7));
#11635=CARTESIAN_POINT('',(-35.,12.65,12.7));
#11636=CARTESIAN_POINT('',(-17.9697662756086,12.65,7.7));
#11637=CARTESIAN_POINT('',(-35.,12.65,7.7));
#11638=CARTESIAN_POINT('',(-17.9697662756086,12.65,-7.7));
#11639=CARTESIAN_POINT('Origin',(0.,12.65,0.));
#11640=CARTESIAN_POINT('',(-35.,12.65,-7.7));
#11641=CARTESIAN_POINT('Origin',(-35.,9.65,12.7));
#11642=CARTESIAN_POINT('',(-37.2370215606994,11.6489333498058,7.7));
#11643=CARTESIAN_POINT('',(-37.2370215606994,11.6489333498058,-7.7));
#11644=CARTESIAN_POINT('',(-37.2370215606994,11.6489333498058,12.7));
#11645=CARTESIAN_POINT('Origin',(-35.,9.65,7.7));
#11646=CARTESIAN_POINT('Origin',(-35.,9.65,-7.7));
#11647=CARTESIAN_POINT('Origin',(-51.7283692678324,-4.56844441699029,12.7));
#11648=CARTESIAN_POINT('',(-51.7283692678324,-4.56844441699029,7.7));
#11649=CARTESIAN_POINT('',(-51.7283692678324,-4.56844441699029,-7.7));
#11650=CARTESIAN_POINT('',(-51.7283692678324,-4.56844441699029,12.7));
#11651=CARTESIAN_POINT('',(-51.7283692678324,-4.56844441699029,7.7));
#11652=CARTESIAN_POINT('',(-51.7283692678324,-4.56844441699029,-7.7));
#11653=CARTESIAN_POINT('Origin',(-48.,-7.90000000000001,12.7));
#11654=CARTESIAN_POINT('',(-53.,-7.90000000000001,7.7));
#11655=CARTESIAN_POINT('',(-53.,-7.90000000000001,-7.7));
#11656=CARTESIAN_POINT('',(-53.,-7.90000000000001,12.7));
#11657=CARTESIAN_POINT('Origin',(-48.,-7.90000000000001,7.7));
#11658=CARTESIAN_POINT('Origin',(-48.,-7.90000000000001,-7.7));
#11659=CARTESIAN_POINT('Origin',(-53.,-22.9,12.7));
#11660=CARTESIAN_POINT('',(-53.,-21.9,-7.7));
#11661=CARTESIAN_POINT('',(-53.,-22.9,-7.7));
#11662=CARTESIAN_POINT('',(-53.,-21.9,7.7));
#11663=CARTESIAN_POINT('',(-53.,-21.9,12.7));
#11664=CARTESIAN_POINT('',(-53.,-22.9,7.7));
#11665=CARTESIAN_POINT('Origin',(4.35361937096884E-15,-22.9,12.7));
#11666=CARTESIAN_POINT('',(-16.8005208252602,-22.9,11.7));
#11667=CARTESIAN_POINT('Origin',(-16.8005208252602,-22.9,19.05));
#11668=CARTESIAN_POINT('',(-48.,-22.9,11.7));
#11669=CARTESIAN_POINT('',(4.35361937096884E-15,-22.9,11.7));
#11670=CARTESIAN_POINT('',(-52.,-22.9,7.7));
#11671=CARTESIAN_POINT('Origin',(-48.,-22.9,7.7));
#11672=CARTESIAN_POINT('',(-52.,-22.9,-7.7));
#11673=CARTESIAN_POINT('',(-52.,-22.9,12.7));
#11674=CARTESIAN_POINT('',(-48.,-22.9,-11.7));
#11675=CARTESIAN_POINT('Origin',(-48.,-22.9,-7.7));
#11676=CARTESIAN_POINT('',(-16.8005208252602,-22.9,-11.7));
#11677=CARTESIAN_POINT('',(-16.8005208252602,-22.9,-11.7));
#11678=CARTESIAN_POINT('Origin',(-16.8005208252602,-22.9,-19.05));
#11679=CARTESIAN_POINT('Origin',(34.998522628062,-7.90000000000001,35.2192193816534));
#11680=CARTESIAN_POINT('',(34.998522628062,-7.9,35.2192193816534));
#11681=CARTESIAN_POINT('',(34.998522628062,-21.9,35.2192193816534));
#11682=CARTESIAN_POINT('',(34.998522628062,-7.90000000000001,35.2192193816534));
#11683=CARTESIAN_POINT('',(19.3987830406924,-21.9,8.19967783148497));
#11684=CARTESIAN_POINT('',(34.998522628062,-21.9,35.2192193816534));
#11685=CARTESIAN_POINT('',(19.3987830406924,7.75488674445212,8.19967783148497));
#11686=CARTESIAN_POINT('',(19.3987830406924,12.65,8.19967783148497));
#11687=CARTESIAN_POINT('',(19.9834057658666,7.65,9.21227409474611));
#11688=CARTESIAN_POINT('Origin',(23.1367961164486,163.404687557813,14.6741063980318));
#11689=CARTESIAN_POINT('',(28.0510228507774,7.65,23.1857967818227));
#11690=CARTESIAN_POINT('',(34.998522628062,7.65,35.2192193816534));
#11691=CARTESIAN_POINT('',(34.998522628062,-7.9,35.2192193816534));
#11692=CARTESIAN_POINT('Origin',(28.4985226280621,12.65,23.9608891324556));
#11693=CARTESIAN_POINT('',(24.1683956091399,12.65,26.4608891324556));
#11694=CARTESIAN_POINT('',(10.8316043908595,12.65,34.1608891324555));
#11695=CARTESIAN_POINT('',(28.4985226280621,12.65,23.9608891324556));
#11696=CARTESIAN_POINT('',(15.6532787469444,12.65,11.7122740947461));
#11697=CARTESIAN_POINT('',(24.1683956091399,12.65,26.4608891324556));
#11698=CARTESIAN_POINT('',(2.31648752866395,12.65,19.4122740947459));
#11699=CARTESIAN_POINT('Origin',(0.,12.65,0.));
#11700=CARTESIAN_POINT('',(10.8316043908595,12.65,34.1608891324555));
#11701=CARTESIAN_POINT('Origin',(28.4985226280621,9.65,23.9608891324556));
#11702=CARTESIAN_POINT('Origin',(10.8316043908595,9.65,34.1608891324555));
#11703=CARTESIAN_POINT('',(25.2869063894896,11.6489333498058,28.3982066328348));
#11704=CARTESIAN_POINT('',(29.6170334084118,11.6489333498058,25.8982066328348));
#11705=CARTESIAN_POINT('Origin',(24.1683956091399,9.65,26.4608891324556));
#11706=CARTESIAN_POINT('Origin',(36.8627072619782,-4.56844441699029,38.4480818822854));
#11707=CARTESIAN_POINT('',(32.532580243056,-4.56844441699029,40.9480818822854));
#11708=CARTESIAN_POINT('',(36.8627072619782,-4.56844441699029,38.4480818822854));
#11709=CARTESIAN_POINT('',(32.532580243056,-4.56844441699029,40.9480818822854));
#11710=CARTESIAN_POINT('Origin',(34.998522628062,-7.90000000000001,35.2192193816534));
#11711=CARTESIAN_POINT('Origin',(17.3316043908594,-7.90000000000001,45.4192193816532));
#11712=CARTESIAN_POINT('',(33.1683956091398,-7.90000000000001,42.0493464005755));
#11713=CARTESIAN_POINT('',(37.498522628062,-7.90000000000001,39.5493464005756));
#11714=CARTESIAN_POINT('Origin',(30.6683956091398,-7.90000000000001,37.7192193816533));
#11715=CARTESIAN_POINT('Origin',(37.498522628062,-22.9,39.5493464005756));
#11716=CARTESIAN_POINT('',(33.1683956091398,-21.9,42.0493464005755));
#11717=CARTESIAN_POINT('',(37.498522628062,-21.9,39.5493464005756));
#11718=CARTESIAN_POINT('',(33.1683956091398,-22.9,42.0493464005755));
#11719=CARTESIAN_POINT('Origin',(10.9985226280624,-22.9,-6.3499999999999));
#11720=CARTESIAN_POINT('',(18.5327576369079,-22.9,8.69967783148497));
#11721=CARTESIAN_POINT('Origin',(24.8980443547236,-22.9,5.02467783148503));
#11722=CARTESIAN_POINT('',(34.1324972242776,-22.9,35.7192193816534));
#11723=CARTESIAN_POINT('',(10.132497224278,-22.9,-5.84999999999991));
#11724=CARTESIAN_POINT('',(32.6683956091398,-22.9,41.1833209967911));
#11725=CARTESIAN_POINT('Origin',(30.6683956091398,-22.9,37.7192193816533));
#11726=CARTESIAN_POINT('',(36.998522628062,-22.9,38.6833209967911));
#11727=CARTESIAN_POINT('',(-1.73223681164803,-22.9,20.3996778314848));
#11728=CARTESIAN_POINT('',(-1.73223681164803,-22.9,20.3996778314848));
#11729=CARTESIAN_POINT('Origin',(-8.09752352946369,-22.9,24.0746778314847));
#11730=CARTESIAN_POINT('Origin',(13.0014773719372,-7.90000000000001,47.9192193816532));
#11731=CARTESIAN_POINT('',(-2.59826221543248,7.75488674445211,20.8996778314848));
#11732=CARTESIAN_POINT('',(-2.59826221543248,-21.9,20.8996778314848));
#11733=CARTESIAN_POINT('',(-2.59826221543248,-7.90000000000001,20.8996778314848));
#11734=CARTESIAN_POINT('',(13.0014773719372,-21.9,47.9192193816532));
#11735=CARTESIAN_POINT('',(-2.01363949025827,7.65,21.9122740947459));
#11736=CARTESIAN_POINT('',(-2.59826221543248,7.65,20.8996778314848));
#11737=CARTESIAN_POINT('Origin',(1.13975086201663,163.404687845728,27.3741064009758));
#11738=CARTESIAN_POINT('Origin',(13.0014773719379,-7.90000000000001,-47.919219381653));
#11739=CARTESIAN_POINT('',(-2.5982622154322,-21.9,-20.8996778314848));
#11740=CARTESIAN_POINT('',(13.0014773719379,-21.9,-47.919219381653));
#11741=CARTESIAN_POINT('',(-2.5982622154322,7.75488674445212,-20.8996778314848));
#11742=CARTESIAN_POINT('',(-2.5982622154322,12.65,-20.8996778314848));
#11743=CARTESIAN_POINT('',(-2.01363949025797,7.65,-21.9122740947459));
#11744=CARTESIAN_POINT('Origin',(1.13975086881472,163.404688086806,-27.3741064127498));
#11745=CARTESIAN_POINT('',(13.0014773719379,7.65,-47.919219381653));
#11746=CARTESIAN_POINT('Origin',(6.5014773719378,12.65,-36.6608891324553));
#11747=CARTESIAN_POINT('',(10.83160439086,12.65,-34.1608891324553));
#11748=CARTESIAN_POINT('',(24.1683956091403,12.65,-26.4608891324553));
#11749=CARTESIAN_POINT('',(6.5014773719378,12.65,-36.6608891324553));
#11750=CARTESIAN_POINT('',(10.83160439086,12.65,-34.1608891324553));
#11751=CARTESIAN_POINT('',(24.1683956091403,12.65,-26.4608891324553));
#11752=CARTESIAN_POINT('Origin',(6.5014773719378,9.65,-36.6608891324553));
#11753=CARTESIAN_POINT('',(25.28690638949,11.6489333498058,-28.3982066328344));
#11754=CARTESIAN_POINT('Origin',(24.1683956091403,9.65,-26.4608891324553));
#11755=CARTESIAN_POINT('',(7.61998815228752,11.6489333498058,-38.5982066328345));
#11756=CARTESIAN_POINT('Origin',(10.83160439086,9.65,-34.1608891324553));
#11757=CARTESIAN_POINT('Origin',(14.8656620058541,-4.56844441699029,-51.148081882285));
#11758=CARTESIAN_POINT('',(32.5325802430566,-4.56844441699029,-40.9480818822849));
#11759=CARTESIAN_POINT('',(32.5325802430566,-4.56844441699029,-40.9480818822849));
#11760=CARTESIAN_POINT('',(14.865662005854,-4.56844441699029,-51.148081882285));
#11761=CARTESIAN_POINT('Origin',(13.0014773719379,-7.90000000000001,-47.919219381653));
#11762=CARTESIAN_POINT('',(33.1683956091404,-7.90000000000001,-42.0493464005751));
#11763=CARTESIAN_POINT('Origin',(30.6683956091404,-7.90000000000001,-37.7192193816529));
#11764=CARTESIAN_POINT('',(15.5014773719379,-7.90000000000001,-52.2493464005752));
#11765=CARTESIAN_POINT('Origin',(17.33160439086,-7.90000000000001,-45.419219381653));
#11766=CARTESIAN_POINT('Origin',(15.5014773719379,-22.9,-52.2493464005752));
#11767=CARTESIAN_POINT('',(33.1683956091404,-21.9,-42.0493464005751));
#11768=CARTESIAN_POINT('',(33.1683956091404,-22.9,-42.0493464005751));
#11769=CARTESIAN_POINT('',(15.5014773719379,-21.9,-52.2493464005752));
#11770=CARTESIAN_POINT('Origin',(-10.9985226280623,-22.9,-6.35000000000005));
#11771=CARTESIAN_POINT('',(18.0131895824795,-22.9,-7.59786161137808));
#11772=CARTESIAN_POINT('',(-2.42665362134758,-22.9,-19.3988105873015));
#11773=CARTESIAN_POINT('Origin',(4.9095947433306E-17,-22.9,-8.50366754002159E-17));
#11774=CARTESIAN_POINT('',(-1.73223681164776,-22.9,-20.3996778314848));
#11775=CARTESIAN_POINT('Origin',(-8.09752352946338,-22.9,-24.0746778314848));
#11776=CARTESIAN_POINT('',(13.8675027757223,-22.9,-47.419219381653));
#11777=CARTESIAN_POINT('',(-10.1324972242779,-22.9,-5.85000000000004));
#11778=CARTESIAN_POINT('',(19.3316043908601,-22.9,-48.8833209967907));
#11779=CARTESIAN_POINT('Origin',(17.33160439086,-22.9,-45.419219381653));
#11780=CARTESIAN_POINT('',(32.6683956091404,-22.9,-41.1833209967907));
#11781=CARTESIAN_POINT('',(15.0014773719379,-22.9,-51.3833209967907));
#11782=CARTESIAN_POINT('',(34.1324972242781,-22.9,-35.7192193816529));
#11783=CARTESIAN_POINT('Origin',(30.6683956091404,-22.9,-37.7192193816529));
#11784=CARTESIAN_POINT('',(18.532757636908,-22.9,-8.6996778314847));
#11785=CARTESIAN_POINT('',(18.532757636908,-22.9,-8.6996778314847));
#11786=CARTESIAN_POINT('Origin',(24.8980443547237,-22.9,-5.02467783148466));
#11787=CARTESIAN_POINT('Origin',(34.9985226280625,-7.90000000000001,-35.2192193816529));
#11788=CARTESIAN_POINT('',(19.3987830406925,7.75488674445212,-8.19967783148469));
#11789=CARTESIAN_POINT('',(19.3987830406925,-21.9,-8.19967783148469));
#11790=CARTESIAN_POINT('',(19.3987830406925,-7.90000000000001,-8.19967783148469));
#11791=CARTESIAN_POINT('',(34.9985226280625,-21.9,-35.2192193816529));
#11792=CARTESIAN_POINT('',(34.9985226280625,-21.9,-35.2192193816529));
#11793=CARTESIAN_POINT('',(34.9985226280625,-7.90000000000001,-35.2192193816529));
#11794=CARTESIAN_POINT('',(34.9985226280625,-7.90000000000001,-35.2192193816529));
#11795=CARTESIAN_POINT('',(28.0510228507777,7.65,-23.1857967818223));
#11796=CARTESIAN_POINT('',(27.752848774496,8.31737776679612,-22.6693441322024));
#11797=CARTESIAN_POINT('',(19.9834057658667,7.65,-9.21227409474582));
#11798=CARTESIAN_POINT('',(19.3987830406925,7.65,-8.19967783148468));
#11799=CARTESIAN_POINT('Origin',(23.136796101799,163.404686601979,-14.6741063726841));
#11800=CARTESIAN_POINT('Origin',(-16.8005208252602,25.4,-19.05));
#11801=CARTESIAN_POINT('',(-15.7517039698567,-21.9,-12.7872144213759));
#11802=CARTESIAN_POINT('Ctrl Pts',(-12.6003906189451,-23.4,-14.2875));
#11803=CARTESIAN_POINT('Ctrl Pts',(-12.7170023297541,-23.3035563482058,
-14.1846581377472));
#11804=CARTESIAN_POINT('Ctrl Pts',(-12.8375066038114,-23.2068396386061,
-14.0859034998214));
#11805=CARTESIAN_POINT('Ctrl Pts',(-12.9620390251358,-23.1112816986106,
-13.9913525639123));
#11806=CARTESIAN_POINT('Ctrl Pts',(-13.0797099390072,-23.0209888254186,
-13.902011210733));
#11807=CARTESIAN_POINT('Ctrl Pts',(-13.2009776026165,-22.931728890007,-13.8164231666886));
#11808=CARTESIAN_POINT('Ctrl Pts',(-13.3259828864208,-22.8447237861406,
-13.7347186102794));
#11809=CARTESIAN_POINT('Ctrl Pts',(-13.4398977695664,-22.7654377276767,
-13.6602628375907));
#11810=CARTESIAN_POINT('Ctrl Pts',(-13.5569167566412,-22.6880233923778,
-13.5890322851068));
#11811=CARTESIAN_POINT('Ctrl Pts',(-13.6771653733519,-22.613433061264,-13.5211502011406));
#11812=CARTESIAN_POINT('Ctrl Pts',(-13.780395816837,-22.5493991191596,-13.46287512219));
#11813=CARTESIAN_POINT('Ctrl Pts',(-13.8860066956812,-22.4874464632126,
-13.4070681378658));
#11814=CARTESIAN_POINT('Ctrl Pts',(-13.994088488402,-22.428202217372,-13.3538221960299));
#11815=CARTESIAN_POINT('Ctrl Pts',(-13.9996382379135,-22.4251601626824,
-13.3510881403462));
#11816=CARTESIAN_POINT('Ctrl Pts',(-14.0051944007122,-22.4221253454026,
-13.3483608913321));
#11817=CARTESIAN_POINT('Ctrl Pts',(-14.0107569982363,-22.4190978469187,
-13.345640457389));
#11818=CARTESIAN_POINT('Ctrl Pts',(-14.1078577207225,-22.3662498224408,
-13.2981525526451));
#11819=CARTESIAN_POINT('Ctrl Pts',(-14.2071599870361,-22.3154805383895,
-13.2526249539681));
#11820=CARTESIAN_POINT('Ctrl Pts',(-14.3089608526168,-22.2675991945199,
-13.2091881241018));
#11821=CARTESIAN_POINT('Ctrl Pts',(-14.4029294513603,-22.2234017040201,
-13.1690931994357));
#11822=CARTESIAN_POINT('Ctrl Pts',(-14.4990269678438,-22.1816645410303,
-13.1307798082167));
#11823=CARTESIAN_POINT('Ctrl Pts',(-14.5975040224041,-22.1430604940455,
-13.0943671154366));
#11824=CARTESIAN_POINT('Ctrl Pts',(-14.6716472726562,-22.1139955557294,
-13.0669520449392));
#11825=CARTESIAN_POINT('Ctrl Pts',(-14.7471396830704,-22.0867072848311,
-13.0406147104802));
#11826=CARTESIAN_POINT('Ctrl Pts',(-14.8240955566372,-22.0614998943554,
-13.0154125395925));
#11827=CARTESIAN_POINT('Ctrl Pts',(-14.8293099770775,-22.0597918774614,
-13.0137048763704));
#11828=CARTESIAN_POINT('Ctrl Pts',(-14.8345302483747,-22.0580937292925,
-13.0120027124143));
#11829=CARTESIAN_POINT('Ctrl Pts',(-14.8397564046443,-22.056405537151,-13.0103060600109));
#11830=CARTESIAN_POINT('Ctrl Pts',(-14.9357824134385,-22.0253864965673,
-12.9791315695807));
#11831=CARTESIAN_POINT('Ctrl Pts',(-15.032901952619,-21.9978800256288,-12.9500987220667));
#11832=CARTESIAN_POINT('Ctrl Pts',(-15.1313475446627,-21.9749039650076,
-12.9232625229759));
#11833=CARTESIAN_POINT('Ctrl Pts',(-15.2241318069018,-21.9532491931723,
-12.8979695984045));
#11834=CARTESIAN_POINT('Ctrl Pts',(-15.3180939370895,-21.9356181609241,
-12.8746280167693));
#11835=CARTESIAN_POINT('Ctrl Pts',(-15.4134375927924,-21.9229055030944,
-12.8532981171489));
#11836=CARTESIAN_POINT('Ctrl Pts',(-15.5029064118453,-21.9109761673178,
-12.8332825123823));
#11837=CARTESIAN_POINT('Ctrl Pts',(-15.5935917299168,-21.9033774739699,
-12.8150383915244));
#11838=CARTESIAN_POINT('Ctrl Pts',(-15.6856704705524,-21.9008931019107,
-12.7986275193415));
#11839=CARTESIAN_POINT('Ctrl Pts',(-15.7076017238433,-21.9003013758236,
-12.7947187887042));
#11840=CARTESIAN_POINT('Ctrl Pts',(-15.7296120665973,-21.9000000019656,
-12.7909141106301));
#11841=CARTESIAN_POINT('Ctrl Pts',(-15.7517039698567,-21.9,-12.7872144213759));
#11842=CARTESIAN_POINT('Origin',(-16.8005208252602,-21.9,-19.05));
#11843=CARTESIAN_POINT('Ctrl Pts',(-16.8005208252602,7.75488674445212,-12.7));
#11844=CARTESIAN_POINT('Ctrl Pts',(-16.7349414235869,7.77600035063442,-12.7));
#11845=CARTESIAN_POINT('Ctrl Pts',(-16.6708099716639,7.79969631458978,-12.7010053967542));
#11846=CARTESIAN_POINT('Ctrl Pts',(-16.6079679401019,7.8256484538807,-12.7029063991874));
#11847=CARTESIAN_POINT('Ctrl Pts',(-16.5435673523868,7.85224423669134,-12.7048545487126));
#11848=CARTESIAN_POINT('Ctrl Pts',(-16.4805209961261,7.88120973563962,-12.7077433417563));
#11849=CARTESIAN_POINT('Ctrl Pts',(-16.4186711504242,7.91224591462863,-12.711471286032));
#11850=CARTESIAN_POINT('Ctrl Pts',(-16.3543372897761,7.94452856936239,-12.7153489520926));
#11851=CARTESIAN_POINT('Ctrl Pts',(-16.2912980137447,7.97905171373885,-12.7201345556429));
#11852=CARTESIAN_POINT('Ctrl Pts',(-16.2293889115104,8.01553158395874,-12.7257310395034));
#11853=CARTESIAN_POINT('Ctrl Pts',(-16.1958378593221,8.0353015044615,-12.7287640009792));
#11854=CARTESIAN_POINT('Ctrl Pts',(-16.1626189581162,8.05564699923813,-12.7320354070764));
#11855=CARTESIAN_POINT('Ctrl Pts',(-16.1297074857929,8.07652873453458,-12.7355317354578));
#11856=CARTESIAN_POINT('Ctrl Pts',(-16.0866738196167,8.10383281917404,-12.7401033883735));
#11857=CARTESIAN_POINT('Ctrl Pts',(-16.0441679035951,8.13206076164089,-12.7450610080348));
#11858=CARTESIAN_POINT('Ctrl Pts',(-16.002143104575,8.16115913750229,-12.7503845705938));
#11859=CARTESIAN_POINT('Ctrl Pts',(-15.9276085615548,8.21276757342653,-12.7598263600091));
#11860=CARTESIAN_POINT('Ctrl Pts',(-15.8548776335165,8.26690043733163,-12.7703819477842));
#11861=CARTESIAN_POINT('Ctrl Pts',(-15.7838082658192,8.32314897453989,-12.7819107053312));
#11862=CARTESIAN_POINT('Ctrl Pts',(-15.7107906519688,8.38093946997536,-12.7937555042089));
#11863=CARTESIAN_POINT('Ctrl Pts',(-15.6395269896275,8.44096333239077,-12.8066275852114));
#11864=CARTESIAN_POINT('Ctrl Pts',(-15.5698762835546,8.50282830727392,-12.8203902527625));
#11865=CARTESIAN_POINT('Ctrl Pts',(-15.5466981609681,8.52341552099364,-12.8249701459697));
#11866=CARTESIAN_POINT('Ctrl Pts',(-15.5236987594059,8.5442070222161,-12.8296487881716));
#11867=CARTESIAN_POINT('Ctrl Pts',(-15.5008731781905,8.56518952756248,-12.8344215077166));
#11868=CARTESIAN_POINT('Ctrl Pts',(-15.4385988825786,8.62243541884092,-12.8474427642187));
#11869=CARTESIAN_POINT('Ctrl Pts',(-15.3777011585566,8.68106595956029,-12.8611612425515));
#11870=CARTESIAN_POINT('Ctrl Pts',(-15.3182018865546,8.74069382312877,-12.8754501442092));
#11871=CARTESIAN_POINT('Ctrl Pts',(-15.2564420923887,8.80258709436762,-12.8902819160199));
#11872=CARTESIAN_POINT('Ctrl Pts',(-15.1960523906305,8.86568736323019,-12.9057609205674));
#11873=CARTESIAN_POINT('Ctrl Pts',(-15.1370245917722,8.92967013781512,-12.9217807326603));
#11874=CARTESIAN_POINT('Ctrl Pts',(-15.0751539679737,8.99673437284488,-12.9385720714277));
#11875=CARTESIAN_POINT('Ctrl Pts',(-15.0147794430409,9.06476837724042,-12.955957604799));
#11876=CARTESIAN_POINT('Ctrl Pts',(-14.9558876408858,9.13345255195956,-12.973832558441));
#11877=CARTESIAN_POINT('Ctrl Pts',(-14.941745213388,9.14994654476789,-12.9781250953759));
#11878=CARTESIAN_POINT('Ctrl Pts',(-14.9276882808297,9.16647825760667,-12.9824459317766));
#11879=CARTESIAN_POINT('Ctrl Pts',(-14.9137166409377,9.18304367617656,-12.9867937549488));
#11880=CARTESIAN_POINT('Ctrl Pts',(-14.8443822685258,9.26524969559609,-13.0083698614999));
#11881=CARTESIAN_POINT('Ctrl Pts',(-14.7769243288711,9.34848879466141,-13.0306551587621));
#11882=CARTESIAN_POINT('Ctrl Pts',(-14.7110830067531,9.43264075175323,-13.0535945525926));
#11883=CARTESIAN_POINT('Ctrl Pts',(-14.6419151645199,9.52104434245437,-13.0776929200364));
#11884=CARTESIAN_POINT('Ctrl Pts',(-14.574531492047,9.61045552746631,-13.1025131517201));
#11885=CARTESIAN_POINT('Ctrl Pts',(-14.508658780167,9.7007827075362,-13.1280111392882));
#11886=CARTESIAN_POINT('Ctrl Pts',(-14.464101115013,9.76188188091148,-13.1452585056063));
#11887=CARTESIAN_POINT('Ctrl Pts',(-14.4202353698703,9.82340116495587,-13.1628163911151));
#11888=CARTESIAN_POINT('Ctrl Pts',(-14.376983382446,9.88532296597228,-13.180675825673));
#11889=CARTESIAN_POINT('Ctrl Pts',(-14.3247407934093,9.96011618116435,-13.2022476228458));
#11890=CARTESIAN_POINT('Ctrl Pts',(-14.2733952776958,10.0354996811099,-13.2242602480238));
#11891=CARTESIAN_POINT('Ctrl Pts',(-14.2228316908371,10.111478019192,-13.2467171132975));
#11892=CARTESIAN_POINT('Ctrl Pts',(-14.1455756462056,10.2275652321953,-13.2810289312213));
#11893=CARTESIAN_POINT('Ctrl Pts',(-14.070305718922,10.3447938290241,-13.3163058267544));
#11894=CARTESIAN_POINT('Ctrl Pts',(-13.9967407810488,10.4630236267724,-13.3525118459524));
#11895=CARTESIAN_POINT('Ctrl Pts',(-13.9578439948862,10.5255365479276,-13.3716554465217));
#11896=CARTESIAN_POINT('Ctrl Pts',(-13.9194243133811,10.5883301347506,-13.3910591092213));
#11897=CARTESIAN_POINT('Ctrl Pts',(-13.8814429470248,10.6513883422587,-13.4107195192154));
#11898=CARTESIAN_POINT('Ctrl Pts',(-13.8087592766334,10.7720607247897,-13.4483429882175));
#11899=CARTESIAN_POINT('Ctrl Pts',(-13.7376959033737,10.8936995222114,-13.4869103870559));
#11900=CARTESIAN_POINT('Ctrl Pts',(-13.6681560963966,11.015983366519,-13.526345490624));
#11901=CARTESIAN_POINT('Ctrl Pts',(-13.592500863716,11.1490210192869,-13.5692485711174));
#11902=CARTESIAN_POINT('Ctrl Pts',(-13.5186486051634,11.282822820578,-13.6131786525212));
#11903=CARTESIAN_POINT('Ctrl Pts',(-13.4464916370684,11.4170275975458,-13.6580628050807));
#11904=CARTESIAN_POINT('Ctrl Pts',(-13.4381590557207,11.4325253692907,-13.6632459615006));
#11905=CARTESIAN_POINT('Ctrl Pts',(-13.4298491021049,11.448028560653,-13.6684418663174));
#11906=CARTESIAN_POINT('Ctrl Pts',(-13.4215616267315,11.4635366486352,-13.6736504266539));
#11907=CARTESIAN_POINT('Ctrl Pts',(-13.3957800509804,11.5117808879307,-13.6898537801265));
#11908=CARTESIAN_POINT('Ctrl Pts',(-13.3701991365705,11.560096143354,-13.706184919204));
#11909=CARTESIAN_POINT('Ctrl Pts',(-13.3448076869915,11.6084844905147,-13.7226484987598));
#11910=CARTESIAN_POINT('Ctrl Pts',(-13.2498225662632,11.7894971177225,-13.7842359668902));
#11911=CARTESIAN_POINT('Ctrl Pts',(-13.1575527637327,11.9714205682347,-13.8476343858048));
#11912=CARTESIAN_POINT('Ctrl Pts',(-13.0676927983035,12.1538289736455,-13.912913228778));
#11913=CARTESIAN_POINT('Ctrl Pts',(-13.0310870527492,12.2281356534171,-13.9395055015942));
#11914=CARTESIAN_POINT('Ctrl Pts',(-12.9948815747046,12.3025233034365,-13.9664097879093));
#11915=CARTESIAN_POINT('Ctrl Pts',(-12.9590571742035,12.3769650887378,-13.9936305724574));
#11916=CARTESIAN_POINT('Ctrl Pts',(-12.8917900984241,12.5167435956483,-14.0447427348763));
#11917=CARTESIAN_POINT('Ctrl Pts',(-12.8256706149678,12.6571275035442,-14.0971253811225));
#11918=CARTESIAN_POINT('Ctrl Pts',(-12.7608591759401,12.7973698710114,-14.1505956618139));
#11919=CARTESIAN_POINT('Ctrl Pts',(-12.7064224840691,12.915162820213,-14.1955066410781));
#11920=CARTESIAN_POINT('Ctrl Pts',(-12.6529076763499,13.0328551936126,-14.2411843088393));
#11921=CARTESIAN_POINT('Ctrl Pts',(-12.6003906189451,13.15,-14.2875));
#11922=CARTESIAN_POINT('Origin',(-8.09752352946338,25.4,-24.0746778314848));
#11923=CARTESIAN_POINT('',(-3.19820054762184,-21.9,-20.0349830014761));
#11924=CARTESIAN_POINT('Origin',(-8.09752352946338,-21.9,-24.0746778314848));
#11925=CARTESIAN_POINT('Ctrl Pts',(-3.19820054762184,-21.9,-20.0349830014761));
#11926=CARTESIAN_POINT('Ctrl Pts',(-3.25878664769386,-21.9000000083571,
-19.961504462885));
#11927=CARTESIAN_POINT('Ctrl Pts',(-3.32027867353187,-21.9054435048663,
-19.8902504786465));
#11928=CARTESIAN_POINT('Ctrl Pts',(-3.38271157237758,-21.9155046710484,
-19.8210264481285));
#11929=CARTESIAN_POINT('Ctrl Pts',(-3.44795761695358,-21.926019180375,-19.7486832722642));
#11930=CARTESIAN_POINT('Ctrl Pts',(-3.51423117414105,-21.9415773497121,
-19.6785571332404));
#11931=CARTESIAN_POINT('Ctrl Pts',(-3.5815792215889,-21.9612924550953,-19.6104423872282));
#11932=CARTESIAN_POINT('Ctrl Pts',(-3.65454948264978,-21.9826533770696,
-19.5366414236227));
#11933=CARTESIAN_POINT('Ctrl Pts',(-3.72878097791152,-22.0088947211577,
-19.4652016366644));
#11934=CARTESIAN_POINT('Ctrl Pts',(-3.80434326748668,-22.0389456239223,
-19.3958807427751));
#11935=CARTESIAN_POINT('Ctrl Pts',(-3.81864012116223,-22.0446314410417,
-19.3827647998601));
#11936=CARTESIAN_POINT('Ctrl Pts',(-3.83298464569427,-22.0504537744497,
-19.3697247637157));
#11937=CARTESIAN_POINT('Ctrl Pts',(-3.84737735413469,-22.056405549946,-19.3567590646729));
#11938=CARTESIAN_POINT('Ctrl Pts',(-3.85146313648624,-22.0580951318189,
-19.3530783797939));
#11939=CARTESIAN_POINT('Ctrl Pts',(-3.85555075261669,-22.0597946861621,
-19.3494055600629));
#11940=CARTESIAN_POINT('Ctrl Pts',(-3.85964020896223,-22.0615041254605,
-19.3457405697024));
#11941=CARTESIAN_POINT('Ctrl Pts',(-3.93897962430439,-22.0946689041092,
-19.2746362057315));
#11942=CARTESIAN_POINT('Ctrl Pts',(-4.01875388994255,-22.1314339084887,
-19.2067072527322));
#11943=CARTESIAN_POINT('Ctrl Pts',(-4.09898053060866,-22.1711120177018,
-19.1416659844961));
#11944=CARTESIAN_POINT('Ctrl Pts',(-4.18540780668146,-22.2138568075937,
-19.0715977428336));
#11945=CARTESIAN_POINT('Ctrl Pts',(-4.2723599814154,-22.2599827034751,-19.0048807754165));
#11946=CARTESIAN_POINT('Ctrl Pts',(-4.35986578198443,-22.3086850460383,
-18.9411866314663));
#11947=CARTESIAN_POINT('Ctrl Pts',(-4.42370622049564,-22.3442161638104,
-18.8947181453324));
#11948=CARTESIAN_POINT('Ctrl Pts',(-4.48784147647386,-22.3811198321359,
-18.8498592500996));
#11949=CARTESIAN_POINT('Ctrl Pts',(-4.55228515966479,-22.4190978671498,
-18.806491720188));
#11950=CARTESIAN_POINT('Ctrl Pts',(-4.55742937494407,-22.4221294627744,
-18.803029908278));
#11951=CARTESIAN_POINT('Ctrl Pts',(-4.56257628221482,-22.4251683970662,
-18.7995771008193));
#11952=CARTESIAN_POINT('Ctrl Pts',(-4.56772588494067,-22.4282145883129,
-18.7961332749495));
#11953=CARTESIAN_POINT('Ctrl Pts',(-4.71481038542885,-22.5152208180672,
-18.6977696856022));
#11954=CARTESIAN_POINT('Ctrl Pts',(-4.86420124525512,-22.6081793599833,
-18.6066604878163));
#11955=CARTESIAN_POINT('Ctrl Pts',(-5.01562596722791,-22.7050300051394,
-18.5225574277292));
#11956=CARTESIAN_POINT('Ctrl Pts',(-5.16862236887894,-22.8028858903173,
-18.4375814383826));
#11957=CARTESIAN_POINT('Ctrl Pts',(-5.32369490141207,-22.9047152085253,
-18.359757839249));
#11958=CARTESIAN_POINT('Ctrl Pts',(-5.48057109348493,-23.0084452512491,
-18.288838145327));
#11959=CARTESIAN_POINT('Ctrl Pts',(-5.64018244583602,-23.1139838430508,
-18.2166819557506));
#11960=CARTESIAN_POINT('Ctrl Pts',(-5.80166083081389,-23.221490118629,-18.1516724956205));
#11961=CARTESIAN_POINT('Ctrl Pts',(-5.96472994459809,-23.3288332572481,
-18.093555430662));
#11962=CARTESIAN_POINT('Ctrl Pts',(-6.00079065213521,-23.3525708580606,
-18.0807035641512));
#11963=CARTESIAN_POINT('Ctrl Pts',(-6.03692919164292,-23.3763006768841,
-18.0681887778408));
#11964=CARTESIAN_POINT('Ctrl Pts',(-6.07314264709753,-23.4,-18.0560083736136));
#11965=CARTESIAN_POINT('Ctrl Pts',(-6.07314264709754,13.15,-18.0560083736136));
#11966=CARTESIAN_POINT('Ctrl Pts',(-5.97181996734248,12.9711603486608,-18.0900882806898));
#11967=CARTESIAN_POINT('Ctrl Pts',(-5.87130801630144,12.7922384032894,-18.1267220226218));
#11968=CARTESIAN_POINT('Ctrl Pts',(-5.77140203340685,12.6135684723799,-18.1660441169748));
#11969=CARTESIAN_POINT('Ctrl Pts',(-5.67731388552087,12.4453030452741,-18.2030763639081));
#11970=CARTESIAN_POINT('Ctrl Pts',(-5.58376322164663,12.2772593406106,-18.2424932633217));
#11971=CARTESIAN_POINT('Ctrl Pts',(-5.49059061374234,12.10972986541,-18.2844480350073));
#11972=CARTESIAN_POINT('Ctrl Pts',(-5.40407677968078,11.9541732319324,-18.3234044218395));
#11973=CARTESIAN_POINT('Ctrl Pts',(-5.31788895518178,11.7990589449033,-18.364549187312));
#11974=CARTESIAN_POINT('Ctrl Pts',(-5.23190911158772,11.6446517025337,-18.4080371962308));
#11975=CARTESIAN_POINT('Ctrl Pts',(-5.22529143778171,11.6327673268408,-18.4113843697714));
#11976=CARTESIAN_POINT('Ctrl Pts',(-5.21867500086194,11.6208871598949,-18.4147454404937));
#11977=CARTESIAN_POINT('Ctrl Pts',(-5.21205974944158,11.6090113330872,-18.4181204869383));
#11978=CARTESIAN_POINT('Ctrl Pts',(-5.1848316235959,11.5601308769573,-18.4320120510659));
#11979=CARTESIAN_POINT('Ctrl Pts',(-5.1576259896201,11.511329719366,-18.4461391252805));
#11980=CARTESIAN_POINT('Ctrl Pts',(-5.13043998234374,11.4626185033488,-18.4605069020915));
#11981=CARTESIAN_POINT('Ctrl Pts',(-5.04825349547858,11.3153587871761,-18.503942375648));
#11982=CARTESIAN_POINT('Ctrl Pts',(-4.96623254825319,11.1688712789634,-18.5495431771531));
#11983=CARTESIAN_POINT('Ctrl Pts',(-4.88422351176766,11.023341194086,-18.5976181451075));
#11984=CARTESIAN_POINT('Ctrl Pts',(-4.80536483798301,10.8834016218021,-18.6438463216304));
#11985=CARTESIAN_POINT('Ctrl Pts',(-4.72651736403294,10.7443469551293,-18.6923620873245));
#11986=CARTESIAN_POINT('Ctrl Pts',(-4.6475479022612,10.6063775970585,-18.7434712498276));
#11987=CARTESIAN_POINT('Ctrl Pts',(-4.57238550279757,10.475059644873,-18.7921164754899));
#11988=CARTESIAN_POINT('Ctrl Pts',(-4.49711275367302,10.344724674812,-18.8431110048543));
#11989=CARTESIAN_POINT('Ctrl Pts',(-4.42161551358169,10.2155824305894,-18.8967487338862));
#11990=CARTESIAN_POINT('Ctrl Pts',(-4.40218914607156,10.1823525443801,-18.9105503806129));
#11991=CARTESIAN_POINT('Ctrl Pts',(-4.38274791199463,10.1492018354882,-18.9245271982718));
#11992=CARTESIAN_POINT('Ctrl Pts',(-4.36328985471379,10.116134325549,-18.9386845498513));
#11993=CARTESIAN_POINT('Ctrl Pts',(-4.31906701210315,10.0409809190982,-18.9708603380942));
#11994=CARTESIAN_POINT('Ctrl Pts',(-4.27475033656031,9.96626705526661,-19.0039731983406));
#11995=CARTESIAN_POINT('Ctrl Pts',(-4.23030242157944,9.89202045142478,-19.038101523747));
#11996=CARTESIAN_POINT('Ctrl Pts',(-4.17007877614573,9.7914217811305,-19.0843428866863));
#11997=CARTESIAN_POINT('Ctrl Pts',(-4.10961908431761,9.69169193896628,-19.1324643246693));
#11998=CARTESIAN_POINT('Ctrl Pts',(-4.04884198562672,9.59300570028752,-19.1827615424047));
#11999=CARTESIAN_POINT('Ctrl Pts',(-4.01019530923867,9.53025352533475,-19.2147443178072));
#12000=CARTESIAN_POINT('Ctrl Pts',(-3.97142032686885,9.46792401681482,-19.2476074389096));
#12001=CARTESIAN_POINT('Ctrl Pts',(-3.93249626019989,9.40607058542615,-19.2814341079721));
#12002=CARTESIAN_POINT('Ctrl Pts',(-3.88593531573127,9.3320815490653,-19.3218975485774));
#12003=CARTESIAN_POINT('Ctrl Pts',(-3.83914319459572,9.25875668204225,-19.3637545119824));
#12004=CARTESIAN_POINT('Ctrl Pts',(-3.79206853549414,9.18618721050011,-19.4071777195395));
#12005=CARTESIAN_POINT('Ctrl Pts',(-3.7419706788984,9.10895723055056,-19.4533896234946));
#12006=CARTESIAN_POINT('Ctrl Pts',(-3.69180314879746,9.03297713417334,-19.501153477267));
#12007=CARTESIAN_POINT('Ctrl Pts',(-3.64157577202708,8.95848778471708,-19.5506232829686));
#12008=CARTESIAN_POINT('Ctrl Pts',(-3.591700633242,8.88452081926863,-19.5997461634312));
#12009=CARTESIAN_POINT('Ctrl Pts',(-3.54176640274007,8.81202334048803,-19.6505510647792));
#12010=CARTESIAN_POINT('Ctrl Pts',(-3.49179225292663,8.74127840230459,-19.703205021262));
#12011=CARTESIAN_POINT('Ctrl Pts',(-3.45031120448795,8.68255655874079,-19.7469104435154));
#12012=CARTESIAN_POINT('Ctrl Pts',(-3.40878815829155,8.62503122998402,-19.791904833991));
#12013=CARTESIAN_POINT('Ctrl Pts',(-3.36721112089652,8.56885520307109,-19.8383298148915));
#12014=CARTESIAN_POINT('Ctrl Pts',(-3.32614372687987,8.51336777115995,-19.8841857272487));
#12015=CARTESIAN_POINT('Ctrl Pts',(-3.28499911832725,8.45914957374367,-19.9314552410215));
#12016=CARTESIAN_POINT('Ctrl Pts',(-3.24375684075465,8.40640557245158,-19.9803399318371));
#12017=CARTESIAN_POINT('Ctrl Pts',(-3.20424421247424,8.35587358829024,-20.0271744601533));
#12018=CARTESIAN_POINT('Ctrl Pts',(-3.16464194043481,8.30669462479412,-20.075491474184));
#12019=CARTESIAN_POINT('Ctrl Pts',(-3.12493769096898,8.25909114270198,-20.12548869821));
#12020=CARTESIAN_POINT('Ctrl Pts',(-3.09875754613535,8.22770241044979,-20.1584558134153));
#12021=CARTESIAN_POINT('Ctrl Pts',(-3.07253317739119,8.19699952044321,-20.1921538645661));
#12022=CARTESIAN_POINT('Ctrl Pts',(-3.04626248231991,8.16705743584219,-20.2266449579396));
#12023=CARTESIAN_POINT('Ctrl Pts',(-3.01950180981585,8.13655689834508,-20.2617793482392));
#12024=CARTESIAN_POINT('Ctrl Pts',(-2.99270944889829,8.10686980879576,-20.2977147377636));
#12025=CARTESIAN_POINT('Ctrl Pts',(-2.96586636824719,8.07806532466685,-20.334544841819));
#12026=CARTESIAN_POINT('Ctrl Pts',(-2.93487296250628,8.04480725435189,-20.377069407956));
#12027=CARTESIAN_POINT('Ctrl Pts',(-2.90383026540122,8.01279246823105,-20.4208041851031));
#12028=CARTESIAN_POINT('Ctrl Pts',(-2.87280600557641,7.98223072787833,-20.465746960996));
#12029=CARTESIAN_POINT('Ctrl Pts',(-2.84276929780852,7.9526418168443,-20.5092591360937));
#12030=CARTESIAN_POINT('Ctrl Pts',(-2.81274971365855,7.92441470275159,-20.5539038580238));
#12031=CARTESIAN_POINT('Ctrl Pts',(-2.78282604631469,7.89778233068622,-20.5996722896361));
#12032=CARTESIAN_POINT('Ctrl Pts',(-2.75380560115464,7.87195383566507,-20.6440592374124));
#12033=CARTESIAN_POINT('Ctrl Pts',(-2.72487522323847,7.84762505828801,-20.6895032879898));
#12034=CARTESIAN_POINT('Ctrl Pts',(-2.69612555324366,7.82505223561181,-20.7359867177464));
#12035=CARTESIAN_POINT('Ctrl Pts',(-2.6685106150068,7.80337034833633,-20.7806354751755));
#12036=CARTESIAN_POINT('Ctrl Pts',(-2.64106230558355,7.78330843075126,-20.8262433432298));
#12037=CARTESIAN_POINT('Ctrl Pts',(-2.61388021809145,7.76513667663637,-20.8727829774746));
#12038=CARTESIAN_POINT('Ctrl Pts',(-2.60866408756246,7.76164959193651,-20.881713741422));
#12039=CARTESIAN_POINT('Ctrl Pts',(-2.60345782197805,7.75823224576018,-20.8906787769713));
#12040=CARTESIAN_POINT('Ctrl Pts',(-2.59826221543221,7.75488674445212,-20.8996778314848));
#12041=CARTESIAN_POINT('Origin',(24.8980443547237,25.4,-5.02467783148466));
#12042=CARTESIAN_POINT('',(18.9499045174787,-21.9,-7.24776858010006));
#12043=CARTESIAN_POINT('Ctrl Pts',(18.6735332660427,-23.4,-3.76850837361349));
#12044=CARTESIAN_POINT('Ctrl Pts',(18.6427754562218,-23.3035563483767,-3.92091800839177));
#12045=CARTESIAN_POINT('Ctrl Pts',(18.6175035681029,-23.2068396389513,-4.07465508966213));
#12046=CARTESIAN_POINT('Ctrl Pts',(18.597886266332,-23.1112816991265,-4.22977879778428));
#12047=CARTESIAN_POINT('Ctrl Pts',(18.5793498417064,-23.0209888255381,-4.37635547570033));
#12048=CARTESIAN_POINT('Ctrl Pts',(18.5658622530517,-22.9317288897395,-4.52417037570528));
#12049=CARTESIAN_POINT('Ctrl Pts',(18.5576066734871,-22.8447237855104,-4.67328040594355));
#12050=CARTESIAN_POINT('Ctrl Pts',(18.550083524438,-22.7654377266669,-4.80916147563916));
#12051=CARTESIAN_POINT('Ctrl Pts',(18.5469055500268,-22.688023391011,-4.94611816810261));
#12052=CARTESIAN_POINT('Ctrl Pts',(18.5482422492798,-22.6134330595748,-5.08419756762781));
#12053=CARTESIAN_POINT('Ctrl Pts',(18.5493897722915,-22.5493991180712,-5.20273529258207));
#12054=CARTESIAN_POINT('Ctrl Pts',(18.5538649455709,-22.4874464626935,-5.32210048770187));
#12055=CARTESIAN_POINT('Ctrl Pts',(18.5617935035834,-22.4282022173725,-5.4423250357486));
#12056=CARTESIAN_POINT('Ctrl Pts',(18.5622006166617,-22.4251601626828,-5.44849828765209));
#12057=CARTESIAN_POINT('Ctrl Pts',(18.5626168311325,-22.4221253454031,-5.45467369029037));
#12058=CARTESIAN_POINT('Ctrl Pts',(18.5630421649904,-22.4190978469191,-5.46085125802884));
#12059=CARTESIAN_POINT('Ctrl Pts',(18.5704667943542,-22.3662498224316,-5.56868690281898));
#12060=CARTESIAN_POINT('Ctrl Pts',(18.5806898704857,-22.3154805383714,-5.67744898745817));
#12061=CARTESIAN_POINT('Ctrl Pts',(18.5939729051555,-22.2675991944941,-5.78732953813166));
#12062=CARTESIAN_POINT('Ctrl Pts',(18.6062339812058,-22.2234017039909,-5.88875619414482));
#12063=CARTESIAN_POINT('Ctrl Pts',(18.6211023693495,-22.1816645409984,-5.9911357802801));
#12064=CARTESIAN_POINT('Ctrl Pts',(18.6388065796653,-22.1430604940117,-6.09462575761987));
#12065=CARTESIAN_POINT('Ctrl Pts',(18.6521360572901,-22.1139955557083,-6.17254323107633));
#12066=CARTESIAN_POINT('Ctrl Pts',(18.6670734617826,-22.0867072848215,-6.25109024348722));
#12067=CARTESIAN_POINT('Ctrl Pts',(18.6837256783403,-22.0614998943556,-6.33033707037954));
#12068=CARTESIAN_POINT('Ctrl Pts',(18.684854008829,-22.0597918774616,-6.3357067225579));
#12069=CARTESIAN_POINT('Ctrl Pts',(18.6859900272502,-22.0580937292927,-6.34107869209401));
#12070=CARTESIAN_POINT('Ctrl Pts',(18.6871337613023,-22.0564055371513,-6.34645300238936));
#12071=CARTESIAN_POINT('Ctrl Pts',(18.708148865036,-22.0253864965688,-6.44520121064056));
#12072=CARTESIAN_POINT('Ctrl Pts',(18.731565451134,-21.9978800256313,-6.54382562252798));
#12073=CARTESIAN_POINT('Ctrl Pts',(18.757547417001,-21.9749039650105,-6.64250010567014));
#12074=CARTESIAN_POINT('Ctrl Pts',(18.7820352329043,-21.9532491931759,-6.73550009612159));
#12075=CARTESIAN_POINT('Ctrl Pts',(18.8088018953359,-21.9356181609281,-6.82854447867061));
#12076=CARTESIAN_POINT('Ctrl Pts',(18.838001488254,-21.922905503098,-6.92177945640448));
#12077=CARTESIAN_POINT('Ctrl Pts',(18.8654018755781,-21.9109761673213,-7.00926952892805));
#12078=CARTESIAN_POINT('Ctrl Pts',(18.8949446624786,-21.9033774739727,-7.09692737855105));
#12079=CARTESIAN_POINT('Ctrl Pts',(18.9267718005847,-21.9008931019119,-7.18487534317515));
#12080=CARTESIAN_POINT('Ctrl Pts',(18.9343523672068,-21.900301375824,-7.20582273099513));
#12081=CARTESIAN_POINT('Ctrl Pts',(18.9420625907237,-21.9000000019656,-7.22678658601776));
#12082=CARTESIAN_POINT('Ctrl Pts',(18.9499045174787,-21.9,-7.24776858010006));
#12083=CARTESIAN_POINT('Origin',(24.8980443547237,-21.9,-5.02467783148466));
#12084=CARTESIAN_POINT('Ctrl Pts',(19.3987830406925,7.75488674445212,-8.19967783148469));
#12085=CARTESIAN_POINT('Ctrl Pts',(19.3659933398565,7.77600035063379,-8.14288440367171));
#12086=CARTESIAN_POINT('Ctrl Pts',(19.3347983130256,7.79969631458858,-8.08684223874884));
#12087=CARTESIAN_POINT('Ctrl Pts',(19.3050236136449,7.82564845387891,-8.03146894177519));
#12088=CARTESIAN_POINT('Ctrl Pts',(19.274510466767,7.85224423668899,-7.97472232203361));
#12089=CARTESIAN_POINT('Ctrl Pts',(19.2454890567992,7.88120973563673,-7.91867817937499));
#12090=CARTESIAN_POINT('Ctrl Pts',(19.2177926283953,7.91224591462514,-7.86325066964015));
#12091=CARTESIAN_POINT('Ctrl Pts',(19.1889838553875,7.9445285693584,-7.80559707896577));
#12092=CARTESIAN_POINT('Ctrl Pts',(19.1616086716191,7.97905171373433,-7.74861066271193));
#12093=CARTESIAN_POINT('Ctrl Pts',(19.1355008176972,8.01553158395357,-7.69219756552196));
#12094=CARTESIAN_POINT('Ctrl Pts',(19.1213519132884,8.03530150445801,-7.66162502126256));
#12095=CARTESIAN_POINT('Ctrl Pts',(19.1075755834705,8.05564699923641,-7.63122090588109));
#12096=CARTESIAN_POINT('Ctrl Pts',(19.0941477565058,8.07652873453469,-7.60097057057968));
#12097=CARTESIAN_POINT('Ctrl Pts',(19.0765900909801,8.10383281917408,-7.56141649599528));
#12098=CARTESIAN_POINT('Ctrl Pts',(19.0596305575383,8.1320607616409,-7.52212648307875));
#12099=CARTESIAN_POINT('Ctrl Pts',(19.0432284984429,8.16115913750229,-7.48307015825894));
#12100=CARTESIAN_POINT('Ctrl Pts',(19.0141380564244,8.21276757342507,-7.41380045583827));
#12101=CARTESIAN_POINT('Ctrl Pts',(18.9869139995712,8.26690043732857,-7.34553583063077));
#12102=CARTESIAN_POINT('Ctrl Pts',(18.9613635126329,8.32314897453513,-7.27822357400233));
#12103=CARTESIAN_POINT('Ctrl Pts',(18.9351126024384,8.3809394699705,-7.20906606604536));
#12104=CARTESIAN_POINT('Ctrl Pts',(18.9106283204154,8.44096333238581,-7.14091388358974));
#12105=CARTESIAN_POINT('Ctrl Pts',(18.887721787102,8.50282830726884,-7.07371326896348));
#12106=CARTESIAN_POINT('Ctrl Pts',(18.8800990296721,8.52341552099025,-7.05135047938608));
#12107=CARTESIAN_POINT('Ctrl Pts',(18.8726511518925,8.54420702221443,-7.02909309225845));
#12108=CARTESIAN_POINT('Ctrl Pts',(18.8653716576552,8.56518952756256,-7.00693919929548));
#12109=CARTESIAN_POINT('Ctrl Pts',(18.8455112487693,8.62243541884095,-6.94649744904164));
#12110=CARTESIAN_POINT('Ctrl Pts',(18.8269429374958,8.68106595956028,-6.88689923383952));
#12111=CARTESIAN_POINT('Ctrl Pts',(18.8095678533225,8.74069382312873,-6.82822690195023));
#12112=CARTESIAN_POINT('Ctrl Pts',(18.7915326474107,8.8025870943678,-6.76732546536456));
#12113=CARTESIAN_POINT('Ctrl Pts',(18.774743007695,8.8656873632306,-6.70728694724099));
#12114=CARTESIAN_POINT('Ctrl Pts',(18.7591026725021,8.92967013781577,-6.64815746785353));
#12115=CARTESIAN_POINT('Ctrl Pts',(18.742709086539,8.9967343728454,-6.58618026651254));
#12116=CARTESIAN_POINT('Ctrl Pts',(18.7275781376305,9.06476837724079,-6.52520162749384));
#12117=CARTESIAN_POINT('Ctrl Pts',(18.7136124004985,9.13345255195979,-6.46526235393202));
#12118=CARTESIAN_POINT('Ctrl Pts',(18.7102586327819,9.14994654476804,-6.45086838398035));
#12119=CARTESIAN_POINT('Ctrl Pts',(18.7069721205914,9.16647825760674,-6.4365343050853));
#12120=CARTESIAN_POINT('Ctrl Pts',(18.7037516259637,9.18304367617655,-6.42226059842027));
#12121=CARTESIAN_POINT('Ctrl Pts',(18.687769896146,9.26524969559492,-6.35142721728163));
#12122=CARTESIAN_POINT('Ctrl Pts',(18.6733405598788,9.3484887946591,-6.28186427922348));
#12123=CARTESIAN_POINT('Ctrl Pts',(18.6602859966245,9.43264075174974,-6.21337432473624));
#12124=CARTESIAN_POINT('Ctrl Pts',(18.646571873904,9.5210443424501,-6.14142403251602));
#12125=CARTESIAN_POINT('Ctrl Pts',(18.6343749888335,9.61045552746124,-6.07065794451291));
#12126=CARTESIAN_POINT('Ctrl Pts',(18.6235205378729,9.70078270753026,-6.00086150882515));
#12127=CARTESIAN_POINT('Ctrl Pts',(18.6161783626755,9.76188188090751,-5.95364975570785));
#12128=CARTESIAN_POINT('Ctrl Pts',(18.6094510649912,9.82340116495387,-5.90688196330237));
#12129=CARTESIAN_POINT('Ctrl Pts',(18.6032917953032,9.88532296597222,-5.86049492614831));
#12130=CARTESIAN_POINT('Ctrl Pts',(18.5958522251418,9.96011618116425,-5.80446561829669));
#12131=CARTESIAN_POINT('Ctrl Pts',(18.5892429598932,10.0354996811098,-5.74899278472943));
#12132=CARTESIAN_POINT('Ctrl Pts',(18.5834093822803,10.1114780191919,-5.69397500136636));
#12133=CARTESIAN_POINT('Ctrl Pts',(18.5744962659343,10.227565232225,-5.60991339513627));
#12134=CARTESIAN_POINT('Ctrl Pts',(18.5674119899894,10.3447938290842,-5.52708927818022));
#12135=CARTESIAN_POINT('Ctrl Pts',(18.5619848534477,10.4630236268635,-5.44527716353466));
#12136=CARTESIAN_POINT('Ctrl Pts',(18.5591153047811,10.5255365479887,-5.40201975832896));
#12137=CARTESIAN_POINT('Ctrl Pts',(18.5567095288543,10.5883301347813,-5.35904550681142));
#12138=CARTESIAN_POINT('Ctrl Pts',(18.5547452601808,10.6513883422589,-5.31632247370023));
#12139=CARTESIAN_POINT('Ctrl Pts',(18.550986304919,10.7720607248062,-5.23456483418908));
#12140=CARTESIAN_POINT('Ctrl Pts',(18.5488549654409,10.8936995222446,-5.15373844823809));
#12141=CARTESIAN_POINT('Ctrl Pts',(18.5482368634436,11.015983366569,-5.07379765702776));
#12142=CARTESIAN_POINT('Ctrl Pts',(18.5475644047114,11.1490210193612,-4.98682676333589));
#12143=CARTESIAN_POINT('Ctrl Pts',(18.548682841922,11.2828228206765,-4.90090379058647));
#12144=CARTESIAN_POINT('Ctrl Pts',(18.5514751742199,11.4170275976682,-4.81597194686246));
#12145=CARTESIAN_POINT('Ctrl Pts',(18.5517976286767,11.4325253693733,-4.80616414155158));
#12146=CARTESIAN_POINT('Ctrl Pts',(18.5521424374349,11.4480285606957,-4.79636955823295));
#12147=CARTESIAN_POINT('Ctrl Pts',(18.5525094453159,11.463536648638,-4.78658811388329));
#12148=CARTESIAN_POINT('Ctrl Pts',(18.5536511731741,11.5117808879334,-4.75615893759702));
#12149=CARTESIAN_POINT('Ctrl Pts',(18.555003897283,11.5600961433565,-4.72583964632702));
#12150=CARTESIAN_POINT('Ctrl Pts',(18.5565660506262,11.6084844905168,-4.69561821617437));
#12151=CARTESIAN_POINT('Ctrl Pts',(18.5624098021704,11.7894971162455,-4.58256495549814));
#12152=CARTESIAN_POINT('Ctrl Pts',(18.5711795421502,11.9714205652654,-4.47095775394613));
#12153=CARTESIAN_POINT('Ctrl Pts',(18.5827826956393,12.1538289691793,-4.36049732049744));
#12154=CARTESIAN_POINT('Ctrl Pts',(18.5875094067414,12.2281356504364,-4.31549967760564));
#12155=CARTESIAN_POINT('Ctrl Pts',(18.5927064632334,12.302523301945,-4.27069266980417));
#12156=CARTESIAN_POINT('Ctrl Pts',(18.5983681540258,12.3769650887378,-4.22605743572654));
#12157=CARTESIAN_POINT('Ctrl Pts',(18.6089990472484,12.5167435958486,-4.14224635793386));
#12158=CARTESIAN_POINT('Ctrl Pts',(18.6213040079066,12.6571275039462,-4.05879388233315));
#12159=CARTESIAN_POINT('Ctrl Pts',(18.6352049098432,12.7973698716139,-3.97593038921648));
#12160=CARTESIAN_POINT('Ctrl Pts',(18.6468806128429,12.9151628206142,-3.9063313416461));
#12161=CARTESIAN_POINT('Ctrl Pts',(18.6596812296299,13.0328551938122,-3.83714732492099));
#12162=CARTESIAN_POINT('Ctrl Pts',(18.6735332660427,13.15,-3.76850837361349));
#12163=CARTESIAN_POINT('Origin',(24.8980443547236,25.4,5.02467783148503));
#12164=CARTESIAN_POINT('',(18.9499045174786,-21.9,7.24776858010033));
#12165=CARTESIAN_POINT('Origin',(24.8980443547236,-21.9,5.02467783148503));
#12166=CARTESIAN_POINT('Ctrl Pts',(18.9499045174786,-21.9,7.24776858010033));
#12167=CARTESIAN_POINT('Ctrl Pts',(18.9165632864596,-21.9000000083571,7.15856020902048));
#12168=CARTESIAN_POINT('Ctrl Pts',(18.8856015389054,-21.905443504867,7.06967956038967));
#12169=CARTESIAN_POINT('Ctrl Pts',(18.8568682193457,-21.9155046710502,6.98099906869269));
#12170=CARTESIAN_POINT('Ctrl Pts',(18.8268402135435,-21.9260191803779,6.88832274865634));
#12171=CARTESIAN_POINT('Ctrl Pts',(18.7992459742723,-21.9415773497166,6.79586509501603));
#12172=CARTESIAN_POINT('Ctrl Pts',(18.7739308975765,-21.9612924551018,6.70348260201988));
#12173=CARTESIAN_POINT('Ctrl Pts',(18.7465025188002,-21.9826533770779,6.60338802041375));
#12174=CARTESIAN_POINT('Ctrl Pts',(18.721749596084,-22.008894721168,6.50338176627315));
#12175=CARTESIAN_POINT('Ctrl Pts',(18.6994970857502,-22.038945623935,6.4032824569844));
#12176=CARTESIAN_POINT('Ctrl Pts',(18.6952867728324,-22.0446314410502,6.38434304706415));
#12177=CARTESIAN_POINT('Ctrl Pts',(18.6911660325344,-22.050453774454,6.36540030635649));
#12178=CARTESIAN_POINT('Ctrl Pts',(18.6871337620087,-22.0564055499457,6.34645300571088));
#12179=CARTESIAN_POINT('Ctrl Pts',(18.685989086576,-22.0580951318186,6.34107427196059));
#12180=CARTESIAN_POINT('Ctrl Pts',(18.6848521394506,-22.0597946861619,6.33569788268522));
#12181=CARTESIAN_POINT('Ctrl Pts',(18.6837228928666,-22.0615041254602,6.33032381442206));
#12182=CARTESIAN_POINT('Ctrl Pts',(18.6618144150191,-22.0946689041087,6.22606168322978));
#12183=CARTESIAN_POINT('Ctrl Pts',(18.6428733488885,-22.1314339084881,6.12301066612014));
#12184=CARTESIAN_POINT('Ctrl Pts',(18.6266592786348,-22.1711120177009,6.02101172312584));
#12185=CARTESIAN_POINT('Ctrl Pts',(18.6091920393942,-22.2138568075897,5.91112938564402));
#12186=CARTESIAN_POINT('Ctrl Pts',(18.5948895381154,-22.2599827034673,5.80246810970979));
#12187=CARTESIAN_POINT('Ctrl Pts',(18.5834816916671,-22.3086850460264,5.6948387914714));
#12188=CARTESIAN_POINT('Ctrl Pts',(18.575159021454,-22.3442161638022,5.61631710685588));
#12189=CARTESIAN_POINT('Ctrl Pts',(18.5683777065849,-22.3811198321318,5.53834489827507));
#12190=CARTESIAN_POINT('Ctrl Pts',(18.5630421655769,-22.4190978671499,5.46085126655351));
#12191=CARTESIAN_POINT('Ctrl Pts',(18.5626162561593,-22.4221294627745,5.4546653394841));
#12192=CARTESIAN_POINT('Ctrl Pts',(18.5621994908211,-22.4251683970663,5.44848158330734));
#12193=CARTESIAN_POINT('Ctrl Pts',(18.5617918514945,-22.4282145883129,5.44229998359246));
#12194=CARTESIAN_POINT('Ctrl Pts',(18.5501487347855,-22.5152208163553,5.26573927846711));
#12195=CARTESIAN_POINT('Ctrl Pts',(18.5459412848334,-22.6081793563307,5.09080840328421));
#12196=CARTESIAN_POINT('Ctrl Pts',(18.5488182589122,-22.7050299994319,4.91761922059265));
#12197=CARTESIAN_POINT('Ctrl Pts',(18.551725093913,-22.8028858825601,4.74263245873062));
#12198=CARTESIAN_POINT('Ctrl Pts',(18.5618641457036,-22.9047151986039,4.56942390981763));
#12199=CARTESIAN_POINT('Ctrl Pts',(18.5788839843097,-23.0084452391659,4.39810529844962));
#12200=CARTESIAN_POINT('Ctrl Pts',(18.5962005664483,-23.1139838291145,4.22379972045343));
#12201=CARTESIAN_POINT('Ctrl Pts',(18.6206399139399,-23.221490102855,4.05145060942632));
#12202=CARTESIAN_POINT('Ctrl Pts',(18.6518436149472,-23.3288332397547,3.88117008435452));
#12203=CARTESIAN_POINT('Ctrl Pts',(18.6587439273645,-23.3525708464022,3.84351465299085));
#12204=CARTESIAN_POINT('Ctrl Pts',(18.6659750759472,-23.3763006710624,3.80596035731296));
#12205=CARTESIAN_POINT('Ctrl Pts',(18.6735332660427,-23.4,3.76850837361377));
#12206=CARTESIAN_POINT('Ctrl Pts',(18.6735332660427,13.15,3.76850837361377));
#12207=CARTESIAN_POINT('Ctrl Pts',(18.6523859914636,12.9711603487853,3.87329634174011));
#12208=CARTESIAN_POINT('Ctrl Pts',(18.6338557671018,12.7922384035346,3.97865911562495));
#12209=CARTESIAN_POINT('Ctrl Pts',(18.6179567083012,12.613568472743,4.0848412819067));
#12210=CARTESIAN_POINT('Ctrl Pts',(18.6029835009531,12.4453030455777,4.18484013167159));
#12211=CARTESIAN_POINT('Ctrl Pts',(18.5903442052403,12.2772593408527,4.28556583286555));
#12212=CARTESIAN_POINT('Ctrl Pts',(18.5800917993731,12.1097298655906,4.3872330641218));
#12213=CARTESIAN_POINT('Ctrl Pts',(18.5705721029945,11.9541732323843,4.48163443544397));
#12214=CARTESIAN_POINT('Ctrl Pts',(18.5631106028855,11.7990589456247,4.57684766352013));
#12215=CARTESIAN_POINT('Ctrl Pts',(18.5577824015727,11.644651703523,4.67305239657088));
#12216=CARTESIAN_POINT('Ctrl Pts',(18.5573723019746,11.6327673274996,4.68045705717646));
#12217=CARTESIAN_POINT('Ctrl Pts',(18.5569748561328,11.6208871602234,4.6878675951984));
#12218=CARTESIAN_POINT('Ctrl Pts',(18.5565901063719,11.6090113330857,4.69528409440914));
#12219=CARTESIAN_POINT('Ctrl Pts',(18.555006490882,11.5601308769556,4.72581012515259));
#12220=CARTESIAN_POINT('Ctrl Pts',(18.5536380790451,11.5113297193643,4.75643443240897));
#12221=CARTESIAN_POINT('Ctrl Pts',(18.5524879351211,11.4626185033473,4.7871620937435));
#12222=CARTESIAN_POINT('Ctrl Pts',(18.5490109152155,11.3153587872477,4.88005541594978));
#12223=CARTESIAN_POINT('Ctrl Pts',(18.5474918941389,11.1688712791072,4.97388804059575));
#12224=CARTESIAN_POINT('Ctrl Pts',(18.5481215194284,11.0233411943008,5.0689474334615));
#12225=CARTESIAN_POINT('Ctrl Pts',(18.5487269577732,10.8834016220832,5.16035513648454));
#12226=CARTESIAN_POINT('Ctrl Pts',(18.5513191063689,10.7443469554757,5.25289693475043));
#12227=CARTESIAN_POINT('Ctrl Pts',(18.5560962085703,10.6063775974687,5.34684107597172));
#12228=CARTESIAN_POINT('Ctrl Pts',(18.5606430100288,10.4750596453383,5.4362562361061));
#12229=CARTESIAN_POINT('Ctrl Pts',(18.5671691933421,10.3447246753313,5.52694161369977));
#12230=CARTESIAN_POINT('Ctrl Pts',(18.5758722092291,10.2155824311613,5.61914300600576));
#12231=CARTESIAN_POINT('Ctrl Pts',(18.5781116021647,10.1823525447605,5.64286755727109));
#12232=CARTESIAN_POINT('Ctrl Pts',(18.5804952642956,10.1492018356779,5.66669256882812));
#12233=CARTESIAN_POINT('Ctrl Pts',(18.583026861788,10.1161343255489,5.6906224166687));
#12234=CARTESIAN_POINT('Ctrl Pts',(18.5887804904878,10.0409809190982,5.7450084159185));
#12235=CARTESIAN_POINT('Ctrl Pts',(18.5952987308817,9.96626705526658,5.79994421287305));
#12236=CARTESIAN_POINT('Ctrl Pts',(18.6026307701818,9.89202045142468,5.85550139909491));
#12237=CARTESIAN_POINT('Ctrl Pts',(18.6125651424763,9.79142178112723,5.93077728742091));
#12238=CARTESIAN_POINT('Ctrl Pts',(18.6240096843225,9.69169193896002,6.00719763544296));
#12239=CARTESIAN_POINT('Ctrl Pts',(18.6371798032762,9.59300570027836,6.08498075574783));
#12240=CARTESIAN_POINT('Ctrl Pts',(18.6455543610639,9.5302535253287,6.13444114697063));
#12241=CARTESIAN_POINT('Ctrl Pts',(18.6546271676009,9.46792401681184,6.18445282728303));
#12242=CARTESIAN_POINT('Ctrl Pts',(18.6644598889995,9.40607058542617,6.23507539236576));
#12243=CARTESIAN_POINT('Ctrl Pts',(18.6762217842539,9.33208154906527,6.2956300734025));
#12244=CARTESIAN_POINT('Ctrl Pts',(18.6890749173201,9.25875668204223,6.35708172070533));
#12245=CARTESIAN_POINT('Ctrl Pts',(18.7031431886276,9.18618721050011,6.41956117514028));
#12246=CARTESIAN_POINT('Ctrl Pts',(18.718114943111,9.10895723055633,6.48605314359989));
#12247=CARTESIAN_POINT('Ctrl Pts',(18.7343958888087,9.03297713418459,6.55338142599361));
#12248=CARTESIAN_POINT('Ctrl Pts',(18.7521243088799,8.95848778473355,6.62161451308793));
#12249=CARTESIAN_POINT('Ctrl Pts',(18.7697284018762,8.88452081927939,6.68936909052928));
#12250=CARTESIAN_POINT('Ctrl Pts',(18.7887596218306,8.81202334049326,6.75801585334146));
#12251=CARTESIAN_POINT('Ctrl Pts',(18.8093722108493,8.74127840230463,6.82762171485896));
#12252=CARTESIAN_POINT('Ctrl Pts',(18.8264816925845,8.68255655874079,6.88539806770923));
#12253=CARTESIAN_POINT('Ctrl Pts',(18.844686454666,8.62503122998396,6.94385527579565));
#12254=CARTESIAN_POINT('Ctrl Pts',(18.8641031487985,8.56885520307105,7.00307453684398));
#12255=CARTESIAN_POINT('Ctrl Pts',(18.883281836806,8.51336777115753,7.06156789951063));
#12256=CARTESIAN_POINT('Ctrl Pts',(18.9036461322825,8.45914957373892,7.12083493263501));
#12257=CARTESIAN_POINT('Ctrl Pts',(18.9253603775997,8.40640557244459,7.18099413813338));
#12258=CARTESIAN_POINT('Ctrl Pts',(18.9461639547566,8.35587358828098,7.23863034215543));
#12259=CARTESIAN_POINT('Ctrl Pts',(18.9682065803238,8.3066946247827,7.2970854228075));
#12260=CARTESIAN_POINT('Ctrl Pts',(18.9916533217175,8.25909114268859,7.35646892349916));
#12261=CARTESIAN_POINT('Ctrl Pts',(19.007113608556,8.22770241044106,7.39562515159708));
#12262=CARTESIAN_POINT('Ctrl Pts',(19.0231847925363,8.19699952043896,7.43518514669757));
#12263=CARTESIAN_POINT('Ctrl Pts',(19.0399196080641,8.16705743584222,7.47518178268543));
#12264=CARTESIAN_POINT('Ctrl Pts',(19.056966546358,8.1365568983451,7.51592440004612));
#12265=CARTESIAN_POINT('Ctrl Pts',(19.0746913261222,8.10686980879578,7.55709495999028));
#12266=CARTESIAN_POINT('Ctrl Pts',(19.0931655915326,8.07806532466688,7.59875680177766));
#12267=CARTESIAN_POINT('Ctrl Pts',(19.1144962432219,8.04480725435168,7.64686016156793));
#12268=CARTESIAN_POINT('Ctrl Pts',(19.1368503227078,8.01279246823063,7.69561131443679));
#12269=CARTESIAN_POINT('Ctrl Pts',(19.1602597784354,7.98223072787771,7.74495049952548));
#12270=CARTESIAN_POINT('Ctrl Pts',(19.1829240735601,7.95264181684349,7.79271913904772));
#12271=CARTESIAN_POINT('Ctrl Pts',(19.2065777448217,7.92441470275061,7.84103922249812));
#12272=CARTESIAN_POINT('Ctrl Pts',(19.2312525356177,7.89778233068509,7.88983809439884));
#12273=CARTESIAN_POINT('Ctrl Pts',(19.2551825374087,7.87195383566371,7.93716401102529));
#12274=CARTESIAN_POINT('Ctrl Pts',(19.2800730507017,7.84762505828644,7.984940478531));
#12275=CARTESIAN_POINT('Ctrl Pts',(19.3059540467289,7.82505223561007,8.0330801379758));
#12276=CARTESIAN_POINT('Ctrl Pts',(19.3308135357918,7.80337034833451,8.07931975472781));
#12277=CARTESIAN_POINT('Ctrl Pts',(19.3565869534279,7.78330843074937,8.1258946220068));
#12278=CARTESIAN_POINT('Ctrl Pts',(19.3833004152209,7.76513667663444,8.17270481742561));
#12279=CARTESIAN_POINT('Ctrl Pts',(19.3884266184092,7.76164959193525,8.18168750094523));
#12280=CARTESIAN_POINT('Ctrl Pts',(19.3935874341475,7.75823224575957,8.19067877697312));
#12281=CARTESIAN_POINT('Ctrl Pts',(19.3987830406924,7.75488674445212,8.19967783148497));
#12282=CARTESIAN_POINT('Origin',(-8.09752352946369,25.4,24.0746778314847));
#12283=CARTESIAN_POINT('',(-3.19820054762209,-21.9,20.0349830014761));
#12284=CARTESIAN_POINT('Ctrl Pts',(-6.07314264709777,-23.4,18.0560083736135));
#12285=CARTESIAN_POINT('Ctrl Pts',(-5.92577312631869,-23.3035563481381,
18.1055761464572));
#12286=CARTESIAN_POINT('Ctrl Pts',(-5.7799969640134,-23.2068396384742,18.1605585901307));
#12287=CARTESIAN_POINT('Ctrl Pts',(-5.63584724081203,-23.1112816984186,
18.2211313626838));
#12288=CARTESIAN_POINT('Ctrl Pts',(-5.4996399026027,-23.0209888253512,18.2783666867219));
#12289=CARTESIAN_POINT('Ctrl Pts',(-5.36488465057871,-22.9317288900636,
18.3405935419584));
#12290=CARTESIAN_POINT('Ctrl Pts',(-5.23162378740032,-22.8447237863145,
18.4079990150367));
#12291=CARTESIAN_POINT('Ctrl Pts',(-5.11018575539893,-22.7654377279672,
18.4694243112679));
#12292=CARTESIAN_POINT('Ctrl Pts',(-4.98998879405928,-22.688023392779,18.5351504504473));
#12293=CARTESIAN_POINT('Ctrl Pts',(-4.87107687669821,-22.6134330617646,
18.6053477651812));
#12294=CARTESIAN_POINT('Ctrl Pts',(-4.7689939559047,-22.5493991194829,18.6656104123483));
#12295=CARTESIAN_POINT('Ctrl Pts',(-4.66785825008194,-22.4874464633674,
18.7291686243386));
#12296=CARTESIAN_POINT('Ctrl Pts',(-4.56770501518154,-22.4282022173721,
18.7961472317784));
#12297=CARTESIAN_POINT('Ctrl Pts',(-4.56256237874832,-22.4251601626824,
18.7995864279981));
#12298=CARTESIAN_POINT('Ctrl Pts',(-4.55742243042036,-22.4221253454027,
18.8030345816224));
#12299=CARTESIAN_POINT('Ctrl Pts',(-4.55228516675424,-22.4190978469188,
18.8064917154177));
#12300=CARTESIAN_POINT('Ctrl Pts',(-4.46260907364606,-22.36624982245,18.8668394554341));
#12301=CARTESIAN_POINT('Ctrl Pts',(-4.37352988347701,-22.3154805384071,
18.9300739413651));
#12302=CARTESIAN_POINT('Ctrl Pts',(-4.28501205257774,-22.2675991945448,
18.9965176621394));
#12303=CARTESIAN_POINT('Ctrl Pts',(-4.20330452989676,-22.223401704052,19.0578493934644));
#12304=CARTESIAN_POINT('Ctrl Pts',(-4.12207540156842,-22.1816645410681,
19.1219155883572));
#12305=CARTESIAN_POINT('Ctrl Pts',(-4.04130255733465,-22.1430604940879,
19.188992872892));
#12306=CARTESIAN_POINT('Ctrl Pts',(-3.98048878468141,-22.113995555756,19.2394952759037));
#12307=CARTESIAN_POINT('Ctrl Pts',(-3.91993377873524,-22.0867072848434,
19.2917049539104));
#12308=CARTESIAN_POINT('Ctrl Pts',(-3.85963012170325,-22.0614998943553,
19.3457496099721));
#12309=CARTESIAN_POINT('Ctrl Pts',(-3.85554403175164,-22.0597918774613,
19.3494115989283));
#12310=CARTESIAN_POINT('Ctrl Pts',(-3.85145977887563,-22.0580937292924,
19.3530814045083));
#12311=CARTESIAN_POINT('Ctrl Pts',(-3.84737735665805,-22.0564055371509,
19.3567590624002));
#12312=CARTESIAN_POINT('Ctrl Pts',(-3.77236645160972,-22.0253864965719,
19.4243327802147));
#12313=CARTESIAN_POINT('Ctrl Pts',(-3.69866349853912,-21.997880025637,19.493924344581));
#12314=CARTESIAN_POINT('Ctrl Pts',(-3.62619987237413,-21.9749039650179,
19.5657626286246));
#12315=CARTESIAN_POINT('Ctrl Pts',(-3.55790342605073,-21.9532491931849,
19.6334696944975));
#12316=CARTESIAN_POINT('Ctrl Pts',(-3.49070795830701,-21.9356181609376,
19.7031724954035));
#12317=CARTESIAN_POINT('Ctrl Pts',(-3.42456389553437,-21.9229055031068,
19.7750775735084));
#12318=CARTESIAN_POINT('Ctrl Pts',(-3.36249546381872,-21.9109761673294,
19.8425520412577));
#12319=CARTESIAN_POINT('Ctrl Pts',(-3.30135293266074,-21.9033774739789,
19.9119657700143));
#12320=CARTESIAN_POINT('Ctrl Pts',(-3.24110133014448,-21.9008931019147,
19.9835028624463));
#12321=CARTESIAN_POINT('Ctrl Pts',(-3.22675064343828,-21.900301375825,20.0005415196519));
#12322=CARTESIAN_POINT('Ctrl Pts',(-3.21245052416384,-21.9000000019656,
20.017700696624));
#12323=CARTESIAN_POINT('Ctrl Pts',(-3.19820054762209,-21.9,20.0349830014761));
#12324=CARTESIAN_POINT('Origin',(-8.09752352946369,-21.9,24.0746778314847));
#12325=CARTESIAN_POINT('Ctrl Pts',(-2.59826221543248,7.75488674445211,20.8996778314848));
#12326=CARTESIAN_POINT('Ctrl Pts',(-2.63105191627123,7.77600035063574,20.8428844036671));
#12327=CARTESIAN_POINT('Ctrl Pts',(-2.66398834136481,7.79969631459274,20.7878476354939));
#12328=CARTESIAN_POINT('Ctrl Pts',(-2.69705567354774,7.82564845388557,20.7343753409493));
#12329=CARTESIAN_POINT('Ctrl Pts',(-2.73094311438655,7.85224423669808,20.6795768707287));
#12330=CARTESIAN_POINT('Ctrl Pts',(-2.76496806068104,7.88120973564853,20.6264215211099));
#12331=CARTESIAN_POINT('Ctrl Pts',(-2.7991214779807,7.91224591463994,20.574721955647));
#12332=CARTESIAN_POINT('Ctrl Pts',(-2.83464656562271,7.94452856937605,20.5209460310299));
#12333=CARTESIAN_POINT('Ctrl Pts',(-2.87031065788748,7.97905171375511,20.4687452183232));
#12334=CARTESIAN_POINT('Ctrl Pts',(-2.90611190620181,8.01553158397781,20.4179286049906));
#12335=CARTESIAN_POINT('Ctrl Pts',(-2.92551405397642,8.03530150447458,20.3903890222189));
#12336=CARTESIAN_POINT('Ctrl Pts',(-2.9449566253594,8.05564699924486,20.3632563129462));
#12337=CARTESIAN_POINT('Ctrl Pts',(-2.9644402707131,8.07652873453461,20.3365023060375));
#12338=CARTESIAN_POINT('Ctrl Pts',(-2.98991627136349,8.1038328191741,20.3015198843688));
#12339=CARTESIAN_POINT('Ctrl Pts',(-3.01546265394331,8.13206076164095,20.2671874911136));
#12340=CARTESIAN_POINT('Ctrl Pts',(-3.04108539386802,8.16115913750231,20.2334547288528));
#12341=CARTESIAN_POINT('Ctrl Pts',(-3.08652949487372,8.21276757343192,20.1736268158392));
#12342=CARTESIAN_POINT('Ctrl Pts',(-3.13203636606265,8.26690043734288,20.1159177783991));
#12343=CARTESIAN_POINT('Ctrl Pts',(-3.17755524682584,8.32314897455742,20.0601342793104));
#12344=CARTESIAN_POINT('Ctrl Pts',(-3.22432195048657,8.38093946999923,20.0028215702257));
#12345=CARTESIAN_POINT('Ctrl Pts',(-3.27110133080977,8.4409633324214,19.9475414687676));
#12346=CARTESIAN_POINT('Ctrl Pts',(-3.31784550357409,8.50282830731164,19.8941035216878));
#12347=CARTESIAN_POINT('Ctrl Pts',(-3.33340086872185,8.52341552101904,19.8763206253306));
#12348=CARTESIAN_POINT('Ctrl Pts',(-3.3489523924956,8.54420702222892,19.8587418804176));
#12349=CARTESIAN_POINT('Ctrl Pts',(-3.36449847946483,8.56518952756249,19.8413607070121));
#12350=CARTESIAN_POINT('Ctrl Pts',(-3.40691236619082,8.62243541884093,19.7939402132604));
#12351=CARTESIAN_POINT('Ctrl Pts',(-3.44924177893934,8.68106595956033,19.7480604763911));
#12352=CARTESIAN_POINT('Ctrl Pts',(-3.49136596676808,8.74069382312879,19.7036770461595));
#12353=CARTESIAN_POINT('Ctrl Pts',(-3.53509055502149,8.80258709436672,19.6576073813855));
#12354=CARTESIAN_POINT('Ctrl Pts',(-3.57869061706342,8.86568736322834,19.6130478678103));
#12355=CARTESIAN_POINT('Ctrl Pts',(-3.62207808072827,8.92967013781227,19.5699382005166));
#12356=CARTESIAN_POINT('Ctrl Pts',(-3.66755511856297,8.99673437284105,19.5247523379434));
#12357=CARTESIAN_POINT('Ctrl Pts',(-3.71279869458657,9.06476837723555,19.4811592322964));
#12358=CARTESIAN_POINT('Ctrl Pts',(-3.75772475960894,9.13345255195358,19.439094912377));
#12359=CARTESIAN_POINT('Ctrl Pts',(-3.76851341939143,9.14994654476389,19.4289934793589));
#12360=CARTESIAN_POINT('Ctrl Pts',(-3.77928383976051,9.16647825760466,19.4189802368632));
#12361=CARTESIAN_POINT('Ctrl Pts',(-3.7900349850261,9.18304367617654,19.4090543533692));
#12362=CARTESIAN_POINT('Ctrl Pts',(-3.84338762762093,9.26524969559742,19.3597970787797));
#12363=CARTESIAN_POINT('Ctrl Pts',(-3.89641623100928,9.34848879466418,19.312519437982));
#12364=CARTESIAN_POINT('Ctrl Pts',(-3.94920298987383,9.43264075175752,19.2669688773235));
#12365=CARTESIAN_POINT('Ctrl Pts',(-4.00465670938737,9.52104434245995,19.2191169525459));
#12366=CARTESIAN_POINT('Ctrl Pts',(-4.05984349679059,9.61045552747327,19.1731710962252));
#12367=CARTESIAN_POINT('Ctrl Pts',(-4.11486175771081,9.7007827075446,19.1288726481045));
#12368=CARTESIAN_POINT('Ctrl Pts',(-4.15207724766588,9.76188188091706,19.0989082613083));
#12369=CARTESIAN_POINT('Ctrl Pts',(-4.18921569512279,9.82340116495859,19.0696983544146));
#12370=CARTESIAN_POINT('Ctrl Pts',(-4.2263084128575,9.88532296597213,19.0411707518213));
#12371=CARTESIAN_POINT('Ctrl Pts',(-4.27111143173269,9.96011618116432,19.0067132411425));
#12372=CARTESIAN_POINT('Ctrl Pts',(-4.31584768219754,10.0354996811099,18.9732530327533));
#12373=CARTESIAN_POINT('Ctrl Pts',(-4.36057769144337,10.111478019192,18.940692114664));
#12374=CARTESIAN_POINT('Ctrl Pts',(-4.42892061974248,10.2275652322147,18.8909423263709));
#12375=CARTESIAN_POINT('Ctrl Pts',(-4.49710627109395,10.3447938290632,18.8433951049612));
#12376=CARTESIAN_POINT('Ctrl Pts',(-4.56524407243742,10.4630236268316,18.7977890095272));
#12377=CARTESIAN_POINT('Ctrl Pts',(-4.6012713099202,10.5255365479672,18.7736752048774));
#12378=CARTESIAN_POINT('Ctrl Pts',(-4.63728521548576,10.5883301347704,18.7501046160461));
#12379=CARTESIAN_POINT('Ctrl Pts',(-4.67330231315613,10.6513883422586,18.7270419929154));
#12380=CARTESIAN_POINT('Ctrl Pts',(-4.74222702829795,10.7720607248103,18.6829078224097));
#12381=CARTESIAN_POINT('Ctrl Pts',(-4.81115906209138,10.8936995222528,18.6406488353005));
#12382=CARTESIAN_POINT('Ctrl Pts',(-4.88008076708229,11.0159833665814,18.600143147662));
#12383=CARTESIAN_POINT('Ctrl Pts',(-4.95506354104002,11.149021019367,18.5560753344731));
#12384=CARTESIAN_POINT('Ctrl Pts',(-5.03003423681176,11.2828228206758,18.5140824431372));
#12385=CARTESIAN_POINT('Ctrl Pts',(-5.10498353721246,11.4170275976618,18.4740347519827));
#12386=CARTESIAN_POINT('Ctrl Pts',(-5.11363857299637,11.4325253693685,18.469410103078));
#12387=CARTESIAN_POINT('Ctrl Pts',(-5.12229333534976,11.4480285606925,18.4648114245623));
#12388=CARTESIAN_POINT('Ctrl Pts',(-5.1309478185836,11.4635366486365,18.4602385405353));
#12389=CARTESIAN_POINT('Ctrl Pts',(-5.15787112219279,11.5117808879322,18.4460127177216));
#12390=CARTESIAN_POINT('Ctrl Pts',(-5.18480476071166,11.5600961433554,18.4320245655294));
#12391=CARTESIAN_POINT('Ctrl Pts',(-5.21175836363394,11.6084844905159,18.4182667149329));
#12392=CARTESIAN_POINT('Ctrl Pts',(-5.31258723548669,11.7894971168827,18.3668009217045));
#12393=CARTESIAN_POINT('Ctrl Pts',(-5.41362677762227,11.9714205665464,18.3185921383772));
#12394=CARTESIAN_POINT('Ctrl Pts',(-5.5150898962066,12.1538289711062,18.2734105472006));
#12395=CARTESIAN_POINT('Ctrl Pts',(-5.55642235325627,12.2281356517223,18.2550051778132));
#12396=CARTESIAN_POINT('Ctrl Pts',(-5.59782488816878,12.3025233025885,18.2371024570184));
#12397=CARTESIAN_POINT('Ctrl Pts',(-5.6393109798215,12.3769650887378,18.2196880081847));
#12398=CARTESIAN_POINT('Ctrl Pts',(-5.71720894883317,12.5167435956931,18.1869890929205));
#12399=CARTESIAN_POINT('Ctrl Pts',(-5.79563339295387,12.6571275036336,18.1559192636753));
#12400=CARTESIAN_POINT('Ctrl Pts',(-5.87434573391953,12.7973698711455,18.1265260513586));
#12401=CARTESIAN_POINT('Ctrl Pts',(-5.94045812878175,12.915162820302,18.1018379829425));
#12402=CARTESIAN_POINT('Ctrl Pts',(-6.00677355328274,13.0328551936566,18.0783316338689));
#12403=CARTESIAN_POINT('Ctrl Pts',(-6.07314264709777,13.15,18.0560083736135));
#12404=CARTESIAN_POINT('Origin',(-16.8005208252602,25.4,19.05));
#12405=CARTESIAN_POINT('',(-15.7517039698567,-21.9,12.7872144213759));
#12406=CARTESIAN_POINT('Origin',(-16.8005208252602,-21.9,19.05));
#12407=CARTESIAN_POINT('Ctrl Pts',(-15.7517039698567,-21.9,12.7872144213759));
#12408=CARTESIAN_POINT('Ctrl Pts',(-15.6577766387567,-21.9000000083571,
12.8029442538608));
#12409=CARTESIAN_POINT('Ctrl Pts',(-15.5653228653555,-21.9054435048675,
12.8205709182498));
#12410=CARTESIAN_POINT('Ctrl Pts',(-15.4741566469411,-21.9155046710518,
12.8400273794258));
#12411=CARTESIAN_POINT('Ctrl Pts',(-15.3788825965547,-21.9260191803806,
12.8603605235955));
#12412=CARTESIAN_POINT('Ctrl Pts',(-15.2850148000878,-21.9415773497208,
12.8826920382101));
#12413=CARTESIAN_POINT('Ctrl Pts',(-15.192351675936,-21.9612924551078,12.9069597851924));
#12414=CARTESIAN_POINT('Ctrl Pts',(-15.0919530360919,-21.9826533770858,
12.9332534031922));
#12415=CARTESIAN_POINT('Ctrl Pts',(-14.9929686181069,-22.008894721178,12.961819870374));
#12416=CARTESIAN_POINT('Ctrl Pts',(-14.895153818191,-22.0389456239473,12.9925982857732));
#12417=CARTESIAN_POINT('Ctrl Pts',(-14.8766466516217,-22.0446314410586,
12.9984217527846));
#12418=CARTESIAN_POINT('Ctrl Pts',(-14.8581813868158,-22.0504537744583,
13.0043244573537));
#12419=CARTESIAN_POINT('Ctrl Pts',(-14.839756407874,-22.0564055499457,13.0103060589621));
#12420=CARTESIAN_POINT('Ctrl Pts',(-14.8345259500896,-22.0580951318186,
13.0120041078334));
#12421=CARTESIAN_POINT('Ctrl Pts',(-14.8293013868339,-22.0597946861619,
13.0137076773778));
#12422=CARTESIAN_POINT('Ctrl Pts',(-14.8240826839043,-22.0615041254602,
13.0154167552805));
#12423=CARTESIAN_POINT('Ctrl Pts',(-14.7228347907064,-22.0946689041117,
13.0485745225054));
#12424=CARTESIAN_POINT('Ctrl Pts',(-14.6241194589298,-22.1314339084946,
13.0836965866196));
#12425=CARTESIAN_POINT('Ctrl Pts',(-14.5276787480026,-22.1711120177115,
13.1206542613819));
#12426=CARTESIAN_POINT('Ctrl Pts',(-14.423784232686,-22.213856807605,13.1604683572107));
#12427=CARTESIAN_POINT('Ctrl Pts',(-14.3225295566706,-22.259982703488,13.2024126657374));
#12428=CARTESIAN_POINT('Ctrl Pts',(-14.2236159096512,-22.3086850460529,
13.2463478400349));
#12429=CARTESIAN_POINT('Ctrl Pts',(-14.1514528009381,-22.3442161638206,
13.2784010385034));
#12430=CARTESIAN_POINT('Ctrl Pts',(-14.0805362301013,-22.3811198321414,
13.3115143518381));
#12431=CARTESIAN_POINT('Ctrl Pts',(-14.0107570059122,-22.4190978671501,
13.3456404536346));
#12432=CARTESIAN_POINT('Ctrl Pts',(-14.0051868812153,-22.4221294627747,
13.348364568794));
#12433=CARTESIAN_POINT('Ctrl Pts',(-13.9996232086063,-22.4251683970665,
13.351095517512));
#12434=CARTESIAN_POINT('Ctrl Pts',(-13.9940659665539,-22.4282145883132,
13.3538332913571));
#12435=CARTESIAN_POINT('Ctrl Pts',(-13.8353383484615,-22.5152208184325,
13.4320304109373));
#12436=CARTESIAN_POINT('Ctrl Pts',(-13.6817400381253,-22.6081793607658,
13.5158520921216));
#12437=CARTESIAN_POINT('Ctrl Pts',(-13.5331922899877,-22.7050300063637,
13.6049382184845));
#12438=CARTESIAN_POINT('Ctrl Pts',(-13.3831027231072,-22.8028858919771,
13.6949489947399));
#12439=CARTESIAN_POINT('Ctrl Pts',(-13.2381692424498,-22.904715210645,13.7903339482295));
#12440=CARTESIAN_POINT('Ctrl Pts',(-13.098312889361,-23.0084452538252,13.890732869345));
#12441=CARTESIAN_POINT('Ctrl Pts',(-12.9560181195809,-23.1139838460137,
13.9928822608513));
#12442=CARTESIAN_POINT('Ctrl Pts',(-12.8189790827752,-23.2214901219724,
14.1002219147977));
#12443=CARTESIAN_POINT('Ctrl Pts',(-12.687113670909,-23.3288332609408,14.2123853779174));
#12444=CARTESIAN_POINT('Ctrl Pts',(-12.6579532757914,-23.3525708605219,
14.2371889322083));
#12445=CARTESIAN_POINT('Ctrl Pts',(-12.6290458846788,-23.3763006781133,
14.2622284310387));
#12446=CARTESIAN_POINT('Ctrl Pts',(-12.6003906189451,-23.4,14.2875));
#12447=CARTESIAN_POINT('Ctrl Pts',(-12.6003906189451,13.15,14.2875));
#12448=CARTESIAN_POINT('Ctrl Pts',(-12.6805660239936,12.9711603489454,14.2167919389926));
#12449=CARTESIAN_POINT('Ctrl Pts',(-12.7625477505346,12.7922384038523,14.1480629070756));
#12450=CARTESIAN_POINT('Ctrl Pts',(-12.8465546744841,12.6135684732185,14.081202835174));
#12451=CARTESIAN_POINT('Ctrl Pts',(-12.9256696150891,12.4453030459724,14.0182362323196));
#12452=CARTESIAN_POINT('Ctrl Pts',(-13.0065809833159,12.2772593411672,13.9569274305183));
#12453=CARTESIAN_POINT('Ctrl Pts',(-13.0895011854204,12.1097298658262,13.8972149709292));
#12454=CARTESIAN_POINT('Ctrl Pts',(-13.1664953235755,11.95417323135,13.8417699859134));
#12455=CARTESIAN_POINT('Ctrl Pts',(-13.2452216484674,11.7990589433282,13.787701522798));
#12456=CARTESIAN_POINT('Ctrl Pts',(-13.3258732912857,11.6446516999771,13.7349847981691));
#12457=CARTESIAN_POINT('Ctrl Pts',(-13.3320808650622,11.6327673251369,13.7309273116015));
#12458=CARTESIAN_POINT('Ctrl Pts',(-13.3382998557066,11.620887159043,13.7268778447985));
#12459=CARTESIAN_POINT('Ctrl Pts',(-13.34453035693,11.6090113330868,13.7228363925281));
#12460=CARTESIAN_POINT('Ctrl Pts',(-13.3701748672856,11.5601308769568,13.7062019259122));
#12461=CARTESIAN_POINT('Ctrl Pts',(-13.3960120894246,11.5113297193656,13.6897046928704));
#12462=CARTESIAN_POINT('Ctrl Pts',(-13.4220479527771,11.4626185033485,13.673344808347));
#12463=CARTESIAN_POINT('Ctrl Pts',(-13.5007574197068,11.3153587872303,13.62388695967));
#12464=CARTESIAN_POINT('Ctrl Pts',(-13.5812593458259,11.1688712790712,13.5756551364999));
#12465=CARTESIAN_POINT('Ctrl Pts',(-13.6638980075716,11.0233411942463,13.528670711557));
#12466=CARTESIAN_POINT('Ctrl Pts',(-13.7433621196739,10.8834016220112,13.4834911850273));
#12467=CARTESIAN_POINT('Ctrl Pts',(-13.8248017421929,10.7443469553863,13.4394651524236));
#12468=CARTESIAN_POINT('Ctrl Pts',(-13.9085483061395,10.6063775973624,13.3966301736711));
#12469=CARTESIAN_POINT('Ctrl Pts',(-13.9882575070387,10.4750596452175,13.3558602391689));
#12470=CARTESIAN_POINT('Ctrl Pts',(-14.0700564394539,10.3447246751962,13.3161693909074));
#12471=CARTESIAN_POINT('Ctrl Pts',(-14.1542566954101,10.2155824310125,13.2776057275986));
#12472=CARTESIAN_POINT('Ctrl Pts',(-14.1759224559351,10.1823525446615,13.2676828231522));
#12473=CARTESIAN_POINT('Ctrl Pts',(-14.1977473522222,10.1492018356285,13.257834629348));
#12474=CARTESIAN_POINT('Ctrl Pts',(-14.2197370070741,10.1161343255489,13.2480621331828));
#12475=CARTESIAN_POINT('Ctrl Pts',(-14.2697134783846,10.0409809190981,13.2258519221759));
#12476=CARTESIAN_POINT('Ctrl Pts',(-14.3205483943213,9.96626705526651,13.2040289854677));
#12477=CARTESIAN_POINT('Ctrl Pts',(-14.3723283486023,9.89202045142466,13.1826001246522));
#12478=CARTESIAN_POINT('Ctrl Pts',(-14.4424863663332,9.79142178112592,13.1535655992665));
#12479=CARTESIAN_POINT('Ctrl Pts',(-14.5143906000105,9.69169193895732,13.1252666892286));
#12480=CARTESIAN_POINT('Ctrl Pts',(-14.5883378176581,9.59300570027429,13.0977807866605));
#12481=CARTESIAN_POINT('Ctrl Pts',(-14.635359051831,9.53025352532599,13.0803031708391));
#12482=CARTESIAN_POINT('Ctrl Pts',(-14.683206840735,9.46792401681048,13.063154611628));
#12483=CARTESIAN_POINT('Ctrl Pts',(-14.7319636287996,9.40607058542615,13.0463587156065));
#12484=CARTESIAN_POINT('Ctrl Pts',(-14.7902864685227,9.33208154906526,13.0262674751751));
#12485=CARTESIAN_POINT('Ctrl Pts',(-14.8499317227244,9.25875668204221,13.0066727912773));
#12486=CARTESIAN_POINT('Ctrl Pts',(-14.9110746531334,9.18618721050011,12.9876165443994));
#12487=CARTESIAN_POINT('Ctrl Pts',(-14.976144264209,9.10895723055615,12.9673364798914));
#12488=CARTESIAN_POINT('Ctrl Pts',(-15.0425927400042,9.03297713418422,12.9477720512664));
#12489=CARTESIAN_POINT('Ctrl Pts',(-15.1105485368423,8.95848778473299,12.9290087698698));
#12490=CARTESIAN_POINT('Ctrl Pts',(-15.1780277686271,8.88452081927902,12.9103770728945));
#12491=CARTESIAN_POINT('Ctrl Pts',(-15.2469932190871,8.81202334049308,12.892535211434));
#12492=CARTESIAN_POINT('Ctrl Pts',(-15.3175799579227,8.74127840230462,12.8755833064032));
#12493=CARTESIAN_POINT('Ctrl Pts',(-15.3761704880966,8.68255655874077,12.8615123758064));
#12494=CARTESIAN_POINT('Ctrl Pts',(-15.4358982963745,8.62503122998396,12.8480495581956));
#12495=CARTESIAN_POINT('Ctrl Pts',(-15.496892027902,8.56885520307108,12.8352552780477));
#12496=CARTESIAN_POINT('Ctrl Pts',(-15.5571381099264,8.51336777115895,12.8226178277404));
#12497=CARTESIAN_POINT('Ctrl Pts',(-15.6186470139557,8.45914957374164,12.8106203083913));
#12498=CARTESIAN_POINT('Ctrl Pts',(-15.6816035368458,8.40640557244853,12.7993457937111));
#12499=CARTESIAN_POINT('Ctrl Pts',(-15.7419197422832,8.35587358828636,12.7885441180079));
#12500=CARTESIAN_POINT('Ctrl Pts',(-15.8035646398897,8.30669462478942,12.7784060513894));
#12501=CARTESIAN_POINT('Ctrl Pts',(-15.8667156307491,8.25909114269656,12.7690197747266));
#12502=CARTESIAN_POINT('Ctrl Pts',(-15.9083560624209,8.22770241044624,12.762830661829));
#12503=CARTESIAN_POINT('Ctrl Pts',(-15.9506516151452,8.19699952044147,12.7569687178741));
#12504=CARTESIAN_POINT('Ctrl Pts',(-15.9936571257441,8.1670574358422,12.7514631752544));
#12505=CARTESIAN_POINT('Ctrl Pts',(-16.0374647365421,8.13655689834508,12.7458549481933));
#12506=CARTESIAN_POINT('Ctrl Pts',(-16.0819818772239,8.10686980879577,12.7406197777735));
#12507=CARTESIAN_POINT('Ctrl Pts',(-16.1272992232855,8.07806532466692,12.7357880400415));
#12508=CARTESIAN_POINT('Ctrl Pts',(-16.1796232807136,8.04480725435319,12.7302092463888));
#12509=CARTESIAN_POINT('Ctrl Pts',(-16.2330200573025,8.01279246823339,12.7251928706675));
#12510=CARTESIAN_POINT('Ctrl Pts',(-16.2874537728527,7.98223072788154,12.7207964614722));
#12511=CARTESIAN_POINT('Ctrl Pts',(-16.3401547757431,7.95264181684838,12.7165399970481));
#12512=CARTESIAN_POINT('Ctrl Pts',(-16.3938280311525,7.92441470275639,12.7128646355283));
#12513=CARTESIAN_POINT('Ctrl Pts',(-16.44842648929,7.89778233069164,12.7098341952403));
#12514=CARTESIAN_POINT('Ctrl Pts',(-16.5013769362388,7.87195383567105,12.7068952263907));
#12515=CARTESIAN_POINT('Ctrl Pts',(-16.5551978274457,7.84762505829446,12.7045628094629));
#12516=CARTESIAN_POINT('Ctrl Pts',(-16.6098284934653,7.82505223561866,12.7029065797752));
#12517=CARTESIAN_POINT('Ctrl Pts',(-16.6623029207626,7.80337034834364,12.7013157204526));
#12518=CARTESIAN_POINT('Ctrl Pts',(-16.7155246478195,7.78330843075896,12.7003487212281));
#12519=CARTESIAN_POINT('Ctrl Pts',(-16.7694201971022,7.76513667664443,12.7000781600543));
#12520=CARTESIAN_POINT('Ctrl Pts',(-16.7797625308285,7.76164959194177,12.7000262404804));
#12521=CARTESIAN_POINT('Ctrl Pts',(-16.7901296121603,7.75823224576275,12.7));
#12522=CARTESIAN_POINT('Ctrl Pts',(-16.8005208252602,7.75488674445212,12.7));
#12523=CARTESIAN_POINT('Origin',(0.,-23.4,0.));
#12524=CARTESIAN_POINT('Ctrl Pts',(-6.07314264709753,-23.4,-18.0560083736136));
#12525=CARTESIAN_POINT('Ctrl Pts',(-5.88858797454276,-23.3670436986155,
-18.1180833809697));
#12526=CARTESIAN_POINT('Ctrl Pts',(-5.70415854699224,-23.3340202714534,
-18.1802846951814));
#12527=CARTESIAN_POINT('Ctrl Pts',(-5.51977350812678,-23.3013555121265,
-18.2428536513247));
#12528=CARTESIAN_POINT('Ctrl Pts',(-5.37004319496178,-23.2748300159497,
-18.2936629222688));
#12529=CARTESIAN_POINT('Ctrl Pts',(-5.22034041400646,-23.2485394306939,
-18.3447134083939));
#12530=CARTESIAN_POINT('Ctrl Pts',(-5.07065077098291,-23.2227118266261,
-18.3961284339486));
#12531=CARTESIAN_POINT('Ctrl Pts',(-4.93247587122431,-23.1988709881352,
-18.4435884041817));
#12532=CARTESIAN_POINT('Ctrl Pts',(-4.79431122189726,-23.175423671515,-18.4913586401195));
#12533=CARTESIAN_POINT('Ctrl Pts',(-4.65618933923002,-23.1525653653545,
-18.5395394451827));
#12534=CARTESIAN_POINT('Ctrl Pts',(-4.53506332264139,-23.1325197685401,
-18.5817916132));
#12535=CARTESIAN_POINT('Ctrl Pts',(-4.41397019874696,-23.1129267585465,
-18.6243594808228));
#12536=CARTESIAN_POINT('Ctrl Pts',(-4.2929717674843,-23.0939393203888,-18.6673155065398));
#12537=CARTESIAN_POINT('Ctrl Pts',(-4.27599380361344,-23.0912750871779,
-18.67334290578));
#12538=CARTESIAN_POINT('Ctrl Pts',(-4.25901777583649,-23.0886228201603,
-18.6793779562881));
#12539=CARTESIAN_POINT('Ctrl Pts',(-4.24204392806113,-23.0859829876026,
-18.6854208674118));
#12540=CARTESIAN_POINT('Ctrl Pts',(-4.21403849285808,-23.0816274837345,
-18.6953911674966));
#12541=CARTESIAN_POINT('Ctrl Pts',(-4.18604700646962,-23.0773075842939,
-18.7053795884347));
#12542=CARTESIAN_POINT('Ctrl Pts',(-4.15807096333259,-23.0730255541513,
-18.7153867564022));
#12543=CARTESIAN_POINT('Ctrl Pts',(-4.04200724753667,-23.0552607713668,
-18.7569033173116));
#12544=CARTESIAN_POINT('Ctrl Pts',(-3.92593006481832,-23.0380976121148,
-18.7988741217285));
#12545=CARTESIAN_POINT('Ctrl Pts',(-3.80990120850084,-23.0218415529602,
-18.8414809578007));
#12546=CARTESIAN_POINT('Ctrl Pts',(-3.70072977930051,-23.0065462439535,
-18.8815696851685));
#12547=CARTESIAN_POINT('Ctrl Pts',(-3.59160104576938,-22.9920537993331,
-18.9222214064209));
#12548=CARTESIAN_POINT('Ctrl Pts',(-3.48259310512416,-22.9786542884005,
-18.963599792128));
#12549=CARTESIAN_POINT('Ctrl Pts',(-3.43157384280193,-22.9723828813891,
-18.982966222705));
#12550=CARTESIAN_POINT('Ctrl Pts',(-3.38058144102074,-22.9663514277305,
-19.0024920199359));
#12551=CARTESIAN_POINT('Ctrl Pts',(-3.32962618541098,-22.9605927752761,
-19.0221950481898));
#12552=CARTESIAN_POINT('Ctrl Pts',(-3.30407684920651,-22.9577053450026,
-19.0320742900282));
#12553=CARTESIAN_POINT('Ctrl Pts',(-3.27849980805422,-22.9548823672324,
-19.0420123529479));
#12554=CARTESIAN_POINT('Ctrl Pts',(-3.2528923075186,-22.9521283805007,-19.052013666249));
#12555=CARTESIAN_POINT('Ctrl Pts',(-3.17837177385048,-22.9441139879725,
-19.0811185452486));
#12556=CARTESIAN_POINT('Ctrl Pts',(-3.10413037938078,-22.9367118504462,
-19.1105498162239));
#12557=CARTESIAN_POINT('Ctrl Pts',(-3.03010916781498,-22.9301299080702,
-19.1404318150206));
#12558=CARTESIAN_POINT('Ctrl Pts',(-2.95870293024803,-22.9237804883428,
-19.1692581616841));
#12559=CARTESIAN_POINT('Ctrl Pts',(-2.88750160968762,-22.9181939831414,
-19.1985038155338));
#12560=CARTESIAN_POINT('Ctrl Pts',(-2.81647463478462,-22.9135965970107,
-19.2282900937695));
#12561=CARTESIAN_POINT('Ctrl Pts',(-2.74923181322827,-22.9092441490057,
-19.2564894278248));
#12562=CARTESIAN_POINT('Ctrl Pts',(-2.68214533086182,-22.9057780702214,
-19.2851732366577));
#12563=CARTESIAN_POINT('Ctrl Pts',(-2.61520888367674,-22.903429789029,-19.3144547693357));
#12564=CARTESIAN_POINT('Ctrl Pts',(-2.55222036166138,-22.9012200099355,
-19.3420092713043));
#12565=CARTESIAN_POINT('Ctrl Pts',(-2.48936478214343,-22.9,-19.3700930276043));
#12566=CARTESIAN_POINT('Ctrl Pts',(-2.42665362134758,-22.9,-19.3988105873015));
#12567=CARTESIAN_POINT('Ctrl Pts',(18.0131895824795,-22.9,-7.59786161137808));
#12568=CARTESIAN_POINT('Ctrl Pts',(18.0202404656926,-22.9,-7.52320647355465));
#12569=CARTESIAN_POINT('Ctrl Pts',(18.028025155963,-22.9014413252167,-7.44877824034678));
#12570=CARTESIAN_POINT('Ctrl Pts',(18.0364209165634,-22.9040302787143,-7.37452199635976));
#12571=CARTESIAN_POINT('Ctrl Pts',(18.0449193548697,-22.9066508943588,-7.2993576201457));
#12572=CARTESIAN_POINT('Ctrl Pts',(18.0540441011123,-22.9104479219793,-7.22436948480864));
#12573=CARTESIAN_POINT('Ctrl Pts',(18.063691899772,-22.9151689742966,-7.14948735848897));
#12574=CARTESIAN_POINT('Ctrl Pts',(18.0738958528035,-22.9201621751089,-7.07028859752707));
#12575=CARTESIAN_POINT('Ctrl Pts',(18.0846849419657,-22.9261892251373,-6.99120855793443));
#12576=CARTESIAN_POINT('Ctrl Pts',(18.0959620640515,-22.9330040852343,-6.91214802540154));
#12577=CARTESIAN_POINT('Ctrl Pts',(18.1056234232792,-22.9388425261932,-6.844415123362));
#12578=CARTESIAN_POINT('Ctrl Pts',(18.1156434929245,-22.9452603057859,-6.77669626729572));
#12579=CARTESIAN_POINT('Ctrl Pts',(18.1259739820853,-22.9521283804573,-6.70891945900388));
#12580=CARTESIAN_POINT('Ctrl Pts',(18.1301164636466,-22.9548824487541,-6.68174125144072));
#12581=CARTESIAN_POINT('Ctrl Pts',(18.1342984943433,-22.9577055122081,-6.65462105077966));
#12582=CARTESIAN_POINT('Ctrl Pts',(18.1385176153026,-22.960593031896,-6.62755425650044));
#12583=CARTESIAN_POINT('Ctrl Pts',(18.1564082194725,-22.9728371633794,-6.51278122504063));
#12584=CARTESIAN_POINT('Ctrl Pts',(18.175074850113,-22.9863118482887,-6.39826461568774));
#12585=CARTESIAN_POINT('Ctrl Pts',(18.1943268007347,-23.0007124806144,-6.28399909928586));
#12586=CARTESIAN_POINT('Ctrl Pts',(18.2147324024488,-23.0159760543397,-6.16288635267795));
#12587=CARTESIAN_POINT('Ctrl Pts',(18.235795699568,-23.032280074281,-6.04205565211729));
#12588=CARTESIAN_POINT('Ctrl Pts',(18.2573203896198,-23.0493077902555,-5.92147920377189));
#12589=CARTESIAN_POINT('Ctrl Pts',(18.2671348228347,-23.0570717757452,-5.86650096730342));
#12590=CARTESIAN_POINT('Ctrl Pts',(18.2770455748766,-23.0649868063112,-5.81157531072592));
#12591=CARTESIAN_POINT('Ctrl Pts',(18.2870358543848,-23.0730255541295,-5.75669829320565));
#12592=CARTESIAN_POINT('Ctrl Pts',(18.2923577031983,-23.0773078167532,-5.72746515810246));
#12593=CARTESIAN_POINT('Ctrl Pts',(18.2977035116034,-23.0816279527548,-5.69822802204645));
#12594=CARTESIAN_POINT('Ctrl Pts',(18.3030719898805,-23.0859836968892,-5.66898786636628));
#12595=CARTESIAN_POINT('Ctrl Pts',(18.326479713442,-23.1049756810869,-5.54149447890509));
#12596=CARTESIAN_POINT('Ctrl Pts',(18.3502967025003,-23.1246111362575,-5.41409447936928));
#12597=CARTESIAN_POINT('Ctrl Pts',(18.3744213032108,-23.1447278442602,-5.28681965750206));
#12598=CARTESIAN_POINT('Ctrl Pts',(18.4018259099811,-23.1675796410191,-5.14224041712917));
#12599=CARTESIAN_POINT('Ctrl Pts',(18.4296274978877,-23.1910529746929,-4.99782274608269));
#12600=CARTESIAN_POINT('Ctrl Pts',(18.4577147532105,-23.214943810437,-4.85356339888911));
#12601=CARTESIAN_POINT('Ctrl Pts',(18.4890884148577,-23.2416300419142,-4.69242469393962));
#12602=CARTESIAN_POINT('Ctrl Pts',(18.5208193133129,-23.2688383567222,-4.53148298254906));
#12603=CARTESIAN_POINT('Ctrl Pts',(18.5527900614526,-23.296309683901,-4.37067927495082));
#12604=CARTESIAN_POINT('Ctrl Pts',(18.5927280414385,-23.3306269701359,-4.16980267276329));
#12605=CARTESIAN_POINT('Ctrl Pts',(18.6330437593144,-23.3653575842487,-3.96914004956012));
#12606=CARTESIAN_POINT('Ctrl Pts',(18.6735332660427,-23.4,-3.76850837361349));
#12607=CARTESIAN_POINT('Origin',(0.,13.15,0.));
#12608=CARTESIAN_POINT('',(1.82293408768446,12.6595351585866,19.3672161093864));
#12609=CARTESIAN_POINT('Ctrl Pts',(-6.07314264709777,13.15,18.0560083736135));
#12610=CARTESIAN_POINT('Ctrl Pts',(-5.89143659083433,13.1379692270487,18.1171252482126));
#12611=CARTESIAN_POINT('Ctrl Pts',(-5.70926339248799,13.1259554920724,18.1757473227728));
#12612=CARTESIAN_POINT('Ctrl Pts',(-5.52650317309585,13.1139455296796,18.2320030637526));
#12613=CARTESIAN_POINT('Ctrl Pts',(-5.34710195439919,13.1021563017123,18.2872248648864));
#12614=CARTESIAN_POINT('Ctrl Pts',(-5.16713396323832,13.0903706662046,18.3401664122538));
#12615=CARTESIAN_POINT('Ctrl Pts',(-4.98648886991423,13.0785760987252,18.3909003151281));
#12616=CARTESIAN_POINT('Ctrl Pts',(-4.81108595020798,13.0671237999969,18.4401619614231));
#12617=CARTESIAN_POINT('Ctrl Pts',(-4.63504371157761,13.0556630399472,18.4873420908706));
#12618=CARTESIAN_POINT('Ctrl Pts',(-4.45827906291381,13.0441829768623,18.5324625404846));
#12619=CARTESIAN_POINT('Ctrl Pts',(-4.29057738820271,13.0332915128753,18.5752696007265));
#12620=CARTESIAN_POINT('Ctrl Pts',(-4.12222485300671,13.0223826439246,18.616222526144));
#12621=CARTESIAN_POINT('Ctrl Pts',(-3.95317780433264,13.0114481775481,18.6553021950897));
#12622=CARTESIAN_POINT('Ctrl Pts',(-3.87704203806503,13.0065234895229,18.6729029788005));
#12623=CARTESIAN_POINT('Ctrl Pts',(-3.80076582857587,13.0015936267076,18.6901232797613));
#12624=CARTESIAN_POINT('Ctrl Pts',(-3.72434765372577,12.996657942793,18.7069588323863));
#12625=CARTESIAN_POINT('Ctrl Pts',(-3.58036899032601,12.987358673681,18.7386785164706));
#12626=CARTESIAN_POINT('Ctrl Pts',(-3.43573644023662,12.9780292666602,18.7690854619261));
#12627=CARTESIAN_POINT('Ctrl Pts',(-3.29066907106318,12.9686821009665,18.798166713184));
#12628=CARTESIAN_POINT('Ctrl Pts',(-3.15493537978566,12.9599363347077,18.825376868043));
#12629=CARTESIAN_POINT('Ctrl Pts',(-3.01882077394898,12.9511750020393,18.8514262764423));
#12630=CARTESIAN_POINT('Ctrl Pts',(-2.88254718378542,12.9424107435028,18.8762907389895));
#12631=CARTESIAN_POINT('Ctrl Pts',(-2.78114456358843,12.9358891660011,18.8947926486335));
#12632=CARTESIAN_POINT('Ctrl Pts',(-2.67965469546404,12.9293660137815,18.9126381832964));
#12633=CARTESIAN_POINT('Ctrl Pts',(-2.57818729839884,12.9228475964189,18.929812644131));
#12634=CARTESIAN_POINT('Ctrl Pts',(-2.44377209138411,12.9142125624618,18.9525638802443));
#12635=CARTESIAN_POINT('Ctrl Pts',(-2.30940063942545,12.9055857664759,18.9741477153703));
#12636=CARTESIAN_POINT('Ctrl Pts',(-2.17514817924979,12.8969734463819,18.9946057570328));
#12637=CARTESIAN_POINT('Ctrl Pts',(-2.05167325408668,12.8890525071477,19.0134214655863));
#12638=CARTESIAN_POINT('Ctrl Pts',(-1.92817267861986,12.8811371827706,19.0313039403008));
#12639=CARTESIAN_POINT('Ctrl Pts',(-1.80456225428477,12.8732239828736,19.0482998974936));
#12640=CARTESIAN_POINT('Ctrl Pts',(-1.70031647335247,12.8665504542666,19.062633290812));
#12641=CARTESIAN_POINT('Ctrl Pts',(-1.59599311213552,12.8598784744128,19.0763358597885));
#12642=CARTESIAN_POINT('Ctrl Pts',(-1.49156999562427,12.8532079839211,19.0894300738828));
#12643=CARTESIAN_POINT('Ctrl Pts',(-1.37302337322002,12.8456352917434,19.1042953154669));
#12644=CARTESIAN_POINT('Ctrl Pts',(-1.25434655584515,12.83806400913,19.1183773452858));
#12645=CARTESIAN_POINT('Ctrl Pts',(-1.13553246318378,12.8305004633234,19.1317219358192));
#12646=CARTESIAN_POINT('Ctrl Pts',(-1.02214813267873,12.8232825688942,19.1444566832688));
#12647=CARTESIAN_POINT('Ctrl Pts',(-0.908638694765087,12.8160717028953,
19.1565195853913));
#12648=CARTESIAN_POINT('Ctrl Pts',(-0.79504399785826,12.8088775452768,19.1679520323113));
#12649=CARTESIAN_POINT('Ctrl Pts',(-0.692063351944374,12.8023555947057,
19.1783162552922));
#12650=CARTESIAN_POINT('Ctrl Pts',(-0.58901291751484,12.795847396274,19.1881621901356));
#12651=CARTESIAN_POINT('Ctrl Pts',(-0.485959105372368,12.7893635951272,
19.1975247440753));
#12652=CARTESIAN_POINT('Ctrl Pts',(-0.397291306545851,12.7837849138173,
19.2055803126366));
#12653=CARTESIAN_POINT('Ctrl Pts',(-0.308450767230545,12.7782136874732,
19.2132892091623));
#12654=CARTESIAN_POINT('Ctrl Pts',(-0.219666931641276,12.7726724740284,
19.2206736432458));
#12655=CARTESIAN_POINT('Ctrl Pts',(-0.207021284979042,12.7718832287019,
19.2217254219124));
#12656=CARTESIAN_POINT('Ctrl Pts',(-0.194376874651241,12.7710945998699,
19.2227706248721));
#12657=CARTESIAN_POINT('Ctrl Pts',(-0.181734451453492,12.7703066605067,
19.2238093232609));
#12658=CARTESIAN_POINT('Ctrl Pts',(-0.112648562634309,12.7660008806426,
19.22948540294));
#12659=CARTESIAN_POINT('Ctrl Pts',(-0.0436037693110482,12.7617151304109,
19.2349679902415));
#12660=CARTESIAN_POINT('Ctrl Pts',(0.02547635923879,12.757449305424,19.2402849388918));
#12661=CARTESIAN_POINT('Ctrl Pts',(0.0916269448846765,12.7533643850993,
19.245376406937));
#12662=CARTESIAN_POINT('Ctrl Pts',(0.157810333253506,12.749297698185,19.250315856965));
#12663=CARTESIAN_POINT('Ctrl Pts',(0.224046235742999,12.7452532521653,19.2551251194837));
#12664=CARTESIAN_POINT('Ctrl Pts',(0.286785346628499,12.74142232456,19.2596804866349));
#12665=CARTESIAN_POINT('Ctrl Pts',(0.34957181954994,12.7376113278546,19.2641189432598));
#12666=CARTESIAN_POINT('Ctrl Pts',(0.412374550348153,12.7338278436746,19.2684582922758));
#12667=CARTESIAN_POINT('Ctrl Pts',(0.415874887835622,12.7336169695399,19.2687001477786));
#12668=CARTESIAN_POINT('Ctrl Pts',(0.419375262237528,12.7334061820621,19.2689416954471));
#12669=CARTESIAN_POINT('Ctrl Pts',(0.422875663239959,12.7331954829858,19.2691829383935));
#12670=CARTESIAN_POINT('Ctrl Pts',(0.490997749735726,12.7290950211557,19.273877821308));
#12671=CARTESIAN_POINT('Ctrl Pts',(0.559094103262397,12.7250294339064,19.2784597940843));
#12672=CARTESIAN_POINT('Ctrl Pts',(0.627197583147417,12.72100812477,19.2829652951132));
#12673=CARTESIAN_POINT('Ctrl Pts',(0.691552601732308,12.7172081511909,19.2872228103376));
#12674=CARTESIAN_POINT('Ctrl Pts',(0.7559138409642,12.7134477064408,19.2914118703163));
#12675=CARTESIAN_POINT('Ctrl Pts',(0.820267024024453,12.7097399996136,19.2955695468785));
#12676=CARTESIAN_POINT('Ctrl Pts',(0.874397449907384,12.706621276653,19.2990667601054));
#12677=CARTESIAN_POINT('Ctrl Pts',(0.928336362683676,12.7035507329861,19.3025295407969));
#12678=CARTESIAN_POINT('Ctrl Pts',(0.982238818325173,12.7005283628061,19.3059969894654));
#12679=CARTESIAN_POINT('Ctrl Pts',(1.03466360068771,12.6975888473977,19.3093693820519));
#12680=CARTESIAN_POINT('Ctrl Pts',(1.08705397397595,12.6946948638824,19.3127459826068));
#12681=CARTESIAN_POINT('Ctrl Pts',(1.13950386109632,12.6918520765328,19.3161671454685));
#12682=CARTESIAN_POINT('Ctrl Pts',(1.15856271360277,12.6908190854669,19.3174103023552));
#12683=CARTESIAN_POINT('Ctrl Pts',(1.17762894267694,12.6897929124046,19.3186594013673));
#12684=CARTESIAN_POINT('Ctrl Pts',(1.19670535537073,12.6887740383049,19.3199166147567));
#12685=CARTESIAN_POINT('Ctrl Pts',(1.2486425919455,12.68600006261,19.3233394904449));
#12686=CARTESIAN_POINT('Ctrl Pts',(1.30066077866098,12.6832787578847,19.3268211239109));
#12687=CARTESIAN_POINT('Ctrl Pts',(1.35277970669886,12.6806283209993,19.3304073273177));
#12688=CARTESIAN_POINT('Ctrl Pts',(1.40175117770664,12.6781379437415,19.3337769602472));
#12689=CARTESIAN_POINT('Ctrl Pts',(1.45081143546155,12.6757101114834,19.3372387703585));
#12690=CARTESIAN_POINT('Ctrl Pts',(1.49992966112441,12.6733674903705,19.3408403785556));
#12691=CARTESIAN_POINT('Ctrl Pts',(1.54792459291616,12.6710784430971,19.3443596209025));
#12692=CARTESIAN_POINT('Ctrl Pts',(1.59597502673672,12.6688706813137,19.348012128234));
#12693=CARTESIAN_POINT('Ctrl Pts',(1.64400519519223,12.666773564035,19.3518544508691));
#12694=CARTESIAN_POINT('Ctrl Pts',(1.6904627290876,12.6647451119144,19.3555709657138));
#12695=CARTESIAN_POINT('Ctrl Pts',(1.73690137116093,12.6628201182928,19.3594648742118));
#12696=CARTESIAN_POINT('Ctrl Pts',(1.78320656534742,12.6610338566191,19.3636017376306));
#12697=CARTESIAN_POINT('Ctrl Pts',(1.79646145024437,12.6605225383254,19.3647859168445));
#12698=CARTESIAN_POINT('Ctrl Pts',(1.80970510015646,12.6600226469239,19.3659901067536));
#12699=CARTESIAN_POINT('Ctrl Pts',(1.82293408768446,12.6595351585866,19.3672161093864));
#12700=CARTESIAN_POINT('Ctrl Pts',(1.82293408768446,12.6595351585866,19.3672161093864));
#12701=CARTESIAN_POINT('Ctrl Pts',(1.92899847198764,12.6556266847333,19.3770456765946));
#12702=CARTESIAN_POINT('Ctrl Pts',(2.03513094440902,12.6527974939074,19.3867477665312));
#12703=CARTESIAN_POINT('Ctrl Pts',(2.14128049080422,12.6512766915374,19.3963919419144));
#12704=CARTESIAN_POINT('Ctrl Pts',(2.19967982607374,12.650440005461,19.4016977906035));
#12705=CARTESIAN_POINT('Ctrl Pts',(2.25808442071507,12.65,19.4069865889968));
#12706=CARTESIAN_POINT('Ctrl Pts',(2.31648752866395,12.65,19.4122740947459));
#12707=CARTESIAN_POINT('',(15.8610341074694,12.6595351585866,11.2623152840528));
#12708=CARTESIAN_POINT('Ctrl Pts',(15.6532787469444,12.65,11.7122740947461));
#12709=CARTESIAN_POINT('Ctrl Pts',(15.6980337221155,12.65,11.6155345352022));
#12710=CARTESIAN_POINT('Ctrl Pts',(15.7427862154013,12.6514513272118,11.5187867449086));
#12711=CARTESIAN_POINT('Ctrl Pts',(15.7874388179956,12.6541030519079,11.4220256779294));
#12712=CARTESIAN_POINT('Ctrl Pts',(15.8120049363218,12.6555619272896,11.3687915172607));
#12713=CARTESIAN_POINT('Ctrl Pts',(15.8365411965293,12.6573848688951,11.3155539383097));
#12714=CARTESIAN_POINT('Ctrl Pts',(15.8610341074694,12.6595351585866,11.2623152840528));
#12715=CARTESIAN_POINT('Ctrl Pts',(15.8610341074694,12.6595351585866,11.2623152840528));
#12716=CARTESIAN_POINT('Ctrl Pts',(15.8755315725394,12.6608079247682,11.2308030834822));
#12717=CARTESIAN_POINT('Ctrl Pts',(15.8902824743543,12.6621745127569,11.1991317971907));
#12718=CARTESIAN_POINT('Ctrl Pts',(15.9051841193332,12.6636122851386,11.1674271960182));
#12719=CARTESIAN_POINT('Ctrl Pts',(15.9206585676617,12.6651053239581,11.1345039037699));
#12720=CARTESIAN_POINT('Ctrl Pts',(15.9362957629233,12.6666751553055,11.1015444562721));
#12721=CARTESIAN_POINT('Ctrl Pts',(15.9520132214841,12.6683023351355,11.0686433208445));
#12722=CARTESIAN_POINT('Ctrl Pts',(15.9687080951478,12.6700307037253,11.0336961760989));
#12723=CARTESIAN_POINT('Ctrl Pts',(15.9854936245323,12.6718237880044,10.998814731488));
#12724=CARTESIAN_POINT('Ctrl Pts',(16.0023047914919,12.6736645084142,10.9640631789662));
#12725=CARTESIAN_POINT('Ctrl Pts',(16.0197345727335,12.6755729633208,10.9280328450984));
#12726=CARTESIAN_POINT('Ctrl Pts',(16.0371921625325,12.6775326648007,10.8921418342238));
#12727=CARTESIAN_POINT('Ctrl Pts',(16.0546374221841,12.679530611801,10.856413971676));
#12728=CARTESIAN_POINT('Ctrl Pts',(16.0730820056298,12.6816430079993,10.8186394956717));
#12729=CARTESIAN_POINT('Ctrl Pts',(16.0915129761836,12.6837981812692,10.781047216685));
#12730=CARTESIAN_POINT('Ctrl Pts',(16.1099151779263,12.6859869025207,10.7436165469437));
#12731=CARTESIAN_POINT('Ctrl Pts',(16.1180616880166,12.6869558322178,10.7270462836133));
#12732=CARTESIAN_POINT('Ctrl Pts',(16.1262029523282,12.6879314118327,10.7105070921922));
#12733=CARTESIAN_POINT('Ctrl Pts',(16.1343393771825,12.6889131739459,10.6939945272582));
#12734=CARTESIAN_POINT('Ctrl Pts',(16.1554826056401,12.6914643706966,10.6510851488677));
#12735=CARTESIAN_POINT('Ctrl Pts',(16.1765726356144,12.6940529314347,10.6083837729401));
#12736=CARTESIAN_POINT('Ctrl Pts',(16.1976696182531,12.69667992237,10.5657060705175));
#12737=CARTESIAN_POINT('Ctrl Pts',(16.2193768925724,12.6993829066707,10.5217937912274));
#12738=CARTESIAN_POINT('Ctrl Pts',(16.2410917763085,12.7021266206828,10.4779065846965));
#12739=CARTESIAN_POINT('Ctrl Pts',(16.2629098463051,12.7049186032388,10.4337975121256));
#12740=CARTESIAN_POINT('Ctrl Pts',(16.275331417334,12.7065081484936,10.4086851177642));
#12741=CARTESIAN_POINT('Ctrl Pts',(16.2877869550192,12.7081134503575,10.3834999760487));
#12742=CARTESIAN_POINT('Ctrl Pts',(16.3002978241236,12.7097367072451,10.3581900732938));
#12743=CARTESIAN_POINT('Ctrl Pts',(16.3332728445508,12.7140151413477,10.2914805143182));
#12744=CARTESIAN_POINT('Ctrl Pts',(16.3662336781026,12.7183664950041,10.2247075060269));
#12745=CARTESIAN_POINT('Ctrl Pts',(16.3990971166876,12.7227674591413,10.1579087130742));
#12746=CARTESIAN_POINT('Ctrl Pts',(16.4256676679983,12.7263257004105,10.1039009514988));
#12747=CARTESIAN_POINT('Ctrl Pts',(16.4521754332255,12.7299165458893,10.0498755479769));
#12748=CARTESIAN_POINT('Ctrl Pts',(16.4785931654052,12.7335310522426,9.99583444252971));
#12749=CARTESIAN_POINT('Ctrl Pts',(16.5112266697307,12.7379960081257,9.9290781200575));
#12750=CARTESIAN_POINT('Ctrl Pts',(16.5437407424326,12.742500292084,9.86225899460185));
#12751=CARTESIAN_POINT('Ctrl Pts',(16.5760904789354,12.7470331104531,9.79538472693205));
#12752=CARTESIAN_POINT('Ctrl Pts',(16.6098424954697,12.7517624151426,9.72561162729884));
#12753=CARTESIAN_POINT('Ctrl Pts',(16.6434158824976,12.7565228077862,9.65577848505558));
#12754=CARTESIAN_POINT('Ctrl Pts',(16.6767921271902,12.7613076794793,9.58584680971152));
#12755=CARTESIAN_POINT('Ctrl Pts',(16.6976670791072,12.7643003458935,9.54210850500634));
#12756=CARTESIAN_POINT('Ctrl Pts',(16.718465539199,12.7673026982108,9.49833072232483));
#12757=CARTESIAN_POINT('Ctrl Pts',(16.7391883141092,12.7703140978295,9.45449535259596));
#12758=CARTESIAN_POINT('Ctrl Pts',(16.7808367856317,12.7763663853155,9.36639536812287));
#12759=CARTESIAN_POINT('Ctrl Pts',(16.8222902539778,12.7824713543034,9.2778265112276));
#12760=CARTESIAN_POINT('Ctrl Pts',(16.8634541590761,12.7886112584458,9.18886180766335));
#12761=CARTESIAN_POINT('Ctrl Pts',(16.8657796830592,12.788958127731,9.18383581337804));
#12762=CARTESIAN_POINT('Ctrl Pts',(16.8681042913027,12.789305109897,9.17880854502639));
#12763=CARTESIAN_POINT('Ctrl Pts',(16.87042796971,12.7896522022311,9.17378001198317));
#12764=CARTESIAN_POINT('Ctrl Pts',(16.9167422154902,12.7965702506232,9.07355413109334));
#12765=CARTESIAN_POINT('Ctrl Pts',(16.962447971316,12.8034966804412,8.97333336966089));
#12766=CARTESIAN_POINT('Ctrl Pts',(17.0075101299617,12.810423211497,8.87310027386457));
#12767=CARTESIAN_POINT('Ctrl Pts',(17.0548200626743,12.8176952492339,8.76786738755362));
#12768=CARTESIAN_POINT('Ctrl Pts',(17.1014209523388,12.8249674208786,8.66262094537315));
#12769=CARTESIAN_POINT('Ctrl Pts',(17.1473021985064,12.8322356635336,8.55728965067821));
#12770=CARTESIAN_POINT('Ctrl Pts',(17.1927178496159,12.8394301493023,8.45302723999089));
#12771=CARTESIAN_POINT('Ctrl Pts',(17.237428958698,12.8466208518308,8.34868128905732));
#12772=CARTESIAN_POINT('Ctrl Pts',(17.2814464207459,12.8538083506489,8.2441373109611));
#12773=CARTESIAN_POINT('Ctrl Pts',(17.3282209127514,12.8614460378386,8.13304522976901));
#12774=CARTESIAN_POINT('Ctrl Pts',(17.3742029960782,12.8690793531583,8.02170985269986));
#12775=CARTESIAN_POINT('Ctrl Pts',(17.4194367848341,12.8767174233848,7.90998003610143));
#12776=CARTESIAN_POINT('Ctrl Pts',(17.4592412159324,12.8834387051615,7.81166101598985));
#12777=CARTESIAN_POINT('Ctrl Pts',(17.4984666249301,12.8901637443241,7.71303551607771));
#12778=CARTESIAN_POINT('Ctrl Pts',(17.537147804236,12.8969009187565,7.61396771456222));
#12779=CARTESIAN_POINT('Ctrl Pts',(17.592514077251,12.9065441676352,7.47216710134099));
#12780=CARTESIAN_POINT('Ctrl Pts',(17.6466111403711,12.9161930408258,7.3298409308964));
#12781=CARTESIAN_POINT('Ctrl Pts',(17.6993823050438,12.9258391470742,7.18703139954518));
#12782=CARTESIAN_POINT('Ctrl Pts',(17.7538795876936,12.9358007725557,7.03955064100196));
#12783=CARTESIAN_POINT('Ctrl Pts',(17.8069632788614,12.9457594336855,6.89155414629607));
#12784=CARTESIAN_POINT('Ctrl Pts',(17.8585858804981,12.9557103540787,6.74303368137663));
#12785=CARTESIAN_POINT('Ctrl Pts',(17.9126720143282,12.9661361519861,6.58742552743936));
#12786=CARTESIAN_POINT('Ctrl Pts',(17.9651548061949,12.9765534332868,6.43124205075313));
#12787=CARTESIAN_POINT('Ctrl Pts',(18.0159880164975,12.9869618042602,6.2744175466783));
#12788=CARTESIAN_POINT('Ctrl Pts',(18.0316413020919,12.9901668979863,6.22612591339651));
#12789=CARTESIAN_POINT('Ctrl Pts',(18.0471381945933,12.9933711829021,6.17777311859869));
#12790=CARTESIAN_POINT('Ctrl Pts',(18.0624773722234,12.9965747421708,6.12935627695676));
#12791=CARTESIAN_POINT('Ctrl Pts',(18.1057590938429,13.0056140507834,5.9927411133419));
#12792=CARTESIAN_POINT('Ctrl Pts',(18.1477566607642,13.0146488660571,5.8556152595047));
#12793=CARTESIAN_POINT('Ctrl Pts',(18.1884785365491,13.0236795201517,5.71803784983784));
#12794=CARTESIAN_POINT('Ctrl Pts',(18.2387485231049,13.0348276033668,5.54820248736866));
#12795=CARTESIAN_POINT('Ctrl Pts',(18.2870623372161,13.0459810891294,5.37771014955191));
#12796=CARTESIAN_POINT('Ctrl Pts',(18.333408890949,13.0571305535019,5.206676417006));
#12797=CARTESIAN_POINT('Ctrl Pts',(18.3822015246055,13.0688684646684,5.02661586054878));
#12798=CARTESIAN_POINT('Ctrl Pts',(18.4288144063872,13.0806018838886,4.84595419871784));
#12799=CARTESIAN_POINT('Ctrl Pts',(18.4732069565691,13.0923262622486,4.66477210676923));
#12800=CARTESIAN_POINT('Ctrl Pts',(18.5198097359117,13.104634377358,4.47456926828994));
#12801=CARTESIAN_POINT('Ctrl Pts',(18.5639664343605,13.1169325338878,4.28379137577915));
#12802=CARTESIAN_POINT('Ctrl Pts',(18.6055886379374,13.1292226566585,4.09249383743625));
#12803=CARTESIAN_POINT('Ctrl Pts',(18.6290505764319,13.1361504519157,3.98466170234839));
#12804=CARTESIAN_POINT('Ctrl Pts',(18.651706382388,13.1430758235437,3.87666390827378));
#12805=CARTESIAN_POINT('Ctrl Pts',(18.6735332660427,13.15,3.76850837361377));
#12806=CARTESIAN_POINT('Origin',(0.,13.15,0.));
#12807=CARTESIAN_POINT('',(-17.6839681951541,12.6595351585866,8.10490082533369));
#12808=CARTESIAN_POINT('Ctrl Pts',(-17.9697662756086,12.65,7.7));
#12809=CARTESIAN_POINT('Ctrl Pts',(-17.9083648469828,12.65,7.78712872535143));
#12810=CARTESIAN_POINT('Ctrl Pts',(-17.8469550493761,12.6514513272162,7.87425941670175));
#12811=CARTESIAN_POINT('Ctrl Pts',(-17.7854838084763,12.6541030519202,7.96131023851809));
#12812=CARTESIAN_POINT('Ctrl Pts',(-17.7516647322465,12.6555619272999,8.00920220125992));
#12813=CARTESIAN_POINT('Ctrl Pts',(-17.7178277666382,12.6573848689011,8.05707001525365));
#12814=CARTESIAN_POINT('Ctrl Pts',(-17.6839681951541,12.6595351585866,8.1049008253337));
#12815=CARTESIAN_POINT('Ctrl Pts',(-17.6839681951541,12.6595351585866,8.1049008253337));
#12816=CARTESIAN_POINT('Ctrl Pts',(-17.6639265614649,12.6608079247683,8.13321209866034));
#12817=CARTESIAN_POINT('Ctrl Pts',(-17.6438738738723,12.6621745127572,8.16182239750707));
#12818=CARTESIAN_POINT('Ctrl Pts',(-17.6238677063287,12.663612285139,8.19057990120395));
#12819=CARTESIAN_POINT('Ctrl Pts',(-17.6030925230288,12.6651053239586,8.22044281269102));
#12820=CARTESIAN_POINT('Ctrl Pts',(-17.5823674018309,12.6666751553062,8.25046474478147));
#12821=CARTESIAN_POINT('Ctrl Pts',(-17.5617329120168,12.6683023351362,8.28052703089315));
#12822=CARTESIAN_POINT('Ctrl Pts',(-17.5398152337084,12.6700307037261,8.31245878797306));
#12823=CARTESIAN_POINT('Ctrl Pts',(-17.5179997812459,12.6718237880053,8.34443620514295));
#12824=CARTESIAN_POINT('Ctrl Pts',(-17.4963096374199,12.6736645084151,8.37637087905986));
#12825=CARTESIAN_POINT('Ctrl Pts',(-17.4738213436033,12.6755729633218,8.4094806793332));
#12826=CARTESIAN_POINT('Ctrl Pts',(-17.451467611317,12.6775326648018,8.44254490102727));
#12827=CARTESIAN_POINT('Ctrl Pts',(-17.4292490045524,12.6795306118022,8.47551687033708));
#12828=CARTESIAN_POINT('Ctrl Pts',(-17.4057576404398,12.6816430080006,8.51037758616752));
#12829=CARTESIAN_POINT('Ctrl Pts',(-17.3824172571268,12.6837981812706,8.5451354143792));
#12830=CARTESIAN_POINT('Ctrl Pts',(-17.3592024471202,12.6859869025222,8.57978752344679));
#12831=CARTESIAN_POINT('Ctrl Pts',(-17.3489254331789,12.6869558322188,8.59512773979505));
#12832=CARTESIAN_POINT('Ctrl Pts',(-17.338672705411,12.6879314118332,8.61044787721113));
#12833=CARTESIAN_POINT('Ctrl Pts',(-17.3284406171285,12.6889131739459,8.62575051029075));
#12834=CARTESIAN_POINT('Ctrl Pts',(-17.3018516196084,12.6914643706967,8.66551577245167));
#12835=CARTESIAN_POINT('Ctrl Pts',(-17.2754161582636,12.6940529314351,8.70513096214322));
#12836=CARTESIAN_POINT('Ctrl Pts',(-17.2490046751076,12.6966799223705,8.74474033626622));
#12837=CARTESIAN_POINT('Ctrl Pts',(-17.2218291628616,12.6993829066715,8.7854955269224));
#12838=CARTESIAN_POINT('Ctrl Pts',(-17.1946791689703,12.7021266206838,8.82624477114721));
#12839=CARTESIAN_POINT('Ctrl Pts',(-17.1673886265825,12.7049186032401,8.86719431031478));
#12840=CARTESIAN_POINT('Ctrl Pts',(-17.1518514406346,12.7065081484945,8.89050790355471));
#12841=CARTESIAN_POINT('Ctrl Pts',(-17.1362682369582,12.7081134503579,8.91388728645879));
#12842=CARTESIAN_POINT('Ctrl Pts',(-17.120604652762,12.709736707245,8.93737696829701));
#12843=CARTESIAN_POINT('Ctrl Pts',(-17.0793199902274,12.7140151413476,8.99928895316511));
#12844=CARTESIAN_POINT('Ctrl Pts',(-17.0379732855358,12.7183664950041,9.06122037649655));
#12845=CARTESIAN_POINT('Ctrl Pts',(-16.996555553189,12.7227674591413,9.12308034564325));
#12846=CARTESIAN_POINT('Ctrl Pts',(-16.9630687353186,12.7263257004105,9.1730949988584));
#12847=CARTESIAN_POINT('Ctrl Pts',(-16.9295352460326,12.7299165458893,9.22306409870345));
#12848=CARTESIAN_POINT('Ctrl Pts',(-16.8959431419567,12.7335310522426,9.2729630786048));
#12849=CARTESIAN_POINT('Ctrl Pts',(-16.8544472229965,12.7379960081256,9.33460268359952));
#12850=CARTESIAN_POINT('Ctrl Pts',(-16.8128371992455,12.7425002920837,9.39617025926588));
#12851=CARTESIAN_POINT('Ctrl Pts',(-16.7710972528366,12.7470331104527,9.45762308671611));
#12852=CARTESIAN_POINT('Ctrl Pts',(-16.7275479843214,12.751762415142,9.52173974027936));
#12853=CARTESIAN_POINT('Ctrl Pts',(-16.6838574026273,12.7565228077855,9.58573171745721));
#12854=CARTESIAN_POINT('Ctrl Pts',(-16.6399829175973,12.7613076794785,9.64960223091488));
#12855=CARTESIAN_POINT('Ctrl Pts',(-16.6125419105606,12.7643003458929,9.68954962193329));
#12856=CARTESIAN_POINT('Ctrl Pts',(-16.5850284686809,12.7673026982104,9.72945050807611));
#12857=CARTESIAN_POINT('Ctrl Pts',(-16.5574273123645,12.7703140978294,9.76931464245264));
#12858=CARTESIAN_POINT('Ctrl Pts',(-16.5019547235018,12.7763663853151,9.84943326905253));
#12859=CARTESIAN_POINT('Ctrl Pts',(-16.4459785776221,12.7824713543027,9.9296174541588));
#12860=CARTESIAN_POINT('Ctrl Pts',(-16.3895148368472,12.788611258445,10.0097487934709));
#12861=CARTESIAN_POINT('Ctrl Pts',(-16.3863249601057,12.7889581277305,10.0142757534639));
#12862=CARTESIAN_POINT('Ctrl Pts',(-16.3831335221205,12.7893051098969,10.0188025574363));
#12863=CARTESIAN_POINT('Ctrl Pts',(-16.3799405239623,12.7896522022313,10.0233291884927));
#12864=CARTESIAN_POINT('Ctrl Pts',(-16.3162994878893,12.796570250623,10.113551442334));
#12865=CARTESIAN_POINT('Ctrl Pts',(-16.2523586404194,12.8034966804406,10.2032441686885));
#12866=CARTESIAN_POINT('Ctrl Pts',(-16.1880853124871,12.8104232114959,10.2923856907174));
#12867=CARTESIAN_POINT('Ctrl Pts',(-16.1206059259881,12.8176952492324,10.3859737374485));
#12868=CARTESIAN_POINT('Ctrl Pts',(-16.0527602782377,12.8249674208766,10.4789545128227));
#12869=CARTESIAN_POINT('Ctrl Pts',(-15.9844813243059,12.8322356635312,10.5713544849041));
#12870=CARTESIAN_POINT('Ctrl Pts',(-15.9168952535378,12.8394301493006,10.6628167978489));
#12871=CARTESIAN_POINT('Ctrl Pts',(-15.8488845637804,12.8466208518299,10.753710729623));
#12872=CARTESIAN_POINT('Ctrl Pts',(-15.7803555539523,12.8538083506489,10.8441029590253));
#12873=CARTESIAN_POINT('Ctrl Pts',(-15.7075342354825,12.8614460378387,10.9401568979484));
#12874=CARTESIAN_POINT('Ctrl Pts',(-15.6341060122632,12.8690793531585,11.035646238764));
#12875=CARTESIAN_POINT('Ctrl Pts',(-15.5599620471059,12.8767174233851,11.1306847572363));
#12876=CARTESIAN_POINT('Ctrl Pts',(-15.4947174935641,12.8834387051617,11.2143159158053));
#12877=CARTESIAN_POINT('Ctrl Pts',(-15.428918009679,12.8901637443243,11.297598866426));
#12878=CARTESIAN_POINT('Ctrl Pts',(-15.3624633665233,12.8969009187565,11.3806316511099));
#12879=CARTESIAN_POINT('Ctrl Pts',(-15.2673435697082,12.9065441676353,11.4994805566654));
#12880=CARTESIAN_POINT('Ctrl Pts',(-15.1711340220391,12.916193040826,11.6174930728209));
#12881=CARTESIAN_POINT('Ctrl Pts',(-15.0738429223219,12.9258391470746,11.7345990076912));
#12882=CARTESIAN_POINT('Ctrl Pts',(-14.9733694801788,12.9358007725561,11.8555354181748));
#12883=CARTESIAN_POINT('Ctrl Pts',(-14.8717426016762,12.945759433686,11.9755054906058));
#12884=CARTESIAN_POINT('Ctrl Pts',(-14.7689314068923,12.9557103540793,12.0944722074925));
#12885=CARTESIAN_POINT('Ctrl Pts',(-14.6612138594637,12.9661361519865,12.219116250348));
#12886=CARTESIAN_POINT('Ctrl Pts',(-14.5521963969374,12.9765534332871,12.3426594197069));
#12887=CARTESIAN_POINT('Ctrl Pts',(-14.441798997626,12.9869618042603,12.4650945232202));
#12888=CARTESIAN_POINT('Ctrl Pts',(-14.4078038592099,12.9901668979865,12.5027964828396));
#12889=CARTESIAN_POINT('Ctrl Pts',(-14.3736775568208,12.9933711829024,12.5403935828256));
#12890=CARTESIAN_POINT('Ctrl Pts',(-14.3394169308019,12.9965747421713,12.5778861211484));
#12891=CARTESIAN_POINT('Ctrl Pts',(-14.242745589379,13.0056140507838,12.683676773398));
#12892=CARTESIAN_POINT('Ctrl Pts',(-14.144989899901,13.0146488660574,12.7886106601676));
#12893=CARTESIAN_POINT('Ctrl Pts',(-14.046205306035,13.0236795201519,12.8926655439204));
#12894=CARTESIAN_POINT('Ctrl Pts',(-13.9242585601308,13.0348276034422,13.0211183114271));
#12895=CARTESIAN_POINT('Ctrl Pts',(-13.8007647706452,13.0459810892792,13.1482054715556));
#12896=CARTESIAN_POINT('Ctrl Pts',(-13.675818489362,13.0571305537241,13.2738596315664));
#12897=CARTESIAN_POINT('Ctrl Pts',(-13.544277788722,13.0688684650071,13.4061455713829));
#12898=CARTESIAN_POINT('Ctrl Pts',(-13.411126639588,13.0806018843413,13.5368443433571));
#12899=CARTESIAN_POINT('Ctrl Pts',(-13.2764146189179,13.0923262628158,13.6658804667858));
#12900=CARTESIAN_POINT('Ctrl Pts',(-13.1349955163823,13.1046343781079,13.8013410788322));
#12901=CARTESIAN_POINT('Ctrl Pts',(-12.9918553619456,13.1169325348207,13.9349708496446));
#12902=CARTESIAN_POINT('Ctrl Pts',(-12.8469979335291,13.1292226577834,14.0666655063646));
#12903=CARTESIAN_POINT('Ctrl Pts',(-12.7653435388819,13.1361504526617,14.1409002045109));
#12904=CARTESIAN_POINT('Ctrl Pts',(-12.6831426131348,13.143075823914,14.2145196009598));
#12905=CARTESIAN_POINT('Ctrl Pts',(-12.6003906189451,13.15,14.2875));
#12906=CARTESIAN_POINT('',(-17.6839681951541,12.6595351585866,-8.10490082533369));
#12907=CARTESIAN_POINT('Ctrl Pts',(-12.6003906189451,13.15,-14.2875));
#12908=CARTESIAN_POINT('Ctrl Pts',(-12.7441724131263,13.1379692270445,-14.1606963765126));
#12909=CARTESIAN_POINT('Ctrl Pts',(-12.8860272181368,13.125955492064,-14.0322407960939));
#12910=CARTESIAN_POINT('Ctrl Pts',(-13.0261262286746,13.113945529667,-13.9020936737457));
#12911=CARTESIAN_POINT('Ctrl Pts',(-13.1636503206767,13.1021563016968,-13.7743385614223));
#12912=CARTESIAN_POINT('Ctrl Pts',(-13.2994830412214,13.0903706661861,-13.6449524828629));
#12913=CARTESIAN_POINT('Ctrl Pts',(-13.4337424366336,13.0785760987039,-13.5138761943818));
#12914=CARTESIAN_POINT('Ctrl Pts',(-13.5641057336281,13.0671237999736,-13.3866036331451));
#12915=CARTESIAN_POINT('Ctrl Pts',(-13.6929860436161,13.0556630399218,-13.2577366470546));
#12916=CARTESIAN_POINT('Ctrl Pts',(-13.8204438235608,13.0441829768352,-13.1272141956059));
#12917=CARTESIAN_POINT('Ctrl Pts',(-13.941366662559,13.0332915128467,-13.0033838151535));
#12918=CARTESIAN_POINT('Ctrl Pts',(-14.0610092039394,13.0223826438948,-12.8780627055743));
#12919=CARTESIAN_POINT('Ctrl Pts',(-14.1793767143662,13.0114481775172,-12.7512035014433));
#12920=CARTESIAN_POINT('Ctrl Pts',(-14.2326873232158,13.0065234895016,-12.6940683856839));
#12921=CARTESIAN_POINT('Ctrl Pts',(-14.2857386459499,13.001593626696,-12.636621401153));
#12922=CARTESIAN_POINT('Ctrl Pts',(-14.3385277495326,12.9966579427912,-12.5788590968463));
#12923=CARTESIAN_POINT('Ctrl Pts',(-14.4379871334572,12.9873586736788,-12.4700297587729));
#12924=CARTESIAN_POINT('Ctrl Pts',(-14.5366365957252,12.9780292666576,-12.3599777689006));
#12925=CARTESIAN_POINT('Ctrl Pts',(-14.6343553826822,12.9686821009635,-12.2488863675566));
#12926=CARTESIAN_POINT('Ctrl Pts',(-14.7257869136757,12.9599363347044,-12.1449426201832));
#12927=CARTESIAN_POINT('Ctrl Pts',(-14.8164036660272,12.9511750020356,-12.040088617895));
#12928=CARTESIAN_POINT('Ctrl Pts',(-14.9060737173319,12.9424107434987,-11.9345044582147));
#12929=CARTESIAN_POINT('Ctrl Pts',(-14.9727981511875,12.9358891659985,-11.8559381679508));
#12930=CARTESIAN_POINT('Ctrl Pts',(-15.038997771599,12.9293660137802,-11.776968131275));
#12931=CARTESIAN_POINT('Ctrl Pts',(-15.104604989498,12.922847596419,-11.6976820181931));
#12932=CARTESIAN_POINT('Ctrl Pts',(-15.191515741447,12.9142125624619,-11.59265065232));
#12933=CARTESIAN_POINT('Ctrl Pts',(-15.2773936169565,12.9055857664761,-11.4870734789433));
#12934=CARTESIAN_POINT('Ctrl Pts',(-15.3622370308358,12.896973446382,-11.3810364587419));
#12935=CARTESIAN_POINT('Ctrl Pts',(-15.4402693750153,12.8890525071477,-11.2835118910966));
#12936=CARTESIAN_POINT('Ctrl Pts',(-15.5175063401343,12.8811371827706,-11.1854984927171));
#12937=CARTESIAN_POINT('Ctrl Pts',(-15.5940304829928,12.8732239828736,-11.0869467036663));
#12938=CARTESIAN_POINT('Ctrl Pts',(-15.6585664561948,12.8665504542666,-11.0038339058012));
#12939=CARTESIAN_POINT('Ctrl Pts',(-15.7225949096337,12.8598784744129,-10.9203385092677));
#12940=CARTESIAN_POINT('Ctrl Pts',(-15.7861463899371,12.8532079839213,-10.8364525446741));
#12941=CARTESIAN_POINT('Ctrl Pts',(-15.8582933779828,12.845635291744,-10.7412207789333));
#12942=CARTESIAN_POINT('Ctrl Pts',(-15.9298271822287,12.8380640091307,-10.645484655158));
#12943=CARTESIAN_POINT('Ctrl Pts',(-16.0007909829629,12.8305004633243,-10.5492609278545));
#12944=CARTESIAN_POINT('Ctrl Pts',(-16.0685117630156,12.8232825688953,-10.4574345909735));
#12945=CARTESIAN_POINT('Ctrl Pts',(-16.135713261652,12.8160717028965,-10.3651639852349));
#12946=CARTESIAN_POINT('Ctrl Pts',(-16.2024113995638,12.8088775452781,-10.2725043154411));
#12947=CARTESIAN_POINT('Ctrl Pts',(-16.2628774029162,12.8023555947066,-10.1885025714674));
#12948=CARTESIAN_POINT('Ctrl Pts',(-16.3229294498328,12.7958473962744,-10.1041812447974));
#12949=CARTESIAN_POINT('Ctrl Pts',(-16.3825645654634,12.7893635951272,-10.0196153024904));
#12950=CARTESIAN_POINT('Ctrl Pts',(-16.4338747918932,12.7837849138171,-9.94685452048908));
#12951=CARTESIAN_POINT('Ctrl Pts',(-16.4849711617777,12.7782136874731,-9.87377080481835));
#12952=CARTESIAN_POINT('Ctrl Pts',(-16.5357581870816,12.7726724740281,-9.80057396479367));
#12953=CARTESIAN_POINT('Ctrl Pts',(-16.5429918774568,12.7718832287017,-9.79014840287087));
#12954=CARTESIAN_POINT('Ctrl Pts',(-16.5502192549354,12.7710945998698,-9.77972062379159));
#12955=CARTESIAN_POINT('Ctrl Pts',(-16.5574400057254,12.7703066605067,-9.76929131333199));
#12956=CARTESIAN_POINT('Ctrl Pts',(-16.5968985793309,12.7660008806426,-9.71229921841124));
#12957=CARTESIAN_POINT('Ctrl Pts',(-16.6361690358739,12.7617151304109,-9.65524596704519));
#12958=CARTESIAN_POINT('Ctrl Pts',(-16.6753137127505,12.757449305424,-9.59807929514968));
#12959=CARTESIAN_POINT('Ctrl Pts',(-16.7127983462431,12.7533643850993,-9.54333694152762));
#12960=CARTESIAN_POINT('Ctrl Pts',(-16.7501677296326,12.7492976981851,-9.48849017090563));
#12961=CARTESIAN_POINT('Ctrl Pts',(-16.787450624392,12.7452532521653,-9.43353282796637));
#12962=CARTESIAN_POINT('Ctrl Pts',(-16.8227652435108,12.7414223245601,-9.38147684770499));
#12963=CARTESIAN_POINT('Ctrl Pts',(-16.8580022961618,12.7376113278547,-9.3293213954541));
#12964=CARTESIAN_POINT('Ctrl Pts',(-16.8931616480444,12.7338278436747,-9.2771023096645));
#12965=CARTESIAN_POINT('Ctrl Pts',(-16.8951212697981,12.73361696954,-9.27419185622914));
#12966=CARTESIAN_POINT('Ctrl Pts',(-16.8970806434167,12.7334061820621,-9.27128121690781));
#12967=CARTESIAN_POINT('Ctrl Pts',(-16.8990397664385,12.7331954829857,-9.26837040218869));
#12968=CARTESIAN_POINT('Ctrl Pts',(-16.9371666975596,12.7290950211555,-9.21172238617983));
#12969=CARTESIAN_POINT('Ctrl Pts',(-16.975182979148,12.7250294339061,-9.15504020050686));
#12970=CARTESIAN_POINT('Ctrl Pts',(-17.0131365974396,12.7210081247695,-9.09831360735279));
#12971=CARTESIAN_POINT('Ctrl Pts',(-17.049001223072,12.7172081511905,-9.04470928401151));
#12972=CARTESIAN_POINT('Ctrl Pts',(-17.0848096750461,12.7134477064406,-8.99106534580903));
#12973=CARTESIAN_POINT('Ctrl Pts',(-17.1205869200985,12.7097399996136,-8.93741269274753));
#12974=CARTESIAN_POINT('Ctrl Pts',(-17.1506808085402,12.7066212766525,-8.89228297542374));
#12975=CARTESIAN_POINT('Ctrl Pts',(-17.1806491209783,12.7035507329854,-8.84730189704762));
#12976=CARTESIAN_POINT('Ctrl Pts',(-17.2106032474357,12.700528362805,-8.80235472546476));
#12977=CARTESIAN_POINT('Ctrl Pts',(-17.2397362162722,12.6975888473963,-8.75863972843841));
#12978=CARTESIAN_POINT('Ctrl Pts',(-17.2688556247791,12.6946948638806,-8.71495663452867));
#12979=CARTESIAN_POINT('Ctrl Pts',(-17.298043382292,12.6918520765307,-8.67124428128174));
#12980=CARTESIAN_POINT('Ctrl Pts',(-17.3086494139828,12.6908190854655,-8.65536040929836));
#12981=CARTESIAN_POINT('Ctrl Pts',(-17.319264279989,12.6897929124039,-8.63947312008266));
#12982=CARTESIAN_POINT('Ctrl Pts',(-17.3298912650618,12.6887740383049,-8.62358106878228));
#12983=CARTESIAN_POINT('Ctrl Pts',(-17.3588241806496,12.68600006261,-8.58031354034972));
#12984=CARTESIAN_POINT('Ctrl Pts',(-17.3878484570357,12.6832787578847,-8.53700528592784));
#12985=CARTESIAN_POINT('Ctrl Pts',(-17.4170136643082,12.6806283209993,-8.49366207193208));
#12986=CARTESIAN_POINT('Ctrl Pts',(-17.4444175875333,12.6781379437412,-8.45293635043883));
#12987=CARTESIAN_POINT('Ctrl Pts',(-17.4719457319131,12.6757101114829,-8.41217982595808));
#12988=CARTESIAN_POINT('Ctrl Pts',(-17.4996239289404,12.6733674903698,-8.37144299883949));
#12989=CARTESIAN_POINT('Ctrl Pts',(-17.5266691481136,12.6710784430962,-8.33163778982419));
#12990=CARTESIAN_POINT('Ctrl Pts',(-17.5538575291632,12.6688706813127,-8.29185114713442));
#12991=CARTESIAN_POINT('Ctrl Pts',(-17.5812001624053,12.6667735640338,-8.2521769624176));
#12992=CARTESIAN_POINT('Ctrl Pts',(-17.6076475256248,12.664745111913,-8.21380181528551));
#12993=CARTESIAN_POINT('Ctrl Pts',(-17.6342390703436,12.6628201182912,-8.17553172577809));
#12994=CARTESIAN_POINT('Ctrl Pts',(-17.6609742962525,12.6610338566174,-8.13749868299144));
#12995=CARTESIAN_POINT('Ctrl Pts',(-17.6686272679742,12.6605225383243,-8.12661170556599));
#12996=CARTESIAN_POINT('Ctrl Pts',(-17.6762919519737,12.6600226469234,-8.11574446327037));
#12997=CARTESIAN_POINT('Ctrl Pts',(-17.6839681951541,12.6595351585866,-8.1049008253337));
#12998=CARTESIAN_POINT('Ctrl Pts',(-17.6839681951541,12.6595351585866,-8.1049008253337));
#12999=CARTESIAN_POINT('Ctrl Pts',(-17.7455130422198,12.6556266847331,-8.01796115768933));
#13000=CARTESIAN_POINT('Ctrl Pts',(-17.8069815347887,12.6527974939074,-7.93089878537348));
#13001=CARTESIAN_POINT('Ctrl Pts',(-17.8684084088704,12.6512766915374,-7.84379266928167));
#13002=CARTESIAN_POINT('Ctrl Pts',(-17.9022030762551,12.6504400054611,-7.79587028572398));
#13003=CARTESIAN_POINT('Ctrl Pts',(-17.9359856073363,12.65,-7.74793482226751));
#13004=CARTESIAN_POINT('Ctrl Pts',(-17.9697662756086,12.65,-7.7));
#13005=CARTESIAN_POINT('Origin',(0.,22.22,7.70000000000001));
#13006=CARTESIAN_POINT('',(2.55537495509676,22.22,-8.00360031633711));
#13007=CARTESIAN_POINT('Ctrl Pts',(2.55537495509672,22.22,-8.00360031633714));
#13008=CARTESIAN_POINT('Ctrl Pts',(2.31636652071332,22.22,-8.05981884049116));
#13009=CARTESIAN_POINT('Ctrl Pts',(2.09333395643987,22.2199999999995,-8.10671764219108));
#13010=CARTESIAN_POINT('Ctrl Pts',(1.62382106309547,22.2199999999995,-8.18876435835048));
#13011=CARTESIAN_POINT('Ctrl Pts',(1.39036720391674,22.22,-8.22145831436959));
#13012=CARTESIAN_POINT('Ctrl Pts',(1.15457232288596,22.22,-8.24555872886889));
#13013=CARTESIAN_POINT('',(4.50738083181344,22.22,8.84193633985987));
#13014=CARTESIAN_POINT('Ctrl Pts',(4.50738083181345,22.22,8.84193633985991));
#13015=CARTESIAN_POINT('Ctrl Pts',(5.50129019941128,22.22,8.24752673459274));
#13016=CARTESIAN_POINT('Ctrl Pts',(6.38273063962348,22.22,7.48282682306534));
#13017=CARTESIAN_POINT('Ctrl Pts',(7.72906558127775,22.22,5.82007728703888));
#13018=CARTESIAN_POINT('Ctrl Pts',(8.42964347032215,22.2199999999936,4.72920057212043));
#13019=CARTESIAN_POINT('Ctrl Pts',(9.2043748646196,22.2199999999936,2.1387789590176));
#13020=CARTESIAN_POINT('Ctrl Pts',(9.31838831238722,22.22,0.915490022079924));
#13021=CARTESIAN_POINT('Ctrl Pts',(9.06300659638671,22.22,-1.507993106964));
#13022=CARTESIAN_POINT('Ctrl Pts',(8.69486484793729,22.22,-2.68367031517768));
#13023=CARTESIAN_POINT('Ctrl Pts',(7.55278087878453,22.22,-4.76564642192656));
#13024=CARTESIAN_POINT('Ctrl Pts',(6.81838193887901,22.219999999987,-5.65268890498168));
#13025=CARTESIAN_POINT('Ctrl Pts',(5.41795245135685,22.219999999987,-6.76839622139175));
#13026=CARTESIAN_POINT('Ctrl Pts',(4.87996243897349,22.2199999976409,-7.10670058837755));
#13027=CARTESIAN_POINT('Ctrl Pts',(3.74918166874661,22.2199999976409,-7.65278819993115));
#13028=CARTESIAN_POINT('Ctrl Pts',(3.16100732091391,22.22,-7.86114610599102));
#13029=CARTESIAN_POINT('Ctrl Pts',(2.55537495509677,22.22,-8.00360031633713));
#13030=CARTESIAN_POINT('',(-7.96780251527898,22.22,-2.66489817109789));
#13031=CARTESIAN_POINT('Ctrl Pts',(-7.96780251527902,22.22,-2.66489817109774));
#13032=CARTESIAN_POINT('Ctrl Pts',(-8.23599312974415,22.22,-2.02792425502546));
#13033=CARTESIAN_POINT('Ctrl Pts',(-8.4263439618362,22.22,-1.36096366704832));
#13034=CARTESIAN_POINT('Ctrl Pts',(-8.64297828766049,22.22,0.00360816572491401));
#13035=CARTESIAN_POINT('Ctrl Pts',(-8.66859900866027,22.22,0.696135165601527));
#13036=CARTESIAN_POINT('Ctrl Pts',(-8.52525050570627,22.22,2.41043360782728));
#13037=CARTESIAN_POINT('Ctrl Pts',(-8.255689969321,22.2199999999164,3.41277917262433));
#13038=CARTESIAN_POINT('Ctrl Pts',(-7.37169226325107,22.2199999999164,5.28253364315786));
#13039=CARTESIAN_POINT('Ctrl Pts',(-6.69159903012222,22.2199999999999,6.31291964415821));
#13040=CARTESIAN_POINT('Ctrl Pts',(-4.74829296569674,22.2199999999999,8.0685409876383));
#13041=CARTESIAN_POINT('Ctrl Pts',(-3.68909457138914,22.22,8.69991320242805));
#13042=CARTESIAN_POINT('Ctrl Pts',(-1.08588604419115,22.22,9.62226726459541));
#13043=CARTESIAN_POINT('Ctrl Pts',(0.195202339552547,22.22,9.67166205579421));
#13044=CARTESIAN_POINT('Ctrl Pts',(2.25253429025285,22.22,9.57488020226816));
#13045=CARTESIAN_POINT('Ctrl Pts',(3.41720895858078,22.22,9.30785410203658));
#13046=CARTESIAN_POINT('Ctrl Pts',(4.50738083181195,22.22,8.84193633986044));
#13047=CARTESIAN_POINT('Ctrl Pts',(-7.30706743901568,22.22,-3.99112032412916));
#13048=CARTESIAN_POINT('Ctrl Pts',(-7.43302521096891,22.22,-3.77868598418148));
#13049=CARTESIAN_POINT('Ctrl Pts',(-7.54996154878007,22.2200000000004,-3.56259441822855));
#13050=CARTESIAN_POINT('Ctrl Pts',(-7.77060228250538,22.2200000000004,-3.1175628528368));
#13051=CARTESIAN_POINT('Ctrl Pts',(-7.86861240549784,22.22,-2.90048252511764));
#13052=CARTESIAN_POINT('Ctrl Pts',(-7.96780251527901,22.22,-2.66489817109778));
#13053=CARTESIAN_POINT('Ctrl Pts',(-1.78726082715848E-11,-144.88675111262,
-9.92453123331945));
#13054=CARTESIAN_POINT('Ctrl Pts',(-5.7299307791557,-144.71175111262,-9.92453123330913));
#13055=CARTESIAN_POINT('Ctrl Pts',(-8.59489616871569,-144.53675111262,-4.96226561664425));
#13056=CARTESIAN_POINT('Ctrl Pts',(-11.4598615582757,-144.36175111262,2.06368086793017E-11));
#13057=CARTESIAN_POINT('Ctrl Pts',(-8.59489616869782,-144.18675111262,4.9622656166752));
#13058=CARTESIAN_POINT('Ctrl Pts',(-5.72993077911996,-144.01175111262,9.92453123332977));
#13059=CARTESIAN_POINT('Ctrl Pts',(1.7871392867044E-11,-143.83675111262,
9.92453123331945));
#13060=CARTESIAN_POINT('Ctrl Pts',(5.7299307791557,-143.66175111262,9.92453123330913));
#13061=CARTESIAN_POINT('Ctrl Pts',(8.59489616871569,-143.48675111262,4.96226561664425));
#13062=CARTESIAN_POINT('Ctrl Pts',(11.4598615582757,-143.31175111262,-2.06354052510241E-11));
#13063=CARTESIAN_POINT('Ctrl Pts',(8.59489616869782,-143.13675111262,-4.9622656166752));
#13064=CARTESIAN_POINT('Ctrl Pts',(5.72993077911996,-142.96175111262,-9.92453123332976));
#13065=CARTESIAN_POINT('Ctrl Pts',(-1.78726082715848E-11,-142.78675111262,
-9.92453123331945));
#13066=CARTESIAN_POINT('Ctrl Pts',(-5.7299307791557,-142.61175111262,-9.92453123330913));
#13067=CARTESIAN_POINT('Ctrl Pts',(-8.59489616871569,-142.43675111262,-4.96226561664425));
#13068=CARTESIAN_POINT('Ctrl Pts',(-11.4598615582757,-142.26175111262,2.06368086793017E-11));
#13069=CARTESIAN_POINT('Ctrl Pts',(-8.59489616869782,-142.08675111262,4.9622656166752));
#13070=CARTESIAN_POINT('Ctrl Pts',(-5.72993077911996,-141.91175111262,9.92453123332977));
#13071=CARTESIAN_POINT('Ctrl Pts',(1.7871392867044E-11,-141.73675111262,
9.92453123331945));
#13072=CARTESIAN_POINT('Ctrl Pts',(5.7299307791557,-141.56175111262,9.92453123330913));
#13073=CARTESIAN_POINT('Ctrl Pts',(8.59489616871569,-141.38675111262,4.96226561664425));
#13074=CARTESIAN_POINT('Ctrl Pts',(11.4598615582757,-141.21175111262,-2.06354052510241E-11));
#13075=CARTESIAN_POINT('Ctrl Pts',(8.59489616869782,-141.03675111262,-4.9622656166752));
#13076=CARTESIAN_POINT('Ctrl Pts',(5.72993077911996,-140.86175111262,-9.92453123332976));
#13077=CARTESIAN_POINT('Ctrl Pts',(-1.78726082715848E-11,-140.68675111262,
-9.92453123331945));
#13078=CARTESIAN_POINT('Ctrl Pts',(-5.7299307791557,-140.51175111262,-9.92453123330913));
#13079=CARTESIAN_POINT('Ctrl Pts',(-8.59489616871569,-140.33675111262,-4.96226561664425));
#13080=CARTESIAN_POINT('Ctrl Pts',(-11.4598615582757,-140.16175111262,2.06368086793017E-11));
#13081=CARTESIAN_POINT('Ctrl Pts',(-8.59489616869782,-139.98675111262,4.9622656166752));
#13082=CARTESIAN_POINT('Ctrl Pts',(-5.72993077911996,-139.81175111262,9.92453123332977));
#13083=CARTESIAN_POINT('Ctrl Pts',(1.7871392867044E-11,-139.63675111262,
9.92453123331945));
#13084=CARTESIAN_POINT('Ctrl Pts',(5.7299307791557,-139.46175111262,9.92453123330913));
#13085=CARTESIAN_POINT('Ctrl Pts',(8.59489616871569,-139.28675111262,4.96226561664425));
#13086=CARTESIAN_POINT('Ctrl Pts',(11.4598615582757,-139.11175111262,-2.06354052510241E-11));
#13087=CARTESIAN_POINT('Ctrl Pts',(8.59489616869782,-138.93675111262,-4.9622656166752));
#13088=CARTESIAN_POINT('Ctrl Pts',(5.72993077911996,-138.76175111262,-9.92453123332976));
#13089=CARTESIAN_POINT('Ctrl Pts',(-1.78726082715848E-11,-138.58675111262,
-9.92453123331945));
#13090=CARTESIAN_POINT('Ctrl Pts',(-5.7299307791557,-138.41175111262,-9.92453123330913));
#13091=CARTESIAN_POINT('Ctrl Pts',(-8.59489616871569,-138.23675111262,-4.96226561664425));
#13092=CARTESIAN_POINT('Ctrl Pts',(-11.4598615582757,-138.06175111262,2.06368086793017E-11));
#13093=CARTESIAN_POINT('Ctrl Pts',(-8.59489616869782,-137.88675111262,4.9622656166752));
#13094=CARTESIAN_POINT('Ctrl Pts',(-5.72993077911996,-137.71175111262,9.92453123332977));
#13095=CARTESIAN_POINT('Ctrl Pts',(1.7871392867044E-11,-137.53675111262,
9.92453123331945));
#13096=CARTESIAN_POINT('Ctrl Pts',(5.7299307791557,-137.36175111262,9.92453123330913));
#13097=CARTESIAN_POINT('Ctrl Pts',(8.59489616871569,-137.18675111262,4.96226561664425));
#13098=CARTESIAN_POINT('Ctrl Pts',(11.4598615582757,-137.01175111262,-2.06354052510241E-11));
#13099=CARTESIAN_POINT('Ctrl Pts',(8.59489616869782,-136.83675111262,-4.9622656166752));
#13100=CARTESIAN_POINT('Ctrl Pts',(5.72993077911996,-136.66175111262,-9.92453123332976));
#13101=CARTESIAN_POINT('Ctrl Pts',(-1.78726082715848E-11,-136.48675111262,
-9.92453123331945));
#13102=CARTESIAN_POINT('Ctrl Pts',(-5.7299307791557,-136.31175111262,-9.92453123330913));
#13103=CARTESIAN_POINT('Ctrl Pts',(-8.59489616871569,-136.13675111262,-4.96226561664425));
#13104=CARTESIAN_POINT('Ctrl Pts',(-11.4598615582757,-135.96175111262,2.06368086793017E-11));
#13105=CARTESIAN_POINT('Ctrl Pts',(-8.59489616869782,-135.78675111262,4.9622656166752));
#13106=CARTESIAN_POINT('Ctrl Pts',(-5.72993077911996,-135.61175111262,9.92453123332977));
#13107=CARTESIAN_POINT('Ctrl Pts',(1.7871392867044E-11,-135.43675111262,
9.92453123331945));
#13108=CARTESIAN_POINT('Ctrl Pts',(5.7299307791557,-135.26175111262,9.92453123330913));
#13109=CARTESIAN_POINT('Ctrl Pts',(8.59489616871569,-135.08675111262,4.96226561664425));
#13110=CARTESIAN_POINT('Ctrl Pts',(11.4598615582757,-134.91175111262,-2.06354052510241E-11));
#13111=CARTESIAN_POINT('Ctrl Pts',(8.59489616869782,-134.73675111262,-4.9622656166752));
#13112=CARTESIAN_POINT('Ctrl Pts',(5.72993077911996,-134.56175111262,-9.92453123332976));
#13113=CARTESIAN_POINT('Ctrl Pts',(-1.78726082715848E-11,-134.38675111262,
-9.92453123331945));
#13114=CARTESIAN_POINT('Ctrl Pts',(-5.7299307791557,-134.21175111262,-9.92453123330913));
#13115=CARTESIAN_POINT('Ctrl Pts',(-8.59489616871569,-134.03675111262,-4.96226561664425));
#13116=CARTESIAN_POINT('Ctrl Pts',(-11.4598615582757,-133.86175111262,2.06368086793017E-11));
#13117=CARTESIAN_POINT('Ctrl Pts',(-8.59489616869782,-133.68675111262,4.9622656166752));
#13118=CARTESIAN_POINT('Ctrl Pts',(-5.72993077911996,-133.51175111262,9.92453123332977));
#13119=CARTESIAN_POINT('Ctrl Pts',(1.7871392867044E-11,-133.33675111262,
9.92453123331945));
#13120=CARTESIAN_POINT('Ctrl Pts',(5.7299307791557,-133.16175111262,9.92453123330913));
#13121=CARTESIAN_POINT('Ctrl Pts',(8.59489616871569,-132.98675111262,4.96226561664425));
#13122=CARTESIAN_POINT('Ctrl Pts',(11.4598615582757,-132.81175111262,-2.06354052510241E-11));
#13123=CARTESIAN_POINT('Ctrl Pts',(8.59489616869782,-132.63675111262,-4.9622656166752));
#13124=CARTESIAN_POINT('Ctrl Pts',(5.72993077911996,-132.46175111262,-9.92453123332976));
#13125=CARTESIAN_POINT('Ctrl Pts',(-1.78726082715848E-11,-132.28675111262,
-9.92453123331945));
#13126=CARTESIAN_POINT('Ctrl Pts',(-5.7299307791557,-132.11175111262,-9.92453123330913));
#13127=CARTESIAN_POINT('Ctrl Pts',(-8.59489616871569,-131.93675111262,-4.96226561664425));
#13128=CARTESIAN_POINT('Ctrl Pts',(-11.4598615582757,-131.76175111262,2.06368086793017E-11));
#13129=CARTESIAN_POINT('Ctrl Pts',(-8.59489616869782,-131.58675111262,4.9622656166752));
#13130=CARTESIAN_POINT('Ctrl Pts',(-5.72993077911996,-131.41175111262,9.92453123332977));
#13131=CARTESIAN_POINT('Ctrl Pts',(1.7871392867044E-11,-131.23675111262,
9.92453123331945));
#13132=CARTESIAN_POINT('Ctrl Pts',(5.7299307791557,-131.06175111262,9.92453123330913));
#13133=CARTESIAN_POINT('Ctrl Pts',(8.59489616871569,-130.88675111262,4.96226561664425));
#13134=CARTESIAN_POINT('Ctrl Pts',(11.4598615582757,-130.71175111262,-2.06354052510241E-11));
#13135=CARTESIAN_POINT('Ctrl Pts',(8.59489616869782,-130.53675111262,-4.9622656166752));
#13136=CARTESIAN_POINT('Ctrl Pts',(5.72993077911996,-130.36175111262,-9.92453123332976));
#13137=CARTESIAN_POINT('Ctrl Pts',(-1.78726082715848E-11,-130.18675111262,
-9.92453123331945));
#13138=CARTESIAN_POINT('Ctrl Pts',(-5.7299307791557,-130.01175111262,-9.92453123330913));
#13139=CARTESIAN_POINT('Ctrl Pts',(-8.59489616871569,-129.83675111262,-4.96226561664425));
#13140=CARTESIAN_POINT('Ctrl Pts',(-11.4598615582757,-129.66175111262,2.06368086793017E-11));
#13141=CARTESIAN_POINT('Ctrl Pts',(-8.59489616869782,-129.48675111262,4.9622656166752));
#13142=CARTESIAN_POINT('Ctrl Pts',(-5.72993077911996,-129.31175111262,9.92453123332977));
#13143=CARTESIAN_POINT('Ctrl Pts',(1.7871392867044E-11,-129.13675111262,
9.92453123331945));
#13144=CARTESIAN_POINT('Ctrl Pts',(5.7299307791557,-128.96175111262,9.92453123330913));
#13145=CARTESIAN_POINT('Ctrl Pts',(8.59489616871569,-128.78675111262,4.96226561664425));
#13146=CARTESIAN_POINT('Ctrl Pts',(11.4598615582757,-128.61175111262,-2.06354052510241E-11));
#13147=CARTESIAN_POINT('Ctrl Pts',(8.59489616869782,-128.43675111262,-4.9622656166752));
#13148=CARTESIAN_POINT('Ctrl Pts',(5.72993077911996,-128.26175111262,-9.92453123332976));
#13149=CARTESIAN_POINT('Ctrl Pts',(-1.78726082715848E-11,-128.08675111262,
-9.92453123331945));
#13150=CARTESIAN_POINT('Ctrl Pts',(-5.7299307791557,-127.91175111262,-9.92453123330913));
#13151=CARTESIAN_POINT('Ctrl Pts',(-8.59489616871569,-127.73675111262,-4.96226561664425));
#13152=CARTESIAN_POINT('Ctrl Pts',(-11.4598615582757,-127.56175111262,2.06368086793017E-11));
#13153=CARTESIAN_POINT('Ctrl Pts',(-8.59489616869782,-127.38675111262,4.9622656166752));
#13154=CARTESIAN_POINT('Ctrl Pts',(-5.72993077911996,-127.21175111262,9.92453123332977));
#13155=CARTESIAN_POINT('Ctrl Pts',(1.7871392867044E-11,-127.03675111262,
9.92453123331945));
#13156=CARTESIAN_POINT('Ctrl Pts',(5.7299307791557,-126.86175111262,9.92453123330913));
#13157=CARTESIAN_POINT('Ctrl Pts',(8.59489616871569,-126.68675111262,4.96226561664425));
#13158=CARTESIAN_POINT('Ctrl Pts',(11.4598615582757,-126.51175111262,-2.06354052510241E-11));
#13159=CARTESIAN_POINT('Ctrl Pts',(8.59489616869782,-126.33675111262,-4.9622656166752));
#13160=CARTESIAN_POINT('Ctrl Pts',(5.72993077911996,-126.16175111262,-9.92453123332976));
#13161=CARTESIAN_POINT('Ctrl Pts',(-1.78726082715848E-11,-125.98675111262,
-9.92453123331945));
#13162=CARTESIAN_POINT('Ctrl Pts',(-5.7299307791557,-125.81175111262,-9.92453123330913));
#13163=CARTESIAN_POINT('Ctrl Pts',(-8.59489616871569,-125.63675111262,-4.96226561664425));
#13164=CARTESIAN_POINT('Ctrl Pts',(-11.4598615582757,-125.46175111262,2.06368086793017E-11));
#13165=CARTESIAN_POINT('Ctrl Pts',(-8.59489616869782,-125.28675111262,4.9622656166752));
#13166=CARTESIAN_POINT('Ctrl Pts',(-5.72993077911996,-125.11175111262,9.92453123332977));
#13167=CARTESIAN_POINT('Ctrl Pts',(1.7871392867044E-11,-124.93675111262,
9.92453123331945));
#13168=CARTESIAN_POINT('Ctrl Pts',(5.7299307791557,-124.76175111262,9.92453123330913));
#13169=CARTESIAN_POINT('Ctrl Pts',(8.59489616871569,-124.58675111262,4.96226561664425));
#13170=CARTESIAN_POINT('Ctrl Pts',(11.4598615582757,-124.41175111262,-2.06354052510241E-11));
#13171=CARTESIAN_POINT('Ctrl Pts',(8.59489616869782,-124.23675111262,-4.9622656166752));
#13172=CARTESIAN_POINT('Ctrl Pts',(5.72993077911996,-124.06175111262,-9.92453123332976));
#13173=CARTESIAN_POINT('Ctrl Pts',(-1.78726082715848E-11,-123.88675111262,
-9.92453123331945));
#13174=CARTESIAN_POINT('Ctrl Pts',(-5.7299307791557,-123.71175111262,-9.92453123330913));
#13175=CARTESIAN_POINT('Ctrl Pts',(-8.59489616871569,-123.53675111262,-4.96226561664425));
#13176=CARTESIAN_POINT('Ctrl Pts',(-11.4598615582757,-123.36175111262,2.06368086793017E-11));
#13177=CARTESIAN_POINT('Ctrl Pts',(-8.59489616869782,-123.18675111262,4.9622656166752));
#13178=CARTESIAN_POINT('Ctrl Pts',(-5.72993077911996,-123.01175111262,9.92453123332977));
#13179=CARTESIAN_POINT('Ctrl Pts',(1.7871392867044E-11,-122.83675111262,
9.92453123331945));
#13180=CARTESIAN_POINT('Ctrl Pts',(5.7299307791557,-122.66175111262,9.92453123330913));
#13181=CARTESIAN_POINT('Ctrl Pts',(8.59489616871569,-122.48675111262,4.96226561664425));
#13182=CARTESIAN_POINT('Ctrl Pts',(11.4598615582757,-122.31175111262,-2.06354052510241E-11));
#13183=CARTESIAN_POINT('Ctrl Pts',(8.59489616869782,-122.13675111262,-4.9622656166752));
#13184=CARTESIAN_POINT('Ctrl Pts',(5.72993077911996,-121.96175111262,-9.92453123332976));
#13185=CARTESIAN_POINT('Ctrl Pts',(-1.78726082715848E-11,-121.78675111262,
-9.92453123331945));
#13186=CARTESIAN_POINT('Ctrl Pts',(-5.7299307791557,-121.61175111262,-9.92453123330913));
#13187=CARTESIAN_POINT('Ctrl Pts',(-8.59489616871569,-121.43675111262,-4.96226561664425));
#13188=CARTESIAN_POINT('Ctrl Pts',(-11.4598615582757,-121.26175111262,2.06368086793017E-11));
#13189=CARTESIAN_POINT('Ctrl Pts',(-8.59489616869782,-121.08675111262,4.9622656166752));
#13190=CARTESIAN_POINT('Ctrl Pts',(-5.72993077911996,-120.91175111262,9.92453123332977));
#13191=CARTESIAN_POINT('Ctrl Pts',(1.7871392867044E-11,-120.73675111262,
9.92453123331945));
#13192=CARTESIAN_POINT('Ctrl Pts',(5.7299307791557,-120.56175111262,9.92453123330913));
#13193=CARTESIAN_POINT('Ctrl Pts',(8.59489616871569,-120.38675111262,4.96226561664425));
#13194=CARTESIAN_POINT('Ctrl Pts',(11.4598615582757,-120.21175111262,-2.06354052510241E-11));
#13195=CARTESIAN_POINT('Ctrl Pts',(8.59489616869782,-120.03675111262,-4.9622656166752));
#13196=CARTESIAN_POINT('Ctrl Pts',(5.72993077911996,-119.86175111262,-9.92453123332976));
#13197=CARTESIAN_POINT('Ctrl Pts',(-1.78726082715848E-11,-119.68675111262,
-9.92453123331945));
#13198=CARTESIAN_POINT('Ctrl Pts',(-5.7299307791557,-119.51175111262,-9.92453123330913));
#13199=CARTESIAN_POINT('Ctrl Pts',(-8.59489616871569,-119.33675111262,-4.96226561664425));
#13200=CARTESIAN_POINT('Ctrl Pts',(-11.4598615582757,-119.16175111262,2.06368086793017E-11));
#13201=CARTESIAN_POINT('Ctrl Pts',(-8.59489616869782,-118.98675111262,4.9622656166752));
#13202=CARTESIAN_POINT('Ctrl Pts',(-5.72993077911996,-118.81175111262,9.92453123332977));
#13203=CARTESIAN_POINT('Ctrl Pts',(1.7871392867044E-11,-118.63675111262,
9.92453123331945));
#13204=CARTESIAN_POINT('Ctrl Pts',(5.7299307791557,-118.46175111262,9.92453123330913));
#13205=CARTESIAN_POINT('Ctrl Pts',(8.59489616871569,-118.28675111262,4.96226561664425));
#13206=CARTESIAN_POINT('Ctrl Pts',(11.4598615582757,-118.11175111262,-2.06354052510241E-11));
#13207=CARTESIAN_POINT('Ctrl Pts',(8.59489616869782,-117.93675111262,-4.9622656166752));
#13208=CARTESIAN_POINT('Ctrl Pts',(5.72993077911996,-117.76175111262,-9.92453123332976));
#13209=CARTESIAN_POINT('Ctrl Pts',(-1.78726082715848E-11,-117.58675111262,
-9.92453123331945));
#13210=CARTESIAN_POINT('Ctrl Pts',(-5.7299307791557,-117.41175111262,-9.92453123330913));
#13211=CARTESIAN_POINT('Ctrl Pts',(-8.59489616871569,-117.23675111262,-4.96226561664425));
#13212=CARTESIAN_POINT('Ctrl Pts',(-11.4598615582757,-117.06175111262,2.06368086793017E-11));
#13213=CARTESIAN_POINT('Ctrl Pts',(-8.59489616869782,-116.88675111262,4.9622656166752));
#13214=CARTESIAN_POINT('Ctrl Pts',(-5.72993077911996,-116.71175111262,9.92453123332977));
#13215=CARTESIAN_POINT('Ctrl Pts',(1.7871392867044E-11,-116.53675111262,
9.92453123331945));
#13216=CARTESIAN_POINT('Ctrl Pts',(5.7299307791557,-116.36175111262,9.92453123330913));
#13217=CARTESIAN_POINT('Ctrl Pts',(8.59489616871569,-116.18675111262,4.96226561664425));
#13218=CARTESIAN_POINT('Ctrl Pts',(11.4598615582757,-116.01175111262,-2.06354052510241E-11));
#13219=CARTESIAN_POINT('Ctrl Pts',(8.59489616869782,-115.83675111262,-4.9622656166752));
#13220=CARTESIAN_POINT('Ctrl Pts',(5.72993077911996,-115.66175111262,-9.92453123332976));
#13221=CARTESIAN_POINT('Ctrl Pts',(-1.78726082715848E-11,-115.48675111262,
-9.92453123331945));
#13222=CARTESIAN_POINT('Ctrl Pts',(-5.7299307791557,-115.31175111262,-9.92453123330913));
#13223=CARTESIAN_POINT('Ctrl Pts',(-8.59489616871569,-115.13675111262,-4.96226561664425));
#13224=CARTESIAN_POINT('Ctrl Pts',(-11.4598615582757,-114.96175111262,2.06368086793017E-11));
#13225=CARTESIAN_POINT('Ctrl Pts',(-8.59489616869782,-114.78675111262,4.9622656166752));
#13226=CARTESIAN_POINT('Ctrl Pts',(-5.72993077911996,-114.61175111262,9.92453123332977));
#13227=CARTESIAN_POINT('Ctrl Pts',(1.7871392867044E-11,-114.43675111262,
9.92453123331945));
#13228=CARTESIAN_POINT('Ctrl Pts',(5.7299307791557,-114.26175111262,9.92453123330913));
#13229=CARTESIAN_POINT('Ctrl Pts',(8.59489616871569,-114.08675111262,4.96226561664425));
#13230=CARTESIAN_POINT('Ctrl Pts',(11.4598615582757,-113.91175111262,-2.06354052510241E-11));
#13231=CARTESIAN_POINT('Ctrl Pts',(8.59489616869782,-113.73675111262,-4.9622656166752));
#13232=CARTESIAN_POINT('Ctrl Pts',(5.72993077911996,-113.56175111262,-9.92453123332976));
#13233=CARTESIAN_POINT('Ctrl Pts',(-1.78726082715848E-11,-113.38675111262,
-9.92453123331945));
#13234=CARTESIAN_POINT('Ctrl Pts',(-5.7299307791557,-113.21175111262,-9.92453123330913));
#13235=CARTESIAN_POINT('Ctrl Pts',(-8.59489616871569,-113.03675111262,-4.96226561664425));
#13236=CARTESIAN_POINT('Ctrl Pts',(-11.4598615582757,-112.86175111262,2.06368086793017E-11));
#13237=CARTESIAN_POINT('Ctrl Pts',(-8.59489616869782,-112.68675111262,4.9622656166752));
#13238=CARTESIAN_POINT('Ctrl Pts',(-5.72993077911996,-112.51175111262,9.92453123332977));
#13239=CARTESIAN_POINT('Ctrl Pts',(1.7871392867044E-11,-112.33675111262,
9.92453123331945));
#13240=CARTESIAN_POINT('Ctrl Pts',(5.7299307791557,-112.16175111262,9.92453123330913));
#13241=CARTESIAN_POINT('Ctrl Pts',(8.59489616871569,-111.98675111262,4.96226561664425));
#13242=CARTESIAN_POINT('Ctrl Pts',(11.4598615582757,-111.81175111262,-2.06354052510241E-11));
#13243=CARTESIAN_POINT('Ctrl Pts',(8.59489616869782,-111.63675111262,-4.9622656166752));
#13244=CARTESIAN_POINT('Ctrl Pts',(5.72993077911996,-111.46175111262,-9.92453123332976));
#13245=CARTESIAN_POINT('Ctrl Pts',(-1.78726082715848E-11,-111.28675111262,
-9.92453123331945));
#13246=CARTESIAN_POINT('Ctrl Pts',(-5.7299307791557,-111.11175111262,-9.92453123330913));
#13247=CARTESIAN_POINT('Ctrl Pts',(-8.59489616871569,-110.93675111262,-4.96226561664425));
#13248=CARTESIAN_POINT('Ctrl Pts',(-11.4598615582757,-110.76175111262,2.06368086793017E-11));
#13249=CARTESIAN_POINT('Ctrl Pts',(-8.59489616869782,-110.58675111262,4.9622656166752));
#13250=CARTESIAN_POINT('Ctrl Pts',(-5.72993077911996,-110.41175111262,9.92453123332977));
#13251=CARTESIAN_POINT('Ctrl Pts',(1.7871392867044E-11,-110.23675111262,
9.92453123331945));
#13252=CARTESIAN_POINT('Ctrl Pts',(5.7299307791557,-110.06175111262,9.92453123330913));
#13253=CARTESIAN_POINT('Ctrl Pts',(8.59489616871569,-109.88675111262,4.96226561664425));
#13254=CARTESIAN_POINT('Ctrl Pts',(11.4598615582757,-109.71175111262,-2.06354052510241E-11));
#13255=CARTESIAN_POINT('Ctrl Pts',(8.59489616869782,-109.53675111262,-4.9622656166752));
#13256=CARTESIAN_POINT('Ctrl Pts',(5.72993077911996,-109.36175111262,-9.92453123332976));
#13257=CARTESIAN_POINT('Ctrl Pts',(-1.78726082715848E-11,-109.18675111262,
-9.92453123331945));
#13258=CARTESIAN_POINT('Ctrl Pts',(-5.7299307791557,-109.01175111262,-9.92453123330913));
#13259=CARTESIAN_POINT('Ctrl Pts',(-8.59489616871569,-108.83675111262,-4.96226561664425));
#13260=CARTESIAN_POINT('Ctrl Pts',(-11.4598615582757,-108.66175111262,2.06368086793017E-11));
#13261=CARTESIAN_POINT('Ctrl Pts',(-8.59489616869782,-108.48675111262,4.9622656166752));
#13262=CARTESIAN_POINT('Ctrl Pts',(-5.72993077911996,-108.31175111262,9.92453123332977));
#13263=CARTESIAN_POINT('Ctrl Pts',(1.7871392867044E-11,-108.13675111262,
9.92453123331945));
#13264=CARTESIAN_POINT('Ctrl Pts',(5.7299307791557,-107.96175111262,9.92453123330913));
#13265=CARTESIAN_POINT('Ctrl Pts',(8.59489616871569,-107.78675111262,4.96226561664425));
#13266=CARTESIAN_POINT('Ctrl Pts',(11.4598615582757,-107.61175111262,-2.06354052510241E-11));
#13267=CARTESIAN_POINT('Ctrl Pts',(8.59489616869782,-107.43675111262,-4.9622656166752));
#13268=CARTESIAN_POINT('Ctrl Pts',(5.72993077911996,-107.26175111262,-9.92453123332976));
#13269=CARTESIAN_POINT('Ctrl Pts',(-1.78726082715848E-11,-107.08675111262,
-9.92453123331945));
#13270=CARTESIAN_POINT('Ctrl Pts',(-5.7299307791557,-106.91175111262,-9.92453123330913));
#13271=CARTESIAN_POINT('Ctrl Pts',(-8.59489616871569,-106.73675111262,-4.96226561664425));
#13272=CARTESIAN_POINT('Ctrl Pts',(-11.4598615582757,-106.56175111262,2.06368086793017E-11));
#13273=CARTESIAN_POINT('Ctrl Pts',(-8.59489616869782,-106.38675111262,4.9622656166752));
#13274=CARTESIAN_POINT('Ctrl Pts',(-5.72993077911996,-106.21175111262,9.92453123332977));
#13275=CARTESIAN_POINT('Ctrl Pts',(1.7871392867044E-11,-106.03675111262,
9.92453123331945));
#13276=CARTESIAN_POINT('Ctrl Pts',(5.7299307791557,-105.86175111262,9.92453123330913));
#13277=CARTESIAN_POINT('Ctrl Pts',(8.59489616871569,-105.68675111262,4.96226561664425));
#13278=CARTESIAN_POINT('Ctrl Pts',(11.4598615582757,-105.51175111262,-2.06354052510241E-11));
#13279=CARTESIAN_POINT('Ctrl Pts',(8.59489616869782,-105.33675111262,-4.9622656166752));
#13280=CARTESIAN_POINT('Ctrl Pts',(5.72993077911996,-105.16175111262,-9.92453123332976));
#13281=CARTESIAN_POINT('Ctrl Pts',(-1.78726082715848E-11,-104.98675111262,
-9.92453123331945));
#13282=CARTESIAN_POINT('Ctrl Pts',(-5.7299307791557,-104.81175111262,-9.92453123330913));
#13283=CARTESIAN_POINT('Ctrl Pts',(-8.59489616871569,-104.63675111262,-4.96226561664425));
#13284=CARTESIAN_POINT('Ctrl Pts',(-11.4598615582757,-104.46175111262,2.06368086793017E-11));
#13285=CARTESIAN_POINT('Ctrl Pts',(-8.59489616869782,-104.28675111262,4.9622656166752));
#13286=CARTESIAN_POINT('Ctrl Pts',(-5.72993077911996,-104.11175111262,9.92453123332977));
#13287=CARTESIAN_POINT('Ctrl Pts',(1.7871392867044E-11,-103.93675111262,
9.92453123331945));
#13288=CARTESIAN_POINT('Ctrl Pts',(5.7299307791557,-103.76175111262,9.92453123330913));
#13289=CARTESIAN_POINT('Ctrl Pts',(8.59489616871569,-103.58675111262,4.96226561664425));
#13290=CARTESIAN_POINT('Ctrl Pts',(11.4598615582757,-103.41175111262,-2.06354052510241E-11));
#13291=CARTESIAN_POINT('Ctrl Pts',(8.59489616869782,-103.23675111262,-4.9622656166752));
#13292=CARTESIAN_POINT('Ctrl Pts',(5.72993077911996,-103.06175111262,-9.92453123332976));
#13293=CARTESIAN_POINT('Ctrl Pts',(-1.78726082715848E-11,-102.88675111262,
-9.92453123331945));
#13294=CARTESIAN_POINT('Ctrl Pts',(-5.7299307791557,-102.71175111262,-9.92453123330913));
#13295=CARTESIAN_POINT('Ctrl Pts',(-8.59489616871569,-102.53675111262,-4.96226561664425));
#13296=CARTESIAN_POINT('Ctrl Pts',(-11.4598615582757,-102.36175111262,2.06368086793017E-11));
#13297=CARTESIAN_POINT('Ctrl Pts',(-8.59489616869782,-102.18675111262,4.9622656166752));
#13298=CARTESIAN_POINT('Ctrl Pts',(-5.72993077911996,-102.01175111262,9.92453123332977));
#13299=CARTESIAN_POINT('Ctrl Pts',(1.7871392867044E-11,-101.83675111262,
9.92453123331945));
#13300=CARTESIAN_POINT('Ctrl Pts',(5.7299307791557,-101.66175111262,9.92453123330913));
#13301=CARTESIAN_POINT('Ctrl Pts',(8.59489616871569,-101.48675111262,4.96226561664425));
#13302=CARTESIAN_POINT('Ctrl Pts',(11.4598615582757,-101.31175111262,-2.06354052510241E-11));
#13303=CARTESIAN_POINT('Ctrl Pts',(8.59489616869782,-101.13675111262,-4.9622656166752));
#13304=CARTESIAN_POINT('Ctrl Pts',(5.72993077911996,-100.96175111262,-9.92453123332976));
#13305=CARTESIAN_POINT('Ctrl Pts',(-1.78726082715848E-11,-100.78675111262,
-9.92453123331945));
#13306=CARTESIAN_POINT('Ctrl Pts',(-5.7299307791557,-100.61175111262,-9.92453123330913));
#13307=CARTESIAN_POINT('Ctrl Pts',(-8.59489616871569,-100.43675111262,-4.96226561664425));
#13308=CARTESIAN_POINT('Ctrl Pts',(-11.4598615582757,-100.26175111262,2.06368086793017E-11));
#13309=CARTESIAN_POINT('Ctrl Pts',(-8.59489616869782,-100.08675111262,4.9622656166752));
#13310=CARTESIAN_POINT('Ctrl Pts',(-5.72993077911996,-99.91175111262,9.92453123332977));
#13311=CARTESIAN_POINT('Ctrl Pts',(1.7871392867044E-11,-99.7367511126201,
9.92453123331945));
#13312=CARTESIAN_POINT('Ctrl Pts',(5.7299307791557,-99.5617511126201,9.92453123330913));
#13313=CARTESIAN_POINT('Ctrl Pts',(8.59489616871569,-99.3867511126201,4.96226561664425));
#13314=CARTESIAN_POINT('Ctrl Pts',(11.4598615582757,-99.2117511126201,-2.06354052510241E-11));
#13315=CARTESIAN_POINT('Ctrl Pts',(8.59489616869782,-99.0367511126201,-4.9622656166752));
#13316=CARTESIAN_POINT('Ctrl Pts',(5.72993077911996,-98.8617511126201,-9.92453123332976));
#13317=CARTESIAN_POINT('Ctrl Pts',(-1.78726082715848E-11,-98.6867511126201,
-9.92453123331945));
#13318=CARTESIAN_POINT('Ctrl Pts',(-5.7299307791557,-98.5117511126201,-9.92453123330913));
#13319=CARTESIAN_POINT('Ctrl Pts',(-8.59489616871569,-98.33675111262,-4.96226561664425));
#13320=CARTESIAN_POINT('Ctrl Pts',(-11.4598615582757,-98.16175111262,2.06368086793017E-11));
#13321=CARTESIAN_POINT('Ctrl Pts',(-8.59489616869782,-97.9867511126201,
4.9622656166752));
#13322=CARTESIAN_POINT('Ctrl Pts',(-5.72993077911996,-97.81175111262,9.92453123332977));
#13323=CARTESIAN_POINT('Ctrl Pts',(1.7871392867044E-11,-97.6367511126201,
9.92453123331945));
#13324=CARTESIAN_POINT('Ctrl Pts',(5.7299307791557,-97.46175111262,9.92453123330913));
#13325=CARTESIAN_POINT('Ctrl Pts',(8.59489616871569,-97.2867511126201,4.96226561664425));
#13326=CARTESIAN_POINT('Ctrl Pts',(11.4598615582757,-97.1117511126201,-2.06354052510241E-11));
#13327=CARTESIAN_POINT('Ctrl Pts',(8.59489616869782,-96.9367511126201,-4.9622656166752));
#13328=CARTESIAN_POINT('Ctrl Pts',(5.72993077911996,-96.7617511126201,-9.92453123332976));
#13329=CARTESIAN_POINT('Ctrl Pts',(-1.78726082715848E-11,-96.5867511126201,
-9.92453123331945));
#13330=CARTESIAN_POINT('Ctrl Pts',(-5.7299307791557,-96.4117511126201,-9.92453123330913));
#13331=CARTESIAN_POINT('Ctrl Pts',(-8.59489616871569,-96.2367511126201,
-4.96226561664425));
#13332=CARTESIAN_POINT('Ctrl Pts',(-11.4598615582757,-96.0617511126201,
2.06368086793017E-11));
#13333=CARTESIAN_POINT('Ctrl Pts',(-8.59489616869782,-95.8867511126201,
4.9622656166752));
#13334=CARTESIAN_POINT('Ctrl Pts',(-5.72993077911996,-95.7117511126201,
9.92453123332977));
#13335=CARTESIAN_POINT('Ctrl Pts',(1.7871392867044E-11,-95.5367511126201,
9.92453123331945));
#13336=CARTESIAN_POINT('Ctrl Pts',(5.7299307791557,-95.3617511126201,9.92453123330913));
#13337=CARTESIAN_POINT('Ctrl Pts',(8.59489616871569,-95.1867511126201,4.96226561664425));
#13338=CARTESIAN_POINT('Ctrl Pts',(11.4598615582757,-95.0117511126201,-2.06354052510241E-11));
#13339=CARTESIAN_POINT('Ctrl Pts',(8.59489616869782,-94.83675111262,-4.9622656166752));
#13340=CARTESIAN_POINT('Ctrl Pts',(5.72993077911996,-94.6617511126201,-9.92453123332976));
#13341=CARTESIAN_POINT('Ctrl Pts',(-1.78726082715848E-11,-94.4867511126201,
-9.92453123331945));
#13342=CARTESIAN_POINT('Ctrl Pts',(-5.7299307791557,-94.3117511126201,-9.92453123330913));
#13343=CARTESIAN_POINT('Ctrl Pts',(-8.59489616871569,-94.1367511126201,
-4.96226561664425));
#13344=CARTESIAN_POINT('Ctrl Pts',(-11.4598615582757,-93.9617511126201,
2.06368086793017E-11));
#13345=CARTESIAN_POINT('Ctrl Pts',(-8.59489616869782,-93.7867511126201,
4.9622656166752));
#13346=CARTESIAN_POINT('Ctrl Pts',(-5.72993077911996,-93.6117511126201,
9.92453123332977));
#13347=CARTESIAN_POINT('Ctrl Pts',(1.7871392867044E-11,-93.4367511126201,
9.92453123331945));
#13348=CARTESIAN_POINT('Ctrl Pts',(5.7299307791557,-93.26175111262,9.92453123330913));
#13349=CARTESIAN_POINT('Ctrl Pts',(8.59489616871569,-93.0867511126201,4.96226561664425));
#13350=CARTESIAN_POINT('Ctrl Pts',(11.4598615582757,-92.9117511126201,-2.06354052510241E-11));
#13351=CARTESIAN_POINT('Ctrl Pts',(8.59489616869782,-92.7367511126201,-4.9622656166752));
#13352=CARTESIAN_POINT('Ctrl Pts',(5.72993077911996,-92.5617511126201,-9.92453123332976));
#13353=CARTESIAN_POINT('Ctrl Pts',(-1.78726082715848E-11,-92.3867511126201,
-9.92453123331945));
#13354=CARTESIAN_POINT('Ctrl Pts',(-5.7299307791557,-92.2117511126201,-9.92453123330913));
#13355=CARTESIAN_POINT('Ctrl Pts',(-8.59489616871569,-92.0367511126201,
-4.96226561664425));
#13356=CARTESIAN_POINT('Ctrl Pts',(-11.4598615582757,-91.8617511126201,
2.06368086793017E-11));
#13357=CARTESIAN_POINT('Ctrl Pts',(-8.59489616869782,-91.6867511126201,
4.9622656166752));
#13358=CARTESIAN_POINT('Ctrl Pts',(-5.72993077911996,-91.5117511126201,
9.92453123332977));
#13359=CARTESIAN_POINT('Ctrl Pts',(1.7871392867044E-11,-91.3367511126201,
9.92453123331945));
#13360=CARTESIAN_POINT('Ctrl Pts',(5.7299307791557,-91.1617511126201,9.92453123330913));
#13361=CARTESIAN_POINT('Ctrl Pts',(8.59489616871569,-90.9867511126201,4.96226561664425));
#13362=CARTESIAN_POINT('Ctrl Pts',(11.4598615582757,-90.8117511126201,-2.06354052510241E-11));
#13363=CARTESIAN_POINT('Ctrl Pts',(8.59489616869782,-90.6367511126201,-4.9622656166752));
#13364=CARTESIAN_POINT('Ctrl Pts',(5.72993077911996,-90.4617511126201,-9.92453123332976));
#13365=CARTESIAN_POINT('Ctrl Pts',(-1.78726082715848E-11,-90.2867511126201,
-9.92453123331945));
#13366=CARTESIAN_POINT('Ctrl Pts',(-5.7299307791557,-90.1117511126201,-9.92453123330913));
#13367=CARTESIAN_POINT('Ctrl Pts',(-8.59489616871569,-89.9367511126201,
-4.96226561664425));
#13368=CARTESIAN_POINT('Ctrl Pts',(-11.4598615582757,-89.7617511126201,
2.06368086793017E-11));
#13369=CARTESIAN_POINT('Ctrl Pts',(-8.59489616869782,-89.5867511126201,
4.9622656166752));
#13370=CARTESIAN_POINT('Ctrl Pts',(-5.72993077911996,-89.4117511126201,
9.92453123332977));
#13371=CARTESIAN_POINT('Ctrl Pts',(1.7871392867044E-11,-89.2367511126201,
9.92453123331945));
#13372=CARTESIAN_POINT('Ctrl Pts',(5.7299307791557,-89.0617511126201,9.92453123330913));
#13373=CARTESIAN_POINT('Ctrl Pts',(8.59489616871569,-88.8867511126201,4.96226561664425));
#13374=CARTESIAN_POINT('Ctrl Pts',(11.4598615582757,-88.7117511126201,-2.06354052510241E-11));
#13375=CARTESIAN_POINT('Ctrl Pts',(8.59489616869782,-88.5367511126201,-4.9622656166752));
#13376=CARTESIAN_POINT('Ctrl Pts',(5.72993077911996,-88.3617511126201,-9.92453123332976));
#13377=CARTESIAN_POINT('Ctrl Pts',(-1.78726082715848E-11,-88.1867511126201,
-9.92453123331945));
#13378=CARTESIAN_POINT('Ctrl Pts',(-5.7299307791557,-88.0117511126201,-9.92453123330913));
#13379=CARTESIAN_POINT('Ctrl Pts',(-8.59489616871569,-87.8367511126201,
-4.96226561664425));
#13380=CARTESIAN_POINT('Ctrl Pts',(-11.4598615582757,-87.6617511126201,
2.06368086793017E-11));
#13381=CARTESIAN_POINT('Ctrl Pts',(-8.59489616869782,-87.4867511126201,
4.9622656166752));
#13382=CARTESIAN_POINT('Ctrl Pts',(-5.72993077911996,-87.3117511126201,
9.92453123332977));
#13383=CARTESIAN_POINT('Ctrl Pts',(1.7871392867044E-11,-87.1367511126201,
9.92453123331945));
#13384=CARTESIAN_POINT('Ctrl Pts',(5.7299307791557,-86.9617511126201,9.92453123330913));
#13385=CARTESIAN_POINT('Ctrl Pts',(8.59489616871569,-86.7867511126201,4.96226561664425));
#13386=CARTESIAN_POINT('Ctrl Pts',(11.4598615582757,-86.6117511126201,-2.06354052510241E-11));
#13387=CARTESIAN_POINT('Ctrl Pts',(8.59489616869782,-86.4367511126201,-4.9622656166752));
#13388=CARTESIAN_POINT('Ctrl Pts',(5.72993077911996,-86.2617511126201,-9.92453123332976));
#13389=CARTESIAN_POINT('Ctrl Pts',(-1.78726082715848E-11,-86.0867511126201,
-9.92453123331945));
#13390=CARTESIAN_POINT('Ctrl Pts',(-5.7299307791557,-85.9117511126201,-9.92453123330913));
#13391=CARTESIAN_POINT('Ctrl Pts',(-8.59489616871569,-85.7367511126201,
-4.96226561664425));
#13392=CARTESIAN_POINT('Ctrl Pts',(-11.4598615582757,-85.5617511126201,
2.06368086793017E-11));
#13393=CARTESIAN_POINT('Ctrl Pts',(-8.59489616869782,-85.3867511126201,
4.9622656166752));
#13394=CARTESIAN_POINT('Ctrl Pts',(-5.72993077911996,-85.2117511126201,
9.92453123332977));
#13395=CARTESIAN_POINT('Ctrl Pts',(1.7871392867044E-11,-85.0367511126201,
9.92453123331945));
#13396=CARTESIAN_POINT('Ctrl Pts',(5.7299307791557,-84.8617511126201,9.92453123330913));
#13397=CARTESIAN_POINT('Ctrl Pts',(8.59489616871569,-84.6867511126201,4.96226561664425));
#13398=CARTESIAN_POINT('Ctrl Pts',(11.4598615582757,-84.5117511126201,-2.06354052510241E-11));
#13399=CARTESIAN_POINT('Ctrl Pts',(8.59489616869782,-84.3367511126201,-4.9622656166752));
#13400=CARTESIAN_POINT('Ctrl Pts',(5.72993077911996,-84.1617511126201,-9.92453123332976));
#13401=CARTESIAN_POINT('Ctrl Pts',(-1.78726082715848E-11,-83.9867511126201,
-9.92453123331945));
#13402=CARTESIAN_POINT('Ctrl Pts',(-5.7299307791557,-83.8117511126201,-9.92453123330913));
#13403=CARTESIAN_POINT('Ctrl Pts',(-8.59489616871569,-83.6367511126201,
-4.96226561664425));
#13404=CARTESIAN_POINT('Ctrl Pts',(-11.4598615582757,-83.4617511126201,
2.06368086793017E-11));
#13405=CARTESIAN_POINT('Ctrl Pts',(-8.59489616869782,-83.2867511126201,
4.9622656166752));
#13406=CARTESIAN_POINT('Ctrl Pts',(-5.72993077911996,-83.1117511126201,
9.92453123332977));
#13407=CARTESIAN_POINT('Ctrl Pts',(1.7871392867044E-11,-82.9367511126201,
9.92453123331945));
#13408=CARTESIAN_POINT('Ctrl Pts',(5.7299307791557,-82.7617511126201,9.92453123330913));
#13409=CARTESIAN_POINT('Ctrl Pts',(8.59489616871569,-82.5867511126201,4.96226561664425));
#13410=CARTESIAN_POINT('Ctrl Pts',(11.4598615582757,-82.4117511126201,-2.06354052510241E-11));
#13411=CARTESIAN_POINT('Ctrl Pts',(8.59489616869782,-82.2367511126201,-4.9622656166752));
#13412=CARTESIAN_POINT('Ctrl Pts',(5.72993077911996,-82.0617511126201,-9.92453123332976));
#13413=CARTESIAN_POINT('Ctrl Pts',(-1.78726082715848E-11,-81.8867511126201,
-9.92453123331945));
#13414=CARTESIAN_POINT('Ctrl Pts',(-5.7299307791557,-81.7117511126201,-9.92453123330913));
#13415=CARTESIAN_POINT('Ctrl Pts',(-8.59489616871569,-81.5367511126201,
-4.96226561664425));
#13416=CARTESIAN_POINT('Ctrl Pts',(-11.4598615582757,-81.3617511126201,
2.06368086793017E-11));
#13417=CARTESIAN_POINT('Ctrl Pts',(-8.59489616869782,-81.1867511126201,
4.9622656166752));
#13418=CARTESIAN_POINT('Ctrl Pts',(-5.72993077911996,-81.0117511126201,
9.92453123332977));
#13419=CARTESIAN_POINT('Ctrl Pts',(1.7871392867044E-11,-80.8367511126201,
9.92453123331945));
#13420=CARTESIAN_POINT('Ctrl Pts',(5.7299307791557,-80.6617511126201,9.92453123330913));
#13421=CARTESIAN_POINT('Ctrl Pts',(8.59489616871569,-80.4867511126201,4.96226561664425));
#13422=CARTESIAN_POINT('Ctrl Pts',(11.4598615582757,-80.3117511126201,-2.06354052510241E-11));
#13423=CARTESIAN_POINT('Ctrl Pts',(8.59489616869782,-80.1367511126201,-4.9622656166752));
#13424=CARTESIAN_POINT('Ctrl Pts',(5.72993077911996,-79.9617511126201,-9.92453123332976));
#13425=CARTESIAN_POINT('Ctrl Pts',(-1.78726082715848E-11,-79.7867511126201,
-9.92453123331945));
#13426=CARTESIAN_POINT('Ctrl Pts',(-5.7299307791557,-79.6117511126201,-9.92453123330913));
#13427=CARTESIAN_POINT('Ctrl Pts',(-8.59489616871569,-79.4367511126201,
-4.96226561664425));
#13428=CARTESIAN_POINT('Ctrl Pts',(-11.4598615582757,-79.2617511126201,
2.06368086793017E-11));
#13429=CARTESIAN_POINT('Ctrl Pts',(-8.59489616869782,-79.0867511126201,
4.9622656166752));
#13430=CARTESIAN_POINT('Ctrl Pts',(-5.72993077911996,-78.9117511126201,
9.92453123332977));
#13431=CARTESIAN_POINT('Ctrl Pts',(1.7871392867044E-11,-78.7367511126201,
9.92453123331945));
#13432=CARTESIAN_POINT('Ctrl Pts',(5.7299307791557,-78.5617511126201,9.92453123330913));
#13433=CARTESIAN_POINT('Ctrl Pts',(8.59489616871569,-78.3867511126201,4.96226561664425));
#13434=CARTESIAN_POINT('Ctrl Pts',(11.4598615582757,-78.2117511126201,-2.06354052510241E-11));
#13435=CARTESIAN_POINT('Ctrl Pts',(8.59489616869782,-78.0367511126201,-4.9622656166752));
#13436=CARTESIAN_POINT('Ctrl Pts',(5.72993077911996,-77.8617511126201,-9.92453123332976));
#13437=CARTESIAN_POINT('Ctrl Pts',(-1.78726082715848E-11,-77.6867511126201,
-9.92453123331945));
#13438=CARTESIAN_POINT('Ctrl Pts',(-5.7299307791557,-77.5117511126201,-9.92453123330913));
#13439=CARTESIAN_POINT('Ctrl Pts',(-8.59489616871569,-77.3367511126201,
-4.96226561664425));
#13440=CARTESIAN_POINT('Ctrl Pts',(-11.4598615582757,-77.1617511126201,
2.06368086793017E-11));
#13441=CARTESIAN_POINT('Ctrl Pts',(-8.59489616869782,-76.9867511126201,
4.9622656166752));
#13442=CARTESIAN_POINT('Ctrl Pts',(-5.72993077911996,-76.8117511126201,
9.92453123332977));
#13443=CARTESIAN_POINT('Ctrl Pts',(1.7871392867044E-11,-76.6367511126201,
9.92453123331945));
#13444=CARTESIAN_POINT('Ctrl Pts',(5.7299307791557,-76.4617511126201,9.92453123330913));
#13445=CARTESIAN_POINT('Ctrl Pts',(8.59489616871569,-76.2867511126201,4.96226561664425));
#13446=CARTESIAN_POINT('Ctrl Pts',(11.4598615582757,-76.1117511126201,-2.06354052510241E-11));
#13447=CARTESIAN_POINT('Ctrl Pts',(8.59489616869782,-75.9367511126201,-4.9622656166752));
#13448=CARTESIAN_POINT('Ctrl Pts',(5.72993077911996,-75.7617511126201,-9.92453123332976));
#13449=CARTESIAN_POINT('Ctrl Pts',(-1.78726082715848E-11,-75.5867511126201,
-9.92453123331945));
#13450=CARTESIAN_POINT('Ctrl Pts',(-5.7299307791557,-75.4117511126201,-9.92453123330913));
#13451=CARTESIAN_POINT('Ctrl Pts',(-8.59489616871569,-75.2367511126201,
-4.96226561664425));
#13452=CARTESIAN_POINT('Ctrl Pts',(-11.4598615582757,-75.0617511126201,
2.06368086793017E-11));
#13453=CARTESIAN_POINT('Ctrl Pts',(-8.59489616869782,-74.8867511126201,
4.9622656166752));
#13454=CARTESIAN_POINT('Ctrl Pts',(-5.72993077911996,-74.7117511126201,
9.92453123332977));
#13455=CARTESIAN_POINT('Ctrl Pts',(1.7871392867044E-11,-74.5367511126201,
9.92453123331945));
#13456=CARTESIAN_POINT('Ctrl Pts',(5.7299307791557,-74.3617511126201,9.92453123330913));
#13457=CARTESIAN_POINT('Ctrl Pts',(8.59489616871569,-74.1867511126201,4.96226561664425));
#13458=CARTESIAN_POINT('Ctrl Pts',(11.4598615582757,-74.0117511126201,-2.06354052510241E-11));
#13459=CARTESIAN_POINT('Ctrl Pts',(8.59489616869782,-73.8367511126201,-4.9622656166752));
#13460=CARTESIAN_POINT('Ctrl Pts',(5.72993077911996,-73.6617511126201,-9.92453123332976));
#13461=CARTESIAN_POINT('Ctrl Pts',(-1.78726082715848E-11,-73.4867511126201,
-9.92453123331945));
#13462=CARTESIAN_POINT('Ctrl Pts',(-5.7299307791557,-73.3117511126201,-9.92453123330913));
#13463=CARTESIAN_POINT('Ctrl Pts',(-8.59489616871569,-73.1367511126201,
-4.96226561664425));
#13464=CARTESIAN_POINT('Ctrl Pts',(-11.4598615582757,-72.9617511126201,
2.06368086793017E-11));
#13465=CARTESIAN_POINT('Ctrl Pts',(-8.59489616869782,-72.7867511126201,
4.9622656166752));
#13466=CARTESIAN_POINT('Ctrl Pts',(-5.72993077911996,-72.6117511126201,
9.92453123332977));
#13467=CARTESIAN_POINT('Ctrl Pts',(1.7871392867044E-11,-72.4367511126201,
9.92453123331945));
#13468=CARTESIAN_POINT('Ctrl Pts',(5.7299307791557,-72.2617511126201,9.92453123330913));
#13469=CARTESIAN_POINT('Ctrl Pts',(8.59489616871569,-72.0867511126201,4.96226561664425));
#13470=CARTESIAN_POINT('Ctrl Pts',(11.4598615582757,-71.9117511126201,-2.06354052510241E-11));
#13471=CARTESIAN_POINT('Ctrl Pts',(8.59489616869782,-71.7367511126201,-4.9622656166752));
#13472=CARTESIAN_POINT('Ctrl Pts',(5.72993077911996,-71.5617511126201,-9.92453123332976));
#13473=CARTESIAN_POINT('Ctrl Pts',(-1.78726082715848E-11,-71.3867511126201,
-9.92453123331945));
#13474=CARTESIAN_POINT('Ctrl Pts',(-5.7299307791557,-71.2117511126201,-9.92453123330913));
#13475=CARTESIAN_POINT('Ctrl Pts',(-8.59489616871569,-71.0367511126201,
-4.96226561664425));
#13476=CARTESIAN_POINT('Ctrl Pts',(-11.4598615582757,-70.8617511126201,
2.06368086793017E-11));
#13477=CARTESIAN_POINT('Ctrl Pts',(-8.59489616869782,-70.6867511126201,
4.9622656166752));
#13478=CARTESIAN_POINT('Ctrl Pts',(-5.72993077911996,-70.5117511126201,
9.92453123332977));
#13479=CARTESIAN_POINT('Ctrl Pts',(1.7871392867044E-11,-70.3367511126201,
9.92453123331945));
#13480=CARTESIAN_POINT('Ctrl Pts',(5.7299307791557,-70.1617511126201,9.92453123330913));
#13481=CARTESIAN_POINT('Ctrl Pts',(8.59489616871569,-69.9867511126201,4.96226561664425));
#13482=CARTESIAN_POINT('Ctrl Pts',(11.4598615582757,-69.8117511126202,-2.06354052510241E-11));
#13483=CARTESIAN_POINT('Ctrl Pts',(8.59489616869782,-69.6367511126201,-4.9622656166752));
#13484=CARTESIAN_POINT('Ctrl Pts',(5.72993077911996,-69.4617511126201,-9.92453123332976));
#13485=CARTESIAN_POINT('Ctrl Pts',(-1.78726082715848E-11,-69.2867511126201,
-9.92453123331945));
#13486=CARTESIAN_POINT('Ctrl Pts',(-5.7299307791557,-69.1117511126201,-9.92453123330913));
#13487=CARTESIAN_POINT('Ctrl Pts',(-8.59489616871569,-68.9367511126201,
-4.96226561664425));
#13488=CARTESIAN_POINT('Ctrl Pts',(-11.4598615582757,-68.7617511126201,
2.06368086793017E-11));
#13489=CARTESIAN_POINT('Ctrl Pts',(-8.59489616869782,-68.5867511126201,
4.9622656166752));
#13490=CARTESIAN_POINT('Ctrl Pts',(-5.72993077911996,-68.4117511126201,
9.92453123332977));
#13491=CARTESIAN_POINT('Ctrl Pts',(1.7871392867044E-11,-68.2367511126201,
9.92453123331945));
#13492=CARTESIAN_POINT('Ctrl Pts',(5.7299307791557,-68.0617511126201,9.92453123330913));
#13493=CARTESIAN_POINT('Ctrl Pts',(8.59489616871569,-67.8867511126201,4.96226561664425));
#13494=CARTESIAN_POINT('Ctrl Pts',(11.4598615582757,-67.7117511126201,-2.06354052510241E-11));
#13495=CARTESIAN_POINT('Ctrl Pts',(8.59489616869782,-67.5367511126201,-4.9622656166752));
#13496=CARTESIAN_POINT('Ctrl Pts',(5.72993077911996,-67.3617511126201,-9.92453123332976));
#13497=CARTESIAN_POINT('Ctrl Pts',(-1.78726082715848E-11,-67.1867511126201,
-9.92453123331945));
#13498=CARTESIAN_POINT('Ctrl Pts',(-5.7299307791557,-67.0117511126201,-9.92453123330913));
#13499=CARTESIAN_POINT('Ctrl Pts',(-8.59489616871569,-66.8367511126201,
-4.96226561664425));
#13500=CARTESIAN_POINT('Ctrl Pts',(-11.4598615582757,-66.6617511126201,
2.06368086793017E-11));
#13501=CARTESIAN_POINT('Ctrl Pts',(-8.59489616869782,-66.4867511126201,
4.9622656166752));
#13502=CARTESIAN_POINT('Ctrl Pts',(-5.72993077911996,-66.3117511126201,
9.92453123332977));
#13503=CARTESIAN_POINT('Ctrl Pts',(1.7871392867044E-11,-66.1367511126201,
9.92453123331945));
#13504=CARTESIAN_POINT('Ctrl Pts',(5.7299307791557,-65.9617511126201,9.92453123330913));
#13505=CARTESIAN_POINT('Ctrl Pts',(8.59489616871569,-65.7867511126201,4.96226561664425));
#13506=CARTESIAN_POINT('Ctrl Pts',(11.4598615582757,-65.6117511126201,-2.06354052510241E-11));
#13507=CARTESIAN_POINT('Ctrl Pts',(8.59489616869782,-65.4367511126201,-4.9622656166752));
#13508=CARTESIAN_POINT('Ctrl Pts',(5.72993077911996,-65.2617511126201,-9.92453123332976));
#13509=CARTESIAN_POINT('Ctrl Pts',(-1.78726082715848E-11,-65.0867511126201,
-9.92453123331945));
#13510=CARTESIAN_POINT('Ctrl Pts',(-5.7299307791557,-64.9117511126201,-9.92453123330913));
#13511=CARTESIAN_POINT('Ctrl Pts',(-8.59489616871569,-64.7367511126201,
-4.96226561664425));
#13512=CARTESIAN_POINT('Ctrl Pts',(-11.4598615582757,-64.5617511126202,
2.06368086793017E-11));
#13513=CARTESIAN_POINT('Ctrl Pts',(-8.59489616869782,-64.3867511126201,
4.9622656166752));
#13514=CARTESIAN_POINT('Ctrl Pts',(-5.72993077911996,-64.2117511126201,
9.92453123332977));
#13515=CARTESIAN_POINT('Ctrl Pts',(1.7871392867044E-11,-64.0367511126202,
9.92453123331945));
#13516=CARTESIAN_POINT('Ctrl Pts',(5.7299307791557,-63.8617511126201,9.92453123330913));
#13517=CARTESIAN_POINT('Ctrl Pts',(8.59489616871569,-63.6867511126202,4.96226561664425));
#13518=CARTESIAN_POINT('Ctrl Pts',(11.4598615582757,-63.5117511126202,-2.06354052510241E-11));
#13519=CARTESIAN_POINT('Ctrl Pts',(8.59489616869782,-63.3367511126201,-4.9622656166752));
#13520=CARTESIAN_POINT('Ctrl Pts',(5.72993077911996,-63.1617511126202,-9.92453123332976));
#13521=CARTESIAN_POINT('Ctrl Pts',(-1.78726082715848E-11,-62.9867511126201,
-9.92453123331945));
#13522=CARTESIAN_POINT('Ctrl Pts',(-5.7299307791557,-62.8117511126201,-9.92453123330913));
#13523=CARTESIAN_POINT('Ctrl Pts',(-8.59489616871569,-62.6367511126202,
-4.96226561664425));
#13524=CARTESIAN_POINT('Ctrl Pts',(-11.4598615582757,-62.4617511126202,
2.06368086793017E-11));
#13525=CARTESIAN_POINT('Ctrl Pts',(-8.59489616869782,-62.2867511126201,
4.9622656166752));
#13526=CARTESIAN_POINT('Ctrl Pts',(-5.72993077911996,-62.1117511126202,
9.92453123332977));
#13527=CARTESIAN_POINT('Ctrl Pts',(1.7871392867044E-11,-61.9367511126202,
9.92453123331945));
#13528=CARTESIAN_POINT('Ctrl Pts',(5.7299307791557,-61.7617511126201,9.92453123330913));
#13529=CARTESIAN_POINT('Ctrl Pts',(8.59489616871569,-61.5867511126202,4.96226561664425));
#13530=CARTESIAN_POINT('Ctrl Pts',(11.4598615582757,-61.4117511126202,-2.06354052510241E-11));
#13531=CARTESIAN_POINT('Ctrl Pts',(8.59489616869782,-61.2367511126201,-4.9622656166752));
#13532=CARTESIAN_POINT('Ctrl Pts',(5.72993077911996,-61.0617511126202,-9.92453123332976));
#13533=CARTESIAN_POINT('Ctrl Pts',(-1.78726082715848E-11,-60.8867511126202,
-9.92453123331945));
#13534=CARTESIAN_POINT('Ctrl Pts',(-5.7299307791557,-60.7117511126201,-9.92453123330913));
#13535=CARTESIAN_POINT('Ctrl Pts',(-8.59489616871569,-60.5367511126202,
-4.96226561664425));
#13536=CARTESIAN_POINT('Ctrl Pts',(-11.4598615582757,-60.3617511126201,
2.06368086793017E-11));
#13537=CARTESIAN_POINT('Ctrl Pts',(-8.59489616869782,-60.1867511126201,
4.9622656166752));
#13538=CARTESIAN_POINT('Ctrl Pts',(-5.72993077911996,-60.0117511126202,
9.92453123332977));
#13539=CARTESIAN_POINT('Ctrl Pts',(1.7871392867044E-11,-59.8367511126201,
9.92453123331945));
#13540=CARTESIAN_POINT('Ctrl Pts',(5.7299307791557,-59.6617511126202,9.92453123330913));
#13541=CARTESIAN_POINT('Ctrl Pts',(8.59489616871569,-59.4867511126202,4.96226561664425));
#13542=CARTESIAN_POINT('Ctrl Pts',(11.4598615582757,-59.3117511126202,-2.06354052510241E-11));
#13543=CARTESIAN_POINT('Ctrl Pts',(8.59489616869782,-59.1367511126202,-4.9622656166752));
#13544=CARTESIAN_POINT('Ctrl Pts',(5.72993077911996,-58.9617511126202,-9.92453123332976));
#13545=CARTESIAN_POINT('Ctrl Pts',(-1.78726082715848E-11,-58.7867511126201,
-9.92453123331945));
#13546=CARTESIAN_POINT('Ctrl Pts',(-5.7299307791557,-58.6117511126201,-9.92453123330913));
#13547=CARTESIAN_POINT('Ctrl Pts',(-8.59489616871569,-58.4367511126202,
-4.96226561664425));
#13548=CARTESIAN_POINT('Ctrl Pts',(-11.4598615582757,-58.2617511126201,
2.06368086793017E-11));
#13549=CARTESIAN_POINT('Ctrl Pts',(-8.59489616869782,-58.0867511126202,
4.9622656166752));
#13550=CARTESIAN_POINT('Ctrl Pts',(-5.72993077911996,-57.9117511126202,
9.92453123332977));
#13551=CARTESIAN_POINT('Ctrl Pts',(1.7871392867044E-11,-57.7367511126201,
9.92453123331945));
#13552=CARTESIAN_POINT('Ctrl Pts',(5.7299307791557,-57.5617511126202,9.92453123330913));
#13553=CARTESIAN_POINT('Ctrl Pts',(8.59489616871569,-57.3867511126202,4.96226561664425));
#13554=CARTESIAN_POINT('Ctrl Pts',(11.4598615582757,-57.2117511126201,-2.06354052510241E-11));
#13555=CARTESIAN_POINT('Ctrl Pts',(8.59489616869782,-57.0367511126202,-4.9622656166752));
#13556=CARTESIAN_POINT('Ctrl Pts',(5.72993077911996,-56.8617511126202,-9.92453123332976));
#13557=CARTESIAN_POINT('Ctrl Pts',(-1.78726082715848E-11,-56.6867511126202,
-9.92453123331945));
#13558=CARTESIAN_POINT('Ctrl Pts',(-5.7299307791557,-56.5117511126202,-9.92453123330913));
#13559=CARTESIAN_POINT('Ctrl Pts',(-8.59489616871569,-56.3367511126202,
-4.96226561664425));
#13560=CARTESIAN_POINT('Ctrl Pts',(-11.4598615582757,-56.1617511126202,
2.06368086793017E-11));
#13561=CARTESIAN_POINT('Ctrl Pts',(-8.59489616869782,-55.9867511126202,
4.9622656166752));
#13562=CARTESIAN_POINT('Ctrl Pts',(-5.72993077911996,-55.8117511126202,
9.92453123332977));
#13563=CARTESIAN_POINT('Ctrl Pts',(1.7871392867044E-11,-55.6367511126201,
9.92453123331945));
#13564=CARTESIAN_POINT('Ctrl Pts',(5.7299307791557,-55.4617511126202,9.92453123330913));
#13565=CARTESIAN_POINT('Ctrl Pts',(8.59489616871569,-55.2867511126202,4.96226561664425));
#13566=CARTESIAN_POINT('Ctrl Pts',(11.4598615582757,-55.1117511126202,-2.06354052510241E-11));
#13567=CARTESIAN_POINT('Ctrl Pts',(8.59489616869782,-54.9367511126202,-4.9622656166752));
#13568=CARTESIAN_POINT('Ctrl Pts',(5.72993077911996,-54.7617511126202,-9.92453123332976));
#13569=CARTESIAN_POINT('Ctrl Pts',(-1.78726082715848E-11,-54.5867511126202,
-9.92453123331945));
#13570=CARTESIAN_POINT('Ctrl Pts',(-5.7299307791557,-54.4117511126202,-9.92453123330913));
#13571=CARTESIAN_POINT('Ctrl Pts',(-8.59489616871569,-54.2367511126202,
-4.96226561664425));
#13572=CARTESIAN_POINT('Ctrl Pts',(-11.4598615582757,-54.0617511126202,
2.06368086793017E-11));
#13573=CARTESIAN_POINT('Ctrl Pts',(-8.59489616869782,-53.8867511126202,
4.9622656166752));
#13574=CARTESIAN_POINT('Ctrl Pts',(-5.72993077911996,-53.7117511126202,
9.92453123332977));
#13575=CARTESIAN_POINT('Ctrl Pts',(1.7871392867044E-11,-53.5367511126202,
9.92453123331945));
#13576=CARTESIAN_POINT('Ctrl Pts',(5.7299307791557,-53.3617511126202,9.92453123330913));
#13577=CARTESIAN_POINT('Ctrl Pts',(8.59489616871569,-53.1867511126202,4.96226561664425));
#13578=CARTESIAN_POINT('Ctrl Pts',(11.4598615582757,-53.0117511126202,-2.06354052510241E-11));
#13579=CARTESIAN_POINT('Ctrl Pts',(8.59489616869782,-52.8367511126202,-4.9622656166752));
#13580=CARTESIAN_POINT('Ctrl Pts',(5.72993077911996,-52.6617511126202,-9.92453123332976));
#13581=CARTESIAN_POINT('Ctrl Pts',(-1.78726082715848E-11,-52.4867511126202,
-9.92453123331945));
#13582=CARTESIAN_POINT('Ctrl Pts',(-5.7299307791557,-52.3117511126202,-9.92453123330913));
#13583=CARTESIAN_POINT('Ctrl Pts',(-8.59489616871569,-52.1367511126202,
-4.96226561664425));
#13584=CARTESIAN_POINT('Ctrl Pts',(-11.4598615582757,-51.9617511126202,
2.06368086793017E-11));
#13585=CARTESIAN_POINT('Ctrl Pts',(-8.59489616869782,-51.7867511126202,
4.9622656166752));
#13586=CARTESIAN_POINT('Ctrl Pts',(-5.72993077911996,-51.6117511126202,
9.92453123332977));
#13587=CARTESIAN_POINT('Ctrl Pts',(1.7871392867044E-11,-51.4367511126202,
9.92453123331945));
#13588=CARTESIAN_POINT('Ctrl Pts',(5.7299307791557,-51.2617511126202,9.92453123330913));
#13589=CARTESIAN_POINT('Ctrl Pts',(8.59489616871569,-51.0867511126202,4.96226561664425));
#13590=CARTESIAN_POINT('Ctrl Pts',(11.4598615582757,-50.9117511126202,-2.06354052510241E-11));
#13591=CARTESIAN_POINT('Ctrl Pts',(8.59489616869782,-50.7367511126202,-4.9622656166752));
#13592=CARTESIAN_POINT('Ctrl Pts',(5.72993077911996,-50.5617511126202,-9.92453123332976));
#13593=CARTESIAN_POINT('Ctrl Pts',(-1.78726082715848E-11,-50.3867511126202,
-9.92453123331945));
#13594=CARTESIAN_POINT('Ctrl Pts',(-5.7299307791557,-50.2117511126202,-9.92453123330913));
#13595=CARTESIAN_POINT('Ctrl Pts',(-8.59489616871569,-50.0367511126202,
-4.96226561664425));
#13596=CARTESIAN_POINT('Ctrl Pts',(-11.4598615582757,-49.8617511126202,
2.06368086793017E-11));
#13597=CARTESIAN_POINT('Ctrl Pts',(-8.59489616869782,-49.6867511126202,
4.9622656166752));
#13598=CARTESIAN_POINT('Ctrl Pts',(-5.72993077911996,-49.5117511126202,
9.92453123332977));
#13599=CARTESIAN_POINT('Ctrl Pts',(1.7871392867044E-11,-49.3367511126202,
9.92453123331945));
#13600=CARTESIAN_POINT('Ctrl Pts',(5.7299307791557,-49.1617511126202,9.92453123330913));
#13601=CARTESIAN_POINT('Ctrl Pts',(8.59489616871569,-48.9867511126202,4.96226561664425));
#13602=CARTESIAN_POINT('Ctrl Pts',(11.4598615582757,-48.8117511126202,-2.06354052510241E-11));
#13603=CARTESIAN_POINT('Ctrl Pts',(8.59489616869782,-48.6367511126202,-4.9622656166752));
#13604=CARTESIAN_POINT('Ctrl Pts',(5.72993077911996,-48.4617511126202,-9.92453123332976));
#13605=CARTESIAN_POINT('Ctrl Pts',(-1.78726082715848E-11,-48.2867511126202,
-9.92453123331945));
#13606=CARTESIAN_POINT('Ctrl Pts',(-5.7299307791557,-48.1117511126202,-9.92453123330913));
#13607=CARTESIAN_POINT('Ctrl Pts',(-8.59489616871569,-47.9367511126202,
-4.96226561664425));
#13608=CARTESIAN_POINT('Ctrl Pts',(-11.4598615582757,-47.7617511126202,
2.06368086793017E-11));
#13609=CARTESIAN_POINT('Ctrl Pts',(-8.59489616869782,-47.5867511126202,
4.9622656166752));
#13610=CARTESIAN_POINT('Ctrl Pts',(-5.72993077911996,-47.4117511126202,
9.92453123332977));
#13611=CARTESIAN_POINT('Ctrl Pts',(1.7871392867044E-11,-47.2367511126202,
9.92453123331945));
#13612=CARTESIAN_POINT('Ctrl Pts',(5.7299307791557,-47.0617511126202,9.92453123330913));
#13613=CARTESIAN_POINT('Ctrl Pts',(8.59489616871569,-46.8867511126202,4.96226561664425));
#13614=CARTESIAN_POINT('Ctrl Pts',(11.4598615582757,-46.7117511126202,-2.06354052510241E-11));
#13615=CARTESIAN_POINT('Ctrl Pts',(8.59489616869782,-46.5367511126202,-4.9622656166752));
#13616=CARTESIAN_POINT('Ctrl Pts',(5.72993077911996,-46.3617511126202,-9.92453123332976));
#13617=CARTESIAN_POINT('Ctrl Pts',(-1.78726082715848E-11,-46.1867511126202,
-9.92453123331945));
#13618=CARTESIAN_POINT('Ctrl Pts',(-5.7299307791557,-46.0117511126202,-9.92453123330913));
#13619=CARTESIAN_POINT('Ctrl Pts',(-8.59489616871569,-45.8367511126202,
-4.96226561664425));
#13620=CARTESIAN_POINT('Ctrl Pts',(-11.4598615582757,-45.6617511126202,
2.06368086793017E-11));
#13621=CARTESIAN_POINT('Ctrl Pts',(-8.59489616869782,-45.4867511126202,
4.9622656166752));
#13622=CARTESIAN_POINT('Ctrl Pts',(-5.72993077911996,-45.3117511126202,
9.92453123332977));
#13623=CARTESIAN_POINT('Ctrl Pts',(1.7871392867044E-11,-45.1367511126202,
9.92453123331945));
#13624=CARTESIAN_POINT('Ctrl Pts',(5.7299307791557,-44.9617511126202,9.92453123330913));
#13625=CARTESIAN_POINT('Ctrl Pts',(8.59489616871569,-44.7867511126202,4.96226561664425));
#13626=CARTESIAN_POINT('Ctrl Pts',(11.4598615582757,-44.6117511126202,-2.06354052510241E-11));
#13627=CARTESIAN_POINT('Ctrl Pts',(8.59489616869782,-44.4367511126202,-4.9622656166752));
#13628=CARTESIAN_POINT('Ctrl Pts',(5.72993077911996,-44.2617511126202,-9.92453123332976));
#13629=CARTESIAN_POINT('Ctrl Pts',(-1.78726082715848E-11,-44.0867511126202,
-9.92453123331945));
#13630=CARTESIAN_POINT('Ctrl Pts',(-5.7299307791557,-43.9117511126202,-9.92453123330913));
#13631=CARTESIAN_POINT('Ctrl Pts',(-8.59489616871569,-43.7367511126202,
-4.96226561664425));
#13632=CARTESIAN_POINT('Ctrl Pts',(-11.4598615582757,-43.5617511126202,
2.06368086793017E-11));
#13633=CARTESIAN_POINT('Ctrl Pts',(-8.59489616869782,-43.3867511126202,
4.9622656166752));
#13634=CARTESIAN_POINT('Ctrl Pts',(-5.72993077911996,-43.2117511126202,
9.92453123332977));
#13635=CARTESIAN_POINT('Ctrl Pts',(1.7871392867044E-11,-43.0367511126202,
9.92453123331945));
#13636=CARTESIAN_POINT('Ctrl Pts',(5.7299307791557,-42.8617511126202,9.92453123330913));
#13637=CARTESIAN_POINT('Ctrl Pts',(8.59489616871569,-42.6867511126202,4.96226561664425));
#13638=CARTESIAN_POINT('Ctrl Pts',(11.4598615582757,-42.5117511126202,-2.06354052510241E-11));
#13639=CARTESIAN_POINT('Ctrl Pts',(8.59489616869782,-42.3367511126202,-4.9622656166752));
#13640=CARTESIAN_POINT('Ctrl Pts',(5.72993077911996,-42.1617511126202,-9.92453123332976));
#13641=CARTESIAN_POINT('Ctrl Pts',(-1.78726082715848E-11,-41.9867511126202,
-9.92453123331945));
#13642=CARTESIAN_POINT('Ctrl Pts',(-5.7299307791557,-41.8117511126202,-9.92453123330913));
#13643=CARTESIAN_POINT('Ctrl Pts',(-8.59489616871569,-41.6367511126202,
-4.96226561664425));
#13644=CARTESIAN_POINT('Ctrl Pts',(-11.4598615582757,-41.4617511126202,
2.06368086793017E-11));
#13645=CARTESIAN_POINT('Ctrl Pts',(-8.59489616869782,-41.2867511126202,
4.9622656166752));
#13646=CARTESIAN_POINT('Ctrl Pts',(-5.72993077911996,-41.1117511126202,
9.92453123332977));
#13647=CARTESIAN_POINT('Ctrl Pts',(1.7871392867044E-11,-40.9367511126202,
9.92453123331945));
#13648=CARTESIAN_POINT('Ctrl Pts',(5.7299307791557,-40.7617511126202,9.92453123330913));
#13649=CARTESIAN_POINT('Ctrl Pts',(8.59489616871569,-40.5867511126202,4.96226561664425));
#13650=CARTESIAN_POINT('Ctrl Pts',(11.4598615582757,-40.4117511126202,-2.06354052510241E-11));
#13651=CARTESIAN_POINT('Ctrl Pts',(8.59489616869782,-40.2367511126202,-4.9622656166752));
#13652=CARTESIAN_POINT('Ctrl Pts',(5.72993077911996,-40.0617511126202,-9.92453123332976));
#13653=CARTESIAN_POINT('Ctrl Pts',(-1.78726082715848E-11,-39.8867511126202,
-9.92453123331945));
#13654=CARTESIAN_POINT('Ctrl Pts',(-5.7299307791557,-39.7117511126202,-9.92453123330913));
#13655=CARTESIAN_POINT('Ctrl Pts',(-8.59489616871569,-39.5367511126202,
-4.96226561664425));
#13656=CARTESIAN_POINT('Ctrl Pts',(-11.4598615582757,-39.3617511126202,
2.06368086793017E-11));
#13657=CARTESIAN_POINT('Ctrl Pts',(-8.59489616869782,-39.1867511126202,
4.9622656166752));
#13658=CARTESIAN_POINT('Ctrl Pts',(-5.72993077911996,-39.0117511126202,
9.92453123332977));
#13659=CARTESIAN_POINT('Ctrl Pts',(1.7871392867044E-11,-38.8367511126202,
9.92453123331945));
#13660=CARTESIAN_POINT('Ctrl Pts',(5.7299307791557,-38.6617511126202,9.92453123330913));
#13661=CARTESIAN_POINT('Ctrl Pts',(8.59489616871569,-38.4867511126202,4.96226561664425));
#13662=CARTESIAN_POINT('Ctrl Pts',(11.4598615582757,-38.3117511126202,-2.06354052510241E-11));
#13663=CARTESIAN_POINT('Ctrl Pts',(8.59489616869782,-38.1367511126202,-4.9622656166752));
#13664=CARTESIAN_POINT('Ctrl Pts',(5.72993077911996,-37.9617511126202,-9.92453123332976));
#13665=CARTESIAN_POINT('Ctrl Pts',(-1.78726082715848E-11,-37.7867511126202,
-9.92453123331945));
#13666=CARTESIAN_POINT('Ctrl Pts',(-5.7299307791557,-37.6117511126202,-9.92453123330913));
#13667=CARTESIAN_POINT('Ctrl Pts',(-8.59489616871569,-37.4367511126202,
-4.96226561664425));
#13668=CARTESIAN_POINT('Ctrl Pts',(-11.4598615582757,-37.2617511126202,
2.06368086793017E-11));
#13669=CARTESIAN_POINT('Ctrl Pts',(-8.59489616869782,-37.0867511126202,
4.9622656166752));
#13670=CARTESIAN_POINT('Ctrl Pts',(-5.72993077911996,-36.9117511126202,
9.92453123332977));
#13671=CARTESIAN_POINT('Ctrl Pts',(1.7871392867044E-11,-36.7367511126202,
9.92453123331945));
#13672=CARTESIAN_POINT('Ctrl Pts',(5.7299307791557,-36.5617511126202,9.92453123330913));
#13673=CARTESIAN_POINT('Ctrl Pts',(8.59489616871569,-36.3867511126202,4.96226561664425));
#13674=CARTESIAN_POINT('Ctrl Pts',(11.4598615582757,-36.2117511126202,-2.06354052510241E-11));
#13675=CARTESIAN_POINT('Ctrl Pts',(8.59489616869782,-36.0367511126202,-4.9622656166752));
#13676=CARTESIAN_POINT('Ctrl Pts',(5.72993077911996,-35.8617511126202,-9.92453123332976));
#13677=CARTESIAN_POINT('Ctrl Pts',(-1.78726082715848E-11,-35.6867511126202,
-9.92453123331945));
#13678=CARTESIAN_POINT('Ctrl Pts',(-5.7299307791557,-35.5117511126202,-9.92453123330913));
#13679=CARTESIAN_POINT('Ctrl Pts',(-8.59489616871569,-35.3367511126202,
-4.96226561664425));
#13680=CARTESIAN_POINT('Ctrl Pts',(-11.4598615582757,-35.1617511126202,
2.06368086793017E-11));
#13681=CARTESIAN_POINT('Ctrl Pts',(-8.59489616869782,-34.9867511126202,
4.9622656166752));
#13682=CARTESIAN_POINT('Ctrl Pts',(-5.72993077911996,-34.8117511126202,
9.92453123332977));
#13683=CARTESIAN_POINT('Ctrl Pts',(1.7871392867044E-11,-34.6367511126202,
9.92453123331945));
#13684=CARTESIAN_POINT('Ctrl Pts',(5.7299307791557,-34.4617511126202,9.92453123330913));
#13685=CARTESIAN_POINT('Ctrl Pts',(8.59489616871569,-34.2867511126202,4.96226561664425));
#13686=CARTESIAN_POINT('Ctrl Pts',(11.4598615582757,-34.1117511126202,-2.06354052510241E-11));
#13687=CARTESIAN_POINT('Ctrl Pts',(8.59489616869782,-33.9367511126202,-4.9622656166752));
#13688=CARTESIAN_POINT('Ctrl Pts',(5.72993077911996,-33.7617511126202,-9.92453123332976));
#13689=CARTESIAN_POINT('Ctrl Pts',(-1.78726082715848E-11,-33.5867511126202,
-9.92453123331945));
#13690=CARTESIAN_POINT('Ctrl Pts',(-5.7299307791557,-33.4117511126202,-9.92453123330913));
#13691=CARTESIAN_POINT('Ctrl Pts',(-8.59489616871569,-33.2367511126202,
-4.96226561664425));
#13692=CARTESIAN_POINT('Ctrl Pts',(-11.4598615582757,-33.0617511126202,
2.06368086793017E-11));
#13693=CARTESIAN_POINT('Ctrl Pts',(-8.59489616869782,-32.8867511126202,
4.9622656166752));
#13694=CARTESIAN_POINT('Ctrl Pts',(-5.72993077911996,-32.7117511126202,
9.92453123332977));
#13695=CARTESIAN_POINT('Ctrl Pts',(1.7871392867044E-11,-32.5367511126202,
9.92453123331945));
#13696=CARTESIAN_POINT('Ctrl Pts',(5.7299307791557,-32.3617511126202,9.92453123330913));
#13697=CARTESIAN_POINT('Ctrl Pts',(8.59489616871569,-32.1867511126202,4.96226561664425));
#13698=CARTESIAN_POINT('Ctrl Pts',(11.4598615582757,-32.0117511126202,-2.06354052510241E-11));
#13699=CARTESIAN_POINT('Ctrl Pts',(8.59489616869782,-31.8367511126202,-4.9622656166752));
#13700=CARTESIAN_POINT('Ctrl Pts',(5.72993077911996,-31.6617511126202,-9.92453123332976));
#13701=CARTESIAN_POINT('Ctrl Pts',(-1.78726082715848E-11,-31.4867511126202,
-9.92453123331945));
#13702=CARTESIAN_POINT('Ctrl Pts',(-5.7299307791557,-31.3117511126202,-9.92453123330913));
#13703=CARTESIAN_POINT('Ctrl Pts',(-8.59489616871569,-31.1367511126202,
-4.96226561664425));
#13704=CARTESIAN_POINT('Ctrl Pts',(-11.4598615582757,-30.9617511126202,
2.06368086793017E-11));
#13705=CARTESIAN_POINT('Ctrl Pts',(-8.59489616869782,-30.7867511126202,
4.9622656166752));
#13706=CARTESIAN_POINT('Ctrl Pts',(-5.72993077911996,-30.6117511126202,
9.92453123332977));
#13707=CARTESIAN_POINT('Ctrl Pts',(1.7871392867044E-11,-30.4367511126202,
9.92453123331945));
#13708=CARTESIAN_POINT('Ctrl Pts',(5.7299307791557,-30.2617511126202,9.92453123330913));
#13709=CARTESIAN_POINT('Ctrl Pts',(8.59489616871569,-30.0867511126202,4.96226561664425));
#13710=CARTESIAN_POINT('Ctrl Pts',(11.4598615582757,-29.9117511126202,-2.06354052510241E-11));
#13711=CARTESIAN_POINT('Ctrl Pts',(8.59489616869782,-29.7367511126202,-4.9622656166752));
#13712=CARTESIAN_POINT('Ctrl Pts',(5.72993077911996,-29.5617511126202,-9.92453123332976));
#13713=CARTESIAN_POINT('Ctrl Pts',(-1.78726082715848E-11,-29.3867511126202,
-9.92453123331945));
#13714=CARTESIAN_POINT('Ctrl Pts',(-5.7299307791557,-29.2117511126202,-9.92453123330913));
#13715=CARTESIAN_POINT('Ctrl Pts',(-8.59489616871569,-29.0367511126202,
-4.96226561664425));
#13716=CARTESIAN_POINT('Ctrl Pts',(-11.4598615582757,-28.8617511126202,
2.06368086793017E-11));
#13717=CARTESIAN_POINT('Ctrl Pts',(-8.59489616869782,-28.6867511126202,
4.9622656166752));
#13718=CARTESIAN_POINT('Ctrl Pts',(-5.72993077911996,-28.5117511126202,
9.92453123332977));
#13719=CARTESIAN_POINT('Ctrl Pts',(1.7871392867044E-11,-28.3367511126202,
9.92453123331945));
#13720=CARTESIAN_POINT('Ctrl Pts',(5.7299307791557,-28.1617511126202,9.92453123330913));
#13721=CARTESIAN_POINT('Ctrl Pts',(8.59489616871569,-27.9867511126202,4.96226561664425));
#13722=CARTESIAN_POINT('Ctrl Pts',(11.4598615582757,-27.8117511126202,-2.06354052510241E-11));
#13723=CARTESIAN_POINT('Ctrl Pts',(8.59489616869782,-27.6367511126202,-4.9622656166752));
#13724=CARTESIAN_POINT('Ctrl Pts',(5.72993077911996,-27.4617511126202,-9.92453123332976));
#13725=CARTESIAN_POINT('Ctrl Pts',(-1.78726082715848E-11,-27.2867511126202,
-9.92453123331945));
#13726=CARTESIAN_POINT('Ctrl Pts',(-5.7299307791557,-27.1117511126202,-9.92453123330913));
#13727=CARTESIAN_POINT('Ctrl Pts',(-8.59489616871569,-26.9367511126202,
-4.96226561664425));
#13728=CARTESIAN_POINT('Ctrl Pts',(-11.4598615582757,-26.7617511126202,
2.06368086793017E-11));
#13729=CARTESIAN_POINT('Ctrl Pts',(-8.59489616869782,-26.5867511126202,
4.9622656166752));
#13730=CARTESIAN_POINT('Ctrl Pts',(-5.72993077911996,-26.4117511126202,
9.92453123332977));
#13731=CARTESIAN_POINT('Ctrl Pts',(1.7871392867044E-11,-26.2367511126202,
9.92453123331945));
#13732=CARTESIAN_POINT('Ctrl Pts',(5.7299307791557,-26.0617511126202,9.92453123330913));
#13733=CARTESIAN_POINT('Ctrl Pts',(8.59489616871569,-25.8867511126202,4.96226561664425));
#13734=CARTESIAN_POINT('Ctrl Pts',(11.4598615582757,-25.7117511126202,-2.06354052510241E-11));
#13735=CARTESIAN_POINT('Ctrl Pts',(8.59489616869782,-25.5367511126202,-4.9622656166752));
#13736=CARTESIAN_POINT('Ctrl Pts',(5.72993077911996,-25.3617511126202,-9.92453123332976));
#13737=CARTESIAN_POINT('Ctrl Pts',(-1.78726082715848E-11,-25.1867511126202,
-9.92453123331945));
#13738=CARTESIAN_POINT('Ctrl Pts',(-5.7299307791557,-25.0117511126202,-9.92453123330913));
#13739=CARTESIAN_POINT('Ctrl Pts',(-8.59489616871569,-24.8367511126202,
-4.96226561664425));
#13740=CARTESIAN_POINT('Ctrl Pts',(-11.4598615582757,-24.6617511126202,
2.06368086793017E-11));
#13741=CARTESIAN_POINT('Ctrl Pts',(-8.59489616869782,-24.4867511126202,
4.9622656166752));
#13742=CARTESIAN_POINT('Ctrl Pts',(-5.72993077911996,-24.3117511126202,
9.92453123332977));
#13743=CARTESIAN_POINT('Ctrl Pts',(1.7871392867044E-11,-24.1367511126202,
9.92453123331945));
#13744=CARTESIAN_POINT('Ctrl Pts',(5.7299307791557,-23.9617511126202,9.92453123330913));
#13745=CARTESIAN_POINT('Ctrl Pts',(8.59489616871569,-23.7867511126202,4.96226561664425));
#13746=CARTESIAN_POINT('Ctrl Pts',(11.4598615582757,-23.6117511126202,-2.06354052510241E-11));
#13747=CARTESIAN_POINT('Ctrl Pts',(8.59489616869782,-23.4367511126202,-4.9622656166752));
#13748=CARTESIAN_POINT('Ctrl Pts',(5.72993077911996,-23.2617511126202,-9.92453123332976));
#13749=CARTESIAN_POINT('Ctrl Pts',(-1.78726082715848E-11,-23.0867511126202,
-9.92453123331945));
#13750=CARTESIAN_POINT('Ctrl Pts',(-5.7299307791557,-22.9117511126202,-9.92453123330913));
#13751=CARTESIAN_POINT('Ctrl Pts',(-8.59489616871569,-22.7367511126202,
-4.96226561664425));
#13752=CARTESIAN_POINT('Ctrl Pts',(-11.4598615582757,-22.5617511126203,
2.06368086793017E-11));
#13753=CARTESIAN_POINT('Ctrl Pts',(-8.59489616869782,-22.3867511126202,
4.9622656166752));
#13754=CARTESIAN_POINT('Ctrl Pts',(-5.72993077911996,-22.2117511126202,
9.92453123332977));
#13755=CARTESIAN_POINT('Ctrl Pts',(1.7871392867044E-11,-22.0367511126202,
9.92453123331945));
#13756=CARTESIAN_POINT('Ctrl Pts',(5.7299307791557,-21.8617511126202,9.92453123330913));
#13757=CARTESIAN_POINT('Ctrl Pts',(8.59489616871569,-21.6867511126202,4.96226561664425));
#13758=CARTESIAN_POINT('Ctrl Pts',(11.4598615582757,-21.5117511126203,-2.06354052510241E-11));
#13759=CARTESIAN_POINT('Ctrl Pts',(8.59489616869782,-21.3367511126202,-4.9622656166752));
#13760=CARTESIAN_POINT('Ctrl Pts',(5.72993077911996,-21.1617511126202,-9.92453123332976));
#13761=CARTESIAN_POINT('Ctrl Pts',(-1.78726082715848E-11,-20.9867511126202,
-9.92453123331945));
#13762=CARTESIAN_POINT('Ctrl Pts',(-5.7299307791557,-20.8117511126202,-9.92453123330913));
#13763=CARTESIAN_POINT('Ctrl Pts',(-8.59489616871569,-20.6367511126202,
-4.96226561664425));
#13764=CARTESIAN_POINT('Ctrl Pts',(-11.4598615582757,-20.4617511126202,
2.06368086793017E-11));
#13765=CARTESIAN_POINT('Ctrl Pts',(-8.59489616869782,-20.2867511126202,
4.9622656166752));
#13766=CARTESIAN_POINT('Ctrl Pts',(-5.72993077911996,-20.1117511126202,
9.92453123332977));
#13767=CARTESIAN_POINT('Ctrl Pts',(1.7871392867044E-11,-19.9367511126202,
9.92453123331945));
#13768=CARTESIAN_POINT('Ctrl Pts',(5.7299307791557,-19.7617511126202,9.92453123330913));
#13769=CARTESIAN_POINT('Ctrl Pts',(8.59489616871569,-19.5867511126202,4.96226561664425));
#13770=CARTESIAN_POINT('Ctrl Pts',(11.4598615582757,-19.4117511126203,-2.06354052510241E-11));
#13771=CARTESIAN_POINT('Ctrl Pts',(8.59489616869782,-19.2367511126202,-4.9622656166752));
#13772=CARTESIAN_POINT('Ctrl Pts',(5.72993077911996,-19.0617511126202,-9.92453123332976));
#13773=CARTESIAN_POINT('Ctrl Pts',(-1.78726082715848E-11,-18.8867511126203,
-9.92453123331945));
#13774=CARTESIAN_POINT('Ctrl Pts',(-5.7299307791557,-18.7117511126203,-9.92453123330913));
#13775=CARTESIAN_POINT('Ctrl Pts',(-8.59489616871569,-18.5367511126202,
-4.96226561664425));
#13776=CARTESIAN_POINT('Ctrl Pts',(-11.4598615582757,-18.3617511126203,
2.06368086793017E-11));
#13777=CARTESIAN_POINT('Ctrl Pts',(-8.59489616869782,-18.1867511126202,
4.9622656166752));
#13778=CARTESIAN_POINT('Ctrl Pts',(-5.72993077911996,-18.0117511126202,
9.92453123332977));
#13779=CARTESIAN_POINT('Ctrl Pts',(1.7871392867044E-11,-17.8367511126203,
9.92453123331945));
#13780=CARTESIAN_POINT('Ctrl Pts',(5.7299307791557,-17.6617511126203,9.92453123330913));
#13781=CARTESIAN_POINT('Ctrl Pts',(8.59489616871569,-17.4867511126202,4.96226561664425));
#13782=CARTESIAN_POINT('Ctrl Pts',(11.4598615582757,-17.3117511126203,-2.06354052510241E-11));
#13783=CARTESIAN_POINT('Ctrl Pts',(8.59489616869782,-17.1367511126203,-4.9622656166752));
#13784=CARTESIAN_POINT('Ctrl Pts',(5.72993077911996,-16.9617511126202,-9.92453123332976));
#13785=CARTESIAN_POINT('Ctrl Pts',(-1.78726082715848E-11,-16.7867511126202,
-9.92453123331945));
#13786=CARTESIAN_POINT('Ctrl Pts',(-5.7299307791557,-16.6117511126203,-9.92453123330913));
#13787=CARTESIAN_POINT('Ctrl Pts',(-8.59489616871569,-16.4367511126202,
-4.96226561664425));
#13788=CARTESIAN_POINT('Ctrl Pts',(-11.4598615582757,-16.2617511126202,
2.06368086793017E-11));
#13789=CARTESIAN_POINT('Ctrl Pts',(-8.59489616869782,-16.0867511126203,
4.9622656166752));
#13790=CARTESIAN_POINT('Ctrl Pts',(-5.72993077911996,-15.9117511126202,
9.92453123332977));
#13791=CARTESIAN_POINT('Ctrl Pts',(1.7871392867044E-11,-15.7367511126202,
9.92453123331945));
#13792=CARTESIAN_POINT('Ctrl Pts',(5.7299307791557,-15.5617511126203,9.92453123330913));
#13793=CARTESIAN_POINT('Ctrl Pts',(8.59489616871569,-15.3867511126203,4.96226561664425));
#13794=CARTESIAN_POINT('Ctrl Pts',(11.4598615582757,-15.2117511126203,-2.06354052510241E-11));
#13795=CARTESIAN_POINT('Ctrl Pts',(8.59489616869782,-15.0367511126203,-4.9622656166752));
#13796=CARTESIAN_POINT('Ctrl Pts',(5.72993077911996,-14.8617511126203,-9.92453123332976));
#13797=CARTESIAN_POINT('Ctrl Pts',(-1.78726082715848E-11,-14.6867511126202,
-9.92453123331945));
#13798=CARTESIAN_POINT('Ctrl Pts',(-5.7299307791557,-14.5117511126203,-9.92453123330913));
#13799=CARTESIAN_POINT('Ctrl Pts',(-8.59489616871569,-14.3367511126203,
-4.96226561664425));
#13800=CARTESIAN_POINT('Ctrl Pts',(-11.4598615582757,-14.1617511126203,
2.06368086793017E-11));
#13801=CARTESIAN_POINT('Ctrl Pts',(-8.59489616869782,-13.9867511126203,
4.9622656166752));
#13802=CARTESIAN_POINT('Ctrl Pts',(-5.72993077911996,-13.8117511126203,
9.92453123332977));
#13803=CARTESIAN_POINT('Ctrl Pts',(1.7871392867044E-11,-13.6367511126203,
9.92453123331945));
#13804=CARTESIAN_POINT('Ctrl Pts',(5.7299307791557,-13.4617511126203,9.92453123330913));
#13805=CARTESIAN_POINT('Ctrl Pts',(8.59489616871569,-13.2867511126203,4.96226561664425));
#13806=CARTESIAN_POINT('Ctrl Pts',(11.4598615582757,-13.1117511126203,-2.06354052510241E-11));
#13807=CARTESIAN_POINT('Ctrl Pts',(8.59489616869782,-12.9367511126203,-4.9622656166752));
#13808=CARTESIAN_POINT('Ctrl Pts',(5.72993077911996,-12.7617511126203,-9.92453123332976));
#13809=CARTESIAN_POINT('Ctrl Pts',(-1.78726082715848E-11,-12.5867511126203,
-9.92453123331945));
#13810=CARTESIAN_POINT('Ctrl Pts',(-5.7299307791557,-12.4117511126202,-9.92453123330913));
#13811=CARTESIAN_POINT('Ctrl Pts',(-8.59489616871569,-12.2367511126203,
-4.96226561664425));
#13812=CARTESIAN_POINT('Ctrl Pts',(-11.4598615582757,-12.0617511126203,
2.06368086793017E-11));
#13813=CARTESIAN_POINT('Ctrl Pts',(-8.59489616869782,-11.8867511126202,
4.9622656166752));
#13814=CARTESIAN_POINT('Ctrl Pts',(-5.72993077911996,-11.7117511126203,
9.92453123332977));
#13815=CARTESIAN_POINT('Ctrl Pts',(1.7871392867044E-11,-11.5367511126203,
9.92453123331945));
#13816=CARTESIAN_POINT('Ctrl Pts',(5.7299307791557,-11.3617511126203,9.92453123330913));
#13817=CARTESIAN_POINT('Ctrl Pts',(8.59489616871569,-11.1867511126203,4.96226561664425));
#13818=CARTESIAN_POINT('Ctrl Pts',(11.4598615582757,-11.0117511126203,-2.06354052510241E-11));
#13819=CARTESIAN_POINT('Ctrl Pts',(8.59489616869782,-10.8367511126203,-4.9622656166752));
#13820=CARTESIAN_POINT('Ctrl Pts',(5.72993077911996,-10.6617511126203,-9.92453123332976));
#13821=CARTESIAN_POINT('Ctrl Pts',(-1.78726082715848E-11,-10.4867511126203,
-9.92453123331945));
#13822=CARTESIAN_POINT('Ctrl Pts',(-5.7299307791557,-10.3117511126203,-9.92453123330913));
#13823=CARTESIAN_POINT('Ctrl Pts',(-8.59489616871569,-10.1367511126203,
-4.96226561664425));
#13824=CARTESIAN_POINT('Ctrl Pts',(-11.4598615582757,-9.96175111262027,
2.06368086793017E-11));
#13825=CARTESIAN_POINT('Ctrl Pts',(-8.59489616869782,-9.78675111262026,
4.9622656166752));
#13826=CARTESIAN_POINT('Ctrl Pts',(-5.72993077911996,-9.61175111262028,
9.92453123332977));
#13827=CARTESIAN_POINT('Ctrl Pts',(1.7871392867044E-11,-9.43675111262027,
9.92453123331945));
#13828=CARTESIAN_POINT('Ctrl Pts',(5.7299307791557,-9.26175111262026,9.92453123330913));
#13829=CARTESIAN_POINT('Ctrl Pts',(8.59489616871569,-9.08675111262028,4.96226561664425));
#13830=CARTESIAN_POINT('Ctrl Pts',(11.4598615582757,-8.91175111262028,-2.06354052510241E-11));
#13831=CARTESIAN_POINT('Ctrl Pts',(8.59489616869782,-8.73675111262026,-4.9622656166752));
#13832=CARTESIAN_POINT('Ctrl Pts',(5.72993077911996,-8.56175111262028,-9.92453123332976));
#13833=CARTESIAN_POINT('Ctrl Pts',(-1.78726082715848E-11,-8.38675111262027,
-9.92453123331945));
#13834=CARTESIAN_POINT('Ctrl Pts',(-5.7299307791557,-8.21175111262026,-9.92453123330913));
#13835=CARTESIAN_POINT('Ctrl Pts',(-8.59489616871569,-8.03675111262026,
-4.96226561664425));
#13836=CARTESIAN_POINT('Ctrl Pts',(-11.4598615582757,-7.86175111262028,
2.06368086793017E-11));
#13837=CARTESIAN_POINT('Ctrl Pts',(-8.59489616869782,-7.68675111262027,
4.9622656166752));
#13838=CARTESIAN_POINT('Ctrl Pts',(-5.72993077911996,-7.51175111262027,
9.92453123332977));
#13839=CARTESIAN_POINT('Ctrl Pts',(1.7871392867044E-11,-7.33675111262028,
9.92453123331945));
#13840=CARTESIAN_POINT('Ctrl Pts',(5.7299307791557,-7.16175111262027,9.92453123330913));
#13841=CARTESIAN_POINT('Ctrl Pts',(8.59489616871569,-6.98675111262026,4.96226561664425));
#13842=CARTESIAN_POINT('Ctrl Pts',(11.4598615582757,-6.81175111262029,-2.06354052510241E-11));
#13843=CARTESIAN_POINT('Ctrl Pts',(8.59489616869782,-6.63675111262027,-4.9622656166752));
#13844=CARTESIAN_POINT('Ctrl Pts',(5.72993077911996,-6.46175111262027,-9.92453123332976));
#13845=CARTESIAN_POINT('Ctrl Pts',(-1.78726082715848E-11,-6.28675111262028,
-9.92453123331945));
#13846=CARTESIAN_POINT('Ctrl Pts',(-5.7299307791557,-6.11175111262027,-9.92453123330913));
#13847=CARTESIAN_POINT('Ctrl Pts',(-8.59489616871569,-5.93675111262026,
-4.96226561664425));
#13848=CARTESIAN_POINT('Ctrl Pts',(-11.4598615582757,-5.76175111262029,
2.06368086793017E-11));
#13849=CARTESIAN_POINT('Ctrl Pts',(-8.59489616869782,-5.58675111262028,
4.9622656166752));
#13850=CARTESIAN_POINT('Ctrl Pts',(-5.72993077911996,-5.41175111262028,
9.92453123332977));
#13851=CARTESIAN_POINT('Ctrl Pts',(1.7871392867044E-11,-5.23675111262029,
9.92453123331945));
#13852=CARTESIAN_POINT('Ctrl Pts',(5.7299307791557,-5.06175111262028,9.92453123330913));
#13853=CARTESIAN_POINT('Ctrl Pts',(8.59489616871569,-4.88675111262027,4.96226561664425));
#13854=CARTESIAN_POINT('Ctrl Pts',(11.4598615582757,-4.7117511126203,-2.06354052510241E-11));
#13855=CARTESIAN_POINT('Ctrl Pts',(8.59489616869782,-4.53675111262028,-4.9622656166752));
#13856=CARTESIAN_POINT('Ctrl Pts',(5.72993077911996,-4.36175111262028,-9.92453123332976));
#13857=CARTESIAN_POINT('Ctrl Pts',(-1.78726082715848E-11,-4.18675111262029,
-9.92453123331945));
#13858=CARTESIAN_POINT('Ctrl Pts',(-5.7299307791557,-4.01175111262028,-9.92453123330913));
#13859=CARTESIAN_POINT('Ctrl Pts',(-8.59489616871569,-3.83675111262027,
-4.96226561664425));
#13860=CARTESIAN_POINT('Ctrl Pts',(-11.4598615582757,-3.66175111262027,
2.06368086793017E-11));
#13861=CARTESIAN_POINT('Ctrl Pts',(-8.59489616869782,-3.48675111262029,
4.9622656166752));
#13862=CARTESIAN_POINT('Ctrl Pts',(-5.72993077911996,-3.31175111262029,
9.92453123332977));
#13863=CARTESIAN_POINT('Ctrl Pts',(1.7871392867044E-11,-3.13675111262027,
9.92453123331945));
#13864=CARTESIAN_POINT('Ctrl Pts',(5.7299307791557,-2.96175111262029,9.92453123330913));
#13865=CARTESIAN_POINT('Ctrl Pts',(8.59489616871569,-2.78675111262028,4.96226561664425));
#13866=CARTESIAN_POINT('Ctrl Pts',(11.4598615582757,-2.61175111262027,-2.06354052510241E-11));
#13867=CARTESIAN_POINT('Ctrl Pts',(8.59489616869782,-2.43675111262029,-4.9622656166752));
#13868=CARTESIAN_POINT('Ctrl Pts',(5.72993077911996,-2.26175111262028,-9.92453123332976));
#13869=CARTESIAN_POINT('Ctrl Pts',(-1.78726082715848E-11,-2.08675111262027,
-9.92453123331945));
#13870=CARTESIAN_POINT('Ctrl Pts',(-5.7299307791557,-1.91175111262029,-9.92453123330913));
#13871=CARTESIAN_POINT('Ctrl Pts',(-8.59489616871569,-1.73675111262028,
-4.96226561664425));
#13872=CARTESIAN_POINT('Ctrl Pts',(-11.4598615582757,-1.56175111262028,
2.06368086793017E-11));
#13873=CARTESIAN_POINT('Ctrl Pts',(-8.59489616869782,-1.38675111262029,
4.9622656166752));
#13874=CARTESIAN_POINT('Ctrl Pts',(-5.72993077911996,-1.21175111262029,
9.92453123332977));
#13875=CARTESIAN_POINT('Ctrl Pts',(1.7871392867044E-11,-1.03675111262028,
9.92453123331945));
#13876=CARTESIAN_POINT('Ctrl Pts',(5.7299307791557,-0.861751112620297,9.92453123330913));
#13877=CARTESIAN_POINT('Ctrl Pts',(8.59489616871569,-0.686751112620287,
4.96226561664425));
#13878=CARTESIAN_POINT('Ctrl Pts',(11.4598615582757,-0.511751112620282,
-2.06354052510241E-11));
#13879=CARTESIAN_POINT('Ctrl Pts',(8.59489616869782,-0.336751112620298,
-4.9622656166752));
#13880=CARTESIAN_POINT('Ctrl Pts',(5.72993077911996,-0.161751112620292,
-9.92453123332976));
#13881=CARTESIAN_POINT('Ctrl Pts',(-1.78726082715848E-11,0.0132488873797187,
-9.92453123331945));
#13882=CARTESIAN_POINT('Ctrl Pts',(-5.7299307791557,0.188248887379698,-9.92453123330913));
#13883=CARTESIAN_POINT('Ctrl Pts',(-8.59489616871569,0.363248887379708,
-4.96226561664425));
#13884=CARTESIAN_POINT('Ctrl Pts',(-11.4598615582757,0.538248887379713,
2.06368086793017E-11));
#13885=CARTESIAN_POINT('Ctrl Pts',(-8.59489616869782,0.713248887379725,
4.9622656166752));
#13886=CARTESIAN_POINT('Ctrl Pts',(-5.72993077911996,0.888248887379703,
9.92453123332977));
#13887=CARTESIAN_POINT('Ctrl Pts',(1.7871392867044E-11,1.06324888737971,
9.92453123331945));
#13888=CARTESIAN_POINT('Ctrl Pts',(5.7299307791557,1.23824888737972,9.92453123330913));
#13889=CARTESIAN_POINT('Ctrl Pts',(8.59489616871569,1.4132488873797,4.96226561664425));
#13890=CARTESIAN_POINT('Ctrl Pts',(11.4598615582757,1.58824888737971,-2.06354052510241E-11));
#13891=CARTESIAN_POINT('Ctrl Pts',(8.59489616869782,1.76324888737972,-4.9622656166752));
#13892=CARTESIAN_POINT('Ctrl Pts',(5.72993077911996,1.9382488873797,-9.92453123332976));
#13893=CARTESIAN_POINT('Ctrl Pts',(-1.78726082715848E-11,2.11324888737971,
-9.92453123331945));
#13894=CARTESIAN_POINT('Ctrl Pts',(-5.7299307791557,2.28824888737971,-9.92453123330913));
#13895=CARTESIAN_POINT('Ctrl Pts',(-8.59489616871569,2.4632488873797,-4.96226561664425));
#13896=CARTESIAN_POINT('Ctrl Pts',(-11.4598615582757,2.6382488873797,2.06368086793017E-11));
#13897=CARTESIAN_POINT('Ctrl Pts',(-8.59489616869782,2.81324888737972,4.9622656166752));
#13898=CARTESIAN_POINT('Ctrl Pts',(-5.72993077911996,2.98824888737969,9.92453123332977));
#13899=CARTESIAN_POINT('Ctrl Pts',(1.7871392867044E-11,3.16324888737971,
9.92453123331945));
#13900=CARTESIAN_POINT('Ctrl Pts',(5.7299307791557,3.33824888737971,9.92453123330913));
#13901=CARTESIAN_POINT('Ctrl Pts',(8.59489616871569,3.51324888737969,4.96226561664425));
#13902=CARTESIAN_POINT('Ctrl Pts',(11.4598615582757,3.6882488873797,-2.06354052510241E-11));
#13903=CARTESIAN_POINT('Ctrl Pts',(8.59489616869782,3.86324888737971,-4.9622656166752));
#13904=CARTESIAN_POINT('Ctrl Pts',(5.72993077911996,4.03824888737969,-9.92453123332976));
#13905=CARTESIAN_POINT('Ctrl Pts',(-1.78726082715848E-11,4.2132488873797,
-9.92453123331945));
#13906=CARTESIAN_POINT('Ctrl Pts',(-5.7299307791557,4.3882488873797,-9.92453123330913));
#13907=CARTESIAN_POINT('Ctrl Pts',(-8.59489616871569,4.56324888737969,-4.96226561664425));
#13908=CARTESIAN_POINT('Ctrl Pts',(-11.4598615582757,4.73824888737969,2.06368086793017E-11));
#13909=CARTESIAN_POINT('Ctrl Pts',(-8.59489616869782,4.91324888737971,4.9622656166752));
#13910=CARTESIAN_POINT('Ctrl Pts',(-5.72993077911996,5.08824888737969,9.92453123332977));
#13911=CARTESIAN_POINT('Ctrl Pts',(1.7871392867044E-11,5.2632488873797,
9.92453123331945));
#13912=CARTESIAN_POINT('Ctrl Pts',(5.7299307791557,5.4382488873797,9.92453123330913));
#13913=CARTESIAN_POINT('Ctrl Pts',(8.59489616871569,5.61324888737971,4.96226561664425));
#13914=CARTESIAN_POINT('Ctrl Pts',(11.4598615582757,5.78824888737969,-2.06354052510241E-11));
#13915=CARTESIAN_POINT('Ctrl Pts',(8.59489616869782,5.9632488873797,-4.9622656166752));
#13916=CARTESIAN_POINT('Ctrl Pts',(5.72993077911996,6.1382488873797,-9.92453123332976));
#13917=CARTESIAN_POINT('Ctrl Pts',(-1.78726082715848E-11,6.31324888737969,
-9.92453123331945));
#13918=CARTESIAN_POINT('Ctrl Pts',(-5.7299307791557,6.4882488873797,-9.92453123330913));
#13919=CARTESIAN_POINT('Ctrl Pts',(-8.59489616871569,6.66324888737971,-4.96226561664425));
#13920=CARTESIAN_POINT('Ctrl Pts',(-11.4598615582757,6.83824888737969,2.06368086793017E-11));
#13921=CARTESIAN_POINT('Ctrl Pts',(-8.59489616869782,7.0132488873797,4.9622656166752));
#13922=CARTESIAN_POINT('Ctrl Pts',(-5.72993077911996,7.1882488873797,9.92453123332977));
#13923=CARTESIAN_POINT('Ctrl Pts',(1.7871392867044E-11,7.36324888737969,
9.92453123331945));
#13924=CARTESIAN_POINT('Ctrl Pts',(5.7299307791557,7.53824888737969,9.92453123330913));
#13925=CARTESIAN_POINT('Ctrl Pts',(8.59489616871569,7.7132488873797,4.96226561664425));
#13926=CARTESIAN_POINT('Ctrl Pts',(11.4598615582757,7.88824888737968,-2.06354052510241E-11));
#13927=CARTESIAN_POINT('Ctrl Pts',(8.59489616869782,8.06324888737969,-4.9622656166752));
#13928=CARTESIAN_POINT('Ctrl Pts',(5.72993077911996,8.2382488873797,-9.92453123332976));
#13929=CARTESIAN_POINT('Ctrl Pts',(-1.78726082715848E-11,8.41324888737968,
-9.92453123331945));
#13930=CARTESIAN_POINT('Ctrl Pts',(-5.7299307791557,8.58824888737968,-9.92453123330913));
#13931=CARTESIAN_POINT('Ctrl Pts',(-8.59489616871569,8.7632488873797,-4.96226561664425));
#13932=CARTESIAN_POINT('Ctrl Pts',(-11.4598615582757,8.93824888737968,2.06368086793017E-11));
#13933=CARTESIAN_POINT('Ctrl Pts',(-8.59489616869782,9.11324888737969,4.9622656166752));
#13934=CARTESIAN_POINT('Ctrl Pts',(-5.72993077911996,9.28824888737969,9.92453123332977));
#13935=CARTESIAN_POINT('Ctrl Pts',(1.7871392867044E-11,9.46324888737968,
9.92453123331945));
#13936=CARTESIAN_POINT('Ctrl Pts',(5.7299307791557,9.63824888737968,9.92453123330913));
#13937=CARTESIAN_POINT('Ctrl Pts',(8.59489616871569,9.81324888737969,4.96226561664425));
#13938=CARTESIAN_POINT('Ctrl Pts',(11.4598615582757,9.9882488873797,-2.06354052510241E-11));
#13939=CARTESIAN_POINT('Ctrl Pts',(8.59489616869782,10.1632488873797,-4.9622656166752));
#13940=CARTESIAN_POINT('Ctrl Pts',(5.72993077911996,10.3382488873797,-9.92453123332976));
#13941=CARTESIAN_POINT('Ctrl Pts',(-1.78726082715848E-11,10.5132488873797,
-9.92453123331945));
#13942=CARTESIAN_POINT('Ctrl Pts',(-5.7299307791557,10.6882488873797,-9.92453123330913));
#13943=CARTESIAN_POINT('Ctrl Pts',(-8.59489616871569,10.8632488873797,-4.96226561664425));
#13944=CARTESIAN_POINT('Ctrl Pts',(-11.4598615582757,11.0382488873797,2.06368086793017E-11));
#13945=CARTESIAN_POINT('Ctrl Pts',(-8.59489616869782,11.2132488873797,4.9622656166752));
#13946=CARTESIAN_POINT('Ctrl Pts',(-5.72993077911996,11.3882488873797,9.92453123332977));
#13947=CARTESIAN_POINT('Ctrl Pts',(1.7871392867044E-11,11.5632488873797,
9.92453123331945));
#13948=CARTESIAN_POINT('Ctrl Pts',(5.7299307791557,11.7382488873797,9.92453123330913));
#13949=CARTESIAN_POINT('Ctrl Pts',(8.59489616871569,11.9132488873797,4.96226561664425));
#13950=CARTESIAN_POINT('Ctrl Pts',(11.4598615582757,12.0882488873797,-2.06354052510241E-11));
#13951=CARTESIAN_POINT('Ctrl Pts',(8.59489616869782,12.2632488873797,-4.9622656166752));
#13952=CARTESIAN_POINT('Ctrl Pts',(5.72993077911996,12.4382488873797,-9.92453123332976));
#13953=CARTESIAN_POINT('Ctrl Pts',(-1.78726082715848E-11,12.6132488873797,
-9.92453123331945));
#13954=CARTESIAN_POINT('Ctrl Pts',(-5.7299307791557,12.7882488873797,-9.92453123330913));
#13955=CARTESIAN_POINT('Ctrl Pts',(-8.59489616871569,12.9632488873797,-4.96226561664425));
#13956=CARTESIAN_POINT('Ctrl Pts',(-11.4598615582757,13.1382488873797,2.06368086793017E-11));
#13957=CARTESIAN_POINT('Ctrl Pts',(-8.59489616869782,13.3132488873797,4.9622656166752));
#13958=CARTESIAN_POINT('Ctrl Pts',(-5.72993077911996,13.4882488873797,9.92453123332977));
#13959=CARTESIAN_POINT('Ctrl Pts',(1.7871392867044E-11,13.6632488873797,
9.92453123331945));
#13960=CARTESIAN_POINT('Ctrl Pts',(5.7299307791557,13.8382488873797,9.92453123330913));
#13961=CARTESIAN_POINT('Ctrl Pts',(8.59489616871569,14.0132488873797,4.96226561664425));
#13962=CARTESIAN_POINT('Ctrl Pts',(11.4598615582757,14.1882488873797,-2.06354052510241E-11));
#13963=CARTESIAN_POINT('Ctrl Pts',(8.59489616869782,14.3632488873797,-4.9622656166752));
#13964=CARTESIAN_POINT('Ctrl Pts',(5.72993077911996,14.5382488873797,-9.92453123332976));
#13965=CARTESIAN_POINT('Ctrl Pts',(-1.78726082715848E-11,14.7132488873797,
-9.92453123331945));
#13966=CARTESIAN_POINT('Ctrl Pts',(-5.7299307791557,14.8882488873797,-9.92453123330913));
#13967=CARTESIAN_POINT('Ctrl Pts',(-8.59489616871569,15.0632488873797,-4.96226561664425));
#13968=CARTESIAN_POINT('Ctrl Pts',(-11.4598615582757,15.2382488873797,2.06368086793017E-11));
#13969=CARTESIAN_POINT('Ctrl Pts',(-8.59489616869782,15.4132488873797,4.9622656166752));
#13970=CARTESIAN_POINT('Ctrl Pts',(-5.72993077911996,15.5882488873797,9.92453123332977));
#13971=CARTESIAN_POINT('Ctrl Pts',(1.7871392867044E-11,15.7632488873797,
9.92453123331945));
#13972=CARTESIAN_POINT('Ctrl Pts',(5.7299307791557,15.9382488873797,9.92453123330913));
#13973=CARTESIAN_POINT('Ctrl Pts',(8.59489616871569,16.1132488873797,4.96226561664425));
#13974=CARTESIAN_POINT('Ctrl Pts',(11.4598615582757,16.2882488873797,-2.06354052510241E-11));
#13975=CARTESIAN_POINT('Ctrl Pts',(8.59489616869782,16.4632488873797,-4.9622656166752));
#13976=CARTESIAN_POINT('Ctrl Pts',(5.72993077911996,16.6382488873797,-9.92453123332976));
#13977=CARTESIAN_POINT('Ctrl Pts',(-1.78726082715848E-11,16.8132488873797,
-9.92453123331945));
#13978=CARTESIAN_POINT('Ctrl Pts',(-5.7299307791557,16.9882488873797,-9.92453123330913));
#13979=CARTESIAN_POINT('Ctrl Pts',(-8.59489616871569,17.1632488873797,-4.96226561664425));
#13980=CARTESIAN_POINT('Ctrl Pts',(-11.4598615582757,17.3382488873797,2.06368086793017E-11));
#13981=CARTESIAN_POINT('Ctrl Pts',(-8.59489616869782,17.5132488873797,4.9622656166752));
#13982=CARTESIAN_POINT('Ctrl Pts',(-5.72993077911996,17.6882488873797,9.92453123332977));
#13983=CARTESIAN_POINT('Ctrl Pts',(1.7871392867044E-11,17.8632488873797,
9.92453123331945));
#13984=CARTESIAN_POINT('Ctrl Pts',(5.7299307791557,18.0382488873797,9.92453123330913));
#13985=CARTESIAN_POINT('Ctrl Pts',(8.59489616871569,18.2132488873797,4.96226561664425));
#13986=CARTESIAN_POINT('Ctrl Pts',(11.4598615582757,18.3882488873797,-2.06354052510241E-11));
#13987=CARTESIAN_POINT('Ctrl Pts',(8.59489616869782,18.5632488873797,-4.9622656166752));
#13988=CARTESIAN_POINT('Ctrl Pts',(5.72993077911996,18.7382488873797,-9.92453123332976));
#13989=CARTESIAN_POINT('Ctrl Pts',(-1.78726082715848E-11,18.9132488873797,
-9.92453123331945));
#13990=CARTESIAN_POINT('Ctrl Pts',(-5.7299307791557,19.0882488873797,-9.92453123330913));
#13991=CARTESIAN_POINT('Ctrl Pts',(-8.59489616871569,19.2632488873797,-4.96226561664425));
#13992=CARTESIAN_POINT('Ctrl Pts',(-11.4598615582757,19.4382488873797,2.06368086793017E-11));
#13993=CARTESIAN_POINT('Ctrl Pts',(-8.59489616869782,19.6132488873797,4.9622656166752));
#13994=CARTESIAN_POINT('Ctrl Pts',(-5.72993077911996,19.7882488873797,9.92453123332977));
#13995=CARTESIAN_POINT('Ctrl Pts',(1.7871392867044E-11,19.9632488873797,
9.92453123331945));
#13996=CARTESIAN_POINT('Ctrl Pts',(5.7299307791557,20.1382488873797,9.92453123330913));
#13997=CARTESIAN_POINT('Ctrl Pts',(8.59489616871569,20.3132488873797,4.96226561664425));
#13998=CARTESIAN_POINT('Ctrl Pts',(11.4598615582757,20.4882488873796,-2.06354052510241E-11));
#13999=CARTESIAN_POINT('Ctrl Pts',(8.59489616869782,20.6632488873797,-4.9622656166752));
#14000=CARTESIAN_POINT('Ctrl Pts',(5.72993077911996,20.8382488873797,-9.92453123332976));
#14001=CARTESIAN_POINT('Ctrl Pts',(-1.78726082715848E-11,21.0132488873797,
-9.92453123331945));
#14002=CARTESIAN_POINT('Ctrl Pts',(-5.7299307791557,21.1882488873797,-9.92453123330913));
#14003=CARTESIAN_POINT('Ctrl Pts',(-8.59489616871569,21.3632488873797,-4.96226561664425));
#14004=CARTESIAN_POINT('Ctrl Pts',(-11.4598615582757,21.5382488873796,2.06368086793017E-11));
#14005=CARTESIAN_POINT('Ctrl Pts',(-8.59489616869782,21.7132488873797,4.9622656166752));
#14006=CARTESIAN_POINT('Ctrl Pts',(-5.72993077911996,21.8882488873797,9.92453123332977));
#14007=CARTESIAN_POINT('Ctrl Pts',(1.7871392867044E-11,22.0632488873797,
9.92453123331945));
#14008=CARTESIAN_POINT('Ctrl Pts',(5.7299307791557,22.2382488873797,9.92453123330913));
#14009=CARTESIAN_POINT('Ctrl Pts',(8.59489616871569,22.4132488873797,4.96226561664425));
#14010=CARTESIAN_POINT('Ctrl Pts',(11.4598615582757,22.5882488873796,-2.06354052510241E-11));
#14011=CARTESIAN_POINT('Ctrl Pts',(8.59489616869782,22.7632488873797,-4.9622656166752));
#14012=CARTESIAN_POINT('Ctrl Pts',(5.72993077911996,22.9382488873797,-9.92453123332976));
#14013=CARTESIAN_POINT('Ctrl Pts',(-1.78726082715848E-11,23.1132488873796,
-9.92453123331945));
#14014=CARTESIAN_POINT('Ctrl Pts',(-5.7299307791557,23.2882488873797,-9.92453123330913));
#14015=CARTESIAN_POINT('Ctrl Pts',(-8.59489616871569,23.4632488873797,-4.96226561664425));
#14016=CARTESIAN_POINT('Ctrl Pts',(-11.4598615582757,23.6382488873797,2.06368086793017E-11));
#14017=CARTESIAN_POINT('Ctrl Pts',(-8.59489616869782,23.8132488873797,4.9622656166752));
#14018=CARTESIAN_POINT('Ctrl Pts',(-5.72993077911996,23.9882488873797,9.92453123332977));
#14019=CARTESIAN_POINT('Ctrl Pts',(1.7871392867044E-11,24.1632488873797,
9.92453123331945));
#14020=CARTESIAN_POINT('Ctrl Pts',(5.7299307791557,24.3382488873796,9.92453123330913));
#14021=CARTESIAN_POINT('Ctrl Pts',(8.59489616871569,24.5132488873797,4.96226561664425));
#14022=CARTESIAN_POINT('Ctrl Pts',(11.4598615582757,24.6882488873797,-2.06354052510241E-11));
#14023=CARTESIAN_POINT('Ctrl Pts',(8.59489616869782,24.8632488873796,-4.9622656166752));
#14024=CARTESIAN_POINT('Ctrl Pts',(5.72993077911996,25.0382488873797,-9.92453123332976));
#14025=CARTESIAN_POINT('Ctrl Pts',(-1.78726082715848E-11,25.2132488873797,
-9.92453123331945));
#14026=CARTESIAN_POINT('Ctrl Pts',(-1.5130096486293E-11,-144.093981044533,
-8.40163410172683));
#14027=CARTESIAN_POINT('Ctrl Pts',(-4.85068571027985,-143.918981044533,
-8.40163410171809));
#14028=CARTESIAN_POINT('Ctrl Pts',(-7.27602856540465,-143.743981044533,
-4.20081705085031));
#14029=CARTESIAN_POINT('Ctrl Pts',(-9.70137142052945,-143.568981044533,
1.74701365207797E-11));
#14030=CARTESIAN_POINT('Ctrl Pts',(-7.27602856538952,-143.393981044533,
4.20081705087652));
#14031=CARTESIAN_POINT('Ctrl Pts',(-4.8506857102496,-143.218981044533,8.40163410173556));
#14032=CARTESIAN_POINT('Ctrl Pts',(1.5129067582862E-11,-143.043981044533,
8.40163410172683));
#14033=CARTESIAN_POINT('Ctrl Pts',(4.85068571027985,-142.868981044533,8.40163410171809));
#14034=CARTESIAN_POINT('Ctrl Pts',(7.27602856540465,-142.693981044533,4.20081705085031));
#14035=CARTESIAN_POINT('Ctrl Pts',(9.70137142052945,-142.518981044533,-1.7468948445434E-11));
#14036=CARTESIAN_POINT('Ctrl Pts',(7.27602856538952,-142.343981044533,-4.20081705087651));
#14037=CARTESIAN_POINT('Ctrl Pts',(4.8506857102496,-142.168981044533,-8.40163410173556));
#14038=CARTESIAN_POINT('Ctrl Pts',(-1.5130096486293E-11,-141.993981044533,
-8.40163410172683));
#14039=CARTESIAN_POINT('Ctrl Pts',(-4.85068571027985,-141.818981044533,
-8.40163410171809));
#14040=CARTESIAN_POINT('Ctrl Pts',(-7.27602856540465,-141.643981044533,
-4.20081705085031));
#14041=CARTESIAN_POINT('Ctrl Pts',(-9.70137142052945,-141.468981044533,
1.74701365207797E-11));
#14042=CARTESIAN_POINT('Ctrl Pts',(-7.27602856538952,-141.293981044533,
4.20081705087652));
#14043=CARTESIAN_POINT('Ctrl Pts',(-4.8506857102496,-141.118981044533,8.40163410173556));
#14044=CARTESIAN_POINT('Ctrl Pts',(1.5129067582862E-11,-140.943981044533,
8.40163410172683));
#14045=CARTESIAN_POINT('Ctrl Pts',(4.85068571027985,-140.768981044533,8.40163410171809));
#14046=CARTESIAN_POINT('Ctrl Pts',(7.27602856540465,-140.593981044533,4.20081705085031));
#14047=CARTESIAN_POINT('Ctrl Pts',(9.70137142052945,-140.418981044533,-1.7468948445434E-11));
#14048=CARTESIAN_POINT('Ctrl Pts',(7.27602856538952,-140.243981044533,-4.20081705087651));
#14049=CARTESIAN_POINT('Ctrl Pts',(4.8506857102496,-140.068981044533,-8.40163410173556));
#14050=CARTESIAN_POINT('Ctrl Pts',(-1.5130096486293E-11,-139.893981044533,
-8.40163410172683));
#14051=CARTESIAN_POINT('Ctrl Pts',(-4.85068571027985,-139.718981044533,
-8.40163410171809));
#14052=CARTESIAN_POINT('Ctrl Pts',(-7.27602856540465,-139.543981044533,
-4.20081705085031));
#14053=CARTESIAN_POINT('Ctrl Pts',(-9.70137142052945,-139.368981044533,
1.74701365207797E-11));
#14054=CARTESIAN_POINT('Ctrl Pts',(-7.27602856538952,-139.193981044533,
4.20081705087652));
#14055=CARTESIAN_POINT('Ctrl Pts',(-4.8506857102496,-139.018981044533,8.40163410173556));
#14056=CARTESIAN_POINT('Ctrl Pts',(1.5129067582862E-11,-138.843981044533,
8.40163410172683));
#14057=CARTESIAN_POINT('Ctrl Pts',(4.85068571027985,-138.668981044533,8.40163410171809));
#14058=CARTESIAN_POINT('Ctrl Pts',(7.27602856540465,-138.493981044533,4.20081705085031));
#14059=CARTESIAN_POINT('Ctrl Pts',(9.70137142052945,-138.318981044533,-1.7468948445434E-11));
#14060=CARTESIAN_POINT('Ctrl Pts',(7.27602856538952,-138.143981044533,-4.20081705087651));
#14061=CARTESIAN_POINT('Ctrl Pts',(4.8506857102496,-137.968981044533,-8.40163410173556));
#14062=CARTESIAN_POINT('Ctrl Pts',(-1.5130096486293E-11,-137.793981044533,
-8.40163410172683));
#14063=CARTESIAN_POINT('Ctrl Pts',(-4.85068571027985,-137.618981044533,
-8.40163410171809));
#14064=CARTESIAN_POINT('Ctrl Pts',(-7.27602856540465,-137.443981044533,
-4.20081705085031));
#14065=CARTESIAN_POINT('Ctrl Pts',(-9.70137142052945,-137.268981044533,
1.74701365207797E-11));
#14066=CARTESIAN_POINT('Ctrl Pts',(-7.27602856538952,-137.093981044533,
4.20081705087652));
#14067=CARTESIAN_POINT('Ctrl Pts',(-4.8506857102496,-136.918981044533,8.40163410173556));
#14068=CARTESIAN_POINT('Ctrl Pts',(1.5129067582862E-11,-136.743981044533,
8.40163410172683));
#14069=CARTESIAN_POINT('Ctrl Pts',(4.85068571027985,-136.568981044533,8.40163410171809));
#14070=CARTESIAN_POINT('Ctrl Pts',(7.27602856540465,-136.393981044533,4.20081705085031));
#14071=CARTESIAN_POINT('Ctrl Pts',(9.70137142052945,-136.218981044533,-1.7468948445434E-11));
#14072=CARTESIAN_POINT('Ctrl Pts',(7.27602856538952,-136.043981044533,-4.20081705087651));
#14073=CARTESIAN_POINT('Ctrl Pts',(4.8506857102496,-135.868981044533,-8.40163410173556));
#14074=CARTESIAN_POINT('Ctrl Pts',(-1.5130096486293E-11,-135.693981044533,
-8.40163410172683));
#14075=CARTESIAN_POINT('Ctrl Pts',(-4.85068571027985,-135.518981044533,
-8.40163410171809));
#14076=CARTESIAN_POINT('Ctrl Pts',(-7.27602856540465,-135.343981044533,
-4.20081705085031));
#14077=CARTESIAN_POINT('Ctrl Pts',(-9.70137142052945,-135.168981044533,
1.74701365207797E-11));
#14078=CARTESIAN_POINT('Ctrl Pts',(-7.27602856538952,-134.993981044533,
4.20081705087652));
#14079=CARTESIAN_POINT('Ctrl Pts',(-4.8506857102496,-134.818981044533,8.40163410173556));
#14080=CARTESIAN_POINT('Ctrl Pts',(1.5129067582862E-11,-134.643981044533,
8.40163410172683));
#14081=CARTESIAN_POINT('Ctrl Pts',(4.85068571027985,-134.468981044533,8.40163410171809));
#14082=CARTESIAN_POINT('Ctrl Pts',(7.27602856540465,-134.293981044533,4.20081705085031));
#14083=CARTESIAN_POINT('Ctrl Pts',(9.70137142052945,-134.118981044533,-1.7468948445434E-11));
#14084=CARTESIAN_POINT('Ctrl Pts',(7.27602856538952,-133.943981044533,-4.20081705087651));
#14085=CARTESIAN_POINT('Ctrl Pts',(4.8506857102496,-133.768981044533,-8.40163410173556));
#14086=CARTESIAN_POINT('Ctrl Pts',(-1.5130096486293E-11,-133.593981044533,
-8.40163410172683));
#14087=CARTESIAN_POINT('Ctrl Pts',(-4.85068571027985,-133.418981044533,
-8.40163410171809));
#14088=CARTESIAN_POINT('Ctrl Pts',(-7.27602856540465,-133.243981044533,
-4.20081705085031));
#14089=CARTESIAN_POINT('Ctrl Pts',(-9.70137142052945,-133.068981044533,
1.74701365207797E-11));
#14090=CARTESIAN_POINT('Ctrl Pts',(-7.27602856538952,-132.893981044533,
4.20081705087652));
#14091=CARTESIAN_POINT('Ctrl Pts',(-4.8506857102496,-132.718981044533,8.40163410173556));
#14092=CARTESIAN_POINT('Ctrl Pts',(1.5129067582862E-11,-132.543981044533,
8.40163410172683));
#14093=CARTESIAN_POINT('Ctrl Pts',(4.85068571027985,-132.368981044533,8.40163410171809));
#14094=CARTESIAN_POINT('Ctrl Pts',(7.27602856540465,-132.193981044533,4.20081705085031));
#14095=CARTESIAN_POINT('Ctrl Pts',(9.70137142052945,-132.018981044533,-1.7468948445434E-11));
#14096=CARTESIAN_POINT('Ctrl Pts',(7.27602856538952,-131.843981044533,-4.20081705087651));
#14097=CARTESIAN_POINT('Ctrl Pts',(4.8506857102496,-131.668981044533,-8.40163410173556));
#14098=CARTESIAN_POINT('Ctrl Pts',(-1.5130096486293E-11,-131.493981044533,
-8.40163410172683));
#14099=CARTESIAN_POINT('Ctrl Pts',(-4.85068571027985,-131.318981044533,
-8.40163410171809));
#14100=CARTESIAN_POINT('Ctrl Pts',(-7.27602856540465,-131.143981044533,
-4.20081705085031));
#14101=CARTESIAN_POINT('Ctrl Pts',(-9.70137142052945,-130.968981044533,
1.74701365207797E-11));
#14102=CARTESIAN_POINT('Ctrl Pts',(-7.27602856538952,-130.793981044533,
4.20081705087652));
#14103=CARTESIAN_POINT('Ctrl Pts',(-4.8506857102496,-130.618981044533,8.40163410173556));
#14104=CARTESIAN_POINT('Ctrl Pts',(1.5129067582862E-11,-130.443981044533,
8.40163410172683));
#14105=CARTESIAN_POINT('Ctrl Pts',(4.85068571027985,-130.268981044533,8.40163410171809));
#14106=CARTESIAN_POINT('Ctrl Pts',(7.27602856540465,-130.093981044533,4.20081705085031));
#14107=CARTESIAN_POINT('Ctrl Pts',(9.70137142052945,-129.918981044533,-1.7468948445434E-11));
#14108=CARTESIAN_POINT('Ctrl Pts',(7.27602856538952,-129.743981044533,-4.20081705087651));
#14109=CARTESIAN_POINT('Ctrl Pts',(4.8506857102496,-129.568981044533,-8.40163410173556));
#14110=CARTESIAN_POINT('Ctrl Pts',(-1.5130096486293E-11,-129.393981044533,
-8.40163410172683));
#14111=CARTESIAN_POINT('Ctrl Pts',(-4.85068571027985,-129.218981044533,
-8.40163410171809));
#14112=CARTESIAN_POINT('Ctrl Pts',(-7.27602856540465,-129.043981044533,
-4.20081705085031));
#14113=CARTESIAN_POINT('Ctrl Pts',(-9.70137142052945,-128.868981044533,
1.74701365207797E-11));
#14114=CARTESIAN_POINT('Ctrl Pts',(-7.27602856538952,-128.693981044533,
4.20081705087652));
#14115=CARTESIAN_POINT('Ctrl Pts',(-4.8506857102496,-128.518981044533,8.40163410173556));
#14116=CARTESIAN_POINT('Ctrl Pts',(1.5129067582862E-11,-128.343981044533,
8.40163410172683));
#14117=CARTESIAN_POINT('Ctrl Pts',(4.85068571027985,-128.168981044533,8.40163410171809));
#14118=CARTESIAN_POINT('Ctrl Pts',(7.27602856540465,-127.993981044533,4.20081705085031));
#14119=CARTESIAN_POINT('Ctrl Pts',(9.70137142052945,-127.818981044533,-1.7468948445434E-11));
#14120=CARTESIAN_POINT('Ctrl Pts',(7.27602856538952,-127.643981044533,-4.20081705087651));
#14121=CARTESIAN_POINT('Ctrl Pts',(4.8506857102496,-127.468981044533,-8.40163410173556));
#14122=CARTESIAN_POINT('Ctrl Pts',(-1.5130096486293E-11,-127.293981044533,
-8.40163410172683));
#14123=CARTESIAN_POINT('Ctrl Pts',(-4.85068571027985,-127.118981044533,
-8.40163410171809));
#14124=CARTESIAN_POINT('Ctrl Pts',(-7.27602856540465,-126.943981044533,
-4.20081705085031));
#14125=CARTESIAN_POINT('Ctrl Pts',(-9.70137142052945,-126.768981044533,
1.74701365207797E-11));
#14126=CARTESIAN_POINT('Ctrl Pts',(-7.27602856538952,-126.593981044533,
4.20081705087652));
#14127=CARTESIAN_POINT('Ctrl Pts',(-4.8506857102496,-126.418981044533,8.40163410173556));
#14128=CARTESIAN_POINT('Ctrl Pts',(1.5129067582862E-11,-126.243981044533,
8.40163410172683));
#14129=CARTESIAN_POINT('Ctrl Pts',(4.85068571027985,-126.068981044533,8.40163410171809));
#14130=CARTESIAN_POINT('Ctrl Pts',(7.27602856540465,-125.893981044533,4.20081705085031));
#14131=CARTESIAN_POINT('Ctrl Pts',(9.70137142052945,-125.718981044533,-1.7468948445434E-11));
#14132=CARTESIAN_POINT('Ctrl Pts',(7.27602856538952,-125.543981044533,-4.20081705087651));
#14133=CARTESIAN_POINT('Ctrl Pts',(4.8506857102496,-125.368981044533,-8.40163410173556));
#14134=CARTESIAN_POINT('Ctrl Pts',(-1.5130096486293E-11,-125.193981044533,
-8.40163410172683));
#14135=CARTESIAN_POINT('Ctrl Pts',(-4.85068571027985,-125.018981044533,
-8.40163410171809));
#14136=CARTESIAN_POINT('Ctrl Pts',(-7.27602856540465,-124.843981044533,
-4.20081705085031));
#14137=CARTESIAN_POINT('Ctrl Pts',(-9.70137142052945,-124.668981044533,
1.74701365207797E-11));
#14138=CARTESIAN_POINT('Ctrl Pts',(-7.27602856538952,-124.493981044533,
4.20081705087652));
#14139=CARTESIAN_POINT('Ctrl Pts',(-4.8506857102496,-124.318981044533,8.40163410173556));
#14140=CARTESIAN_POINT('Ctrl Pts',(1.5129067582862E-11,-124.143981044533,
8.40163410172683));
#14141=CARTESIAN_POINT('Ctrl Pts',(4.85068571027985,-123.968981044533,8.40163410171809));
#14142=CARTESIAN_POINT('Ctrl Pts',(7.27602856540465,-123.793981044533,4.20081705085031));
#14143=CARTESIAN_POINT('Ctrl Pts',(9.70137142052945,-123.618981044533,-1.7468948445434E-11));
#14144=CARTESIAN_POINT('Ctrl Pts',(7.27602856538952,-123.443981044533,-4.20081705087651));
#14145=CARTESIAN_POINT('Ctrl Pts',(4.8506857102496,-123.268981044533,-8.40163410173556));
#14146=CARTESIAN_POINT('Ctrl Pts',(-1.5130096486293E-11,-123.093981044533,
-8.40163410172683));
#14147=CARTESIAN_POINT('Ctrl Pts',(-4.85068571027985,-122.918981044533,
-8.40163410171809));
#14148=CARTESIAN_POINT('Ctrl Pts',(-7.27602856540465,-122.743981044533,
-4.20081705085031));
#14149=CARTESIAN_POINT('Ctrl Pts',(-9.70137142052945,-122.568981044533,
1.74701365207797E-11));
#14150=CARTESIAN_POINT('Ctrl Pts',(-7.27602856538952,-122.393981044533,
4.20081705087652));
#14151=CARTESIAN_POINT('Ctrl Pts',(-4.8506857102496,-122.218981044533,8.40163410173556));
#14152=CARTESIAN_POINT('Ctrl Pts',(1.5129067582862E-11,-122.043981044533,
8.40163410172683));
#14153=CARTESIAN_POINT('Ctrl Pts',(4.85068571027985,-121.868981044533,8.40163410171809));
#14154=CARTESIAN_POINT('Ctrl Pts',(7.27602856540465,-121.693981044533,4.20081705085031));
#14155=CARTESIAN_POINT('Ctrl Pts',(9.70137142052945,-121.518981044533,-1.7468948445434E-11));
#14156=CARTESIAN_POINT('Ctrl Pts',(7.27602856538952,-121.343981044533,-4.20081705087651));
#14157=CARTESIAN_POINT('Ctrl Pts',(4.8506857102496,-121.168981044533,-8.40163410173556));
#14158=CARTESIAN_POINT('Ctrl Pts',(-1.5130096486293E-11,-120.993981044533,
-8.40163410172683));
#14159=CARTESIAN_POINT('Ctrl Pts',(-4.85068571027985,-120.818981044533,
-8.40163410171809));
#14160=CARTESIAN_POINT('Ctrl Pts',(-7.27602856540465,-120.643981044533,
-4.20081705085031));
#14161=CARTESIAN_POINT('Ctrl Pts',(-9.70137142052945,-120.468981044533,
1.74701365207797E-11));
#14162=CARTESIAN_POINT('Ctrl Pts',(-7.27602856538952,-120.293981044533,
4.20081705087652));
#14163=CARTESIAN_POINT('Ctrl Pts',(-4.8506857102496,-120.118981044533,8.40163410173556));
#14164=CARTESIAN_POINT('Ctrl Pts',(1.5129067582862E-11,-119.943981044533,
8.40163410172683));
#14165=CARTESIAN_POINT('Ctrl Pts',(4.85068571027985,-119.768981044533,8.40163410171809));
#14166=CARTESIAN_POINT('Ctrl Pts',(7.27602856540465,-119.593981044533,4.20081705085031));
#14167=CARTESIAN_POINT('Ctrl Pts',(9.70137142052945,-119.418981044533,-1.7468948445434E-11));
#14168=CARTESIAN_POINT('Ctrl Pts',(7.27602856538952,-119.243981044533,-4.20081705087651));
#14169=CARTESIAN_POINT('Ctrl Pts',(4.8506857102496,-119.068981044533,-8.40163410173556));
#14170=CARTESIAN_POINT('Ctrl Pts',(-1.5130096486293E-11,-118.893981044533,
-8.40163410172683));
#14171=CARTESIAN_POINT('Ctrl Pts',(-4.85068571027985,-118.718981044533,
-8.40163410171809));
#14172=CARTESIAN_POINT('Ctrl Pts',(-7.27602856540465,-118.543981044533,
-4.20081705085031));
#14173=CARTESIAN_POINT('Ctrl Pts',(-9.70137142052945,-118.368981044533,
1.74701365207797E-11));
#14174=CARTESIAN_POINT('Ctrl Pts',(-7.27602856538952,-118.193981044533,
4.20081705087652));
#14175=CARTESIAN_POINT('Ctrl Pts',(-4.8506857102496,-118.018981044533,8.40163410173556));
#14176=CARTESIAN_POINT('Ctrl Pts',(1.5129067582862E-11,-117.843981044533,
8.40163410172683));
#14177=CARTESIAN_POINT('Ctrl Pts',(4.85068571027985,-117.668981044533,8.40163410171809));
#14178=CARTESIAN_POINT('Ctrl Pts',(7.27602856540465,-117.493981044533,4.20081705085031));
#14179=CARTESIAN_POINT('Ctrl Pts',(9.70137142052945,-117.318981044533,-1.7468948445434E-11));
#14180=CARTESIAN_POINT('Ctrl Pts',(7.27602856538952,-117.143981044533,-4.20081705087651));
#14181=CARTESIAN_POINT('Ctrl Pts',(4.8506857102496,-116.968981044533,-8.40163410173556));
#14182=CARTESIAN_POINT('Ctrl Pts',(-1.5130096486293E-11,-116.793981044533,
-8.40163410172683));
#14183=CARTESIAN_POINT('Ctrl Pts',(-4.85068571027985,-116.618981044533,
-8.40163410171809));
#14184=CARTESIAN_POINT('Ctrl Pts',(-7.27602856540465,-116.443981044533,
-4.20081705085031));
#14185=CARTESIAN_POINT('Ctrl Pts',(-9.70137142052945,-116.268981044533,
1.74701365207797E-11));
#14186=CARTESIAN_POINT('Ctrl Pts',(-7.27602856538952,-116.093981044533,
4.20081705087652));
#14187=CARTESIAN_POINT('Ctrl Pts',(-4.8506857102496,-115.918981044533,8.40163410173556));
#14188=CARTESIAN_POINT('Ctrl Pts',(1.5129067582862E-11,-115.743981044533,
8.40163410172683));
#14189=CARTESIAN_POINT('Ctrl Pts',(4.85068571027985,-115.568981044533,8.40163410171809));
#14190=CARTESIAN_POINT('Ctrl Pts',(7.27602856540465,-115.393981044533,4.20081705085031));
#14191=CARTESIAN_POINT('Ctrl Pts',(9.70137142052945,-115.218981044533,-1.7468948445434E-11));
#14192=CARTESIAN_POINT('Ctrl Pts',(7.27602856538952,-115.043981044533,-4.20081705087651));
#14193=CARTESIAN_POINT('Ctrl Pts',(4.8506857102496,-114.868981044533,-8.40163410173556));
#14194=CARTESIAN_POINT('Ctrl Pts',(-1.5130096486293E-11,-114.693981044533,
-8.40163410172683));
#14195=CARTESIAN_POINT('Ctrl Pts',(-4.85068571027985,-114.518981044533,
-8.40163410171809));
#14196=CARTESIAN_POINT('Ctrl Pts',(-7.27602856540465,-114.343981044533,
-4.20081705085031));
#14197=CARTESIAN_POINT('Ctrl Pts',(-9.70137142052945,-114.168981044533,
1.74701365207797E-11));
#14198=CARTESIAN_POINT('Ctrl Pts',(-7.27602856538952,-113.993981044533,
4.20081705087652));
#14199=CARTESIAN_POINT('Ctrl Pts',(-4.8506857102496,-113.818981044533,8.40163410173556));
#14200=CARTESIAN_POINT('Ctrl Pts',(1.5129067582862E-11,-113.643981044533,
8.40163410172683));
#14201=CARTESIAN_POINT('Ctrl Pts',(4.85068571027985,-113.468981044533,8.40163410171809));
#14202=CARTESIAN_POINT('Ctrl Pts',(7.27602856540465,-113.293981044533,4.20081705085031));
#14203=CARTESIAN_POINT('Ctrl Pts',(9.70137142052945,-113.118981044533,-1.7468948445434E-11));
#14204=CARTESIAN_POINT('Ctrl Pts',(7.27602856538952,-112.943981044533,-4.20081705087651));
#14205=CARTESIAN_POINT('Ctrl Pts',(4.8506857102496,-112.768981044533,-8.40163410173556));
#14206=CARTESIAN_POINT('Ctrl Pts',(-1.5130096486293E-11,-112.593981044533,
-8.40163410172683));
#14207=CARTESIAN_POINT('Ctrl Pts',(-4.85068571027985,-112.418981044533,
-8.40163410171809));
#14208=CARTESIAN_POINT('Ctrl Pts',(-7.27602856540465,-112.243981044533,
-4.20081705085031));
#14209=CARTESIAN_POINT('Ctrl Pts',(-9.70137142052945,-112.068981044533,
1.74701365207797E-11));
#14210=CARTESIAN_POINT('Ctrl Pts',(-7.27602856538952,-111.893981044533,
4.20081705087652));
#14211=CARTESIAN_POINT('Ctrl Pts',(-4.8506857102496,-111.718981044533,8.40163410173556));
#14212=CARTESIAN_POINT('Ctrl Pts',(1.5129067582862E-11,-111.543981044533,
8.40163410172683));
#14213=CARTESIAN_POINT('Ctrl Pts',(4.85068571027985,-111.368981044533,8.40163410171809));
#14214=CARTESIAN_POINT('Ctrl Pts',(7.27602856540465,-111.193981044533,4.20081705085031));
#14215=CARTESIAN_POINT('Ctrl Pts',(9.70137142052945,-111.018981044533,-1.7468948445434E-11));
#14216=CARTESIAN_POINT('Ctrl Pts',(7.27602856538952,-110.843981044533,-4.20081705087651));
#14217=CARTESIAN_POINT('Ctrl Pts',(4.8506857102496,-110.668981044533,-8.40163410173556));
#14218=CARTESIAN_POINT('Ctrl Pts',(-1.5130096486293E-11,-110.493981044533,
-8.40163410172683));
#14219=CARTESIAN_POINT('Ctrl Pts',(-4.85068571027985,-110.318981044533,
-8.40163410171809));
#14220=CARTESIAN_POINT('Ctrl Pts',(-7.27602856540465,-110.143981044533,
-4.20081705085031));
#14221=CARTESIAN_POINT('Ctrl Pts',(-9.70137142052945,-109.968981044533,
1.74701365207797E-11));
#14222=CARTESIAN_POINT('Ctrl Pts',(-7.27602856538952,-109.793981044533,
4.20081705087652));
#14223=CARTESIAN_POINT('Ctrl Pts',(-4.8506857102496,-109.618981044533,8.40163410173556));
#14224=CARTESIAN_POINT('Ctrl Pts',(1.5129067582862E-11,-109.443981044533,
8.40163410172683));
#14225=CARTESIAN_POINT('Ctrl Pts',(4.85068571027985,-109.268981044533,8.40163410171809));
#14226=CARTESIAN_POINT('Ctrl Pts',(7.27602856540465,-109.093981044533,4.20081705085031));
#14227=CARTESIAN_POINT('Ctrl Pts',(9.70137142052945,-108.918981044533,-1.7468948445434E-11));
#14228=CARTESIAN_POINT('Ctrl Pts',(7.27602856538952,-108.743981044533,-4.20081705087651));
#14229=CARTESIAN_POINT('Ctrl Pts',(4.8506857102496,-108.568981044533,-8.40163410173556));
#14230=CARTESIAN_POINT('Ctrl Pts',(-1.5130096486293E-11,-108.393981044533,
-8.40163410172683));
#14231=CARTESIAN_POINT('Ctrl Pts',(-4.85068571027985,-108.218981044533,
-8.40163410171809));
#14232=CARTESIAN_POINT('Ctrl Pts',(-7.27602856540465,-108.043981044533,
-4.20081705085031));
#14233=CARTESIAN_POINT('Ctrl Pts',(-9.70137142052945,-107.868981044533,
1.74701365207797E-11));
#14234=CARTESIAN_POINT('Ctrl Pts',(-7.27602856538952,-107.693981044533,
4.20081705087652));
#14235=CARTESIAN_POINT('Ctrl Pts',(-4.8506857102496,-107.518981044533,8.40163410173556));
#14236=CARTESIAN_POINT('Ctrl Pts',(1.5129067582862E-11,-107.343981044533,
8.40163410172683));
#14237=CARTESIAN_POINT('Ctrl Pts',(4.85068571027985,-107.168981044533,8.40163410171809));
#14238=CARTESIAN_POINT('Ctrl Pts',(7.27602856540465,-106.993981044533,4.20081705085031));
#14239=CARTESIAN_POINT('Ctrl Pts',(9.70137142052945,-106.818981044533,-1.7468948445434E-11));
#14240=CARTESIAN_POINT('Ctrl Pts',(7.27602856538952,-106.643981044533,-4.20081705087651));
#14241=CARTESIAN_POINT('Ctrl Pts',(4.8506857102496,-106.468981044533,-8.40163410173556));
#14242=CARTESIAN_POINT('Ctrl Pts',(-1.5130096486293E-11,-106.293981044533,
-8.40163410172683));
#14243=CARTESIAN_POINT('Ctrl Pts',(-4.85068571027985,-106.118981044533,
-8.40163410171809));
#14244=CARTESIAN_POINT('Ctrl Pts',(-7.27602856540465,-105.943981044533,
-4.20081705085031));
#14245=CARTESIAN_POINT('Ctrl Pts',(-9.70137142052945,-105.768981044533,
1.74701365207797E-11));
#14246=CARTESIAN_POINT('Ctrl Pts',(-7.27602856538952,-105.593981044533,
4.20081705087652));
#14247=CARTESIAN_POINT('Ctrl Pts',(-4.8506857102496,-105.418981044533,8.40163410173556));
#14248=CARTESIAN_POINT('Ctrl Pts',(1.5129067582862E-11,-105.243981044533,
8.40163410172683));
#14249=CARTESIAN_POINT('Ctrl Pts',(4.85068571027985,-105.068981044533,8.40163410171809));
#14250=CARTESIAN_POINT('Ctrl Pts',(7.27602856540465,-104.893981044533,4.20081705085031));
#14251=CARTESIAN_POINT('Ctrl Pts',(9.70137142052945,-104.718981044533,-1.7468948445434E-11));
#14252=CARTESIAN_POINT('Ctrl Pts',(7.27602856538952,-104.543981044533,-4.20081705087651));
#14253=CARTESIAN_POINT('Ctrl Pts',(4.8506857102496,-104.368981044533,-8.40163410173556));
#14254=CARTESIAN_POINT('Ctrl Pts',(-1.5130096486293E-11,-104.193981044533,
-8.40163410172683));
#14255=CARTESIAN_POINT('Ctrl Pts',(-4.85068571027985,-104.018981044533,
-8.40163410171809));
#14256=CARTESIAN_POINT('Ctrl Pts',(-7.27602856540465,-103.843981044533,
-4.20081705085031));
#14257=CARTESIAN_POINT('Ctrl Pts',(-9.70137142052945,-103.668981044533,
1.74701365207797E-11));
#14258=CARTESIAN_POINT('Ctrl Pts',(-7.27602856538952,-103.493981044533,
4.20081705087652));
#14259=CARTESIAN_POINT('Ctrl Pts',(-4.8506857102496,-103.318981044533,8.40163410173556));
#14260=CARTESIAN_POINT('Ctrl Pts',(1.5129067582862E-11,-103.143981044533,
8.40163410172683));
#14261=CARTESIAN_POINT('Ctrl Pts',(4.85068571027985,-102.968981044533,8.40163410171809));
#14262=CARTESIAN_POINT('Ctrl Pts',(7.27602856540465,-102.793981044533,4.20081705085031));
#14263=CARTESIAN_POINT('Ctrl Pts',(9.70137142052945,-102.618981044533,-1.7468948445434E-11));
#14264=CARTESIAN_POINT('Ctrl Pts',(7.27602856538952,-102.443981044533,-4.20081705087651));
#14265=CARTESIAN_POINT('Ctrl Pts',(4.8506857102496,-102.268981044533,-8.40163410173556));
#14266=CARTESIAN_POINT('Ctrl Pts',(-1.5130096486293E-11,-102.093981044533,
-8.40163410172683));
#14267=CARTESIAN_POINT('Ctrl Pts',(-4.85068571027985,-101.918981044533,
-8.40163410171809));
#14268=CARTESIAN_POINT('Ctrl Pts',(-7.27602856540465,-101.743981044533,
-4.20081705085031));
#14269=CARTESIAN_POINT('Ctrl Pts',(-9.70137142052945,-101.568981044533,
1.74701365207797E-11));
#14270=CARTESIAN_POINT('Ctrl Pts',(-7.27602856538952,-101.393981044533,
4.20081705087652));
#14271=CARTESIAN_POINT('Ctrl Pts',(-4.8506857102496,-101.218981044533,8.40163410173556));
#14272=CARTESIAN_POINT('Ctrl Pts',(1.5129067582862E-11,-101.043981044533,
8.40163410172683));
#14273=CARTESIAN_POINT('Ctrl Pts',(4.85068571027985,-100.868981044533,8.40163410171809));
#14274=CARTESIAN_POINT('Ctrl Pts',(7.27602856540465,-100.693981044533,4.20081705085031));
#14275=CARTESIAN_POINT('Ctrl Pts',(9.70137142052945,-100.518981044533,-1.7468948445434E-11));
#14276=CARTESIAN_POINT('Ctrl Pts',(7.27602856538952,-100.343981044533,-4.20081705087651));
#14277=CARTESIAN_POINT('Ctrl Pts',(4.8506857102496,-100.168981044533,-8.40163410173556));
#14278=CARTESIAN_POINT('Ctrl Pts',(-1.5130096486293E-11,-99.9939810445332,
-8.40163410172683));
#14279=CARTESIAN_POINT('Ctrl Pts',(-4.85068571027985,-99.8189810445332,
-8.40163410171809));
#14280=CARTESIAN_POINT('Ctrl Pts',(-7.27602856540465,-99.6439810445332,
-4.20081705085031));
#14281=CARTESIAN_POINT('Ctrl Pts',(-9.70137142052945,-99.4689810445332,
1.74701365207797E-11));
#14282=CARTESIAN_POINT('Ctrl Pts',(-7.27602856538952,-99.2939810445332,
4.20081705087652));
#14283=CARTESIAN_POINT('Ctrl Pts',(-4.8506857102496,-99.1189810445332,8.40163410173556));
#14284=CARTESIAN_POINT('Ctrl Pts',(1.5129067582862E-11,-98.9439810445332,
8.40163410172683));
#14285=CARTESIAN_POINT('Ctrl Pts',(4.85068571027985,-98.7689810445332,8.40163410171809));
#14286=CARTESIAN_POINT('Ctrl Pts',(7.27602856540465,-98.5939810445332,4.20081705085031));
#14287=CARTESIAN_POINT('Ctrl Pts',(9.70137142052945,-98.4189810445332,-1.7468948445434E-11));
#14288=CARTESIAN_POINT('Ctrl Pts',(7.27602856538952,-98.2439810445332,-4.20081705087651));
#14289=CARTESIAN_POINT('Ctrl Pts',(4.8506857102496,-98.0689810445332,-8.40163410173556));
#14290=CARTESIAN_POINT('Ctrl Pts',(-1.5130096486293E-11,-97.8939810445332,
-8.40163410172683));
#14291=CARTESIAN_POINT('Ctrl Pts',(-4.85068571027985,-97.7189810445332,
-8.40163410171809));
#14292=CARTESIAN_POINT('Ctrl Pts',(-7.27602856540465,-97.5439810445332,
-4.20081705085031));
#14293=CARTESIAN_POINT('Ctrl Pts',(-9.70137142052945,-97.3689810445332,
1.74701365207797E-11));
#14294=CARTESIAN_POINT('Ctrl Pts',(-7.27602856538952,-97.1939810445332,
4.20081705087652));
#14295=CARTESIAN_POINT('Ctrl Pts',(-4.8506857102496,-97.0189810445332,8.40163410173556));
#14296=CARTESIAN_POINT('Ctrl Pts',(1.5129067582862E-11,-96.8439810445332,
8.40163410172683));
#14297=CARTESIAN_POINT('Ctrl Pts',(4.85068571027985,-96.6689810445332,8.40163410171809));
#14298=CARTESIAN_POINT('Ctrl Pts',(7.27602856540465,-96.4939810445332,4.20081705085031));
#14299=CARTESIAN_POINT('Ctrl Pts',(9.70137142052945,-96.3189810445332,-1.7468948445434E-11));
#14300=CARTESIAN_POINT('Ctrl Pts',(7.27602856538952,-96.1439810445332,-4.20081705087651));
#14301=CARTESIAN_POINT('Ctrl Pts',(4.8506857102496,-95.9689810445332,-8.40163410173556));
#14302=CARTESIAN_POINT('Ctrl Pts',(-1.5130096486293E-11,-95.7939810445332,
-8.40163410172683));
#14303=CARTESIAN_POINT('Ctrl Pts',(-4.85068571027985,-95.6189810445332,
-8.40163410171809));
#14304=CARTESIAN_POINT('Ctrl Pts',(-7.27602856540465,-95.4439810445332,
-4.20081705085031));
#14305=CARTESIAN_POINT('Ctrl Pts',(-9.70137142052945,-95.2689810445332,
1.74701365207797E-11));
#14306=CARTESIAN_POINT('Ctrl Pts',(-7.27602856538952,-95.0939810445332,
4.20081705087652));
#14307=CARTESIAN_POINT('Ctrl Pts',(-4.8506857102496,-94.9189810445332,8.40163410173556));
#14308=CARTESIAN_POINT('Ctrl Pts',(1.5129067582862E-11,-94.7439810445332,
8.40163410172683));
#14309=CARTESIAN_POINT('Ctrl Pts',(4.85068571027985,-94.5689810445332,8.40163410171809));
#14310=CARTESIAN_POINT('Ctrl Pts',(7.27602856540465,-94.3939810445332,4.20081705085031));
#14311=CARTESIAN_POINT('Ctrl Pts',(9.70137142052945,-94.2189810445331,-1.7468948445434E-11));
#14312=CARTESIAN_POINT('Ctrl Pts',(7.27602856538952,-94.0439810445332,-4.20081705087651));
#14313=CARTESIAN_POINT('Ctrl Pts',(4.8506857102496,-93.8689810445332,-8.40163410173556));
#14314=CARTESIAN_POINT('Ctrl Pts',(-1.5130096486293E-11,-93.6939810445332,
-8.40163410172683));
#14315=CARTESIAN_POINT('Ctrl Pts',(-4.85068571027985,-93.5189810445332,
-8.40163410171809));
#14316=CARTESIAN_POINT('Ctrl Pts',(-7.27602856540465,-93.3439810445332,
-4.20081705085031));
#14317=CARTESIAN_POINT('Ctrl Pts',(-9.70137142052945,-93.1689810445332,
1.74701365207797E-11));
#14318=CARTESIAN_POINT('Ctrl Pts',(-7.27602856538952,-92.9939810445332,
4.20081705087652));
#14319=CARTESIAN_POINT('Ctrl Pts',(-4.8506857102496,-92.8189810445332,8.40163410173556));
#14320=CARTESIAN_POINT('Ctrl Pts',(1.5129067582862E-11,-92.6439810445332,
8.40163410172683));
#14321=CARTESIAN_POINT('Ctrl Pts',(4.85068571027985,-92.4689810445332,8.40163410171809));
#14322=CARTESIAN_POINT('Ctrl Pts',(7.27602856540465,-92.2939810445332,4.20081705085031));
#14323=CARTESIAN_POINT('Ctrl Pts',(9.70137142052945,-92.1189810445332,-1.7468948445434E-11));
#14324=CARTESIAN_POINT('Ctrl Pts',(7.27602856538952,-91.9439810445332,-4.20081705087651));
#14325=CARTESIAN_POINT('Ctrl Pts',(4.8506857102496,-91.7689810445332,-8.40163410173556));
#14326=CARTESIAN_POINT('Ctrl Pts',(-1.5130096486293E-11,-91.5939810445332,
-8.40163410172683));
#14327=CARTESIAN_POINT('Ctrl Pts',(-4.85068571027985,-91.4189810445332,
-8.40163410171809));
#14328=CARTESIAN_POINT('Ctrl Pts',(-7.27602856540465,-91.2439810445332,
-4.20081705085031));
#14329=CARTESIAN_POINT('Ctrl Pts',(-9.70137142052945,-91.0689810445332,
1.74701365207797E-11));
#14330=CARTESIAN_POINT('Ctrl Pts',(-7.27602856538952,-90.8939810445332,
4.20081705087652));
#14331=CARTESIAN_POINT('Ctrl Pts',(-4.8506857102496,-90.7189810445332,8.40163410173556));
#14332=CARTESIAN_POINT('Ctrl Pts',(1.5129067582862E-11,-90.5439810445332,
8.40163410172683));
#14333=CARTESIAN_POINT('Ctrl Pts',(4.85068571027985,-90.3689810445332,8.40163410171809));
#14334=CARTESIAN_POINT('Ctrl Pts',(7.27602856540465,-90.1939810445332,4.20081705085031));
#14335=CARTESIAN_POINT('Ctrl Pts',(9.70137142052945,-90.0189810445332,-1.7468948445434E-11));
#14336=CARTESIAN_POINT('Ctrl Pts',(7.27602856538952,-89.8439810445332,-4.20081705087651));
#14337=CARTESIAN_POINT('Ctrl Pts',(4.8506857102496,-89.6689810445332,-8.40163410173556));
#14338=CARTESIAN_POINT('Ctrl Pts',(-1.5130096486293E-11,-89.4939810445332,
-8.40163410172683));
#14339=CARTESIAN_POINT('Ctrl Pts',(-4.85068571027985,-89.3189810445332,
-8.40163410171809));
#14340=CARTESIAN_POINT('Ctrl Pts',(-7.27602856540465,-89.1439810445332,
-4.20081705085031));
#14341=CARTESIAN_POINT('Ctrl Pts',(-9.70137142052945,-88.9689810445332,
1.74701365207797E-11));
#14342=CARTESIAN_POINT('Ctrl Pts',(-7.27602856538952,-88.7939810445332,
4.20081705087652));
#14343=CARTESIAN_POINT('Ctrl Pts',(-4.8506857102496,-88.6189810445332,8.40163410173556));
#14344=CARTESIAN_POINT('Ctrl Pts',(1.5129067582862E-11,-88.4439810445332,
8.40163410172683));
#14345=CARTESIAN_POINT('Ctrl Pts',(4.85068571027985,-88.2689810445332,8.40163410171809));
#14346=CARTESIAN_POINT('Ctrl Pts',(7.27602856540465,-88.0939810445332,4.20081705085031));
#14347=CARTESIAN_POINT('Ctrl Pts',(9.70137142052945,-87.9189810445332,-1.7468948445434E-11));
#14348=CARTESIAN_POINT('Ctrl Pts',(7.27602856538952,-87.7439810445332,-4.20081705087651));
#14349=CARTESIAN_POINT('Ctrl Pts',(4.8506857102496,-87.5689810445332,-8.40163410173556));
#14350=CARTESIAN_POINT('Ctrl Pts',(-1.5130096486293E-11,-87.3939810445332,
-8.40163410172683));
#14351=CARTESIAN_POINT('Ctrl Pts',(-4.85068571027985,-87.2189810445332,
-8.40163410171809));
#14352=CARTESIAN_POINT('Ctrl Pts',(-7.27602856540465,-87.0439810445332,
-4.20081705085031));
#14353=CARTESIAN_POINT('Ctrl Pts',(-9.70137142052945,-86.8689810445332,
1.74701365207797E-11));
#14354=CARTESIAN_POINT('Ctrl Pts',(-7.27602856538952,-86.6939810445332,
4.20081705087652));
#14355=CARTESIAN_POINT('Ctrl Pts',(-4.8506857102496,-86.5189810445332,8.40163410173556));
#14356=CARTESIAN_POINT('Ctrl Pts',(1.5129067582862E-11,-86.3439810445332,
8.40163410172683));
#14357=CARTESIAN_POINT('Ctrl Pts',(4.85068571027985,-86.1689810445332,8.40163410171809));
#14358=CARTESIAN_POINT('Ctrl Pts',(7.27602856540465,-85.9939810445332,4.20081705085031));
#14359=CARTESIAN_POINT('Ctrl Pts',(9.70137142052945,-85.8189810445332,-1.7468948445434E-11));
#14360=CARTESIAN_POINT('Ctrl Pts',(7.27602856538952,-85.6439810445332,-4.20081705087651));
#14361=CARTESIAN_POINT('Ctrl Pts',(4.8506857102496,-85.4689810445332,-8.40163410173556));
#14362=CARTESIAN_POINT('Ctrl Pts',(-1.5130096486293E-11,-85.2939810445332,
-8.40163410172683));
#14363=CARTESIAN_POINT('Ctrl Pts',(-4.85068571027985,-85.1189810445332,
-8.40163410171809));
#14364=CARTESIAN_POINT('Ctrl Pts',(-7.27602856540465,-84.9439810445332,
-4.20081705085031));
#14365=CARTESIAN_POINT('Ctrl Pts',(-9.70137142052945,-84.7689810445332,
1.74701365207797E-11));
#14366=CARTESIAN_POINT('Ctrl Pts',(-7.27602856538952,-84.5939810445332,
4.20081705087652));
#14367=CARTESIAN_POINT('Ctrl Pts',(-4.8506857102496,-84.4189810445332,8.40163410173556));
#14368=CARTESIAN_POINT('Ctrl Pts',(1.5129067582862E-11,-84.2439810445332,
8.40163410172683));
#14369=CARTESIAN_POINT('Ctrl Pts',(4.85068571027985,-84.0689810445332,8.40163410171809));
#14370=CARTESIAN_POINT('Ctrl Pts',(7.27602856540465,-83.8939810445332,4.20081705085031));
#14371=CARTESIAN_POINT('Ctrl Pts',(9.70137142052945,-83.7189810445332,-1.7468948445434E-11));
#14372=CARTESIAN_POINT('Ctrl Pts',(7.27602856538952,-83.5439810445332,-4.20081705087651));
#14373=CARTESIAN_POINT('Ctrl Pts',(4.8506857102496,-83.3689810445332,-8.40163410173556));
#14374=CARTESIAN_POINT('Ctrl Pts',(-1.5130096486293E-11,-83.1939810445332,
-8.40163410172683));
#14375=CARTESIAN_POINT('Ctrl Pts',(-4.85068571027985,-83.0189810445332,
-8.40163410171809));
#14376=CARTESIAN_POINT('Ctrl Pts',(-7.27602856540465,-82.8439810445332,
-4.20081705085031));
#14377=CARTESIAN_POINT('Ctrl Pts',(-9.70137142052945,-82.6689810445332,
1.74701365207797E-11));
#14378=CARTESIAN_POINT('Ctrl Pts',(-7.27602856538952,-82.4939810445332,
4.20081705087652));
#14379=CARTESIAN_POINT('Ctrl Pts',(-4.8506857102496,-82.3189810445332,8.40163410173556));
#14380=CARTESIAN_POINT('Ctrl Pts',(1.5129067582862E-11,-82.1439810445332,
8.40163410172683));
#14381=CARTESIAN_POINT('Ctrl Pts',(4.85068571027985,-81.9689810445332,8.40163410171809));
#14382=CARTESIAN_POINT('Ctrl Pts',(7.27602856540465,-81.7939810445332,4.20081705085031));
#14383=CARTESIAN_POINT('Ctrl Pts',(9.70137142052945,-81.6189810445332,-1.7468948445434E-11));
#14384=CARTESIAN_POINT('Ctrl Pts',(7.27602856538952,-81.4439810445332,-4.20081705087651));
#14385=CARTESIAN_POINT('Ctrl Pts',(4.8506857102496,-81.2689810445332,-8.40163410173556));
#14386=CARTESIAN_POINT('Ctrl Pts',(-1.5130096486293E-11,-81.0939810445332,
-8.40163410172683));
#14387=CARTESIAN_POINT('Ctrl Pts',(-4.85068571027985,-80.9189810445332,
-8.40163410171809));
#14388=CARTESIAN_POINT('Ctrl Pts',(-7.27602856540465,-80.7439810445332,
-4.20081705085031));
#14389=CARTESIAN_POINT('Ctrl Pts',(-9.70137142052945,-80.5689810445332,
1.74701365207797E-11));
#14390=CARTESIAN_POINT('Ctrl Pts',(-7.27602856538952,-80.3939810445332,
4.20081705087652));
#14391=CARTESIAN_POINT('Ctrl Pts',(-4.8506857102496,-80.2189810445333,8.40163410173556));
#14392=CARTESIAN_POINT('Ctrl Pts',(1.5129067582862E-11,-80.0439810445332,
8.40163410172683));
#14393=CARTESIAN_POINT('Ctrl Pts',(4.85068571027985,-79.8689810445333,8.40163410171809));
#14394=CARTESIAN_POINT('Ctrl Pts',(7.27602856540465,-79.6939810445332,4.20081705085031));
#14395=CARTESIAN_POINT('Ctrl Pts',(9.70137142052945,-79.5189810445332,-1.7468948445434E-11));
#14396=CARTESIAN_POINT('Ctrl Pts',(7.27602856538952,-79.3439810445332,-4.20081705087651));
#14397=CARTESIAN_POINT('Ctrl Pts',(4.8506857102496,-79.1689810445332,-8.40163410173556));
#14398=CARTESIAN_POINT('Ctrl Pts',(-1.5130096486293E-11,-78.9939810445332,
-8.40163410172683));
#14399=CARTESIAN_POINT('Ctrl Pts',(-4.85068571027985,-78.8189810445332,
-8.40163410171809));
#14400=CARTESIAN_POINT('Ctrl Pts',(-7.27602856540465,-78.6439810445332,
-4.20081705085031));
#14401=CARTESIAN_POINT('Ctrl Pts',(-9.70137142052945,-78.4689810445332,
1.74701365207797E-11));
#14402=CARTESIAN_POINT('Ctrl Pts',(-7.27602856538952,-78.2939810445332,
4.20081705087652));
#14403=CARTESIAN_POINT('Ctrl Pts',(-4.8506857102496,-78.1189810445332,8.40163410173556));
#14404=CARTESIAN_POINT('Ctrl Pts',(1.5129067582862E-11,-77.9439810445332,
8.40163410172683));
#14405=CARTESIAN_POINT('Ctrl Pts',(4.85068571027985,-77.7689810445333,8.40163410171809));
#14406=CARTESIAN_POINT('Ctrl Pts',(7.27602856540465,-77.5939810445332,4.20081705085031));
#14407=CARTESIAN_POINT('Ctrl Pts',(9.70137142052945,-77.4189810445332,-1.7468948445434E-11));
#14408=CARTESIAN_POINT('Ctrl Pts',(7.27602856538952,-77.2439810445332,-4.20081705087651));
#14409=CARTESIAN_POINT('Ctrl Pts',(4.8506857102496,-77.0689810445332,-8.40163410173556));
#14410=CARTESIAN_POINT('Ctrl Pts',(-1.5130096486293E-11,-76.8939810445332,
-8.40163410172683));
#14411=CARTESIAN_POINT('Ctrl Pts',(-4.85068571027985,-76.7189810445333,
-8.40163410171809));
#14412=CARTESIAN_POINT('Ctrl Pts',(-7.27602856540465,-76.5439810445332,
-4.20081705085031));
#14413=CARTESIAN_POINT('Ctrl Pts',(-9.70137142052945,-76.3689810445332,
1.74701365207797E-11));
#14414=CARTESIAN_POINT('Ctrl Pts',(-7.27602856538952,-76.1939810445332,
4.20081705087652));
#14415=CARTESIAN_POINT('Ctrl Pts',(-4.8506857102496,-76.0189810445332,8.40163410173556));
#14416=CARTESIAN_POINT('Ctrl Pts',(1.5129067582862E-11,-75.8439810445332,
8.40163410172683));
#14417=CARTESIAN_POINT('Ctrl Pts',(4.85068571027985,-75.6689810445332,8.40163410171809));
#14418=CARTESIAN_POINT('Ctrl Pts',(7.27602856540465,-75.4939810445332,4.20081705085031));
#14419=CARTESIAN_POINT('Ctrl Pts',(9.70137142052945,-75.3189810445332,-1.7468948445434E-11));
#14420=CARTESIAN_POINT('Ctrl Pts',(7.27602856538952,-75.1439810445332,-4.20081705087651));
#14421=CARTESIAN_POINT('Ctrl Pts',(4.8506857102496,-74.9689810445332,-8.40163410173556));
#14422=CARTESIAN_POINT('Ctrl Pts',(-1.5130096486293E-11,-74.7939810445332,
-8.40163410172683));
#14423=CARTESIAN_POINT('Ctrl Pts',(-4.85068571027985,-74.6189810445332,
-8.40163410171809));
#14424=CARTESIAN_POINT('Ctrl Pts',(-7.27602856540465,-74.4439810445332,
-4.20081705085031));
#14425=CARTESIAN_POINT('Ctrl Pts',(-9.70137142052945,-74.2689810445332,
1.74701365207797E-11));
#14426=CARTESIAN_POINT('Ctrl Pts',(-7.27602856538952,-74.0939810445332,
4.20081705087652));
#14427=CARTESIAN_POINT('Ctrl Pts',(-4.8506857102496,-73.9189810445332,8.40163410173556));
#14428=CARTESIAN_POINT('Ctrl Pts',(1.5129067582862E-11,-73.7439810445332,
8.40163410172683));
#14429=CARTESIAN_POINT('Ctrl Pts',(4.85068571027985,-73.5689810445332,8.40163410171809));
#14430=CARTESIAN_POINT('Ctrl Pts',(7.27602856540465,-73.3939810445332,4.20081705085031));
#14431=CARTESIAN_POINT('Ctrl Pts',(9.70137142052945,-73.2189810445333,-1.7468948445434E-11));
#14432=CARTESIAN_POINT('Ctrl Pts',(7.27602856538952,-73.0439810445332,-4.20081705087651));
#14433=CARTESIAN_POINT('Ctrl Pts',(4.8506857102496,-72.8689810445332,-8.40163410173556));
#14434=CARTESIAN_POINT('Ctrl Pts',(-1.5130096486293E-11,-72.6939810445332,
-8.40163410172683));
#14435=CARTESIAN_POINT('Ctrl Pts',(-4.85068571027985,-72.5189810445332,
-8.40163410171809));
#14436=CARTESIAN_POINT('Ctrl Pts',(-7.27602856540465,-72.3439810445332,
-4.20081705085031));
#14437=CARTESIAN_POINT('Ctrl Pts',(-9.70137142052945,-72.1689810445333,
1.74701365207797E-11));
#14438=CARTESIAN_POINT('Ctrl Pts',(-7.27602856538952,-71.9939810445332,
4.20081705087652));
#14439=CARTESIAN_POINT('Ctrl Pts',(-4.8506857102496,-71.8189810445332,8.40163410173556));
#14440=CARTESIAN_POINT('Ctrl Pts',(1.5129067582862E-11,-71.6439810445332,
8.40163410172683));
#14441=CARTESIAN_POINT('Ctrl Pts',(4.85068571027985,-71.4689810445332,8.40163410171809));
#14442=CARTESIAN_POINT('Ctrl Pts',(7.27602856540465,-71.2939810445332,4.20081705085031));
#14443=CARTESIAN_POINT('Ctrl Pts',(9.70137142052945,-71.1189810445332,-1.7468948445434E-11));
#14444=CARTESIAN_POINT('Ctrl Pts',(7.27602856538952,-70.9439810445332,-4.20081705087651));
#14445=CARTESIAN_POINT('Ctrl Pts',(4.8506857102496,-70.7689810445332,-8.40163410173556));
#14446=CARTESIAN_POINT('Ctrl Pts',(-1.5130096486293E-11,-70.5939810445332,
-8.40163410172683));
#14447=CARTESIAN_POINT('Ctrl Pts',(-4.85068571027985,-70.4189810445332,
-8.40163410171809));
#14448=CARTESIAN_POINT('Ctrl Pts',(-7.27602856540465,-70.2439810445332,
-4.20081705085031));
#14449=CARTESIAN_POINT('Ctrl Pts',(-9.70137142052945,-70.0689810445332,
1.74701365207797E-11));
#14450=CARTESIAN_POINT('Ctrl Pts',(-7.27602856538952,-69.8939810445332,
4.20081705087652));
#14451=CARTESIAN_POINT('Ctrl Pts',(-4.8506857102496,-69.7189810445333,8.40163410173556));
#14452=CARTESIAN_POINT('Ctrl Pts',(1.5129067582862E-11,-69.5439810445333,
8.40163410172683));
#14453=CARTESIAN_POINT('Ctrl Pts',(4.85068571027985,-69.3689810445332,8.40163410171809));
#14454=CARTESIAN_POINT('Ctrl Pts',(7.27602856540465,-69.1939810445332,4.20081705085031));
#14455=CARTESIAN_POINT('Ctrl Pts',(9.70137142052945,-69.0189810445333,-1.7468948445434E-11));
#14456=CARTESIAN_POINT('Ctrl Pts',(7.27602856538952,-68.8439810445332,-4.20081705087651));
#14457=CARTESIAN_POINT('Ctrl Pts',(4.8506857102496,-68.6689810445332,-8.40163410173556));
#14458=CARTESIAN_POINT('Ctrl Pts',(-1.5130096486293E-11,-68.4939810445333,
-8.40163410172683));
#14459=CARTESIAN_POINT('Ctrl Pts',(-4.85068571027985,-68.3189810445332,
-8.40163410171809));
#14460=CARTESIAN_POINT('Ctrl Pts',(-7.27602856540465,-68.1439810445332,
-4.20081705085031));
#14461=CARTESIAN_POINT('Ctrl Pts',(-9.70137142052945,-67.9689810445333,
1.74701365207797E-11));
#14462=CARTESIAN_POINT('Ctrl Pts',(-7.27602856538952,-67.7939810445332,
4.20081705087652));
#14463=CARTESIAN_POINT('Ctrl Pts',(-4.8506857102496,-67.6189810445333,8.40163410173556));
#14464=CARTESIAN_POINT('Ctrl Pts',(1.5129067582862E-11,-67.4439810445333,
8.40163410172683));
#14465=CARTESIAN_POINT('Ctrl Pts',(4.85068571027985,-67.2689810445332,8.40163410171809));
#14466=CARTESIAN_POINT('Ctrl Pts',(7.27602856540465,-67.0939810445333,4.20081705085031));
#14467=CARTESIAN_POINT('Ctrl Pts',(9.70137142052945,-66.9189810445333,-1.7468948445434E-11));
#14468=CARTESIAN_POINT('Ctrl Pts',(7.27602856538952,-66.7439810445332,-4.20081705087651));
#14469=CARTESIAN_POINT('Ctrl Pts',(4.8506857102496,-66.5689810445333,-8.40163410173556));
#14470=CARTESIAN_POINT('Ctrl Pts',(-1.5130096486293E-11,-66.3939810445332,
-8.40163410172683));
#14471=CARTESIAN_POINT('Ctrl Pts',(-4.85068571027985,-66.2189810445332,
-8.40163410171809));
#14472=CARTESIAN_POINT('Ctrl Pts',(-7.27602856540465,-66.0439810445333,
-4.20081705085031));
#14473=CARTESIAN_POINT('Ctrl Pts',(-9.70137142052945,-65.8689810445332,
1.74701365207797E-11));
#14474=CARTESIAN_POINT('Ctrl Pts',(-7.27602856538952,-65.6939810445332,
4.20081705087652));
#14475=CARTESIAN_POINT('Ctrl Pts',(-4.8506857102496,-65.5189810445333,8.40163410173556));
#14476=CARTESIAN_POINT('Ctrl Pts',(1.5129067582862E-11,-65.3439810445333,
8.40163410172683));
#14477=CARTESIAN_POINT('Ctrl Pts',(4.85068571027985,-65.1689810445333,8.40163410171809));
#14478=CARTESIAN_POINT('Ctrl Pts',(7.27602856540465,-64.9939810445333,4.20081705085031));
#14479=CARTESIAN_POINT('Ctrl Pts',(9.70137142052945,-64.8189810445332,-1.7468948445434E-11));
#14480=CARTESIAN_POINT('Ctrl Pts',(7.27602856538952,-64.6439810445332,-4.20081705087651));
#14481=CARTESIAN_POINT('Ctrl Pts',(4.8506857102496,-64.4689810445333,-8.40163410173556));
#14482=CARTESIAN_POINT('Ctrl Pts',(-1.5130096486293E-11,-64.2939810445333,
-8.40163410172683));
#14483=CARTESIAN_POINT('Ctrl Pts',(-4.85068571027985,-64.1189810445333,
-8.40163410171809));
#14484=CARTESIAN_POINT('Ctrl Pts',(-7.27602856540465,-63.9439810445333,
-4.20081705085031));
#14485=CARTESIAN_POINT('Ctrl Pts',(-9.70137142052945,-63.7689810445333,
1.74701365207797E-11));
#14486=CARTESIAN_POINT('Ctrl Pts',(-7.27602856538952,-63.5939810445333,
4.20081705087652));
#14487=CARTESIAN_POINT('Ctrl Pts',(-4.8506857102496,-63.4189810445333,8.40163410173556));
#14488=CARTESIAN_POINT('Ctrl Pts',(1.5129067582862E-11,-63.2439810445333,
8.40163410172683));
#14489=CARTESIAN_POINT('Ctrl Pts',(4.85068571027985,-63.0689810445333,8.40163410171809));
#14490=CARTESIAN_POINT('Ctrl Pts',(7.27602856540465,-62.8939810445333,4.20081705085031));
#14491=CARTESIAN_POINT('Ctrl Pts',(9.70137142052945,-62.7189810445333,-1.7468948445434E-11));
#14492=CARTESIAN_POINT('Ctrl Pts',(7.27602856538952,-62.5439810445333,-4.20081705087651));
#14493=CARTESIAN_POINT('Ctrl Pts',(4.8506857102496,-62.3689810445333,-8.40163410173556));
#14494=CARTESIAN_POINT('Ctrl Pts',(-1.5130096486293E-11,-62.1939810445333,
-8.40163410172683));
#14495=CARTESIAN_POINT('Ctrl Pts',(-4.85068571027985,-62.0189810445333,
-8.40163410171809));
#14496=CARTESIAN_POINT('Ctrl Pts',(-7.27602856540465,-61.8439810445333,
-4.20081705085031));
#14497=CARTESIAN_POINT('Ctrl Pts',(-9.70137142052945,-61.6689810445332,
1.74701365207797E-11));
#14498=CARTESIAN_POINT('Ctrl Pts',(-7.27602856538952,-61.4939810445333,
4.20081705087652));
#14499=CARTESIAN_POINT('Ctrl Pts',(-4.8506857102496,-61.3189810445333,8.40163410173556));
#14500=CARTESIAN_POINT('Ctrl Pts',(1.5129067582862E-11,-61.1439810445333,
8.40163410172683));
#14501=CARTESIAN_POINT('Ctrl Pts',(4.85068571027985,-60.9689810445333,8.40163410171809));
#14502=CARTESIAN_POINT('Ctrl Pts',(7.27602856540465,-60.7939810445333,4.20081705085031));
#14503=CARTESIAN_POINT('Ctrl Pts',(9.70137142052945,-60.6189810445333,-1.7468948445434E-11));
#14504=CARTESIAN_POINT('Ctrl Pts',(7.27602856538952,-60.4439810445333,-4.20081705087651));
#14505=CARTESIAN_POINT('Ctrl Pts',(4.8506857102496,-60.2689810445333,-8.40163410173556));
#14506=CARTESIAN_POINT('Ctrl Pts',(-1.5130096486293E-11,-60.0939810445333,
-8.40163410172683));
#14507=CARTESIAN_POINT('Ctrl Pts',(-4.85068571027985,-59.9189810445333,
-8.40163410171809));
#14508=CARTESIAN_POINT('Ctrl Pts',(-7.27602856540465,-59.7439810445333,
-4.20081705085031));
#14509=CARTESIAN_POINT('Ctrl Pts',(-9.70137142052945,-59.5689810445332,
1.74701365207797E-11));
#14510=CARTESIAN_POINT('Ctrl Pts',(-7.27602856538952,-59.3939810445333,
4.20081705087652));
#14511=CARTESIAN_POINT('Ctrl Pts',(-4.8506857102496,-59.2189810445333,8.40163410173556));
#14512=CARTESIAN_POINT('Ctrl Pts',(1.5129067582862E-11,-59.0439810445332,
8.40163410172683));
#14513=CARTESIAN_POINT('Ctrl Pts',(4.85068571027985,-58.8689810445333,8.40163410171809));
#14514=CARTESIAN_POINT('Ctrl Pts',(7.27602856540465,-58.6939810445333,4.20081705085031));
#14515=CARTESIAN_POINT('Ctrl Pts',(9.70137142052945,-58.5189810445332,-1.7468948445434E-11));
#14516=CARTESIAN_POINT('Ctrl Pts',(7.27602856538952,-58.3439810445333,-4.20081705087651));
#14517=CARTESIAN_POINT('Ctrl Pts',(4.8506857102496,-58.1689810445333,-8.40163410173556));
#14518=CARTESIAN_POINT('Ctrl Pts',(-1.5130096486293E-11,-57.9939810445333,
-8.40163410172683));
#14519=CARTESIAN_POINT('Ctrl Pts',(-4.85068571027985,-57.8189810445333,
-8.40163410171809));
#14520=CARTESIAN_POINT('Ctrl Pts',(-7.27602856540465,-57.6439810445333,
-4.20081705085031));
#14521=CARTESIAN_POINT('Ctrl Pts',(-9.70137142052945,-57.4689810445332,
1.74701365207797E-11));
#14522=CARTESIAN_POINT('Ctrl Pts',(-7.27602856538952,-57.2939810445333,
4.20081705087652));
#14523=CARTESIAN_POINT('Ctrl Pts',(-4.8506857102496,-57.1189810445333,8.40163410173556));
#14524=CARTESIAN_POINT('Ctrl Pts',(1.5129067582862E-11,-56.9439810445333,
8.40163410172683));
#14525=CARTESIAN_POINT('Ctrl Pts',(4.85068571027985,-56.7689810445333,8.40163410171809));
#14526=CARTESIAN_POINT('Ctrl Pts',(7.27602856540465,-56.5939810445333,4.20081705085031));
#14527=CARTESIAN_POINT('Ctrl Pts',(9.70137142052945,-56.4189810445332,-1.7468948445434E-11));
#14528=CARTESIAN_POINT('Ctrl Pts',(7.27602856538952,-56.2439810445333,-4.20081705087651));
#14529=CARTESIAN_POINT('Ctrl Pts',(4.8506857102496,-56.0689810445333,-8.40163410173556));
#14530=CARTESIAN_POINT('Ctrl Pts',(-1.5130096486293E-11,-55.8939810445333,
-8.40163410172683));
#14531=CARTESIAN_POINT('Ctrl Pts',(-4.85068571027985,-55.7189810445333,
-8.40163410171809));
#14532=CARTESIAN_POINT('Ctrl Pts',(-7.27602856540465,-55.5439810445333,
-4.20081705085031));
#14533=CARTESIAN_POINT('Ctrl Pts',(-9.70137142052945,-55.3689810445333,
1.74701365207797E-11));
#14534=CARTESIAN_POINT('Ctrl Pts',(-7.27602856538952,-55.1939810445333,
4.20081705087652));
#14535=CARTESIAN_POINT('Ctrl Pts',(-4.8506857102496,-55.0189810445333,8.40163410173556));
#14536=CARTESIAN_POINT('Ctrl Pts',(1.5129067582862E-11,-54.8439810445333,
8.40163410172683));
#14537=CARTESIAN_POINT('Ctrl Pts',(4.85068571027985,-54.6689810445333,8.40163410171809));
#14538=CARTESIAN_POINT('Ctrl Pts',(7.27602856540465,-54.4939810445333,4.20081705085031));
#14539=CARTESIAN_POINT('Ctrl Pts',(9.70137142052945,-54.3189810445333,-1.7468948445434E-11));
#14540=CARTESIAN_POINT('Ctrl Pts',(7.27602856538952,-54.1439810445333,-4.20081705087651));
#14541=CARTESIAN_POINT('Ctrl Pts',(4.8506857102496,-53.9689810445333,-8.40163410173556));
#14542=CARTESIAN_POINT('Ctrl Pts',(-1.5130096486293E-11,-53.7939810445333,
-8.40163410172683));
#14543=CARTESIAN_POINT('Ctrl Pts',(-4.85068571027985,-53.6189810445333,
-8.40163410171809));
#14544=CARTESIAN_POINT('Ctrl Pts',(-7.27602856540465,-53.4439810445333,
-4.20081705085031));
#14545=CARTESIAN_POINT('Ctrl Pts',(-9.70137142052945,-53.2689810445333,
1.74701365207797E-11));
#14546=CARTESIAN_POINT('Ctrl Pts',(-7.27602856538952,-53.0939810445333,
4.20081705087652));
#14547=CARTESIAN_POINT('Ctrl Pts',(-4.8506857102496,-52.9189810445333,8.40163410173556));
#14548=CARTESIAN_POINT('Ctrl Pts',(1.5129067582862E-11,-52.7439810445333,
8.40163410172683));
#14549=CARTESIAN_POINT('Ctrl Pts',(4.85068571027985,-52.5689810445333,8.40163410171809));
#14550=CARTESIAN_POINT('Ctrl Pts',(7.27602856540465,-52.3939810445333,4.20081705085031));
#14551=CARTESIAN_POINT('Ctrl Pts',(9.70137142052945,-52.2189810445333,-1.7468948445434E-11));
#14552=CARTESIAN_POINT('Ctrl Pts',(7.27602856538952,-52.0439810445333,-4.20081705087651));
#14553=CARTESIAN_POINT('Ctrl Pts',(4.8506857102496,-51.8689810445333,-8.40163410173556));
#14554=CARTESIAN_POINT('Ctrl Pts',(-1.5130096486293E-11,-51.6939810445333,
-8.40163410172683));
#14555=CARTESIAN_POINT('Ctrl Pts',(-4.85068571027985,-51.5189810445333,
-8.40163410171809));
#14556=CARTESIAN_POINT('Ctrl Pts',(-7.27602856540465,-51.3439810445333,
-4.20081705085031));
#14557=CARTESIAN_POINT('Ctrl Pts',(-9.70137142052945,-51.1689810445333,
1.74701365207797E-11));
#14558=CARTESIAN_POINT('Ctrl Pts',(-7.27602856538952,-50.9939810445333,
4.20081705087652));
#14559=CARTESIAN_POINT('Ctrl Pts',(-4.8506857102496,-50.8189810445333,8.40163410173556));
#14560=CARTESIAN_POINT('Ctrl Pts',(1.5129067582862E-11,-50.6439810445333,
8.40163410172683));
#14561=CARTESIAN_POINT('Ctrl Pts',(4.85068571027985,-50.4689810445333,8.40163410171809));
#14562=CARTESIAN_POINT('Ctrl Pts',(7.27602856540465,-50.2939810445333,4.20081705085031));
#14563=CARTESIAN_POINT('Ctrl Pts',(9.70137142052945,-50.1189810445333,-1.7468948445434E-11));
#14564=CARTESIAN_POINT('Ctrl Pts',(7.27602856538952,-49.9439810445333,-4.20081705087651));
#14565=CARTESIAN_POINT('Ctrl Pts',(4.8506857102496,-49.7689810445333,-8.40163410173556));
#14566=CARTESIAN_POINT('Ctrl Pts',(-1.5130096486293E-11,-49.5939810445333,
-8.40163410172683));
#14567=CARTESIAN_POINT('Ctrl Pts',(-4.85068571027985,-49.4189810445333,
-8.40163410171809));
#14568=CARTESIAN_POINT('Ctrl Pts',(-7.27602856540465,-49.2439810445333,
-4.20081705085031));
#14569=CARTESIAN_POINT('Ctrl Pts',(-9.70137142052945,-49.0689810445333,
1.74701365207797E-11));
#14570=CARTESIAN_POINT('Ctrl Pts',(-7.27602856538952,-48.8939810445333,
4.20081705087652));
#14571=CARTESIAN_POINT('Ctrl Pts',(-4.8506857102496,-48.7189810445333,8.40163410173556));
#14572=CARTESIAN_POINT('Ctrl Pts',(1.5129067582862E-11,-48.5439810445333,
8.40163410172683));
#14573=CARTESIAN_POINT('Ctrl Pts',(4.85068571027985,-48.3689810445333,8.40163410171809));
#14574=CARTESIAN_POINT('Ctrl Pts',(7.27602856540465,-48.1939810445333,4.20081705085031));
#14575=CARTESIAN_POINT('Ctrl Pts',(9.70137142052945,-48.0189810445333,-1.7468948445434E-11));
#14576=CARTESIAN_POINT('Ctrl Pts',(7.27602856538952,-47.8439810445333,-4.20081705087651));
#14577=CARTESIAN_POINT('Ctrl Pts',(4.8506857102496,-47.6689810445333,-8.40163410173556));
#14578=CARTESIAN_POINT('Ctrl Pts',(-1.5130096486293E-11,-47.4939810445333,
-8.40163410172683));
#14579=CARTESIAN_POINT('Ctrl Pts',(-4.85068571027985,-47.3189810445333,
-8.40163410171809));
#14580=CARTESIAN_POINT('Ctrl Pts',(-7.27602856540465,-47.1439810445333,
-4.20081705085031));
#14581=CARTESIAN_POINT('Ctrl Pts',(-9.70137142052945,-46.9689810445333,
1.74701365207797E-11));
#14582=CARTESIAN_POINT('Ctrl Pts',(-7.27602856538952,-46.7939810445333,
4.20081705087652));
#14583=CARTESIAN_POINT('Ctrl Pts',(-4.8506857102496,-46.6189810445333,8.40163410173556));
#14584=CARTESIAN_POINT('Ctrl Pts',(1.5129067582862E-11,-46.4439810445333,
8.40163410172683));
#14585=CARTESIAN_POINT('Ctrl Pts',(4.85068571027985,-46.2689810445333,8.40163410171809));
#14586=CARTESIAN_POINT('Ctrl Pts',(7.27602856540465,-46.0939810445333,4.20081705085031));
#14587=CARTESIAN_POINT('Ctrl Pts',(9.70137142052945,-45.9189810445333,-1.7468948445434E-11));
#14588=CARTESIAN_POINT('Ctrl Pts',(7.27602856538952,-45.7439810445333,-4.20081705087651));
#14589=CARTESIAN_POINT('Ctrl Pts',(4.8506857102496,-45.5689810445333,-8.40163410173556));
#14590=CARTESIAN_POINT('Ctrl Pts',(-1.5130096486293E-11,-45.3939810445333,
-8.40163410172683));
#14591=CARTESIAN_POINT('Ctrl Pts',(-4.85068571027985,-45.2189810445333,
-8.40163410171809));
#14592=CARTESIAN_POINT('Ctrl Pts',(-7.27602856540465,-45.0439810445333,
-4.20081705085031));
#14593=CARTESIAN_POINT('Ctrl Pts',(-9.70137142052945,-44.8689810445333,
1.74701365207797E-11));
#14594=CARTESIAN_POINT('Ctrl Pts',(-7.27602856538952,-44.6939810445333,
4.20081705087652));
#14595=CARTESIAN_POINT('Ctrl Pts',(-4.8506857102496,-44.5189810445333,8.40163410173556));
#14596=CARTESIAN_POINT('Ctrl Pts',(1.5129067582862E-11,-44.3439810445333,
8.40163410172683));
#14597=CARTESIAN_POINT('Ctrl Pts',(4.85068571027985,-44.1689810445333,8.40163410171809));
#14598=CARTESIAN_POINT('Ctrl Pts',(7.27602856540465,-43.9939810445333,4.20081705085031));
#14599=CARTESIAN_POINT('Ctrl Pts',(9.70137142052945,-43.8189810445333,-1.7468948445434E-11));
#14600=CARTESIAN_POINT('Ctrl Pts',(7.27602856538952,-43.6439810445333,-4.20081705087651));
#14601=CARTESIAN_POINT('Ctrl Pts',(4.8506857102496,-43.4689810445333,-8.40163410173556));
#14602=CARTESIAN_POINT('Ctrl Pts',(-1.5130096486293E-11,-43.2939810445333,
-8.40163410172683));
#14603=CARTESIAN_POINT('Ctrl Pts',(-4.85068571027985,-43.1189810445333,
-8.40163410171809));
#14604=CARTESIAN_POINT('Ctrl Pts',(-7.27602856540465,-42.9439810445333,
-4.20081705085031));
#14605=CARTESIAN_POINT('Ctrl Pts',(-9.70137142052945,-42.7689810445333,
1.74701365207797E-11));
#14606=CARTESIAN_POINT('Ctrl Pts',(-7.27602856538952,-42.5939810445333,
4.20081705087652));
#14607=CARTESIAN_POINT('Ctrl Pts',(-4.8506857102496,-42.4189810445333,8.40163410173556));
#14608=CARTESIAN_POINT('Ctrl Pts',(1.5129067582862E-11,-42.2439810445333,
8.40163410172683));
#14609=CARTESIAN_POINT('Ctrl Pts',(4.85068571027985,-42.0689810445333,8.40163410171809));
#14610=CARTESIAN_POINT('Ctrl Pts',(7.27602856540465,-41.8939810445333,4.20081705085031));
#14611=CARTESIAN_POINT('Ctrl Pts',(9.70137142052945,-41.7189810445333,-1.7468948445434E-11));
#14612=CARTESIAN_POINT('Ctrl Pts',(7.27602856538952,-41.5439810445333,-4.20081705087651));
#14613=CARTESIAN_POINT('Ctrl Pts',(4.8506857102496,-41.3689810445333,-8.40163410173556));
#14614=CARTESIAN_POINT('Ctrl Pts',(-1.5130096486293E-11,-41.1939810445333,
-8.40163410172683));
#14615=CARTESIAN_POINT('Ctrl Pts',(-4.85068571027985,-41.0189810445333,
-8.40163410171809));
#14616=CARTESIAN_POINT('Ctrl Pts',(-7.27602856540465,-40.8439810445333,
-4.20081705085031));
#14617=CARTESIAN_POINT('Ctrl Pts',(-9.70137142052945,-40.6689810445333,
1.74701365207797E-11));
#14618=CARTESIAN_POINT('Ctrl Pts',(-7.27602856538952,-40.4939810445333,
4.20081705087652));
#14619=CARTESIAN_POINT('Ctrl Pts',(-4.8506857102496,-40.3189810445333,8.40163410173556));
#14620=CARTESIAN_POINT('Ctrl Pts',(1.5129067582862E-11,-40.1439810445333,
8.40163410172683));
#14621=CARTESIAN_POINT('Ctrl Pts',(4.85068571027985,-39.9689810445333,8.40163410171809));
#14622=CARTESIAN_POINT('Ctrl Pts',(7.27602856540465,-39.7939810445333,4.20081705085031));
#14623=CARTESIAN_POINT('Ctrl Pts',(9.70137142052945,-39.6189810445333,-1.7468948445434E-11));
#14624=CARTESIAN_POINT('Ctrl Pts',(7.27602856538952,-39.4439810445333,-4.20081705087651));
#14625=CARTESIAN_POINT('Ctrl Pts',(4.8506857102496,-39.2689810445333,-8.40163410173556));
#14626=CARTESIAN_POINT('Ctrl Pts',(-1.5130096486293E-11,-39.0939810445333,
-8.40163410172683));
#14627=CARTESIAN_POINT('Ctrl Pts',(-4.85068571027985,-38.9189810445333,
-8.40163410171809));
#14628=CARTESIAN_POINT('Ctrl Pts',(-7.27602856540465,-38.7439810445333,
-4.20081705085031));
#14629=CARTESIAN_POINT('Ctrl Pts',(-9.70137142052945,-38.5689810445333,
1.74701365207797E-11));
#14630=CARTESIAN_POINT('Ctrl Pts',(-7.27602856538952,-38.3939810445333,
4.20081705087652));
#14631=CARTESIAN_POINT('Ctrl Pts',(-4.8506857102496,-38.2189810445333,8.40163410173556));
#14632=CARTESIAN_POINT('Ctrl Pts',(1.5129067582862E-11,-38.0439810445333,
8.40163410172683));
#14633=CARTESIAN_POINT('Ctrl Pts',(4.85068571027985,-37.8689810445333,8.40163410171809));
#14634=CARTESIAN_POINT('Ctrl Pts',(7.27602856540465,-37.6939810445333,4.20081705085031));
#14635=CARTESIAN_POINT('Ctrl Pts',(9.70137142052945,-37.5189810445333,-1.7468948445434E-11));
#14636=CARTESIAN_POINT('Ctrl Pts',(7.27602856538952,-37.3439810445333,-4.20081705087651));
#14637=CARTESIAN_POINT('Ctrl Pts',(4.8506857102496,-37.1689810445333,-8.40163410173556));
#14638=CARTESIAN_POINT('Ctrl Pts',(-1.5130096486293E-11,-36.9939810445333,
-8.40163410172683));
#14639=CARTESIAN_POINT('Ctrl Pts',(-4.85068571027985,-36.8189810445333,
-8.40163410171809));
#14640=CARTESIAN_POINT('Ctrl Pts',(-7.27602856540465,-36.6439810445333,
-4.20081705085031));
#14641=CARTESIAN_POINT('Ctrl Pts',(-9.70137142052945,-36.4689810445333,
1.74701365207797E-11));
#14642=CARTESIAN_POINT('Ctrl Pts',(-7.27602856538952,-36.2939810445333,
4.20081705087652));
#14643=CARTESIAN_POINT('Ctrl Pts',(-4.8506857102496,-36.1189810445333,8.40163410173556));
#14644=CARTESIAN_POINT('Ctrl Pts',(1.5129067582862E-11,-35.9439810445333,
8.40163410172683));
#14645=CARTESIAN_POINT('Ctrl Pts',(4.85068571027985,-35.7689810445333,8.40163410171809));
#14646=CARTESIAN_POINT('Ctrl Pts',(7.27602856540465,-35.5939810445333,4.20081705085031));
#14647=CARTESIAN_POINT('Ctrl Pts',(9.70137142052945,-35.4189810445333,-1.7468948445434E-11));
#14648=CARTESIAN_POINT('Ctrl Pts',(7.27602856538952,-35.2439810445333,-4.20081705087651));
#14649=CARTESIAN_POINT('Ctrl Pts',(4.8506857102496,-35.0689810445333,-8.40163410173556));
#14650=CARTESIAN_POINT('Ctrl Pts',(-1.5130096486293E-11,-34.8939810445333,
-8.40163410172683));
#14651=CARTESIAN_POINT('Ctrl Pts',(-4.85068571027985,-34.7189810445333,
-8.40163410171809));
#14652=CARTESIAN_POINT('Ctrl Pts',(-7.27602856540465,-34.5439810445333,
-4.20081705085031));
#14653=CARTESIAN_POINT('Ctrl Pts',(-9.70137142052945,-34.3689810445333,
1.74701365207797E-11));
#14654=CARTESIAN_POINT('Ctrl Pts',(-7.27602856538952,-34.1939810445333,
4.20081705087652));
#14655=CARTESIAN_POINT('Ctrl Pts',(-4.8506857102496,-34.0189810445333,8.40163410173556));
#14656=CARTESIAN_POINT('Ctrl Pts',(1.5129067582862E-11,-33.8439810445333,
8.40163410172683));
#14657=CARTESIAN_POINT('Ctrl Pts',(4.85068571027985,-33.6689810445333,8.40163410171809));
#14658=CARTESIAN_POINT('Ctrl Pts',(7.27602856540465,-33.4939810445333,4.20081705085031));
#14659=CARTESIAN_POINT('Ctrl Pts',(9.70137142052945,-33.3189810445333,-1.7468948445434E-11));
#14660=CARTESIAN_POINT('Ctrl Pts',(7.27602856538952,-33.1439810445333,-4.20081705087651));
#14661=CARTESIAN_POINT('Ctrl Pts',(4.8506857102496,-32.9689810445333,-8.40163410173556));
#14662=CARTESIAN_POINT('Ctrl Pts',(-1.5130096486293E-11,-32.7939810445333,
-8.40163410172683));
#14663=CARTESIAN_POINT('Ctrl Pts',(-4.85068571027985,-32.6189810445333,
-8.40163410171809));
#14664=CARTESIAN_POINT('Ctrl Pts',(-7.27602856540465,-32.4439810445333,
-4.20081705085031));
#14665=CARTESIAN_POINT('Ctrl Pts',(-9.70137142052945,-32.2689810445333,
1.74701365207797E-11));
#14666=CARTESIAN_POINT('Ctrl Pts',(-7.27602856538952,-32.0939810445333,
4.20081705087652));
#14667=CARTESIAN_POINT('Ctrl Pts',(-4.8506857102496,-31.9189810445333,8.40163410173556));
#14668=CARTESIAN_POINT('Ctrl Pts',(1.5129067582862E-11,-31.7439810445333,
8.40163410172683));
#14669=CARTESIAN_POINT('Ctrl Pts',(4.85068571027985,-31.5689810445333,8.40163410171809));
#14670=CARTESIAN_POINT('Ctrl Pts',(7.27602856540465,-31.3939810445333,4.20081705085031));
#14671=CARTESIAN_POINT('Ctrl Pts',(9.70137142052945,-31.2189810445333,-1.7468948445434E-11));
#14672=CARTESIAN_POINT('Ctrl Pts',(7.27602856538952,-31.0439810445333,-4.20081705087651));
#14673=CARTESIAN_POINT('Ctrl Pts',(4.8506857102496,-30.8689810445333,-8.40163410173556));
#14674=CARTESIAN_POINT('Ctrl Pts',(-1.5130096486293E-11,-30.6939810445333,
-8.40163410172683));
#14675=CARTESIAN_POINT('Ctrl Pts',(-4.85068571027985,-30.5189810445333,
-8.40163410171809));
#14676=CARTESIAN_POINT('Ctrl Pts',(-7.27602856540465,-30.3439810445333,
-4.20081705085031));
#14677=CARTESIAN_POINT('Ctrl Pts',(-9.70137142052945,-30.1689810445333,
1.74701365207797E-11));
#14678=CARTESIAN_POINT('Ctrl Pts',(-7.27602856538952,-29.9939810445333,
4.20081705087652));
#14679=CARTESIAN_POINT('Ctrl Pts',(-4.8506857102496,-29.8189810445333,8.40163410173556));
#14680=CARTESIAN_POINT('Ctrl Pts',(1.5129067582862E-11,-29.6439810445333,
8.40163410172683));
#14681=CARTESIAN_POINT('Ctrl Pts',(4.85068571027985,-29.4689810445333,8.40163410171809));
#14682=CARTESIAN_POINT('Ctrl Pts',(7.27602856540465,-29.2939810445333,4.20081705085031));
#14683=CARTESIAN_POINT('Ctrl Pts',(9.70137142052945,-29.1189810445333,-1.7468948445434E-11));
#14684=CARTESIAN_POINT('Ctrl Pts',(7.27602856538952,-28.9439810445333,-4.20081705087651));
#14685=CARTESIAN_POINT('Ctrl Pts',(4.8506857102496,-28.7689810445333,-8.40163410173556));
#14686=CARTESIAN_POINT('Ctrl Pts',(-1.5130096486293E-11,-28.5939810445333,
-8.40163410172683));
#14687=CARTESIAN_POINT('Ctrl Pts',(-4.85068571027985,-28.4189810445333,
-8.40163410171809));
#14688=CARTESIAN_POINT('Ctrl Pts',(-7.27602856540465,-28.2439810445333,
-4.20081705085031));
#14689=CARTESIAN_POINT('Ctrl Pts',(-9.70137142052945,-28.0689810445333,
1.74701365207797E-11));
#14690=CARTESIAN_POINT('Ctrl Pts',(-7.27602856538952,-27.8939810445333,
4.20081705087652));
#14691=CARTESIAN_POINT('Ctrl Pts',(-4.8506857102496,-27.7189810445334,8.40163410173556));
#14692=CARTESIAN_POINT('Ctrl Pts',(1.5129067582862E-11,-27.5439810445333,
8.40163410172683));
#14693=CARTESIAN_POINT('Ctrl Pts',(4.85068571027985,-27.3689810445333,8.40163410171809));
#14694=CARTESIAN_POINT('Ctrl Pts',(7.27602856540465,-27.1939810445333,4.20081705085031));
#14695=CARTESIAN_POINT('Ctrl Pts',(9.70137142052945,-27.0189810445333,-1.7468948445434E-11));
#14696=CARTESIAN_POINT('Ctrl Pts',(7.27602856538952,-26.8439810445333,-4.20081705087651));
#14697=CARTESIAN_POINT('Ctrl Pts',(4.8506857102496,-26.6689810445333,-8.40163410173556));
#14698=CARTESIAN_POINT('Ctrl Pts',(-1.5130096486293E-11,-26.4939810445333,
-8.40163410172683));
#14699=CARTESIAN_POINT('Ctrl Pts',(-4.85068571027985,-26.3189810445333,
-8.40163410171809));
#14700=CARTESIAN_POINT('Ctrl Pts',(-7.27602856540465,-26.1439810445333,
-4.20081705085031));
#14701=CARTESIAN_POINT('Ctrl Pts',(-9.70137142052945,-25.9689810445333,
1.74701365207797E-11));
#14702=CARTESIAN_POINT('Ctrl Pts',(-7.27602856538952,-25.7939810445333,
4.20081705087652));
#14703=CARTESIAN_POINT('Ctrl Pts',(-4.8506857102496,-25.6189810445334,8.40163410173556));
#14704=CARTESIAN_POINT('Ctrl Pts',(1.5129067582862E-11,-25.4439810445333,
8.40163410172683));
#14705=CARTESIAN_POINT('Ctrl Pts',(4.85068571027985,-25.2689810445333,8.40163410171809));
#14706=CARTESIAN_POINT('Ctrl Pts',(7.27602856540465,-25.0939810445334,4.20081705085031));
#14707=CARTESIAN_POINT('Ctrl Pts',(9.70137142052945,-24.9189810445333,-1.7468948445434E-11));
#14708=CARTESIAN_POINT('Ctrl Pts',(7.27602856538952,-24.7439810445333,-4.20081705087651));
#14709=CARTESIAN_POINT('Ctrl Pts',(4.8506857102496,-24.5689810445334,-8.40163410173556));
#14710=CARTESIAN_POINT('Ctrl Pts',(-1.5130096486293E-11,-24.3939810445333,
-8.40163410172683));
#14711=CARTESIAN_POINT('Ctrl Pts',(-4.85068571027985,-24.2189810445334,
-8.40163410171809));
#14712=CARTESIAN_POINT('Ctrl Pts',(-7.27602856540465,-24.0439810445333,
-4.20081705085031));
#14713=CARTESIAN_POINT('Ctrl Pts',(-9.70137142052945,-23.8689810445333,
1.74701365207797E-11));
#14714=CARTESIAN_POINT('Ctrl Pts',(-7.27602856538952,-23.6939810445334,
4.20081705087652));
#14715=CARTESIAN_POINT('Ctrl Pts',(-4.8506857102496,-23.5189810445334,8.40163410173556));
#14716=CARTESIAN_POINT('Ctrl Pts',(1.5129067582862E-11,-23.3439810445333,
8.40163410172683));
#14717=CARTESIAN_POINT('Ctrl Pts',(4.85068571027985,-23.1689810445334,8.40163410171809));
#14718=CARTESIAN_POINT('Ctrl Pts',(7.27602856540465,-22.9939810445333,4.20081705085031));
#14719=CARTESIAN_POINT('Ctrl Pts',(9.70137142052945,-22.8189810445333,-1.7468948445434E-11));
#14720=CARTESIAN_POINT('Ctrl Pts',(7.27602856538952,-22.6439810445334,-4.20081705087651));
#14721=CARTESIAN_POINT('Ctrl Pts',(4.8506857102496,-22.4689810445334,-8.40163410173556));
#14722=CARTESIAN_POINT('Ctrl Pts',(-1.5130096486293E-11,-22.2939810445333,
-8.40163410172683));
#14723=CARTESIAN_POINT('Ctrl Pts',(-4.85068571027985,-22.1189810445334,
-8.40163410171809));
#14724=CARTESIAN_POINT('Ctrl Pts',(-7.27602856540465,-21.9439810445333,
-4.20081705085031));
#14725=CARTESIAN_POINT('Ctrl Pts',(-9.70137142052945,-21.7689810445334,
1.74701365207797E-11));
#14726=CARTESIAN_POINT('Ctrl Pts',(-7.27602856538952,-21.5939810445333,
4.20081705087652));
#14727=CARTESIAN_POINT('Ctrl Pts',(-4.8506857102496,-21.4189810445334,8.40163410173556));
#14728=CARTESIAN_POINT('Ctrl Pts',(1.5129067582862E-11,-21.2439810445334,
8.40163410172683));
#14729=CARTESIAN_POINT('Ctrl Pts',(4.85068571027985,-21.0689810445333,8.40163410171809));
#14730=CARTESIAN_POINT('Ctrl Pts',(7.27602856540465,-20.8939810445334,4.20081705085031));
#14731=CARTESIAN_POINT('Ctrl Pts',(9.70137142052945,-20.7189810445334,-1.7468948445434E-11));
#14732=CARTESIAN_POINT('Ctrl Pts',(7.27602856538952,-20.5439810445333,-4.20081705087651));
#14733=CARTESIAN_POINT('Ctrl Pts',(4.8506857102496,-20.3689810445334,-8.40163410173556));
#14734=CARTESIAN_POINT('Ctrl Pts',(-1.5130096486293E-11,-20.1939810445334,
-8.40163410172683));
#14735=CARTESIAN_POINT('Ctrl Pts',(-4.85068571027985,-20.0189810445333,
-8.40163410171809));
#14736=CARTESIAN_POINT('Ctrl Pts',(-7.27602856540465,-19.8439810445334,
-4.20081705085031));
#14737=CARTESIAN_POINT('Ctrl Pts',(-9.70137142052945,-19.6689810445333,
1.74701365207797E-11));
#14738=CARTESIAN_POINT('Ctrl Pts',(-7.27602856538952,-19.4939810445334,
4.20081705087652));
#14739=CARTESIAN_POINT('Ctrl Pts',(-4.8506857102496,-19.3189810445334,8.40163410173556));
#14740=CARTESIAN_POINT('Ctrl Pts',(1.5129067582862E-11,-19.1439810445333,
8.40163410172683));
#14741=CARTESIAN_POINT('Ctrl Pts',(4.85068571027985,-18.9689810445334,8.40163410171809));
#14742=CARTESIAN_POINT('Ctrl Pts',(7.27602856540465,-18.7939810445333,4.20081705085031));
#14743=CARTESIAN_POINT('Ctrl Pts',(9.70137142052945,-18.6189810445334,-1.7468948445434E-11));
#14744=CARTESIAN_POINT('Ctrl Pts',(7.27602856538952,-18.4439810445334,-4.20081705087651));
#14745=CARTESIAN_POINT('Ctrl Pts',(4.8506857102496,-18.2689810445334,-8.40163410173556));
#14746=CARTESIAN_POINT('Ctrl Pts',(-1.5130096486293E-11,-18.0939810445334,
-8.40163410172683));
#14747=CARTESIAN_POINT('Ctrl Pts',(-4.85068571027985,-17.9189810445334,
-8.40163410171809));
#14748=CARTESIAN_POINT('Ctrl Pts',(-7.27602856540465,-17.7439810445334,
-4.20081705085031));
#14749=CARTESIAN_POINT('Ctrl Pts',(-9.70137142052945,-17.5689810445334,
1.74701365207797E-11));
#14750=CARTESIAN_POINT('Ctrl Pts',(-7.27602856538952,-17.3939810445334,
4.20081705087652));
#14751=CARTESIAN_POINT('Ctrl Pts',(-4.8506857102496,-17.2189810445334,8.40163410173556));
#14752=CARTESIAN_POINT('Ctrl Pts',(1.5129067582862E-11,-17.0439810445334,
8.40163410172683));
#14753=CARTESIAN_POINT('Ctrl Pts',(4.85068571027985,-16.8689810445334,8.40163410171809));
#14754=CARTESIAN_POINT('Ctrl Pts',(7.27602856540465,-16.6939810445334,4.20081705085031));
#14755=CARTESIAN_POINT('Ctrl Pts',(9.70137142052945,-16.5189810445334,-1.7468948445434E-11));
#14756=CARTESIAN_POINT('Ctrl Pts',(7.27602856538952,-16.3439810445334,-4.20081705087651));
#14757=CARTESIAN_POINT('Ctrl Pts',(4.8506857102496,-16.1689810445334,-8.40163410173556));
#14758=CARTESIAN_POINT('Ctrl Pts',(-1.5130096486293E-11,-15.9939810445334,
-8.40163410172683));
#14759=CARTESIAN_POINT('Ctrl Pts',(-4.85068571027985,-15.8189810445334,
-8.40163410171809));
#14760=CARTESIAN_POINT('Ctrl Pts',(-7.27602856540465,-15.6439810445334,
-4.20081705085031));
#14761=CARTESIAN_POINT('Ctrl Pts',(-9.70137142052945,-15.4689810445334,
1.74701365207797E-11));
#14762=CARTESIAN_POINT('Ctrl Pts',(-7.27602856538952,-15.2939810445334,
4.20081705087652));
#14763=CARTESIAN_POINT('Ctrl Pts',(-4.8506857102496,-15.1189810445334,8.40163410173556));
#14764=CARTESIAN_POINT('Ctrl Pts',(1.5129067582862E-11,-14.9439810445334,
8.40163410172683));
#14765=CARTESIAN_POINT('Ctrl Pts',(4.85068571027985,-14.7689810445334,8.40163410171809));
#14766=CARTESIAN_POINT('Ctrl Pts',(7.27602856540465,-14.5939810445334,4.20081705085031));
#14767=CARTESIAN_POINT('Ctrl Pts',(9.70137142052945,-14.4189810445334,-1.7468948445434E-11));
#14768=CARTESIAN_POINT('Ctrl Pts',(7.27602856538952,-14.2439810445334,-4.20081705087651));
#14769=CARTESIAN_POINT('Ctrl Pts',(4.8506857102496,-14.0689810445334,-8.40163410173556));
#14770=CARTESIAN_POINT('Ctrl Pts',(-1.5130096486293E-11,-13.8939810445334,
-8.40163410172683));
#14771=CARTESIAN_POINT('Ctrl Pts',(-4.85068571027985,-13.7189810445334,
-8.40163410171809));
#14772=CARTESIAN_POINT('Ctrl Pts',(-7.27602856540465,-13.5439810445334,
-4.20081705085031));
#14773=CARTESIAN_POINT('Ctrl Pts',(-9.70137142052945,-13.3689810445334,
1.74701365207797E-11));
#14774=CARTESIAN_POINT('Ctrl Pts',(-7.27602856538952,-13.1939810445334,
4.20081705087652));
#14775=CARTESIAN_POINT('Ctrl Pts',(-4.8506857102496,-13.0189810445334,8.40163410173556));
#14776=CARTESIAN_POINT('Ctrl Pts',(1.5129067582862E-11,-12.8439810445334,
8.40163410172683));
#14777=CARTESIAN_POINT('Ctrl Pts',(4.85068571027985,-12.6689810445334,8.40163410171809));
#14778=CARTESIAN_POINT('Ctrl Pts',(7.27602856540465,-12.4939810445334,4.20081705085031));
#14779=CARTESIAN_POINT('Ctrl Pts',(9.70137142052945,-12.3189810445334,-1.7468948445434E-11));
#14780=CARTESIAN_POINT('Ctrl Pts',(7.27602856538952,-12.1439810445334,-4.20081705087651));
#14781=CARTESIAN_POINT('Ctrl Pts',(4.8506857102496,-11.9689810445334,-8.40163410173556));
#14782=CARTESIAN_POINT('Ctrl Pts',(-1.5130096486293E-11,-11.7939810445334,
-8.40163410172683));
#14783=CARTESIAN_POINT('Ctrl Pts',(-4.85068571027985,-11.6189810445334,
-8.40163410171809));
#14784=CARTESIAN_POINT('Ctrl Pts',(-7.27602856540465,-11.4439810445334,
-4.20081705085031));
#14785=CARTESIAN_POINT('Ctrl Pts',(-9.70137142052945,-11.2689810445334,
1.74701365207797E-11));
#14786=CARTESIAN_POINT('Ctrl Pts',(-7.27602856538952,-11.0939810445334,
4.20081705087652));
#14787=CARTESIAN_POINT('Ctrl Pts',(-4.8506857102496,-10.9189810445334,8.40163410173556));
#14788=CARTESIAN_POINT('Ctrl Pts',(1.5129067582862E-11,-10.7439810445334,
8.40163410172683));
#14789=CARTESIAN_POINT('Ctrl Pts',(4.85068571027985,-10.5689810445334,8.40163410171809));
#14790=CARTESIAN_POINT('Ctrl Pts',(7.27602856540465,-10.3939810445334,4.20081705085031));
#14791=CARTESIAN_POINT('Ctrl Pts',(9.70137142052945,-10.2189810445334,-1.7468948445434E-11));
#14792=CARTESIAN_POINT('Ctrl Pts',(7.27602856538952,-10.0439810445334,-4.20081705087651));
#14793=CARTESIAN_POINT('Ctrl Pts',(4.8506857102496,-9.86898104453339,-8.40163410173556));
#14794=CARTESIAN_POINT('Ctrl Pts',(-1.5130096486293E-11,-9.69398104453338,
-8.40163410172683));
#14795=CARTESIAN_POINT('Ctrl Pts',(-4.85068571027985,-9.51898104453338,
-8.40163410171809));
#14796=CARTESIAN_POINT('Ctrl Pts',(-7.27602856540465,-9.34398104453339,
-4.20081705085031));
#14797=CARTESIAN_POINT('Ctrl Pts',(-9.70137142052945,-9.16898104453338,
1.74701365207797E-11));
#14798=CARTESIAN_POINT('Ctrl Pts',(-7.27602856538952,-8.99398104453337,
4.20081705087652));
#14799=CARTESIAN_POINT('Ctrl Pts',(-4.8506857102496,-8.8189810445334,8.40163410173556));
#14800=CARTESIAN_POINT('Ctrl Pts',(1.5129067582862E-11,-8.64398104453338,
8.40163410172683));
#14801=CARTESIAN_POINT('Ctrl Pts',(4.85068571027985,-8.46898104453338,8.40163410171809));
#14802=CARTESIAN_POINT('Ctrl Pts',(7.27602856540465,-8.29398104453339,4.20081705085031));
#14803=CARTESIAN_POINT('Ctrl Pts',(9.70137142052945,-8.11898104453338,-1.7468948445434E-11));
#14804=CARTESIAN_POINT('Ctrl Pts',(7.27602856538952,-7.94398104453338,-4.20081705087651));
#14805=CARTESIAN_POINT('Ctrl Pts',(4.8506857102496,-7.7689810445334,-8.40163410173556));
#14806=CARTESIAN_POINT('Ctrl Pts',(-1.5130096486293E-11,-7.59398104453339,
-8.40163410172683));
#14807=CARTESIAN_POINT('Ctrl Pts',(-4.85068571027985,-7.41898104453339,
-8.40163410171809));
#14808=CARTESIAN_POINT('Ctrl Pts',(-7.27602856540465,-7.24398104453337,
-4.20081705085031));
#14809=CARTESIAN_POINT('Ctrl Pts',(-9.70137142052945,-7.06898104453339,
1.74701365207797E-11));
#14810=CARTESIAN_POINT('Ctrl Pts',(-7.27602856538952,-6.89398104453338,
4.20081705087652));
#14811=CARTESIAN_POINT('Ctrl Pts',(-4.8506857102496,-6.71898104453338,8.40163410173556));
#14812=CARTESIAN_POINT('Ctrl Pts',(1.5129067582862E-11,-6.54398104453339,
8.40163410172683));
#14813=CARTESIAN_POINT('Ctrl Pts',(4.85068571027985,-6.36898104453339,8.40163410171809));
#14814=CARTESIAN_POINT('Ctrl Pts',(7.27602856540465,-6.19398104453338,4.20081705085031));
#14815=CARTESIAN_POINT('Ctrl Pts',(9.70137142052945,-6.01898104453339,-1.7468948445434E-11));
#14816=CARTESIAN_POINT('Ctrl Pts',(7.27602856538952,-5.84398104453339,-4.20081705087651));
#14817=CARTESIAN_POINT('Ctrl Pts',(4.8506857102496,-5.66898104453338,-8.40163410173556));
#14818=CARTESIAN_POINT('Ctrl Pts',(-1.5130096486293E-11,-5.4939810445334,
-8.40163410172683));
#14819=CARTESIAN_POINT('Ctrl Pts',(-4.85068571027985,-5.3189810445334,-8.40163410171809));
#14820=CARTESIAN_POINT('Ctrl Pts',(-7.27602856540465,-5.14398104453338,
-4.20081705085031));
#14821=CARTESIAN_POINT('Ctrl Pts',(-9.70137142052945,-4.9689810445334,1.74701365207797E-11));
#14822=CARTESIAN_POINT('Ctrl Pts',(-7.27602856538952,-4.79398104453339,
4.20081705087652));
#14823=CARTESIAN_POINT('Ctrl Pts',(-4.8506857102496,-4.61898104453338,8.40163410173556));
#14824=CARTESIAN_POINT('Ctrl Pts',(1.5129067582862E-11,-4.4439810445334,
8.40163410172683));
#14825=CARTESIAN_POINT('Ctrl Pts',(4.85068571027985,-4.2689810445334,8.40163410171809));
#14826=CARTESIAN_POINT('Ctrl Pts',(7.27602856540465,-4.09398104453338,4.20081705085031));
#14827=CARTESIAN_POINT('Ctrl Pts',(9.70137142052945,-3.9189810445334,-1.7468948445434E-11));
#14828=CARTESIAN_POINT('Ctrl Pts',(7.27602856538952,-3.74398104453339,-4.20081705087651));
#14829=CARTESIAN_POINT('Ctrl Pts',(4.8506857102496,-3.56898104453339,-8.40163410173556));
#14830=CARTESIAN_POINT('Ctrl Pts',(-1.5130096486293E-11,-3.39398104453341,
-8.40163410172683));
#14831=CARTESIAN_POINT('Ctrl Pts',(-4.85068571027985,-3.21898104453341,
-8.40163410171809));
#14832=CARTESIAN_POINT('Ctrl Pts',(-7.27602856540465,-3.04398104453339,
-4.20081705085031));
#14833=CARTESIAN_POINT('Ctrl Pts',(-9.70137142052945,-2.86898104453339,
1.74701365207797E-11));
#14834=CARTESIAN_POINT('Ctrl Pts',(-7.27602856538952,-2.6939810445334,4.20081705087652));
#14835=CARTESIAN_POINT('Ctrl Pts',(-4.8506857102496,-2.51898104453339,8.40163410173556));
#14836=CARTESIAN_POINT('Ctrl Pts',(1.5129067582862E-11,-2.34398104453338,
8.40163410172683));
#14837=CARTESIAN_POINT('Ctrl Pts',(4.85068571027985,-2.1689810445334,8.40163410171809));
#14838=CARTESIAN_POINT('Ctrl Pts',(7.27602856540465,-1.99398104453339,4.20081705085031));
#14839=CARTESIAN_POINT('Ctrl Pts',(9.70137142052945,-1.81898104453339,-1.7468948445434E-11));
#14840=CARTESIAN_POINT('Ctrl Pts',(7.27602856538952,-1.6439810445334,-4.20081705087651));
#14841=CARTESIAN_POINT('Ctrl Pts',(4.8506857102496,-1.4689810445334,-8.40163410173556));
#14842=CARTESIAN_POINT('Ctrl Pts',(-1.5130096486293E-11,-1.29398104453339,
-8.40163410172683));
#14843=CARTESIAN_POINT('Ctrl Pts',(-4.85068571027985,-1.11898104453341,
-8.40163410171809));
#14844=CARTESIAN_POINT('Ctrl Pts',(-7.27602856540465,-0.943981044533398,
-4.20081705085031));
#14845=CARTESIAN_POINT('Ctrl Pts',(-9.70137142052945,-0.768981044533393,
1.74701365207797E-11));
#14846=CARTESIAN_POINT('Ctrl Pts',(-7.27602856538952,-0.593981044533408,
4.20081705087652));
#14847=CARTESIAN_POINT('Ctrl Pts',(-4.8506857102496,-0.418981044533402,
8.40163410173556));
#14848=CARTESIAN_POINT('Ctrl Pts',(1.5129067582862E-11,-0.243981044533391,
8.40163410172683));
#14849=CARTESIAN_POINT('Ctrl Pts',(4.85068571027985,-0.0689810445334119,
8.40163410171809));
#14850=CARTESIAN_POINT('Ctrl Pts',(7.27602856540465,0.106018955466598,4.20081705085031));
#14851=CARTESIAN_POINT('Ctrl Pts',(9.70137142052945,0.281018955466602,-1.7468948445434E-11));
#14852=CARTESIAN_POINT('Ctrl Pts',(7.27602856538952,0.456018955466587,-4.20081705087651));
#14853=CARTESIAN_POINT('Ctrl Pts',(4.8506857102496,0.631018955466593,-8.40163410173556));
#14854=CARTESIAN_POINT('Ctrl Pts',(-1.5130096486293E-11,0.806018955466604,
-8.40163410172683));
#14855=CARTESIAN_POINT('Ctrl Pts',(-4.85068571027985,0.981018955466583,
-8.40163410171809));
#14856=CARTESIAN_POINT('Ctrl Pts',(-7.27602856540465,1.15601895546659,-4.20081705085031));
#14857=CARTESIAN_POINT('Ctrl Pts',(-9.70137142052945,1.3310189554666,1.74701365207797E-11));
#14858=CARTESIAN_POINT('Ctrl Pts',(-7.27602856538952,1.50601895546661,4.20081705087652));
#14859=CARTESIAN_POINT('Ctrl Pts',(-4.8506857102496,1.68101895546659,8.40163410173556));
#14860=CARTESIAN_POINT('Ctrl Pts',(1.5129067582862E-11,1.8560189554666,
8.40163410172683));
#14861=CARTESIAN_POINT('Ctrl Pts',(4.85068571027985,2.0310189554666,8.40163410171809));
#14862=CARTESIAN_POINT('Ctrl Pts',(7.27602856540465,2.20601895546659,4.20081705085031));
#14863=CARTESIAN_POINT('Ctrl Pts',(9.70137142052945,2.38101895546659,-1.7468948445434E-11));
#14864=CARTESIAN_POINT('Ctrl Pts',(7.27602856538952,2.55601895546661,-4.20081705087651));
#14865=CARTESIAN_POINT('Ctrl Pts',(4.8506857102496,2.73101895546658,-8.40163410173556));
#14866=CARTESIAN_POINT('Ctrl Pts',(-1.5130096486293E-11,2.9060189554666,
-8.40163410172683));
#14867=CARTESIAN_POINT('Ctrl Pts',(-4.85068571027985,3.0810189554666,-8.40163410171809));
#14868=CARTESIAN_POINT('Ctrl Pts',(-7.27602856540465,3.25601895546658,-4.20081705085031));
#14869=CARTESIAN_POINT('Ctrl Pts',(-9.70137142052945,3.43101895546659,1.74701365207797E-11));
#14870=CARTESIAN_POINT('Ctrl Pts',(-7.27602856538952,3.6060189554666,4.20081705087652));
#14871=CARTESIAN_POINT('Ctrl Pts',(-4.8506857102496,3.78101895546658,8.40163410173556));
#14872=CARTESIAN_POINT('Ctrl Pts',(1.5129067582862E-11,3.95601895546659,
8.40163410172683));
#14873=CARTESIAN_POINT('Ctrl Pts',(4.85068571027985,4.13101895546659,8.40163410171809));
#14874=CARTESIAN_POINT('Ctrl Pts',(7.27602856540465,4.30601895546658,4.20081705085031));
#14875=CARTESIAN_POINT('Ctrl Pts',(9.70137142052945,4.48101895546658,-1.7468948445434E-11));
#14876=CARTESIAN_POINT('Ctrl Pts',(7.27602856538952,4.6560189554666,-4.20081705087651));
#14877=CARTESIAN_POINT('Ctrl Pts',(4.8506857102496,4.83101895546658,-8.40163410173556));
#14878=CARTESIAN_POINT('Ctrl Pts',(-1.5130096486293E-11,5.00601895546659,
-8.40163410172683));
#14879=CARTESIAN_POINT('Ctrl Pts',(-4.85068571027985,5.18101895546659,-8.40163410171809));
#14880=CARTESIAN_POINT('Ctrl Pts',(-7.27602856540465,5.35601895546657,-4.20081705085031));
#14881=CARTESIAN_POINT('Ctrl Pts',(-9.70137142052945,5.53101895546658,1.74701365207797E-11));
#14882=CARTESIAN_POINT('Ctrl Pts',(-7.27602856538952,5.70601895546659,4.20081705087652));
#14883=CARTESIAN_POINT('Ctrl Pts',(-4.8506857102496,5.88101895546657,8.40163410173556));
#14884=CARTESIAN_POINT('Ctrl Pts',(1.5129067582862E-11,6.05601895546658,
8.40163410172683));
#14885=CARTESIAN_POINT('Ctrl Pts',(4.85068571027985,6.23101895546658,8.40163410171809));
#14886=CARTESIAN_POINT('Ctrl Pts',(7.27602856540465,6.4060189554666,4.20081705085031));
#14887=CARTESIAN_POINT('Ctrl Pts',(9.70137142052945,6.58101895546657,-1.7468948445434E-11));
#14888=CARTESIAN_POINT('Ctrl Pts',(7.27602856538952,6.75601895546659,-4.20081705087651));
#14889=CARTESIAN_POINT('Ctrl Pts',(4.8506857102496,6.93101895546659,-8.40163410173556));
#14890=CARTESIAN_POINT('Ctrl Pts',(-1.5130096486293E-11,7.10601895546658,
-8.40163410172683));
#14891=CARTESIAN_POINT('Ctrl Pts',(-4.85068571027985,7.28101895546658,-8.40163410171809));
#14892=CARTESIAN_POINT('Ctrl Pts',(-7.27602856540465,7.45601895546659,-4.20081705085031));
#14893=CARTESIAN_POINT('Ctrl Pts',(-9.70137142052945,7.63101895546657,1.74701365207797E-11));
#14894=CARTESIAN_POINT('Ctrl Pts',(-7.27602856538952,7.80601895546658,4.20081705087652));
#14895=CARTESIAN_POINT('Ctrl Pts',(-4.8506857102496,7.98101895546658,8.40163410173556));
#14896=CARTESIAN_POINT('Ctrl Pts',(1.5129067582862E-11,8.15601895546657,
8.40163410172683));
#14897=CARTESIAN_POINT('Ctrl Pts',(4.85068571027985,8.33101895546658,8.40163410171809));
#14898=CARTESIAN_POINT('Ctrl Pts',(7.27602856540465,8.50601895546659,4.20081705085031));
#14899=CARTESIAN_POINT('Ctrl Pts',(9.70137142052945,8.68101895546657,-1.7468948445434E-11));
#14900=CARTESIAN_POINT('Ctrl Pts',(7.27602856538952,8.85601895546658,-4.20081705087651));
#14901=CARTESIAN_POINT('Ctrl Pts',(4.8506857102496,9.03101895546658,-8.40163410173556));
#14902=CARTESIAN_POINT('Ctrl Pts',(-1.5130096486293E-11,9.20601895546657,
-8.40163410172683));
#14903=CARTESIAN_POINT('Ctrl Pts',(-4.85068571027985,9.38101895546657,-8.40163410171809));
#14904=CARTESIAN_POINT('Ctrl Pts',(-7.27602856540465,9.55601895546659,-4.20081705085031));
#14905=CARTESIAN_POINT('Ctrl Pts',(-9.70137142052945,9.73101895546656,1.74701365207797E-11));
#14906=CARTESIAN_POINT('Ctrl Pts',(-7.27602856538952,9.90601895546657,4.20081705087652));
#14907=CARTESIAN_POINT('Ctrl Pts',(-4.8506857102496,10.0810189554666,8.40163410173556));
#14908=CARTESIAN_POINT('Ctrl Pts',(1.5129067582862E-11,10.2560189554666,
8.40163410172683));
#14909=CARTESIAN_POINT('Ctrl Pts',(4.85068571027985,10.4310189554666,8.40163410171809));
#14910=CARTESIAN_POINT('Ctrl Pts',(7.27602856540465,10.6060189554666,4.20081705085031));
#14911=CARTESIAN_POINT('Ctrl Pts',(9.70137142052945,10.7810189554666,-1.7468948445434E-11));
#14912=CARTESIAN_POINT('Ctrl Pts',(7.27602856538952,10.9560189554666,-4.20081705087651));
#14913=CARTESIAN_POINT('Ctrl Pts',(4.8506857102496,11.1310189554666,-8.40163410173556));
#14914=CARTESIAN_POINT('Ctrl Pts',(-1.5130096486293E-11,11.3060189554666,
-8.40163410172683));
#14915=CARTESIAN_POINT('Ctrl Pts',(-4.85068571027985,11.4810189554666,-8.40163410171809));
#14916=CARTESIAN_POINT('Ctrl Pts',(-7.27602856540465,11.6560189554666,-4.20081705085031));
#14917=CARTESIAN_POINT('Ctrl Pts',(-9.70137142052945,11.8310189554666,1.74701365207797E-11));
#14918=CARTESIAN_POINT('Ctrl Pts',(-7.27602856538952,12.0060189554666,4.20081705087652));
#14919=CARTESIAN_POINT('Ctrl Pts',(-4.8506857102496,12.1810189554666,8.40163410173556));
#14920=CARTESIAN_POINT('Ctrl Pts',(1.5129067582862E-11,12.3560189554666,
8.40163410172683));
#14921=CARTESIAN_POINT('Ctrl Pts',(4.85068571027985,12.5310189554666,8.40163410171809));
#14922=CARTESIAN_POINT('Ctrl Pts',(7.27602856540465,12.7060189554666,4.20081705085031));
#14923=CARTESIAN_POINT('Ctrl Pts',(9.70137142052945,12.8810189554666,-1.7468948445434E-11));
#14924=CARTESIAN_POINT('Ctrl Pts',(7.27602856538952,13.0560189554666,-4.20081705087651));
#14925=CARTESIAN_POINT('Ctrl Pts',(4.8506857102496,13.2310189554666,-8.40163410173556));
#14926=CARTESIAN_POINT('Ctrl Pts',(-1.5130096486293E-11,13.4060189554666,
-8.40163410172683));
#14927=CARTESIAN_POINT('Ctrl Pts',(-4.85068571027985,13.5810189554666,-8.40163410171809));
#14928=CARTESIAN_POINT('Ctrl Pts',(-7.27602856540465,13.7560189554666,-4.20081705085031));
#14929=CARTESIAN_POINT('Ctrl Pts',(-9.70137142052945,13.9310189554666,1.74701365207797E-11));
#14930=CARTESIAN_POINT('Ctrl Pts',(-7.27602856538952,14.1060189554666,4.20081705087652));
#14931=CARTESIAN_POINT('Ctrl Pts',(-4.8506857102496,14.2810189554666,8.40163410173556));
#14932=CARTESIAN_POINT('Ctrl Pts',(1.5129067582862E-11,14.4560189554666,
8.40163410172683));
#14933=CARTESIAN_POINT('Ctrl Pts',(4.85068571027985,14.6310189554665,8.40163410171809));
#14934=CARTESIAN_POINT('Ctrl Pts',(7.27602856540465,14.8060189554666,4.20081705085031));
#14935=CARTESIAN_POINT('Ctrl Pts',(9.70137142052945,14.9810189554666,-1.7468948445434E-11));
#14936=CARTESIAN_POINT('Ctrl Pts',(7.27602856538952,15.1560189554666,-4.20081705087651));
#14937=CARTESIAN_POINT('Ctrl Pts',(4.8506857102496,15.3310189554666,-8.40163410173556));
#14938=CARTESIAN_POINT('Ctrl Pts',(-1.5130096486293E-11,15.5060189554666,
-8.40163410172683));
#14939=CARTESIAN_POINT('Ctrl Pts',(-4.85068571027985,15.6810189554666,-8.40163410171809));
#14940=CARTESIAN_POINT('Ctrl Pts',(-7.27602856540465,15.8560189554666,-4.20081705085031));
#14941=CARTESIAN_POINT('Ctrl Pts',(-9.70137142052945,16.0310189554666,1.74701365207797E-11));
#14942=CARTESIAN_POINT('Ctrl Pts',(-7.27602856538952,16.2060189554666,4.20081705087652));
#14943=CARTESIAN_POINT('Ctrl Pts',(-4.8506857102496,16.3810189554665,8.40163410173556));
#14944=CARTESIAN_POINT('Ctrl Pts',(1.5129067582862E-11,16.5560189554666,
8.40163410172683));
#14945=CARTESIAN_POINT('Ctrl Pts',(4.85068571027985,16.7310189554666,8.40163410171809));
#14946=CARTESIAN_POINT('Ctrl Pts',(7.27602856540465,16.9060189554666,4.20081705085031));
#14947=CARTESIAN_POINT('Ctrl Pts',(9.70137142052945,17.0810189554666,-1.7468948445434E-11));
#14948=CARTESIAN_POINT('Ctrl Pts',(7.27602856538952,17.2560189554666,-4.20081705087651));
#14949=CARTESIAN_POINT('Ctrl Pts',(4.8506857102496,17.4310189554665,-8.40163410173556));
#14950=CARTESIAN_POINT('Ctrl Pts',(-1.5130096486293E-11,17.6060189554666,
-8.40163410172683));
#14951=CARTESIAN_POINT('Ctrl Pts',(-4.85068571027985,17.7810189554666,-8.40163410171809));
#14952=CARTESIAN_POINT('Ctrl Pts',(-7.27602856540465,17.9560189554665,-4.20081705085031));
#14953=CARTESIAN_POINT('Ctrl Pts',(-9.70137142052945,18.1310189554665,1.74701365207797E-11));
#14954=CARTESIAN_POINT('Ctrl Pts',(-7.27602856538952,18.3060189554666,4.20081705087652));
#14955=CARTESIAN_POINT('Ctrl Pts',(-4.8506857102496,18.4810189554665,8.40163410173556));
#14956=CARTESIAN_POINT('Ctrl Pts',(1.5129067582862E-11,18.6560189554666,
8.40163410172683));
#14957=CARTESIAN_POINT('Ctrl Pts',(4.85068571027985,18.8310189554666,8.40163410171809));
#14958=CARTESIAN_POINT('Ctrl Pts',(7.27602856540465,19.0060189554665,4.20081705085031));
#14959=CARTESIAN_POINT('Ctrl Pts',(9.70137142052945,19.1810189554665,-1.7468948445434E-11));
#14960=CARTESIAN_POINT('Ctrl Pts',(7.27602856538952,19.3560189554666,-4.20081705087651));
#14961=CARTESIAN_POINT('Ctrl Pts',(4.8506857102496,19.5310189554666,-8.40163410173556));
#14962=CARTESIAN_POINT('Ctrl Pts',(-1.5130096486293E-11,19.7060189554665,
-8.40163410172683));
#14963=CARTESIAN_POINT('Ctrl Pts',(-4.85068571027985,19.8810189554666,-8.40163410171809));
#14964=CARTESIAN_POINT('Ctrl Pts',(-7.27602856540465,20.0560189554666,-4.20081705085031));
#14965=CARTESIAN_POINT('Ctrl Pts',(-9.70137142052945,20.2310189554665,1.74701365207797E-11));
#14966=CARTESIAN_POINT('Ctrl Pts',(-7.27602856538952,20.4060189554666,4.20081705087652));
#14967=CARTESIAN_POINT('Ctrl Pts',(-4.8506857102496,20.5810189554666,8.40163410173556));
#14968=CARTESIAN_POINT('Ctrl Pts',(1.5129067582862E-11,20.7560189554665,
8.40163410172683));
#14969=CARTESIAN_POINT('Ctrl Pts',(4.85068571027985,20.9310189554666,8.40163410171809));
#14970=CARTESIAN_POINT('Ctrl Pts',(7.27602856540465,21.1060189554666,4.20081705085031));
#14971=CARTESIAN_POINT('Ctrl Pts',(9.70137142052945,21.2810189554665,-1.7468948445434E-11));
#14972=CARTESIAN_POINT('Ctrl Pts',(7.27602856538952,21.4560189554666,-4.20081705087651));
#14973=CARTESIAN_POINT('Ctrl Pts',(4.8506857102496,21.6310189554666,-8.40163410173556));
#14974=CARTESIAN_POINT('Ctrl Pts',(-1.5130096486293E-11,21.8060189554665,
-8.40163410172683));
#14975=CARTESIAN_POINT('Ctrl Pts',(-4.85068571027985,21.9810189554665,-8.40163410171809));
#14976=CARTESIAN_POINT('Ctrl Pts',(-7.27602856540465,22.1560189554666,-4.20081705085031));
#14977=CARTESIAN_POINT('Ctrl Pts',(-9.70137142052945,22.3310189554665,1.74701365207797E-11));
#14978=CARTESIAN_POINT('Ctrl Pts',(-7.27602856538952,22.5060189554665,4.20081705087652));
#14979=CARTESIAN_POINT('Ctrl Pts',(-4.8506857102496,22.6810189554666,8.40163410173556));
#14980=CARTESIAN_POINT('Ctrl Pts',(1.5129067582862E-11,22.8560189554665,
8.40163410172683));
#14981=CARTESIAN_POINT('Ctrl Pts',(4.85068571027985,23.0310189554665,8.40163410171809));
#14982=CARTESIAN_POINT('Ctrl Pts',(7.27602856540465,23.2060189554666,4.20081705085031));
#14983=CARTESIAN_POINT('Ctrl Pts',(9.70137142052945,23.3810189554665,-1.7468948445434E-11));
#14984=CARTESIAN_POINT('Ctrl Pts',(7.27602856538952,23.5560189554665,-4.20081705087651));
#14985=CARTESIAN_POINT('Ctrl Pts',(4.8506857102496,23.7310189554665,-8.40163410173556));
#14986=CARTESIAN_POINT('Ctrl Pts',(-1.5130096486293E-11,23.9060189554665,
-8.40163410172683));
#14987=CARTESIAN_POINT('Ctrl Pts',(-4.85068571027985,24.0810189554665,-8.40163410171809));
#14988=CARTESIAN_POINT('Ctrl Pts',(-7.27602856540465,24.2560189554665,-4.20081705085031));
#14989=CARTESIAN_POINT('Ctrl Pts',(-9.70137142052945,24.4310189554665,1.74701365207797E-11));
#14990=CARTESIAN_POINT('Ctrl Pts',(-7.27602856538952,24.6060189554665,4.20081705087652));
#14991=CARTESIAN_POINT('Ctrl Pts',(-4.8506857102496,24.7810189554665,8.40163410173556));
#14992=CARTESIAN_POINT('Ctrl Pts',(1.5129067582862E-11,24.9560189554666,
8.40163410172683));
#14993=CARTESIAN_POINT('Ctrl Pts',(4.85068571027985,25.1310189554665,8.40163410171809));
#14994=CARTESIAN_POINT('Ctrl Pts',(7.27602856540465,25.3060189554665,4.20081705085031));
#14995=CARTESIAN_POINT('Ctrl Pts',(9.70137142052945,25.4810189554665,-1.7468948445434E-11));
#14996=CARTESIAN_POINT('Ctrl Pts',(7.27602856538952,25.6560189554665,-4.20081705087651));
#14997=CARTESIAN_POINT('Ctrl Pts',(4.8506857102496,25.8310189554665,-8.40163410173556));
#14998=CARTESIAN_POINT('Ctrl Pts',(-1.5130096486293E-11,26.0060189554665,
-8.40163410172683));
#14999=CARTESIAN_POINT('Ctrl Pts',(8.29083424217445,-24.9756402675196,1.3600098358447));
#15000=CARTESIAN_POINT('Ctrl Pts',(8.77665986763609,-24.8522614613838,-1.60165972355344));
#15001=CARTESIAN_POINT('Ctrl Pts',(7.27603390512277,-24.7439842542419,-4.20082013377283));
#15002=CARTESIAN_POINT('Ctrl Pts',(4.85068927007217,-24.5689842542419,-8.40164026752811));
#15003=CARTESIAN_POINT('Ctrl Pts',(-1.48337207789367E-11,-24.3939842542419,
-8.40164026751963));
#15004=CARTESIAN_POINT('Ctrl Pts',(-4.85068927010184,-24.2189842542419,
-8.40164026751098));
#15005=CARTESIAN_POINT('Ctrl Pts',(-7.27603390513761,-24.0439842542419,
-4.20082013374713));
#15006=CARTESIAN_POINT('Ctrl Pts',(-9.70137854017372,-23.8689842542419,
1.70762120011325E-11));
#15007=CARTESIAN_POINT('Ctrl Pts',(-7.27603390512282,-23.6939842542419,
4.20082013377275));
#15008=CARTESIAN_POINT('Ctrl Pts',(-4.85068927007226,-23.5189842542419,
8.40164026752806));
#15009=CARTESIAN_POINT('Ctrl Pts',(1.47431460078422E-11,-23.3439842542419,
8.40164026751963));
#15010=CARTESIAN_POINT('Ctrl Pts',(4.85068927010175,-23.1689842542419,8.40164026751103));
#15011=CARTESIAN_POINT('Ctrl Pts',(7.2760339051378,-22.9939842542419,4.2008201337468));
#15012=CARTESIAN_POINT('Ctrl Pts',(9.70137854017372,-22.8189842542419,-1.69716252641861E-11));
#15013=CARTESIAN_POINT('Ctrl Pts',(7.27603390512287,-22.6439842542419,-4.20082013377267));
#15014=CARTESIAN_POINT('Ctrl Pts',(4.85068927007187,-22.4689842542419,-8.40164026752828));
#15015=CARTESIAN_POINT('Ctrl Pts',(-1.46525712367478E-11,-22.2939842542419,
-8.40164026751963));
#15016=CARTESIAN_POINT('Ctrl Pts',(-4.85068927010165,-22.1189842542419,
-8.40164026751109));
#15017=CARTESIAN_POINT('Ctrl Pts',(-7.27603390513776,-21.9439842542419,
-4.20082013374688));
#15018=CARTESIAN_POINT('Ctrl Pts',(-9.70137854017372,-21.7689842542419,
1.68670385272398E-11));
#15019=CARTESIAN_POINT('Ctrl Pts',(-7.27603390512291,-21.5939842542419,
4.20082013377259));
#15020=CARTESIAN_POINT('Ctrl Pts',(-4.85068927007196,-21.4189842542419,
8.40164026752823));
#15021=CARTESIAN_POINT('Ctrl Pts',(1.45619964656533E-11,-21.2439842542419,
8.40164026751963));
#15022=CARTESIAN_POINT('Ctrl Pts',(4.85068927010157,-21.0689842542419,8.40164026751114));
#15023=CARTESIAN_POINT('Ctrl Pts',(7.27603390513771,-20.8939842542419,4.20082013374695));
#15024=CARTESIAN_POINT('Ctrl Pts',(9.70137854017372,-20.7189842542419,-1.73139113141798E-11));
#15025=CARTESIAN_POINT('Ctrl Pts',(7.27603390512296,-20.5439842542419,-4.20082013377251));
#15026=CARTESIAN_POINT('Ctrl Pts',(4.85068927007205,-20.3689842542419,-8.40164026752818));
#15027=CARTESIAN_POINT('Ctrl Pts',(-1.49489996514033E-11,-20.1939842542419,
-8.40164026751963));
#15028=CARTESIAN_POINT('Ctrl Pts',(-4.85068927010147,-20.0189842542419,
-8.40164026751119));
#15029=CARTESIAN_POINT('Ctrl Pts',(-7.27603390513767,-19.8439842542419,
-4.20082013374703));
#15030=CARTESIAN_POINT('Ctrl Pts',(-9.70137854017372,-19.6689842542419,
1.72093245772335E-11));
#15031=CARTESIAN_POINT('Ctrl Pts',(-7.276033905123,-19.4939842542419,4.20082013377243));
#15032=CARTESIAN_POINT('Ctrl Pts',(-4.85068927007214,-19.3189842542419,
8.40164026752813));
#15033=CARTESIAN_POINT('Ctrl Pts',(1.48584248803088E-11,-19.1439842542419,
8.40164026751963));
#15034=CARTESIAN_POINT('Ctrl Pts',(4.85068927010186,-18.9689842542419,8.40164026751097));
#15035=CARTESIAN_POINT('Ctrl Pts',(7.27603390513762,-18.7939842542419,4.20082013374711));
#15036=CARTESIAN_POINT('Ctrl Pts',(9.70137854017372,-18.6189842542419,-1.71047378402871E-11));
#15037=CARTESIAN_POINT('Ctrl Pts',(7.27603390512281,-18.4439842542419,-4.20082013377277));
#15038=CARTESIAN_POINT('Ctrl Pts',(4.85068927007223,-18.2689842542419,-8.40164026752807));
#15039=CARTESIAN_POINT('Ctrl Pts',(-1.47678501092144E-11,-18.0939842542419,
-8.40164026751963));
#15040=CARTESIAN_POINT('Ctrl Pts',(-4.85068927010177,-17.9189842542419,
-8.40164026751102));
#15041=CARTESIAN_POINT('Ctrl Pts',(-7.27603390513758,-17.7439842542419,
-4.20082013374719));
#15042=CARTESIAN_POINT('Ctrl Pts',(-9.70137854017372,-17.5689842542419,
1.70001511033408E-11));
#15043=CARTESIAN_POINT('Ctrl Pts',(-7.27603390512285,-17.3939842542419,
4.20082013377269));
#15044=CARTESIAN_POINT('Ctrl Pts',(-4.85068927007185,-17.2189842542419,
8.4016402675283));
#15045=CARTESIAN_POINT('Ctrl Pts',(1.46772753381199E-11,-17.0439842542419,
8.40164026751963));
#15046=CARTESIAN_POINT('Ctrl Pts',(4.85068927010168,-16.8689842542419,8.40164026751107));
#15047=CARTESIAN_POINT('Ctrl Pts',(7.27603390513777,-16.6939842542419,4.20082013374685));
#15048=CARTESIAN_POINT('Ctrl Pts',(9.70137854017372,-16.5189842542419,-1.68955643663944E-11));
#15049=CARTESIAN_POINT('Ctrl Pts',(7.2760339051229,-16.3439842542419,-4.20082013377261));
#15050=CARTESIAN_POINT('Ctrl Pts',(4.85068927007194,-16.1689842542419,-8.40164026752825));
#15051=CARTESIAN_POINT('Ctrl Pts',(-1.45867005670255E-11,-15.9939842542419,
-8.40164026751963));
#15052=CARTESIAN_POINT('Ctrl Pts',(-4.85068927010159,-15.8189842542419,
-8.40164026751112));
#15053=CARTESIAN_POINT('Ctrl Pts',(-7.27603390513773,-15.6439842542419,
-4.20082013374693));
#15054=CARTESIAN_POINT('Ctrl Pts',(-9.70137854017372,-15.4689842542419,
1.67909776294481E-11));
#15055=CARTESIAN_POINT('Ctrl Pts',(-7.27603390512294,-15.2939842542419,
4.20082013377253));
#15056=CARTESIAN_POINT('Ctrl Pts',(-4.85068927007203,-15.1189842542419,
8.40164026752819));
#15057=CARTESIAN_POINT('Ctrl Pts',(1.49737037527755E-11,-14.9439842542419,
8.40164026751963));
#15058=CARTESIAN_POINT('Ctrl Pts',(4.8506892701015,-14.7689842542419,8.40164026751117));
#15059=CARTESIAN_POINT('Ctrl Pts',(7.27603390513768,-14.5939842542419,4.20082013374701));
#15060=CARTESIAN_POINT('Ctrl Pts',(9.70137854017372,-14.4189842542419,-1.72378504163881E-11));
#15061=CARTESIAN_POINT('Ctrl Pts',(7.27603390512299,-14.2439842542419,-4.20082013377245));
#15062=CARTESIAN_POINT('Ctrl Pts',(4.85068927007212,-14.0689842542419,-8.40164026752814));
#15063=CARTESIAN_POINT('Ctrl Pts',(-1.4883128981681E-11,-13.8939842542419,
-8.40164026751963));
#15064=CARTESIAN_POINT('Ctrl Pts',(-4.85068927010141,-13.7189842542419,
-8.40164026751123));
#15065=CARTESIAN_POINT('Ctrl Pts',(-7.27603390513763,-13.5439842542419,
-4.20082013374709));
#15066=CARTESIAN_POINT('Ctrl Pts',(-9.70137854017372,-13.3689842542419,
1.71332636794417E-11));
#15067=CARTESIAN_POINT('Ctrl Pts',(-7.2760339051228,-13.193984254242,4.20082013377279));
#15068=CARTESIAN_POINT('Ctrl Pts',(-4.85068927007221,-13.018984254242,8.40164026752809));
#15069=CARTESIAN_POINT('Ctrl Pts',(1.47925542105866E-11,-12.8439842542419,
8.40164026751963));
#15070=CARTESIAN_POINT('Ctrl Pts',(4.85068927010179,-12.668984254242,8.401640267511));
#15071=CARTESIAN_POINT('Ctrl Pts',(7.27603390513759,-12.4939842542419,4.20082013374717));
#15072=CARTESIAN_POINT('Ctrl Pts',(9.70137854017372,-12.3189842542419,-1.70286769424954E-11));
#15073=CARTESIAN_POINT('Ctrl Pts',(7.27603390512284,-12.143984254242,-4.20082013377271));
#15074=CARTESIAN_POINT('Ctrl Pts',(4.8506892700723,-11.968984254242,-8.40164026752804));
#15075=CARTESIAN_POINT('Ctrl Pts',(-1.47019794394921E-11,-11.7939842542419,
-8.40164026751963));
#15076=CARTESIAN_POINT('Ctrl Pts',(-4.8506892701017,-11.6189842542419,-8.40164026751106));
#15077=CARTESIAN_POINT('Ctrl Pts',(-7.27603390513778,-11.443984254242,-4.20082013374683));
#15078=CARTESIAN_POINT('Ctrl Pts',(-9.70137854017372,-11.2689842542419,
1.69240902055491E-11));
#15079=CARTESIAN_POINT('Ctrl Pts',(-7.27603390512289,-11.0939842542419,
4.20082013377263));
#15080=CARTESIAN_POINT('Ctrl Pts',(-4.85068927007191,-10.918984254242,8.40164026752826));
#15081=CARTESIAN_POINT('Ctrl Pts',(1.46114046683977E-11,-10.7439842542419,
8.40164026751963));
#15082=CARTESIAN_POINT('Ctrl Pts',(4.85068927010161,-10.5689842542419,8.40164026751111));
#15083=CARTESIAN_POINT('Ctrl Pts',(7.27603390513774,-10.393984254242,4.20082013374691));
#15084=CARTESIAN_POINT('Ctrl Pts',(9.70137854017372,-10.2189842542419,-1.68195034686027E-11));
#15085=CARTESIAN_POINT('Ctrl Pts',(7.27603390512293,-10.0439842542419,-4.20082013377256));
#15086=CARTESIAN_POINT('Ctrl Pts',(4.850689270072,-9.86898425424196,-8.40164026752821));
#15087=CARTESIAN_POINT('Ctrl Pts',(-1.49984078541476E-11,-9.69398425424195,
-8.40164026751963));
#15088=CARTESIAN_POINT('Ctrl Pts',(-4.85068927010152,-9.51898425424195,
-8.40164026751116));
#15089=CARTESIAN_POINT('Ctrl Pts',(-7.27603390513769,-9.34398425424196,
-4.20082013374699));
#15090=CARTESIAN_POINT('Ctrl Pts',(-9.70137854017372,-9.16898425424195,
1.72663762555427E-11));
#15091=CARTESIAN_POINT('Ctrl Pts',(-7.27603390512298,-8.99398425424194,
4.20082013377248));
#15092=CARTESIAN_POINT('Ctrl Pts',(-4.85068927007209,-8.81898425424197,
8.40164026752815));
#15093=CARTESIAN_POINT('Ctrl Pts',(1.49078330830532E-11,-8.64398425424195,
8.40164026751963));
#15094=CARTESIAN_POINT('Ctrl Pts',(4.85068927010143,-8.46898425424195,8.40164026751122));
#15095=CARTESIAN_POINT('Ctrl Pts',(7.27603390513765,-8.29398425424196,4.20082013374707));
#15096=CARTESIAN_POINT('Ctrl Pts',(9.70137854017372,-8.11898425424196,-1.71617895185964E-11));
#15097=CARTESIAN_POINT('Ctrl Pts',(7.27603390512302,-7.94398425424195,-4.2008201337724));
#15098=CARTESIAN_POINT('Ctrl Pts',(4.85068927007219,-7.76898425424197,-8.4016402675281));
#15099=CARTESIAN_POINT('Ctrl Pts',(-1.48172583119587E-11,-7.59398425424196,
-8.40164026751963));
#15100=CARTESIAN_POINT('Ctrl Pts',(-4.85068927010182,-7.41898425424196,
-8.40164026751099));
#15101=CARTESIAN_POINT('Ctrl Pts',(-7.2760339051376,-7.24398425424194,-4.20082013374715));
#15102=CARTESIAN_POINT('Ctrl Pts',(-9.70137854017372,-7.06898425424196,
1.705720278165E-11));
#15103=CARTESIAN_POINT('Ctrl Pts',(-7.27603390512283,-6.89398425424195,
4.20082013377273));
#15104=CARTESIAN_POINT('Ctrl Pts',(-4.85068927007227,-6.71898425424195,
8.40164026752805));
#15105=CARTESIAN_POINT('Ctrl Pts',(1.47266835408643E-11,-6.54398425424196,
8.40164026751963));
#15106=CARTESIAN_POINT('Ctrl Pts',(4.85068927010173,-6.36898425424197,8.40164026751104));
#15107=CARTESIAN_POINT('Ctrl Pts',(7.27603390513756,-6.19398425424195,4.20082013374722));
#15108=CARTESIAN_POINT('Ctrl Pts',(9.70137854017372,-6.01898425424197,-1.69526160447037E-11));
#15109=CARTESIAN_POINT('Ctrl Pts',(7.27603390512287,-5.84398425424196,-4.20082013377265));
#15110=CARTESIAN_POINT('Ctrl Pts',(4.85068927007189,-5.66898425424195,-8.40164026752827));
#15111=CARTESIAN_POINT('Ctrl Pts',(-1.46361087697698E-11,-5.49398425424197,
-8.40164026751963));
#15112=CARTESIAN_POINT('Ctrl Pts',(-4.85068927010164,-5.31898425424197,
-8.40164026751109));
#15113=CARTESIAN_POINT('Ctrl Pts',(-7.27603390513775,-5.14398425424195,
-4.20082013374689));
#15114=CARTESIAN_POINT('Ctrl Pts',(-9.70137854017372,-4.96898425424197,
1.68480293077573E-11));
#15115=CARTESIAN_POINT('Ctrl Pts',(-7.27603390512292,-4.79398425424196,
4.20082013377258));
#15116=CARTESIAN_POINT('Ctrl Pts',(-4.85068927007198,-4.61898425424196,
8.40164026752822));
#15117=CARTESIAN_POINT('Ctrl Pts',(1.45455339986754E-11,-4.44398425424197,
8.40164026751963));
#15118=CARTESIAN_POINT('Ctrl Pts',(4.85068927010155,-4.26898425424197,8.40164026751115));
#15119=CARTESIAN_POINT('Ctrl Pts',(7.2760339051377,-4.09398425424196,4.20082013374697));
#15120=CARTESIAN_POINT('Ctrl Pts',(9.70137854017372,-3.91898425424198,-1.72949020946973E-11));
#15121=CARTESIAN_POINT('Ctrl Pts',(7.27603390512296,-3.74398425424197,-4.2008201337725));
#15122=CARTESIAN_POINT('Ctrl Pts',(4.85068927007207,-3.56898425424196,-8.40164026752817));
#15123=CARTESIAN_POINT('Ctrl Pts',(-1.49325371844254E-11,-3.39398425424198,
-8.40164026751963));
#15124=CARTESIAN_POINT('Ctrl Pts',(-4.85068927010146,-3.21898425424198,
-8.4016402675112));
#15125=CARTESIAN_POINT('Ctrl Pts',(-7.27603390513766,-3.04398425424196,
-4.20082013374705));
#15126=CARTESIAN_POINT('Ctrl Pts',(-9.70137854017372,-2.86898425424196,
1.7190315357751E-11));
#15127=CARTESIAN_POINT('Ctrl Pts',(-7.27603390512301,-2.69398425424197,
4.20082013377242));
#15128=CARTESIAN_POINT('Ctrl Pts',(-4.85068927007216,-2.51898425424197,
8.40164026752812));
#15129=CARTESIAN_POINT('Ctrl Pts',(1.48419624133309E-11,-2.34398425424195,
8.40164026751963));
#15130=CARTESIAN_POINT('Ctrl Pts',(4.85068927010137,-2.16898425424197,8.40164026751125));
#15131=CARTESIAN_POINT('Ctrl Pts',(7.27603390513761,-1.99398425424197,4.20082013374713));
#15132=CARTESIAN_POINT('Ctrl Pts',(9.70137854017372,-1.81898425424196,-1.70857286208046E-11));
#15133=CARTESIAN_POINT('Ctrl Pts',(7.27603390512282,-1.64398425424198,-4.20082013377275));
#15134=CARTESIAN_POINT('Ctrl Pts',(4.85068927007225,-1.46898425424197,-8.40164026752806));
#15135=CARTESIAN_POINT('Ctrl Pts',(-1.47513876422365E-11,-1.29398425424196,
-8.40164026751963));
#15136=CARTESIAN_POINT('Ctrl Pts',(-4.85068927010175,-1.11898425424198,
-8.40164026751103));
#15137=CARTESIAN_POINT('Ctrl Pts',(-7.27603390513757,-0.94398425424197,
-4.2008201337472));
#15138=CARTESIAN_POINT('Ctrl Pts',(-9.70137854017372,-0.768984254241965,
1.69811418838583E-11));
#15139=CARTESIAN_POINT('Ctrl Pts',(-7.27603390512286,-0.59398425424198,
4.20082013377267));
#15140=CARTESIAN_POINT('Ctrl Pts',(-4.85068927007234,-0.418984254241974,
8.40164026752801));
#15141=CARTESIAN_POINT('Ctrl Pts',(1.4660812871142E-11,-0.243984254241963,
8.40164026751963));
#15142=CARTESIAN_POINT('Ctrl Pts',(4.85068927010166,-0.068984254241984,
8.40164026751108));
#15143=CARTESIAN_POINT('Ctrl Pts',(7.27603390513776,0.106015745758026,4.20082013374687));
#15144=CARTESIAN_POINT('Ctrl Pts',(9.70137854017372,0.28101574575803,-1.6876555146912E-11));
#15145=CARTESIAN_POINT('Ctrl Pts',(7.27603390512291,0.456015745758015,-4.2008201337726));
#15146=CARTESIAN_POINT('Ctrl Pts',(4.85068927007195,0.631015745758021,-8.40164026752823));
#15147=CARTESIAN_POINT('Ctrl Pts',(-1.45702381000475E-11,0.806015745758032,
-8.40164026751963));
#15148=CARTESIAN_POINT('Ctrl Pts',(-4.85068927010157,0.981015745758011,
-8.40164026751113));
#15149=CARTESIAN_POINT('Ctrl Pts',(-7.27603390513772,1.15601574575802,-4.20082013374695));
#15150=CARTESIAN_POINT('Ctrl Pts',(-9.70137854017372,1.33101574575803,1.67719684099656E-11));
#15151=CARTESIAN_POINT('Ctrl Pts',(-7.27603390512295,1.50601574575804,4.20082013377252));
#15152=CARTESIAN_POINT('Ctrl Pts',(-4.85068927007204,1.68101574575802,8.40164026752818));
#15153=CARTESIAN_POINT('Ctrl Pts',(1.49572412857975E-11,1.85601574575803,
8.40164026751963));
#15154=CARTESIAN_POINT('Ctrl Pts',(4.85068927010148,2.03101574575803,8.40164026751119));
#15155=CARTESIAN_POINT('Ctrl Pts',(7.27603390513767,2.20601574575802,4.20082013374703));
#15156=CARTESIAN_POINT('Ctrl Pts',(9.70137854017372,2.38101574575802,-1.72188411969056E-11));
#15157=CARTESIAN_POINT('Ctrl Pts',(7.276033905123,2.55601574575803,-4.20082013377244));
#15158=CARTESIAN_POINT('Ctrl Pts',(4.85068927007213,2.73101574575801,-8.40164026752813));
#15159=CARTESIAN_POINT('Ctrl Pts',(-1.48666665147031E-11,2.90601574575802,
-8.40164026751963));
#15160=CARTESIAN_POINT('Ctrl Pts',(-4.85068927010139,3.08101574575803,-8.40164026751124));
#15161=CARTESIAN_POINT('Ctrl Pts',(-7.27603390513763,3.25601574575801,-4.2008201337471));
#15162=CARTESIAN_POINT('Ctrl Pts',(-9.70137854017372,3.43101574575802,1.71142544599593E-11));
#15163=CARTESIAN_POINT('Ctrl Pts',(-7.27603390512304,3.60601574575803,4.20082013377236));
#15164=CARTESIAN_POINT('Ctrl Pts',(-4.85068927007222,3.78101574575801,8.40164026752808));
#15165=CARTESIAN_POINT('Ctrl Pts',(1.47760917436086E-11,3.95601574575802,
8.40164026751963));
#15166=CARTESIAN_POINT('Ctrl Pts',(4.85068927010178,4.13101574575802,8.40164026751101));
#15167=CARTESIAN_POINT('Ctrl Pts',(7.27603390513758,4.30601574575801,4.20082013374718));
#15168=CARTESIAN_POINT('Ctrl Pts',(9.70137854017372,4.48101574575801,-1.70096677230129E-11));
#15169=CARTESIAN_POINT('Ctrl Pts',(7.27603390512285,4.65601574575802,-4.2008201337727));
#15170=CARTESIAN_POINT('Ctrl Pts',(4.85068927007232,4.831015745758,-8.40164026752803));
#15171=CARTESIAN_POINT('Ctrl Pts',(-1.46855169725142E-11,5.00601574575801,
-8.40164026751963));
#15172=CARTESIAN_POINT('Ctrl Pts',(-4.85068927010169,5.18101574575802,-8.40164026751107));
#15173=CARTESIAN_POINT('Ctrl Pts',(-7.27603390513754,5.356015745758,-4.20082013374726));
#15174=CARTESIAN_POINT('Ctrl Pts',(-9.70137854017372,5.53101574575801,1.69050809860666E-11));
#15175=CARTESIAN_POINT('Ctrl Pts',(-7.27603390512289,5.70601574575802,4.20082013377262));
#15176=CARTESIAN_POINT('Ctrl Pts',(-4.85068927007193,5.881015745758,8.40164026752825));
#15177=CARTESIAN_POINT('Ctrl Pts',(1.45949422014197E-11,6.05601574575801,
8.40164026751963));
#15178=CARTESIAN_POINT('Ctrl Pts',(4.8506892701016,6.23101574575801,8.40164026751112));
#15179=CARTESIAN_POINT('Ctrl Pts',(7.27603390513773,6.40601574575803,4.20082013374692));
#15180=CARTESIAN_POINT('Ctrl Pts',(9.70137854017372,6.581015745758,-1.68004942491202E-11));
#15181=CARTESIAN_POINT('Ctrl Pts',(7.27603390512294,6.75601574575802,-4.20082013377254));
#15182=CARTESIAN_POINT('Ctrl Pts',(4.85068927007202,6.93101574575802,-8.4016402675282));
#15183=CARTESIAN_POINT('Ctrl Pts',(-1.45043674303253E-11,7.106015745758,
-8.40164026751963));
#15184=CARTESIAN_POINT('Ctrl Pts',(-4.85068927010151,7.28101574575801,-8.40164026751117));
#15185=CARTESIAN_POINT('Ctrl Pts',(-7.27603390513768,7.45601574575802,-4.200820133747));
#15186=CARTESIAN_POINT('Ctrl Pts',(-9.70137854017372,7.631015745758,1.72473670360602E-11));
#15187=CARTESIAN_POINT('Ctrl Pts',(-7.27603390512298,7.80601574575801,4.20082013377246));
#15188=CARTESIAN_POINT('Ctrl Pts',(-4.85068927007211,7.98101574575801,8.40164026752814));
#15189=CARTESIAN_POINT('Ctrl Pts',(1.48913706160753E-11,8.156015745758,
8.40164026751963));
#15190=CARTESIAN_POINT('Ctrl Pts',(4.85068927010141,8.331015745758,8.40164026751122));
#15191=CARTESIAN_POINT('Ctrl Pts',(7.27603390513764,8.50601574575802,4.20082013374708));
#15192=CARTESIAN_POINT('Ctrl Pts',(9.70137854017372,8.68101574575799,-1.71427802991139E-11));
#15193=CARTESIAN_POINT('Ctrl Pts',(7.27603390512303,8.85601574575801,-4.20082013377238));
#15194=CARTESIAN_POINT('Ctrl Pts',(4.8506892700722,9.03101574575801,-8.40164026752809));
#15195=CARTESIAN_POINT('Ctrl Pts',(-1.48007958449808E-11,9.20601574575799,
-8.40164026751963));
#15196=CARTESIAN_POINT('Ctrl Pts',(-4.8506892701018,9.381015745758,-8.401640267511));
#15197=CARTESIAN_POINT('Ctrl Pts',(-7.27603390513759,9.55601574575801,-4.20082013374716));
#15198=CARTESIAN_POINT('Ctrl Pts',(-9.70137854017372,9.73101574575799,1.70381935621676E-11));
#15199=CARTESIAN_POINT('Ctrl Pts',(-7.27603390512284,9.906015745758,4.20082013377272));
#15200=CARTESIAN_POINT('Ctrl Pts',(-4.85068927007229,10.081015745758,8.40164026752804));
#15201=CARTESIAN_POINT('Ctrl Pts',(1.47102210738864E-11,10.256015745758,
8.40164026751963));
#15202=CARTESIAN_POINT('Ctrl Pts',(4.85068927010171,10.431015745758,8.40164026751105));
#15203=CARTESIAN_POINT('Ctrl Pts',(7.27603390513755,10.606015745758,4.20082013374724));
#15204=CARTESIAN_POINT('Ctrl Pts',(9.70137854017372,10.781015745758,-1.69336068252212E-11));
#15205=CARTESIAN_POINT('Ctrl Pts',(7.27603390512288,10.956015745758,-4.20082013377264));
#15206=CARTESIAN_POINT('Ctrl Pts',(4.85068927007238,11.131015745758,-8.40164026752799));
#15207=CARTESIAN_POINT('Ctrl Pts',(-1.46196463027919E-11,11.306015745758,
-8.40164026751963));
#15208=CARTESIAN_POINT('Ctrl Pts',(-4.85068927010162,11.481015745758,-8.40164026751111));
#15209=CARTESIAN_POINT('Ctrl Pts',(-7.27603390513774,11.656015745758,-4.2008201337469));
#15210=CARTESIAN_POINT('Ctrl Pts',(-9.70137854017372,11.831015745758,1.68290200882749E-11));
#15211=CARTESIAN_POINT('Ctrl Pts',(-7.27603390512293,12.006015745758,4.20082013377256));
#15212=CARTESIAN_POINT('Ctrl Pts',(-4.85068927007199,12.181015745758,8.40164026752821));
#15213=CARTESIAN_POINT('Ctrl Pts',(1.45290715316974E-11,12.356015745758,
8.40164026751963));
#15214=CARTESIAN_POINT('Ctrl Pts',(4.85068927010153,12.531015745758,8.40164026751116));
#15215=CARTESIAN_POINT('Ctrl Pts',(7.2760339051377,12.706015745758,4.20082013374698));
#15216=CARTESIAN_POINT('Ctrl Pts',(9.70137854017372,12.881015745758,-1.67244333513285E-11));
#15217=CARTESIAN_POINT('Ctrl Pts',(7.27603390512297,13.056015745758,-4.20082013377248));
#15218=CARTESIAN_POINT('Ctrl Pts',(4.85068927007208,13.231015745758,-8.40164026752816));
#15219=CARTESIAN_POINT('Ctrl Pts',(-1.49160747174474E-11,13.406015745758,
-8.40164026751963));
#15220=CARTESIAN_POINT('Ctrl Pts',(-4.85068927010144,13.581015745758,-8.40164026751121));
#15221=CARTESIAN_POINT('Ctrl Pts',(-7.27603390513765,13.756015745758,-4.20082013374706));
#15222=CARTESIAN_POINT('Ctrl Pts',(-9.70137854017372,13.931015745758,1.71713061382685E-11));
#15223=CARTESIAN_POINT('Ctrl Pts',(-7.27603390512302,14.106015745758,4.2008201337724));
#15224=CARTESIAN_POINT('Ctrl Pts',(-4.85068927007218,14.281015745758,8.40164026752811));
#15225=CARTESIAN_POINT('Ctrl Pts',(1.4825499946353E-11,14.456015745758,
8.40164026751963));
#15226=CARTESIAN_POINT('Ctrl Pts',(4.85068927010135,14.631015745758,8.40164026751126));
#15227=CARTESIAN_POINT('Ctrl Pts',(7.27603390513761,14.806015745758,4.20082013374714));
#15228=CARTESIAN_POINT('Ctrl Pts',(9.70137854017372,14.981015745758,-1.70667194013222E-11));
#15229=CARTESIAN_POINT('Ctrl Pts',(7.27603390512282,15.156015745758,-4.20082013377274));
#15230=CARTESIAN_POINT('Ctrl Pts',(4.85068927007227,15.331015745758,-8.40164026752806));
#15231=CARTESIAN_POINT('Ctrl Pts',(-1.47349251752585E-11,15.506015745758,
-8.40164026751963));
#15232=CARTESIAN_POINT('Ctrl Pts',(-4.85068927010174,15.681015745758,-8.40164026751104));
#15233=CARTESIAN_POINT('Ctrl Pts',(-7.27603390513756,15.856015745758,-4.20082013374722));
#15234=CARTESIAN_POINT('Ctrl Pts',(-9.70137854017372,16.031015745758,1.69621326643758E-11));
#15235=CARTESIAN_POINT('Ctrl Pts',(-7.27603390512287,16.206015745758,4.20082013377266));
#15236=CARTESIAN_POINT('Ctrl Pts',(-4.85068927007236,16.381015745758,8.401640267528));
#15237=CARTESIAN_POINT('Ctrl Pts',(1.46443504041641E-11,16.556015745758,
8.40164026751963));
#15238=CARTESIAN_POINT('Ctrl Pts',(4.85068927010165,16.731015745758,8.40164026751109));
#15239=CARTESIAN_POINT('Ctrl Pts',(7.27603390513752,16.906015745758,4.2008201337473));
#15240=CARTESIAN_POINT('Ctrl Pts',(9.70137854017372,17.081015745758,-1.68575459274295E-11));
#15241=CARTESIAN_POINT('Ctrl Pts',(7.27603390512292,17.256015745758,-4.20082013377258));
#15242=CARTESIAN_POINT('Ctrl Pts',(4.85068927007197,17.431015745758,-8.40164026752823));
#15243=CARTESIAN_POINT('Ctrl Pts',(-1.45537756330696E-11,17.606015745758,
-8.40164026751963));
#15244=CARTESIAN_POINT('Ctrl Pts',(-4.85068927010155,17.781015745758,-8.40164026751114));
#15245=CARTESIAN_POINT('Ctrl Pts',(-7.27603390513771,17.956015745758,-4.20082013374696));
#15246=CARTESIAN_POINT('Ctrl Pts',(-9.70137854017372,18.131015745758,1.67529591904832E-11));
#15247=CARTESIAN_POINT('Ctrl Pts',(-7.27603390512296,18.306015745758,4.2008201337725));
#15248=CARTESIAN_POINT('Ctrl Pts',(-4.85068927007206,18.481015745758,8.40164026752817));
#15249=CARTESIAN_POINT('Ctrl Pts',(1.44632008619752E-11,18.656015745758,
8.40164026751963));
#15250=CARTESIAN_POINT('Ctrl Pts',(4.85068927010146,18.831015745758,8.4016402675112));
#15251=CARTESIAN_POINT('Ctrl Pts',(7.27603390513766,19.006015745758,4.20082013374704));
#15252=CARTESIAN_POINT('Ctrl Pts',(9.70137854017372,19.181015745758,-1.71998319774232E-11));
#15253=CARTESIAN_POINT('Ctrl Pts',(7.27603390512301,19.356015745758,-4.20082013377243));
#15254=CARTESIAN_POINT('Ctrl Pts',(4.85068927007215,19.531015745758,-8.40164026752812));
#15255=CARTESIAN_POINT('Ctrl Pts',(-1.48502040477252E-11,19.706015745758,
-8.40164026751963));
#15256=CARTESIAN_POINT('Ctrl Pts',(-4.85068927010137,19.881015745758,-8.40164026751125));
#15257=CARTESIAN_POINT('Ctrl Pts',(-7.27603390513762,20.056015745758,-4.20082013374712));
#15258=CARTESIAN_POINT('Ctrl Pts',(-9.70137854017372,20.231015745758,1.70952452404768E-11));
#15259=CARTESIAN_POINT('Ctrl Pts',(-7.27603390512305,20.406015745758,4.20082013377235));
#15260=CARTESIAN_POINT('Ctrl Pts',(-4.85068927007224,20.581015745758,8.40164026752807));
#15261=CARTESIAN_POINT('Ctrl Pts',(1.47596292766307E-11,20.756015745758,
8.40164026751963));
#15262=CARTESIAN_POINT('Ctrl Pts',(4.85068927010176,20.931015745758,8.40164026751102));
#15263=CARTESIAN_POINT('Ctrl Pts',(7.27603390513757,21.106015745758,4.2008201337472));
#15264=CARTESIAN_POINT('Ctrl Pts',(9.70137854017372,21.281015745758,-1.69906585035305E-11));
#15265=CARTESIAN_POINT('Ctrl Pts',(7.27603390512286,21.456015745758,-4.20082013377268));
#15266=CARTESIAN_POINT('Ctrl Pts',(4.85068927007233,21.631015745758,-8.40164026752802));
#15267=CARTESIAN_POINT('Ctrl Pts',(-1.46690545055362E-11,21.806015745758,
-8.40164026751963));
#15268=CARTESIAN_POINT('Ctrl Pts',(-4.85068927010167,21.981015745758,-8.40164026751108));
#15269=CARTESIAN_POINT('Ctrl Pts',(-7.27603390513753,22.156015745758,-4.20082013374728));
#15270=CARTESIAN_POINT('Ctrl Pts',(-7.69929559114725,22.1865560631964,-3.46770938867822));
#15271=CARTESIAN_POINT('Ctrl Pts',(-7.96780251527898,22.22,-2.66489817109789));
#15272=CARTESIAN_POINT('Ctrl Pts',(5.8718173029053,-25.4,-8.00113003034161));
#15273=CARTESIAN_POINT('Ctrl Pts',(3.25092800548582,-25.2860389439906,-9.92453123332517));
#15274=CARTESIAN_POINT('Ctrl Pts',(-1.76294905048704E-11,-25.1867511126202,
-9.92453123331945));
#15275=CARTESIAN_POINT('Ctrl Pts',(-5.72993077915507,-25.0117511126202,
-9.9245312333095));
#15276=CARTESIAN_POINT('Ctrl Pts',(-8.59489616871545,-24.8367511126202,
-4.96226561664465));
#15277=CARTESIAN_POINT('Ctrl Pts',(-11.4598615582757,-24.6617511126202,
2.02950100528141E-11));
#15278=CARTESIAN_POINT('Ctrl Pts',(-8.59489616869816,-24.4867511126202,
4.9622656166746));
#15279=CARTESIAN_POINT('Ctrl Pts',(-5.72993077912048,-24.3117511126203,
9.92453123332946));
#15280=CARTESIAN_POINT('Ctrl Pts',(1.75224980467247E-11,-24.1367511126202,
9.92453123331945));
#15281=CARTESIAN_POINT('Ctrl Pts',(5.72993077915496,-23.9617511126202,9.92453123330956));
#15282=CARTESIAN_POINT('Ctrl Pts',(8.5948961687154,-23.7867511126202,4.96226561664474));
#15283=CARTESIAN_POINT('Ctrl Pts',(11.4598615582757,-23.6117511126202,-2.01714658037908E-11));
#15284=CARTESIAN_POINT('Ctrl Pts',(8.59489616869793,-23.4367511126202,-4.962265616675));
#15285=CARTESIAN_POINT('Ctrl Pts',(5.72993077912059,-23.2617511126202,-9.9245312333294));
#15286=CARTESIAN_POINT('Ctrl Pts',(-1.74155055885791E-11,-23.0867511126202,
-9.92453123331945));
#15287=CARTESIAN_POINT('Ctrl Pts',(-5.72993077915542,-22.9117511126202,
-9.92453123330929));
#15288=CARTESIAN_POINT('Ctrl Pts',(-8.59489616871534,-22.7367511126202,
-4.96226561664484));
#15289=CARTESIAN_POINT('Ctrl Pts',(-11.4598615582757,-22.5617511126202,
2.00479215547674E-11));
#15290=CARTESIAN_POINT('Ctrl Pts',(-8.59489616869798,-22.3867511126202,
4.96226561667491));
#15291=CARTESIAN_POINT('Ctrl Pts',(-5.72993077912069,-22.2117511126202,
9.92453123332934));
#15292=CARTESIAN_POINT('Ctrl Pts',(1.73085131304334E-11,-22.0367511126202,
9.92453123331945));
#15293=CARTESIAN_POINT('Ctrl Pts',(5.72993077915531,-21.8617511126203,9.92453123330936));
#15294=CARTESIAN_POINT('Ctrl Pts',(8.59489616871557,-21.6867511126202,4.96226561664444));
#15295=CARTESIAN_POINT('Ctrl Pts',(11.4598615582757,-21.5117511126203,-1.99243773057441E-11));
#15296=CARTESIAN_POINT('Ctrl Pts',(8.59489616869803,-21.3367511126203,-4.96226561667481));
#15297=CARTESIAN_POINT('Ctrl Pts',(5.72993077912024,-21.1617511126202,-9.92453123332961));
#15298=CARTESIAN_POINT('Ctrl Pts',(-1.72015206722877E-11,-20.9867511126202,
-9.92453123331945));
#15299=CARTESIAN_POINT('Ctrl Pts',(-5.7299307791552,-20.8117511126203,-9.92453123330942));
#15300=CARTESIAN_POINT('Ctrl Pts',(-8.59489616871552,-20.6367511126202,
-4.96226561664453));
#15301=CARTESIAN_POINT('Ctrl Pts',(-11.4598615582757,-20.4617511126203,
1.98008330567208E-11));
#15302=CARTESIAN_POINT('Ctrl Pts',(-8.59489616869809,-20.2867511126202,
4.96226561667472));
#15303=CARTESIAN_POINT('Ctrl Pts',(-5.72993077912034,-20.1117511126202,
9.92453123332955));
#15304=CARTESIAN_POINT('Ctrl Pts',(1.7094528214142E-11,-19.9367511126203,
9.92453123331945));
#15305=CARTESIAN_POINT('Ctrl Pts',(5.7299307791551,-19.7617511126202,9.92453123330948));
#15306=CARTESIAN_POINT('Ctrl Pts',(8.59489616871547,-19.5867511126202,4.96226561664462));
#15307=CARTESIAN_POINT('Ctrl Pts',(11.4598615582757,-19.4117511126203,-2.03287065183413E-11));
#15308=CARTESIAN_POINT('Ctrl Pts',(8.59489616869814,-19.2367511126202,-4.96226561667463));
#15309=CARTESIAN_POINT('Ctrl Pts',(5.72993077912045,-19.0617511126202,-9.92453123332948));
#15310=CARTESIAN_POINT('Ctrl Pts',(-1.75516800418891E-11,-18.8867511126203,
-9.92453123331945));
#15311=CARTESIAN_POINT('Ctrl Pts',(-5.72993077915499,-18.7117511126202,
-9.92453123330954));
#15312=CARTESIAN_POINT('Ctrl Pts',(-8.59489616871541,-18.5367511126203,
-4.96226561664472));
#15313=CARTESIAN_POINT('Ctrl Pts',(-11.4598615582757,-18.3617511126203,
2.0205162269318E-11));
#15314=CARTESIAN_POINT('Ctrl Pts',(-8.5948961686982,-18.1867511126202,4.96226561667454));
#15315=CARTESIAN_POINT('Ctrl Pts',(-5.72993077912056,-18.0117511126203,
9.92453123332942));
#15316=CARTESIAN_POINT('Ctrl Pts',(1.74446875837434E-11,-17.8367511126202,
9.92453123331945));
#15317=CARTESIAN_POINT('Ctrl Pts',(5.72993077915545,-17.6617511126203,9.92453123330928));
#15318=CARTESIAN_POINT('Ctrl Pts',(8.59489616871536,-17.4867511126202,4.96226561664481));
#15319=CARTESIAN_POINT('Ctrl Pts',(11.4598615582757,-17.3117511126203,-2.00816180202947E-11));
#15320=CARTESIAN_POINT('Ctrl Pts',(8.59489616869797,-17.1367511126203,-4.96226561667493));
#15321=CARTESIAN_POINT('Ctrl Pts',(5.72993077912066,-16.9617511126202,-9.92453123332936));
#15322=CARTESIAN_POINT('Ctrl Pts',(-1.73376951255977E-11,-16.7867511126203,
-9.92453123331945));
#15323=CARTESIAN_POINT('Ctrl Pts',(-5.72993077915534,-16.6117511126203,
-9.92453123330934));
#15324=CARTESIAN_POINT('Ctrl Pts',(-8.59489616871531,-16.4367511126202,
-4.9622656166449));
#15325=CARTESIAN_POINT('Ctrl Pts',(-11.4598615582757,-16.2617511126203,
1.99580737712713E-11));
#15326=CARTESIAN_POINT('Ctrl Pts',(-8.59489616869802,-16.0867511126203,
4.96226561667484));
#15327=CARTESIAN_POINT('Ctrl Pts',(-5.72993077912021,-15.9117511126202,
9.92453123332962));
#15328=CARTESIAN_POINT('Ctrl Pts',(1.7230702667452E-11,-15.7367511126203,
9.92453123331945));
#15329=CARTESIAN_POINT('Ctrl Pts',(5.72993077915523,-15.5617511126203,9.9245312333094));
#15330=CARTESIAN_POINT('Ctrl Pts',(8.59489616871553,-15.3867511126203,4.96226561664451));
#15331=CARTESIAN_POINT('Ctrl Pts',(11.4598615582757,-15.2117511126203,-1.9834529522248E-11));
#15332=CARTESIAN_POINT('Ctrl Pts',(8.59489616869807,-15.0367511126203,-4.96226561667475));
#15333=CARTESIAN_POINT('Ctrl Pts',(5.72993077912031,-14.8617511126203,-9.92453123332956));
#15334=CARTESIAN_POINT('Ctrl Pts',(-1.71237102093063E-11,-14.6867511126202,
-9.92453123331945));
#15335=CARTESIAN_POINT('Ctrl Pts',(-5.72993077915512,-14.5117511126203,
-9.92453123330946));
#15336=CARTESIAN_POINT('Ctrl Pts',(-8.59489616871548,-14.3367511126203,
-4.9622656166446));
#15337=CARTESIAN_POINT('Ctrl Pts',(-11.4598615582757,-14.1617511126203,
1.97109852732247E-11));
#15338=CARTESIAN_POINT('Ctrl Pts',(-8.59489616869813,-13.9867511126203,
4.96226561667465));
#15339=CARTESIAN_POINT('Ctrl Pts',(-5.72993077912042,-13.8117511126203,
9.9245312333295));
#15340=CARTESIAN_POINT('Ctrl Pts',(1.75808620370534E-11,-13.6367511126203,
9.92453123331945));
#15341=CARTESIAN_POINT('Ctrl Pts',(5.72993077915502,-13.4617511126203,9.92453123330952));
#15342=CARTESIAN_POINT('Ctrl Pts',(8.59489616871543,-13.2867511126203,4.96226561664469));
#15343=CARTESIAN_POINT('Ctrl Pts',(11.4598615582757,-13.1117511126203,-2.02388587348453E-11));
#15344=CARTESIAN_POINT('Ctrl Pts',(8.59489616869818,-12.9367511126203,-4.96226561667456));
#15345=CARTESIAN_POINT('Ctrl Pts',(5.72993077912053,-12.7617511126203,-9.92453123332944));
#15346=CARTESIAN_POINT('Ctrl Pts',(-1.74738695789077E-11,-12.5867511126203,
-9.92453123331945));
#15347=CARTESIAN_POINT('Ctrl Pts',(-5.72993077915491,-12.4117511126203,
-9.92453123330959));
#15348=CARTESIAN_POINT('Ctrl Pts',(-8.59489616871537,-12.2367511126203,
-4.96226561664478));
#15349=CARTESIAN_POINT('Ctrl Pts',(-11.4598615582757,-12.0617511126203,
2.01153144858219E-11));
#15350=CARTESIAN_POINT('Ctrl Pts',(-8.59489616869795,-11.8867511126203,
4.96226561667496));
#15351=CARTESIAN_POINT('Ctrl Pts',(-5.72993077912063,-11.7117511126203,
9.92453123332938));
#15352=CARTESIAN_POINT('Ctrl Pts',(1.7366877120762E-11,-11.5367511126203,
9.92453123331945));
#15353=CARTESIAN_POINT('Ctrl Pts',(5.72993077915537,-11.3617511126203,9.92453123330932));
#15354=CARTESIAN_POINT('Ctrl Pts',(8.59489616871532,-11.1867511126203,4.96226561664488));
#15355=CARTESIAN_POINT('Ctrl Pts',(11.4598615582757,-11.0117511126203,-1.99917702367986E-11));
#15356=CARTESIAN_POINT('Ctrl Pts',(8.59489616869801,-10.8367511126203,-4.96226561667487));
#15357=CARTESIAN_POINT('Ctrl Pts',(5.72993077912074,-10.6617511126203,-9.92453123332931));
#15358=CARTESIAN_POINT('Ctrl Pts',(-1.72598846626164E-11,-10.4867511126203,
-9.92453123331945));
#15359=CARTESIAN_POINT('Ctrl Pts',(-5.72993077915526,-10.3117511126203,
-9.92453123330938));
#15360=CARTESIAN_POINT('Ctrl Pts',(-8.59489616871555,-10.1367511126203,
-4.96226561664448));
#15361=CARTESIAN_POINT('Ctrl Pts',(-11.4598615582757,-9.96175111262027,
1.98682259877752E-11));
#15362=CARTESIAN_POINT('Ctrl Pts',(-8.59489616869806,-9.78675111262026,
4.96226561667477));
#15363=CARTESIAN_POINT('Ctrl Pts',(-5.72993077912029,-9.61175111262028,
9.92453123332958));
#15364=CARTESIAN_POINT('Ctrl Pts',(1.71528922044707E-11,-9.43675111262027,
9.92453123331945));
#15365=CARTESIAN_POINT('Ctrl Pts',(5.72993077915515,-9.26175111262026,9.92453123330944));
#15366=CARTESIAN_POINT('Ctrl Pts',(8.59489616871549,-9.08675111262028,4.96226561664457));
#15367=CARTESIAN_POINT('Ctrl Pts',(11.4598615582757,-8.91175111262028,-1.97446817387519E-11));
#15368=CARTESIAN_POINT('Ctrl Pts',(8.59489616869811,-8.73675111262026,-4.96226561667468));
#15369=CARTESIAN_POINT('Ctrl Pts',(5.72993077912039,-8.56175111262028,-9.92453123332952));
#15370=CARTESIAN_POINT('Ctrl Pts',(-1.76100440322177E-11,-8.38675111262027,
-9.92453123331945));
#15371=CARTESIAN_POINT('Ctrl Pts',(-5.72993077915505,-8.21175111262026,
-9.92453123330951));
#15372=CARTESIAN_POINT('Ctrl Pts',(-8.59489616871544,-8.03675111262028,
-4.96226561664467));
#15373=CARTESIAN_POINT('Ctrl Pts',(-11.4598615582757,-7.86175111262028,
2.02725552003725E-11));
#15374=CARTESIAN_POINT('Ctrl Pts',(-8.59489616869817,-7.68675111262027,
4.96226561667459));
#15375=CARTESIAN_POINT('Ctrl Pts',(-5.7299307791205,-7.51175111262028,9.92453123332946));
#15376=CARTESIAN_POINT('Ctrl Pts',(1.75030515740721E-11,-7.33675111262028,
9.92453123331945));
#15377=CARTESIAN_POINT('Ctrl Pts',(5.72993077915494,-7.16175111262027,9.92453123330957));
#15378=CARTESIAN_POINT('Ctrl Pts',(8.59489616871539,-6.98675111262029,4.96226561664476));
#15379=CARTESIAN_POINT('Ctrl Pts',(11.4598615582757,-6.81175111262029,-2.01490109513492E-11));
#15380=CARTESIAN_POINT('Ctrl Pts',(8.59489616869822,-6.63675111262027,-4.96226561667449));
#15381=CARTESIAN_POINT('Ctrl Pts',(5.72993077912061,-6.46175111262029,-9.92453123332939));
#15382=CARTESIAN_POINT('Ctrl Pts',(-1.73960591159264E-11,-6.28675111262028,
-9.92453123331945));
#15383=CARTESIAN_POINT('Ctrl Pts',(-5.7299307791554,-6.11175111262027,-9.92453123330931));
#15384=CARTESIAN_POINT('Ctrl Pts',(-8.59489616871534,-5.93675111262026,
-4.96226561664485));
#15385=CARTESIAN_POINT('Ctrl Pts',(-11.4598615582757,-5.76175111262029,
2.00254667023258E-11));
#15386=CARTESIAN_POINT('Ctrl Pts',(-8.59489616869799,-5.58675111262028,
4.96226561667489));
#15387=CARTESIAN_POINT('Ctrl Pts',(-5.72993077912071,-5.41175111262028,
9.92453123332933));
#15388=CARTESIAN_POINT('Ctrl Pts',(1.72890666577807E-11,-5.23675111262029,
9.92453123331945));
#15389=CARTESIAN_POINT('Ctrl Pts',(5.72993077915529,-5.06175111262028,9.92453123330937));
#15390=CARTESIAN_POINT('Ctrl Pts',(8.59489616871528,-4.88675111262027,4.96226561664494));
#15391=CARTESIAN_POINT('Ctrl Pts',(11.4598615582757,-4.7117511126203,-1.99019224533025E-11));
#15392=CARTESIAN_POINT('Ctrl Pts',(8.59489616869805,-4.53675111262028,-4.9622656166748));
#15393=CARTESIAN_POINT('Ctrl Pts',(5.72993077912025,-4.36175111262028,-9.9245312333296));
#15394=CARTESIAN_POINT('Ctrl Pts',(-1.7182074199635E-11,-4.18675111262029,
-9.92453123331945));
#15395=CARTESIAN_POINT('Ctrl Pts',(-5.72993077915518,-4.01175111262028,
-9.92453123330943));
#15396=CARTESIAN_POINT('Ctrl Pts',(-8.59489616871551,-3.83675111262027,
-4.96226561664455));
#15397=CARTESIAN_POINT('Ctrl Pts',(-11.4598615582757,-3.6617511126203,1.97783782042791E-11));
#15398=CARTESIAN_POINT('Ctrl Pts',(-8.5948961686981,-3.48675111262029,4.9622656166747));
#15399=CARTESIAN_POINT('Ctrl Pts',(-5.72993077912036,-3.31175111262029,
9.92453123332954));
#15400=CARTESIAN_POINT('Ctrl Pts',(1.70750817414893E-11,-3.1367511126203,
9.92453123331945));
#15401=CARTESIAN_POINT('Ctrl Pts',(5.72993077915508,-2.96175111262029,9.92453123330949));
#15402=CARTESIAN_POINT('Ctrl Pts',(8.59489616871546,-2.78675111262028,4.96226561664464));
#15403=CARTESIAN_POINT('Ctrl Pts',(11.4598615582757,-2.61175111262031,-2.03062516658997E-11));
#15404=CARTESIAN_POINT('Ctrl Pts',(8.59489616869815,-2.43675111262029,-4.96226561667461));
#15405=CARTESIAN_POINT('Ctrl Pts',(5.72993077912047,-2.26175111262028,-9.92453123332947));
#15406=CARTESIAN_POINT('Ctrl Pts',(-1.75322335692364E-11,-2.0867511126203,
-9.92453123331945));
#15407=CARTESIAN_POINT('Ctrl Pts',(-5.72993077915497,-1.91175111262029,
-9.92453123330955));
#15408=CARTESIAN_POINT('Ctrl Pts',(-8.5948961687154,-1.73675111262028,-4.96226561664473));
#15409=CARTESIAN_POINT('Ctrl Pts',(-11.4598615582757,-1.56175111262028,
2.01827074168764E-11));
#15410=CARTESIAN_POINT('Ctrl Pts',(-8.59489616869821,-1.38675111262029,
4.96226561667452));
#15411=CARTESIAN_POINT('Ctrl Pts',(-5.72993077912058,-1.21175111262029,
9.92453123332941));
#15412=CARTESIAN_POINT('Ctrl Pts',(1.74252411110907E-11,-1.03675111262028,
9.92453123331945));
#15413=CARTESIAN_POINT('Ctrl Pts',(5.72993077915486,-0.861751112620297,
9.92453123330961));
#15414=CARTESIAN_POINT('Ctrl Pts',(8.59489616871535,-0.686751112620287,
4.96226561664483));
#15415=CARTESIAN_POINT('Ctrl Pts',(11.4598615582757,-0.511751112620282,
-2.0059163167853E-11));
#15416=CARTESIAN_POINT('Ctrl Pts',(8.59489616869798,-0.336751112620298,
-4.96226561667492));
#15417=CARTESIAN_POINT('Ctrl Pts',(5.72993077912068,-0.161751112620292,
-9.92453123332935));
#15418=CARTESIAN_POINT('Ctrl Pts',(-1.7318248652945E-11,0.0132488873797187,
-9.92453123331945));
#15419=CARTESIAN_POINT('Ctrl Pts',(-5.72993077915532,0.188248887379698,
-9.92453123330935));
#15420=CARTESIAN_POINT('Ctrl Pts',(-8.59489616871529,0.363248887379708,
-4.96226561664492));
#15421=CARTESIAN_POINT('Ctrl Pts',(-11.4598615582757,0.538248887379713,
1.99356189188297E-11));
#15422=CARTESIAN_POINT('Ctrl Pts',(-8.59489616869803,0.713248887379697,
4.96226561667482));
#15423=CARTESIAN_POINT('Ctrl Pts',(-5.72993077912079,0.888248887379703,
9.92453123332929));
#15424=CARTESIAN_POINT('Ctrl Pts',(1.72112561947994E-11,1.06324888737971,
9.92453123331945));
#15425=CARTESIAN_POINT('Ctrl Pts',(5.72993077915521,1.23824888737969,9.92453123330941));
#15426=CARTESIAN_POINT('Ctrl Pts',(8.59489616871553,1.4132488873797,4.96226561664452));
#15427=CARTESIAN_POINT('Ctrl Pts',(11.4598615582757,1.58824888737971,-1.98120746698064E-11));
#15428=CARTESIAN_POINT('Ctrl Pts',(8.59489616869808,1.76324888737969,-4.96226561667473));
#15429=CARTESIAN_POINT('Ctrl Pts',(5.72993077912033,1.9382488873797,-9.92453123332955));
#15430=CARTESIAN_POINT('Ctrl Pts',(-1.71042637366537E-11,2.11324888737971,
-9.92453123331945));
#15431=CARTESIAN_POINT('Ctrl Pts',(-5.72993077915511,2.28824888737969,-9.92453123330947));
#15432=CARTESIAN_POINT('Ctrl Pts',(-8.59489616871547,2.4632488873797,-4.96226561664462));
#15433=CARTESIAN_POINT('Ctrl Pts',(-11.4598615582757,2.6382488873797,1.9688530420783E-11));
#15434=CARTESIAN_POINT('Ctrl Pts',(-8.59489616869814,2.81324888737972,4.96226561667464));
#15435=CARTESIAN_POINT('Ctrl Pts',(-5.72993077912044,2.98824888737969,9.92453123332949));
#15436=CARTESIAN_POINT('Ctrl Pts',(1.75614155644007E-11,3.16324888737971,
9.92453123331945));
#15437=CARTESIAN_POINT('Ctrl Pts',(5.729930779155,3.33824888737971,9.92453123330953));
#15438=CARTESIAN_POINT('Ctrl Pts',(8.59489616871542,3.51324888737969,4.96226561664471));
#15439=CARTESIAN_POINT('Ctrl Pts',(11.4598615582757,3.6882488873797,-2.02164038824036E-11));
#15440=CARTESIAN_POINT('Ctrl Pts',(8.59489616869819,3.86324888737971,-4.96226561667455));
#15441=CARTESIAN_POINT('Ctrl Pts',(5.72993077912055,4.03824888737969,-9.92453123332943));
#15442=CARTESIAN_POINT('Ctrl Pts',(-1.74544231062551E-11,4.2132488873797,
-9.92453123331945));
#15443=CARTESIAN_POINT('Ctrl Pts',(-5.72993077915489,4.3882488873797,-9.9245312333096));
#15444=CARTESIAN_POINT('Ctrl Pts',(-8.59489616871537,4.56324888737969,-4.9622656166448));
#15445=CARTESIAN_POINT('Ctrl Pts',(-11.4598615582757,4.73824888737969,2.00928596333803E-11));
#15446=CARTESIAN_POINT('Ctrl Pts',(-8.59489616869824,4.91324888737971,4.96226561667445));
#15447=CARTESIAN_POINT('Ctrl Pts',(-5.72993077912065,5.08824888737968,9.92453123332936));
#15448=CARTESIAN_POINT('Ctrl Pts',(1.73474306481094E-11,5.2632488873797,
9.92453123331945));
#15449=CARTESIAN_POINT('Ctrl Pts',(5.72993077915535,5.4382488873797,9.92453123330933));
#15450=CARTESIAN_POINT('Ctrl Pts',(8.59489616871531,5.61324888737968,4.96226561664489));
#15451=CARTESIAN_POINT('Ctrl Pts',(11.4598615582757,5.78824888737969,-1.9969315384357E-11));
#15452=CARTESIAN_POINT('Ctrl Pts',(8.59489616869802,5.9632488873797,-4.96226561667485));
#15453=CARTESIAN_POINT('Ctrl Pts',(5.72993077912076,6.13824888737968,-9.9245312333293));
#15454=CARTESIAN_POINT('Ctrl Pts',(-1.72404381899637E-11,6.31324888737969,
-9.92453123331945));
#15455=CARTESIAN_POINT('Ctrl Pts',(-5.72993077915524,6.4882488873797,-9.92453123330939));
#15456=CARTESIAN_POINT('Ctrl Pts',(-8.59489616871526,6.66324888737968,-4.96226561664499));
#15457=CARTESIAN_POINT('Ctrl Pts',(-11.4598615582757,6.83824888737969,1.98457711353336E-11));
#15458=CARTESIAN_POINT('Ctrl Pts',(-8.59489616869807,7.0132488873797,4.96226561667476));
#15459=CARTESIAN_POINT('Ctrl Pts',(-5.7299307791203,7.18824888737968,9.92453123332957));
#15460=CARTESIAN_POINT('Ctrl Pts',(1.7133445731818E-11,7.36324888737969,
9.92453123331945));
#15461=CARTESIAN_POINT('Ctrl Pts',(5.72993077915513,7.53824888737969,9.92453123330946));
#15462=CARTESIAN_POINT('Ctrl Pts',(8.59489616871549,7.7132488873797,4.96226561664459));
#15463=CARTESIAN_POINT('Ctrl Pts',(11.4598615582757,7.88824888737968,-1.97222268863103E-11));
#15464=CARTESIAN_POINT('Ctrl Pts',(8.59489616869812,8.06324888737969,-4.96226561667466));
#15465=CARTESIAN_POINT('Ctrl Pts',(5.72993077912041,8.2382488873797,-9.92453123332951));
#15466=CARTESIAN_POINT('Ctrl Pts',(-1.70264532736723E-11,8.41324888737968,
-9.92453123331945));
#15467=CARTESIAN_POINT('Ctrl Pts',(-5.72993077915503,8.58824888737968,-9.92453123330952));
#15468=CARTESIAN_POINT('Ctrl Pts',(-8.59489616871543,8.7632488873797,-4.96226561664468));
#15469=CARTESIAN_POINT('Ctrl Pts',(-11.4598615582757,8.93824888737968,2.02501003479309E-11));
#15470=CARTESIAN_POINT('Ctrl Pts',(-8.59489616869817,9.11324888737969,4.96226561667457));
#15471=CARTESIAN_POINT('Ctrl Pts',(-5.72993077912052,9.28824888737969,9.92453123332944));
#15472=CARTESIAN_POINT('Ctrl Pts',(1.74836051014194E-11,9.46324888737968,
9.92453123331945));
#15473=CARTESIAN_POINT('Ctrl Pts',(5.72993077915492,9.63824888737968,9.92453123330958));
#15474=CARTESIAN_POINT('Ctrl Pts',(8.59489616871538,9.81324888737969,4.96226561664478));
#15475=CARTESIAN_POINT('Ctrl Pts',(11.4598615582757,9.98824888737967,-2.01265560989075E-11));
#15476=CARTESIAN_POINT('Ctrl Pts',(8.59489616869823,10.1632488873797,-4.96226561667448));
#15477=CARTESIAN_POINT('Ctrl Pts',(5.72993077912063,10.3382488873797,-9.92453123332938));
#15478=CARTESIAN_POINT('Ctrl Pts',(-1.73766126432737E-11,10.5132488873797,
-9.92453123331945));
#15479=CARTESIAN_POINT('Ctrl Pts',(-5.72993077915538,10.6882488873797,-9.92453123330931));
#15480=CARTESIAN_POINT('Ctrl Pts',(-8.59489616871532,10.8632488873797,-4.96226561664487));
#15481=CARTESIAN_POINT('Ctrl Pts',(-11.4598615582757,11.0382488873797,2.00030118498842E-11));
#15482=CARTESIAN_POINT('Ctrl Pts',(-8.594896168698,11.2132488873797,4.96226561667487));
#15483=CARTESIAN_POINT('Ctrl Pts',(-5.72993077912073,11.3882488873797,9.92453123332932));
#15484=CARTESIAN_POINT('Ctrl Pts',(1.7269620185128E-11,11.5632488873797,
9.92453123331945));
#15485=CARTESIAN_POINT('Ctrl Pts',(5.72993077915527,11.7382488873797,9.92453123330938));
#15486=CARTESIAN_POINT('Ctrl Pts',(8.59489616871527,11.9132488873797,4.96226561664496));
#15487=CARTESIAN_POINT('Ctrl Pts',(11.4598615582757,12.0882488873797,-1.98794676008609E-11));
#15488=CARTESIAN_POINT('Ctrl Pts',(8.59489616869805,12.2632488873797,-4.96226561667478));
#15489=CARTESIAN_POINT('Ctrl Pts',(5.72993077912084,12.4382488873797,-9.92453123332926));
#15490=CARTESIAN_POINT('Ctrl Pts',(-1.71626277269823E-11,12.6132488873797,
-9.92453123331945));
#15491=CARTESIAN_POINT('Ctrl Pts',(-5.72993077915516,12.7882488873797,-9.92453123330944));
#15492=CARTESIAN_POINT('Ctrl Pts',(-8.5948961687155,12.9632488873797,-4.96226561664457));
#15493=CARTESIAN_POINT('Ctrl Pts',(-11.4598615582757,13.1382488873797,1.97559233518375E-11));
#15494=CARTESIAN_POINT('Ctrl Pts',(-8.59489616869811,13.3132488873797,4.96226561667469));
#15495=CARTESIAN_POINT('Ctrl Pts',(-5.72993077912038,13.4882488873797,9.92453123332952));
#15496=CARTESIAN_POINT('Ctrl Pts',(1.70556352688367E-11,13.6632488873797,
9.92453123331945));
#15497=CARTESIAN_POINT('Ctrl Pts',(5.72993077915506,13.8382488873797,9.9245312333095));
#15498=CARTESIAN_POINT('Ctrl Pts',(8.59489616871545,14.0132488873797,4.96226561664466));
#15499=CARTESIAN_POINT('Ctrl Pts',(11.4598615582757,14.1882488873797,-1.96323791028142E-11));
#15500=CARTESIAN_POINT('Ctrl Pts',(8.59489616869816,14.3632488873797,-4.96226561667459));
#15501=CARTESIAN_POINT('Ctrl Pts',(5.72993077912049,14.5382488873797,-9.92453123332946));
#15502=CARTESIAN_POINT('Ctrl Pts',(-1.75127870965837E-11,14.7132488873797,
-9.92453123331945));
#15503=CARTESIAN_POINT('Ctrl Pts',(-5.72993077915495,14.8882488873797,-9.92453123330957));
#15504=CARTESIAN_POINT('Ctrl Pts',(-8.59489616871539,15.0632488873797,-4.96226561664475));
#15505=CARTESIAN_POINT('Ctrl Pts',(-11.4598615582757,15.2382488873797,2.01602525644348E-11));
#15506=CARTESIAN_POINT('Ctrl Pts',(-8.59489616869821,15.4132488873797,4.9622656166745));
#15507=CARTESIAN_POINT('Ctrl Pts',(-5.7299307791206,15.5882488873797,9.9245312333294));
#15508=CARTESIAN_POINT('Ctrl Pts',(1.7405794638438E-11,15.7632488873797,
9.92453123331945));
#15509=CARTESIAN_POINT('Ctrl Pts',(5.72993077915484,15.9382488873797,9.92453123330963));
#15510=CARTESIAN_POINT('Ctrl Pts',(8.59489616871534,16.1132488873797,4.96226561664484));
#15511=CARTESIAN_POINT('Ctrl Pts',(11.4598615582757,16.2882488873797,-2.00367083154114E-11));
#15512=CARTESIAN_POINT('Ctrl Pts',(8.59489616869799,16.4632488873797,-4.9622656166749));
#15513=CARTESIAN_POINT('Ctrl Pts',(5.7299307791207,16.6382488873797,-9.92453123332934));
#15514=CARTESIAN_POINT('Ctrl Pts',(-1.72988021802924E-11,16.8132488873797,
-9.92453123331945));
#15515=CARTESIAN_POINT('Ctrl Pts',(-5.7299307791553,16.9882488873797,-9.92453123330936));
#15516=CARTESIAN_POINT('Ctrl Pts',(-8.59489616871529,17.1632488873797,-4.96226561664494));
#15517=CARTESIAN_POINT('Ctrl Pts',(-11.4598615582757,17.3382488873797,1.99131640663881E-11));
#15518=CARTESIAN_POINT('Ctrl Pts',(-8.59489616869804,17.5132488873797,4.96226561667481));
#15519=CARTESIAN_POINT('Ctrl Pts',(-5.72993077912081,17.6882488873797,9.92453123332928));
#15520=CARTESIAN_POINT('Ctrl Pts',(1.71918097221467E-11,17.8632488873797,
9.92453123331945));
#15521=CARTESIAN_POINT('Ctrl Pts',(5.72993077915519,18.0382488873797,9.92453123330942));
#15522=CARTESIAN_POINT('Ctrl Pts',(8.59489616871523,18.2132488873797,4.96226561664503));
#15523=CARTESIAN_POINT('Ctrl Pts',(11.4598615582757,18.3882488873797,-1.97896198173647E-11));
#15524=CARTESIAN_POINT('Ctrl Pts',(8.59489616869809,18.5632488873797,-4.96226561667471));
#15525=CARTESIAN_POINT('Ctrl Pts',(5.72993077912035,18.7382488873796,-9.92453123332954));
#15526=CARTESIAN_POINT('Ctrl Pts',(-1.7084817264001E-11,18.9132488873797,
-9.92453123331945));
#15527=CARTESIAN_POINT('Ctrl Pts',(-5.72993077915509,19.0882488873797,-9.92453123330948));
#15528=CARTESIAN_POINT('Ctrl Pts',(-8.59489616871546,19.2632488873797,-4.96226561664463));
#15529=CARTESIAN_POINT('Ctrl Pts',(-11.4598615582757,19.4382488873797,1.96660755683414E-11));
#15530=CARTESIAN_POINT('Ctrl Pts',(-8.59489616869815,19.6132488873797,4.96226561667462));
#15531=CARTESIAN_POINT('Ctrl Pts',(-5.72993077912046,19.7882488873796,9.92453123332948));
#15532=CARTESIAN_POINT('Ctrl Pts',(1.69778248058553E-11,19.9632488873797,
9.92453123331945));
#15533=CARTESIAN_POINT('Ctrl Pts',(5.72993077915498,20.1382488873797,9.92453123330955));
#15534=CARTESIAN_POINT('Ctrl Pts',(8.59489616871541,20.3132488873796,4.96226561664473));
#15535=CARTESIAN_POINT('Ctrl Pts',(11.4598615582757,20.4882488873797,-2.0193949029962E-11));
#15536=CARTESIAN_POINT('Ctrl Pts',(8.5948961686982,20.6632488873797,-4.96226561667453));
#15537=CARTESIAN_POINT('Ctrl Pts',(5.72993077912057,20.8382488873797,-9.92453123332941));
#15538=CARTESIAN_POINT('Ctrl Pts',(-1.74349766336024E-11,21.0132488873797,
-9.92453123331945));
#15539=CARTESIAN_POINT('Ctrl Pts',(-5.72993077915487,21.1882488873797,-9.92453123330961));
#15540=CARTESIAN_POINT('Ctrl Pts',(-8.59489616871535,21.3632488873797,-4.96226561664482));
#15541=CARTESIAN_POINT('Ctrl Pts',(-11.4598615582757,21.5382488873796,2.00704047809387E-11));
#15542=CARTESIAN_POINT('Ctrl Pts',(-8.59489616869825,21.7132488873797,4.96226561667444));
#15543=CARTESIAN_POINT('Ctrl Pts',(-5.72993077912067,21.8882488873797,9.92453123332935));
#15544=CARTESIAN_POINT('Ctrl Pts',(1.73279841754567E-11,22.0632488873797,
9.92453123331945));
#15545=CARTESIAN_POINT('Ctrl Pts',(2.38370069761474,22.1360503989788,9.92453123331524));
#15546=CARTESIAN_POINT('Ctrl Pts',(4.50738083181344,22.22,8.84193633985987));
#15547=CARTESIAN_POINT('Ctrl Pts',(-1.51301075899711E-11,-144.093984254242,
-8.40164026751963));
#15548=CARTESIAN_POINT('Ctrl Pts',(-4.85068927010199,-143.918984254242,
-8.4016402675109));
#15549=CARTESIAN_POINT('Ctrl Pts',(-7.27603390513785,-143.743984254242,
-4.20082013374671));
#15550=CARTESIAN_POINT('Ctrl Pts',(-9.70137854017372,-143.568984254242,
1.74701493417668E-11));
#15551=CARTESIAN_POINT('Ctrl Pts',(-7.27603390512272,-143.393984254242,
4.20082013377292));
#15552=CARTESIAN_POINT('Ctrl Pts',(-4.85068927007173,-143.218984254242,
8.40164026752836));
#15553=CARTESIAN_POINT('Ctrl Pts',(1.5129078685785E-11,-143.043984254242,
8.40164026751963));
#15554=CARTESIAN_POINT('Ctrl Pts',(4.85068927010198,-142.868984254242,8.4016402675109));
#15555=CARTESIAN_POINT('Ctrl Pts',(7.27603390513785,-142.693984254242,4.20082013374672));
#15556=CARTESIAN_POINT('Ctrl Pts',(9.70137854017372,-142.518984254242,-1.74689612655491E-11));
#15557=CARTESIAN_POINT('Ctrl Pts',(7.27603390512273,-142.343984254242,-4.20082013377291));
#15558=CARTESIAN_POINT('Ctrl Pts',(4.85068927007173,-142.168984254242,-8.40164026752836));
#15559=CARTESIAN_POINT('Ctrl Pts',(-1.51301075899711E-11,-141.993984254242,
-8.40164026751963));
#15560=CARTESIAN_POINT('Ctrl Pts',(-4.85068927010199,-141.818984254242,
-8.4016402675109));
#15561=CARTESIAN_POINT('Ctrl Pts',(-7.27603390513785,-141.643984254242,
-4.20082013374671));
#15562=CARTESIAN_POINT('Ctrl Pts',(-9.70137854017372,-141.468984254242,
1.74701493417668E-11));
#15563=CARTESIAN_POINT('Ctrl Pts',(-7.27603390512272,-141.293984254242,
4.20082013377292));
#15564=CARTESIAN_POINT('Ctrl Pts',(-4.85068927007173,-141.118984254242,
8.40164026752836));
#15565=CARTESIAN_POINT('Ctrl Pts',(1.5129078685785E-11,-140.943984254242,
8.40164026751963));
#15566=CARTESIAN_POINT('Ctrl Pts',(4.85068927010198,-140.768984254242,8.4016402675109));
#15567=CARTESIAN_POINT('Ctrl Pts',(7.27603390513785,-140.593984254242,4.20082013374672));
#15568=CARTESIAN_POINT('Ctrl Pts',(9.70137854017372,-140.418984254242,-1.74689612655491E-11));
#15569=CARTESIAN_POINT('Ctrl Pts',(7.27603390512273,-140.243984254242,-4.20082013377291));
#15570=CARTESIAN_POINT('Ctrl Pts',(4.85068927007173,-140.068984254242,-8.40164026752836));
#15571=CARTESIAN_POINT('Ctrl Pts',(-1.51301075899711E-11,-139.893984254242,
-8.40164026751963));
#15572=CARTESIAN_POINT('Ctrl Pts',(-4.85068927010199,-139.718984254242,
-8.4016402675109));
#15573=CARTESIAN_POINT('Ctrl Pts',(-7.27603390513785,-139.543984254242,
-4.20082013374671));
#15574=CARTESIAN_POINT('Ctrl Pts',(-9.70137854017372,-139.368984254242,
1.74701493417668E-11));
#15575=CARTESIAN_POINT('Ctrl Pts',(-7.27603390512272,-139.193984254242,
4.20082013377292));
#15576=CARTESIAN_POINT('Ctrl Pts',(-4.85068927007173,-139.018984254242,
8.40164026752836));
#15577=CARTESIAN_POINT('Ctrl Pts',(1.5129078685785E-11,-138.843984254242,
8.40164026751963));
#15578=CARTESIAN_POINT('Ctrl Pts',(4.85068927010198,-138.668984254242,8.4016402675109));
#15579=CARTESIAN_POINT('Ctrl Pts',(7.27603390513785,-138.493984254242,4.20082013374672));
#15580=CARTESIAN_POINT('Ctrl Pts',(9.70137854017372,-138.318984254242,-1.74689612655491E-11));
#15581=CARTESIAN_POINT('Ctrl Pts',(7.27603390512273,-138.143984254242,-4.20082013377291));
#15582=CARTESIAN_POINT('Ctrl Pts',(4.85068927007173,-137.968984254242,-8.40164026752836));
#15583=CARTESIAN_POINT('Ctrl Pts',(-1.51301075899711E-11,-137.793984254242,
-8.40164026751963));
#15584=CARTESIAN_POINT('Ctrl Pts',(-4.85068927010199,-137.618984254242,
-8.4016402675109));
#15585=CARTESIAN_POINT('Ctrl Pts',(-7.27603390513785,-137.443984254242,
-4.20082013374671));
#15586=CARTESIAN_POINT('Ctrl Pts',(-9.70137854017372,-137.268984254242,
1.74701493417668E-11));
#15587=CARTESIAN_POINT('Ctrl Pts',(-7.27603390512272,-137.093984254242,
4.20082013377292));
#15588=CARTESIAN_POINT('Ctrl Pts',(-4.85068927007173,-136.918984254242,
8.40164026752836));
#15589=CARTESIAN_POINT('Ctrl Pts',(1.5129078685785E-11,-136.743984254242,
8.40164026751963));
#15590=CARTESIAN_POINT('Ctrl Pts',(4.85068927010198,-136.568984254242,8.4016402675109));
#15591=CARTESIAN_POINT('Ctrl Pts',(7.27603390513785,-136.393984254242,4.20082013374672));
#15592=CARTESIAN_POINT('Ctrl Pts',(9.70137854017372,-136.218984254242,-1.74689612655491E-11));
#15593=CARTESIAN_POINT('Ctrl Pts',(7.27603390512273,-136.043984254242,-4.20082013377291));
#15594=CARTESIAN_POINT('Ctrl Pts',(4.85068927007173,-135.868984254242,-8.40164026752836));
#15595=CARTESIAN_POINT('Ctrl Pts',(-1.51301075899711E-11,-135.693984254242,
-8.40164026751963));
#15596=CARTESIAN_POINT('Ctrl Pts',(-4.85068927010199,-135.518984254242,
-8.4016402675109));
#15597=CARTESIAN_POINT('Ctrl Pts',(-7.27603390513785,-135.343984254242,
-4.20082013374671));
#15598=CARTESIAN_POINT('Ctrl Pts',(-9.70137854017372,-135.168984254242,
1.74701493417668E-11));
#15599=CARTESIAN_POINT('Ctrl Pts',(-7.27603390512272,-134.993984254242,
4.20082013377292));
#15600=CARTESIAN_POINT('Ctrl Pts',(-4.85068927007173,-134.818984254242,
8.40164026752836));
#15601=CARTESIAN_POINT('Ctrl Pts',(1.5129078685785E-11,-134.643984254242,
8.40164026751963));
#15602=CARTESIAN_POINT('Ctrl Pts',(4.85068927010198,-134.468984254242,8.4016402675109));
#15603=CARTESIAN_POINT('Ctrl Pts',(7.27603390513785,-134.293984254242,4.20082013374672));
#15604=CARTESIAN_POINT('Ctrl Pts',(9.70137854017372,-134.118984254242,-1.74689612655491E-11));
#15605=CARTESIAN_POINT('Ctrl Pts',(7.27603390512273,-133.943984254242,-4.20082013377291));
#15606=CARTESIAN_POINT('Ctrl Pts',(4.85068927007173,-133.768984254242,-8.40164026752836));
#15607=CARTESIAN_POINT('Ctrl Pts',(-1.51301075899711E-11,-133.593984254242,
-8.40164026751963));
#15608=CARTESIAN_POINT('Ctrl Pts',(-4.85068927010199,-133.418984254242,
-8.4016402675109));
#15609=CARTESIAN_POINT('Ctrl Pts',(-7.27603390513785,-133.243984254242,
-4.20082013374671));
#15610=CARTESIAN_POINT('Ctrl Pts',(-9.70137854017372,-133.068984254242,
1.74701493417668E-11));
#15611=CARTESIAN_POINT('Ctrl Pts',(-7.27603390512272,-132.893984254242,
4.20082013377292));
#15612=CARTESIAN_POINT('Ctrl Pts',(-4.85068927007173,-132.718984254242,
8.40164026752836));
#15613=CARTESIAN_POINT('Ctrl Pts',(1.5129078685785E-11,-132.543984254242,
8.40164026751963));
#15614=CARTESIAN_POINT('Ctrl Pts',(4.85068927010198,-132.368984254242,8.4016402675109));
#15615=CARTESIAN_POINT('Ctrl Pts',(7.27603390513785,-132.193984254242,4.20082013374672));
#15616=CARTESIAN_POINT('Ctrl Pts',(9.70137854017372,-132.018984254242,-1.74689612655491E-11));
#15617=CARTESIAN_POINT('Ctrl Pts',(7.27603390512273,-131.843984254242,-4.20082013377291));
#15618=CARTESIAN_POINT('Ctrl Pts',(4.85068927007173,-131.668984254242,-8.40164026752836));
#15619=CARTESIAN_POINT('Ctrl Pts',(-1.51301075899711E-11,-131.493984254242,
-8.40164026751963));
#15620=CARTESIAN_POINT('Ctrl Pts',(-4.85068927010199,-131.318984254242,
-8.4016402675109));
#15621=CARTESIAN_POINT('Ctrl Pts',(-7.27603390513785,-131.143984254242,
-4.20082013374671));
#15622=CARTESIAN_POINT('Ctrl Pts',(-9.70137854017372,-130.968984254242,
1.74701493417668E-11));
#15623=CARTESIAN_POINT('Ctrl Pts',(-7.27603390512272,-130.793984254242,
4.20082013377292));
#15624=CARTESIAN_POINT('Ctrl Pts',(-4.85068927007173,-130.618984254242,
8.40164026752836));
#15625=CARTESIAN_POINT('Ctrl Pts',(1.5129078685785E-11,-130.443984254242,
8.40164026751963));
#15626=CARTESIAN_POINT('Ctrl Pts',(4.85068927010198,-130.268984254242,8.4016402675109));
#15627=CARTESIAN_POINT('Ctrl Pts',(7.27603390513785,-130.093984254242,4.20082013374672));
#15628=CARTESIAN_POINT('Ctrl Pts',(9.70137854017372,-129.918984254242,-1.74689612655491E-11));
#15629=CARTESIAN_POINT('Ctrl Pts',(7.27603390512273,-129.743984254242,-4.20082013377291));
#15630=CARTESIAN_POINT('Ctrl Pts',(4.85068927007173,-129.568984254242,-8.40164026752836));
#15631=CARTESIAN_POINT('Ctrl Pts',(-1.51301075899711E-11,-129.393984254242,
-8.40164026751963));
#15632=CARTESIAN_POINT('Ctrl Pts',(-4.85068927010199,-129.218984254242,
-8.4016402675109));
#15633=CARTESIAN_POINT('Ctrl Pts',(-7.27603390513785,-129.043984254242,
-4.20082013374671));
#15634=CARTESIAN_POINT('Ctrl Pts',(-9.70137854017372,-128.868984254242,
1.74701493417668E-11));
#15635=CARTESIAN_POINT('Ctrl Pts',(-7.27603390512272,-128.693984254242,
4.20082013377292));
#15636=CARTESIAN_POINT('Ctrl Pts',(-4.85068927007173,-128.518984254242,
8.40164026752836));
#15637=CARTESIAN_POINT('Ctrl Pts',(1.5129078685785E-11,-128.343984254242,
8.40164026751963));
#15638=CARTESIAN_POINT('Ctrl Pts',(4.85068927010198,-128.168984254242,8.4016402675109));
#15639=CARTESIAN_POINT('Ctrl Pts',(7.27603390513785,-127.993984254242,4.20082013374672));
#15640=CARTESIAN_POINT('Ctrl Pts',(9.70137854017372,-127.818984254242,-1.74689612655491E-11));
#15641=CARTESIAN_POINT('Ctrl Pts',(7.27603390512273,-127.643984254242,-4.20082013377291));
#15642=CARTESIAN_POINT('Ctrl Pts',(4.85068927007173,-127.468984254242,-8.40164026752836));
#15643=CARTESIAN_POINT('Ctrl Pts',(-1.51301075899711E-11,-127.293984254242,
-8.40164026751963));
#15644=CARTESIAN_POINT('Ctrl Pts',(-4.85068927010199,-127.118984254242,
-8.4016402675109));
#15645=CARTESIAN_POINT('Ctrl Pts',(-7.27603390513785,-126.943984254242,
-4.20082013374671));
#15646=CARTESIAN_POINT('Ctrl Pts',(-9.70137854017372,-126.768984254242,
1.74701493417668E-11));
#15647=CARTESIAN_POINT('Ctrl Pts',(-7.27603390512272,-126.593984254242,
4.20082013377292));
#15648=CARTESIAN_POINT('Ctrl Pts',(-4.85068927007173,-126.418984254242,
8.40164026752836));
#15649=CARTESIAN_POINT('Ctrl Pts',(1.5129078685785E-11,-126.243984254242,
8.40164026751963));
#15650=CARTESIAN_POINT('Ctrl Pts',(4.85068927010198,-126.068984254242,8.4016402675109));
#15651=CARTESIAN_POINT('Ctrl Pts',(7.27603390513785,-125.893984254242,4.20082013374672));
#15652=CARTESIAN_POINT('Ctrl Pts',(9.70137854017372,-125.718984254242,-1.74689612655491E-11));
#15653=CARTESIAN_POINT('Ctrl Pts',(7.27603390512273,-125.543984254242,-4.20082013377291));
#15654=CARTESIAN_POINT('Ctrl Pts',(4.85068927007173,-125.368984254242,-8.40164026752836));
#15655=CARTESIAN_POINT('Ctrl Pts',(-1.51301075899711E-11,-125.193984254242,
-8.40164026751963));
#15656=CARTESIAN_POINT('Ctrl Pts',(-4.85068927010199,-125.018984254242,
-8.4016402675109));
#15657=CARTESIAN_POINT('Ctrl Pts',(-7.27603390513785,-124.843984254242,
-4.20082013374671));
#15658=CARTESIAN_POINT('Ctrl Pts',(-9.70137854017372,-124.668984254242,
1.74701493417668E-11));
#15659=CARTESIAN_POINT('Ctrl Pts',(-7.27603390512272,-124.493984254242,
4.20082013377292));
#15660=CARTESIAN_POINT('Ctrl Pts',(-4.85068927007173,-124.318984254242,
8.40164026752836));
#15661=CARTESIAN_POINT('Ctrl Pts',(1.5129078685785E-11,-124.143984254242,
8.40164026751963));
#15662=CARTESIAN_POINT('Ctrl Pts',(4.85068927010198,-123.968984254242,8.4016402675109));
#15663=CARTESIAN_POINT('Ctrl Pts',(7.27603390513785,-123.793984254242,4.20082013374672));
#15664=CARTESIAN_POINT('Ctrl Pts',(9.70137854017372,-123.618984254242,-1.74689612655491E-11));
#15665=CARTESIAN_POINT('Ctrl Pts',(7.27603390512273,-123.443984254242,-4.20082013377291));
#15666=CARTESIAN_POINT('Ctrl Pts',(4.85068927007173,-123.268984254242,-8.40164026752836));
#15667=CARTESIAN_POINT('Ctrl Pts',(-1.51301075899711E-11,-123.093984254242,
-8.40164026751963));
#15668=CARTESIAN_POINT('Ctrl Pts',(-4.85068927010199,-122.918984254242,
-8.4016402675109));
#15669=CARTESIAN_POINT('Ctrl Pts',(-7.27603390513785,-122.743984254242,
-4.20082013374671));
#15670=CARTESIAN_POINT('Ctrl Pts',(-9.70137854017372,-122.568984254242,
1.74701493417668E-11));
#15671=CARTESIAN_POINT('Ctrl Pts',(-7.27603390512272,-122.393984254242,
4.20082013377292));
#15672=CARTESIAN_POINT('Ctrl Pts',(-4.85068927007173,-122.218984254242,
8.40164026752836));
#15673=CARTESIAN_POINT('Ctrl Pts',(1.5129078685785E-11,-122.043984254242,
8.40164026751963));
#15674=CARTESIAN_POINT('Ctrl Pts',(4.85068927010198,-121.868984254242,8.4016402675109));
#15675=CARTESIAN_POINT('Ctrl Pts',(7.27603390513785,-121.693984254242,4.20082013374672));
#15676=CARTESIAN_POINT('Ctrl Pts',(9.70137854017372,-121.518984254242,-1.74689612655491E-11));
#15677=CARTESIAN_POINT('Ctrl Pts',(7.27603390512273,-121.343984254242,-4.20082013377291));
#15678=CARTESIAN_POINT('Ctrl Pts',(4.85068927007173,-121.168984254242,-8.40164026752836));
#15679=CARTESIAN_POINT('Ctrl Pts',(-1.51301075899711E-11,-120.993984254242,
-8.40164026751963));
#15680=CARTESIAN_POINT('Ctrl Pts',(-4.85068927010199,-120.818984254242,
-8.4016402675109));
#15681=CARTESIAN_POINT('Ctrl Pts',(-7.27603390513785,-120.643984254242,
-4.20082013374671));
#15682=CARTESIAN_POINT('Ctrl Pts',(-9.70137854017372,-120.468984254242,
1.74701493417668E-11));
#15683=CARTESIAN_POINT('Ctrl Pts',(-7.27603390512272,-120.293984254242,
4.20082013377292));
#15684=CARTESIAN_POINT('Ctrl Pts',(-4.85068927007173,-120.118984254242,
8.40164026752836));
#15685=CARTESIAN_POINT('Ctrl Pts',(1.5129078685785E-11,-119.943984254242,
8.40164026751963));
#15686=CARTESIAN_POINT('Ctrl Pts',(4.85068927010198,-119.768984254242,8.4016402675109));
#15687=CARTESIAN_POINT('Ctrl Pts',(7.27603390513785,-119.593984254242,4.20082013374672));
#15688=CARTESIAN_POINT('Ctrl Pts',(9.70137854017372,-119.418984254242,-1.74689612655491E-11));
#15689=CARTESIAN_POINT('Ctrl Pts',(7.27603390512273,-119.243984254242,-4.20082013377291));
#15690=CARTESIAN_POINT('Ctrl Pts',(4.85068927007173,-119.068984254242,-8.40164026752836));
#15691=CARTESIAN_POINT('Ctrl Pts',(-1.51301075899711E-11,-118.893984254242,
-8.40164026751963));
#15692=CARTESIAN_POINT('Ctrl Pts',(-4.85068927010199,-118.718984254242,
-8.4016402675109));
#15693=CARTESIAN_POINT('Ctrl Pts',(-7.27603390513785,-118.543984254242,
-4.20082013374671));
#15694=CARTESIAN_POINT('Ctrl Pts',(-9.70137854017372,-118.368984254242,
1.74701493417668E-11));
#15695=CARTESIAN_POINT('Ctrl Pts',(-7.27603390512272,-118.193984254242,
4.20082013377292));
#15696=CARTESIAN_POINT('Ctrl Pts',(-4.85068927007173,-118.018984254242,
8.40164026752836));
#15697=CARTESIAN_POINT('Ctrl Pts',(1.5129078685785E-11,-117.843984254242,
8.40164026751963));
#15698=CARTESIAN_POINT('Ctrl Pts',(4.85068927010198,-117.668984254242,8.4016402675109));
#15699=CARTESIAN_POINT('Ctrl Pts',(7.27603390513785,-117.493984254242,4.20082013374672));
#15700=CARTESIAN_POINT('Ctrl Pts',(9.70137854017372,-117.318984254242,-1.74689612655491E-11));
#15701=CARTESIAN_POINT('Ctrl Pts',(7.27603390512273,-117.143984254242,-4.20082013377291));
#15702=CARTESIAN_POINT('Ctrl Pts',(4.85068927007173,-116.968984254242,-8.40164026752836));
#15703=CARTESIAN_POINT('Ctrl Pts',(-1.51301075899711E-11,-116.793984254242,
-8.40164026751963));
#15704=CARTESIAN_POINT('Ctrl Pts',(-4.85068927010199,-116.618984254242,
-8.4016402675109));
#15705=CARTESIAN_POINT('Ctrl Pts',(-7.27603390513785,-116.443984254242,
-4.20082013374671));
#15706=CARTESIAN_POINT('Ctrl Pts',(-9.70137854017372,-116.268984254242,
1.74701493417668E-11));
#15707=CARTESIAN_POINT('Ctrl Pts',(-7.27603390512272,-116.093984254242,
4.20082013377292));
#15708=CARTESIAN_POINT('Ctrl Pts',(-4.85068927007173,-115.918984254242,
8.40164026752836));
#15709=CARTESIAN_POINT('Ctrl Pts',(1.5129078685785E-11,-115.743984254242,
8.40164026751963));
#15710=CARTESIAN_POINT('Ctrl Pts',(4.85068927010198,-115.568984254242,8.4016402675109));
#15711=CARTESIAN_POINT('Ctrl Pts',(7.27603390513785,-115.393984254242,4.20082013374672));
#15712=CARTESIAN_POINT('Ctrl Pts',(9.70137854017372,-115.218984254242,-1.74689612655491E-11));
#15713=CARTESIAN_POINT('Ctrl Pts',(7.27603390512273,-115.043984254242,-4.20082013377291));
#15714=CARTESIAN_POINT('Ctrl Pts',(4.85068927007173,-114.868984254242,-8.40164026752836));
#15715=CARTESIAN_POINT('Ctrl Pts',(-1.51301075899711E-11,-114.693984254242,
-8.40164026751963));
#15716=CARTESIAN_POINT('Ctrl Pts',(-4.85068927010199,-114.518984254242,
-8.4016402675109));
#15717=CARTESIAN_POINT('Ctrl Pts',(-7.27603390513785,-114.343984254242,
-4.20082013374671));
#15718=CARTESIAN_POINT('Ctrl Pts',(-9.70137854017372,-114.168984254242,
1.74701493417668E-11));
#15719=CARTESIAN_POINT('Ctrl Pts',(-7.27603390512272,-113.993984254242,
4.20082013377292));
#15720=CARTESIAN_POINT('Ctrl Pts',(-4.85068927007173,-113.818984254242,
8.40164026752836));
#15721=CARTESIAN_POINT('Ctrl Pts',(1.5129078685785E-11,-113.643984254242,
8.40164026751963));
#15722=CARTESIAN_POINT('Ctrl Pts',(4.85068927010198,-113.468984254242,8.4016402675109));
#15723=CARTESIAN_POINT('Ctrl Pts',(7.27603390513785,-113.293984254242,4.20082013374672));
#15724=CARTESIAN_POINT('Ctrl Pts',(9.70137854017372,-113.118984254242,-1.74689612655491E-11));
#15725=CARTESIAN_POINT('Ctrl Pts',(7.27603390512273,-112.943984254242,-4.20082013377291));
#15726=CARTESIAN_POINT('Ctrl Pts',(4.85068927007173,-112.768984254242,-8.40164026752836));
#15727=CARTESIAN_POINT('Ctrl Pts',(-1.51301075899711E-11,-112.593984254242,
-8.40164026751963));
#15728=CARTESIAN_POINT('Ctrl Pts',(-4.85068927010199,-112.418984254242,
-8.4016402675109));
#15729=CARTESIAN_POINT('Ctrl Pts',(-7.27603390513785,-112.243984254242,
-4.20082013374671));
#15730=CARTESIAN_POINT('Ctrl Pts',(-9.70137854017372,-112.068984254242,
1.74701493417668E-11));
#15731=CARTESIAN_POINT('Ctrl Pts',(-7.27603390512272,-111.893984254242,
4.20082013377292));
#15732=CARTESIAN_POINT('Ctrl Pts',(-4.85068927007173,-111.718984254242,
8.40164026752836));
#15733=CARTESIAN_POINT('Ctrl Pts',(1.5129078685785E-11,-111.543984254242,
8.40164026751963));
#15734=CARTESIAN_POINT('Ctrl Pts',(4.85068927010198,-111.368984254242,8.4016402675109));
#15735=CARTESIAN_POINT('Ctrl Pts',(7.27603390513785,-111.193984254242,4.20082013374672));
#15736=CARTESIAN_POINT('Ctrl Pts',(9.70137854017372,-111.018984254242,-1.74689612655491E-11));
#15737=CARTESIAN_POINT('Ctrl Pts',(7.27603390512273,-110.843984254242,-4.20082013377291));
#15738=CARTESIAN_POINT('Ctrl Pts',(4.85068927007173,-110.668984254242,-8.40164026752836));
#15739=CARTESIAN_POINT('Ctrl Pts',(-1.51301075899711E-11,-110.493984254242,
-8.40164026751963));
#15740=CARTESIAN_POINT('Ctrl Pts',(-4.85068927010199,-110.318984254242,
-8.4016402675109));
#15741=CARTESIAN_POINT('Ctrl Pts',(-7.27603390513785,-110.143984254242,
-4.20082013374671));
#15742=CARTESIAN_POINT('Ctrl Pts',(-9.70137854017372,-109.968984254242,
1.74701493417668E-11));
#15743=CARTESIAN_POINT('Ctrl Pts',(-7.27603390512272,-109.793984254242,
4.20082013377292));
#15744=CARTESIAN_POINT('Ctrl Pts',(-4.85068927007173,-109.618984254242,
8.40164026752836));
#15745=CARTESIAN_POINT('Ctrl Pts',(1.5129078685785E-11,-109.443984254242,
8.40164026751963));
#15746=CARTESIAN_POINT('Ctrl Pts',(4.85068927010198,-109.268984254242,8.4016402675109));
#15747=CARTESIAN_POINT('Ctrl Pts',(7.27603390513785,-109.093984254242,4.20082013374672));
#15748=CARTESIAN_POINT('Ctrl Pts',(9.70137854017372,-108.918984254242,-1.74689612655491E-11));
#15749=CARTESIAN_POINT('Ctrl Pts',(7.27603390512273,-108.743984254242,-4.20082013377291));
#15750=CARTESIAN_POINT('Ctrl Pts',(4.85068927007173,-108.568984254242,-8.40164026752836));
#15751=CARTESIAN_POINT('Ctrl Pts',(-1.51301075899711E-11,-108.393984254242,
-8.40164026751963));
#15752=CARTESIAN_POINT('Ctrl Pts',(-4.85068927010199,-108.218984254242,
-8.4016402675109));
#15753=CARTESIAN_POINT('Ctrl Pts',(-7.27603390513785,-108.043984254242,
-4.20082013374671));
#15754=CARTESIAN_POINT('Ctrl Pts',(-9.70137854017372,-107.868984254242,
1.74701493417668E-11));
#15755=CARTESIAN_POINT('Ctrl Pts',(-7.27603390512272,-107.693984254242,
4.20082013377292));
#15756=CARTESIAN_POINT('Ctrl Pts',(-4.85068927007173,-107.518984254242,
8.40164026752836));
#15757=CARTESIAN_POINT('Ctrl Pts',(1.5129078685785E-11,-107.343984254242,
8.40164026751963));
#15758=CARTESIAN_POINT('Ctrl Pts',(4.85068927010198,-107.168984254242,8.4016402675109));
#15759=CARTESIAN_POINT('Ctrl Pts',(7.27603390513785,-106.993984254242,4.20082013374672));
#15760=CARTESIAN_POINT('Ctrl Pts',(9.70137854017372,-106.818984254242,-1.74689612655491E-11));
#15761=CARTESIAN_POINT('Ctrl Pts',(7.27603390512273,-106.643984254242,-4.20082013377291));
#15762=CARTESIAN_POINT('Ctrl Pts',(4.85068927007173,-106.468984254242,-8.40164026752836));
#15763=CARTESIAN_POINT('Ctrl Pts',(-1.51301075899711E-11,-106.293984254242,
-8.40164026751963));
#15764=CARTESIAN_POINT('Ctrl Pts',(-4.85068927010199,-106.118984254242,
-8.4016402675109));
#15765=CARTESIAN_POINT('Ctrl Pts',(-7.27603390513785,-105.943984254242,
-4.20082013374671));
#15766=CARTESIAN_POINT('Ctrl Pts',(-9.70137854017372,-105.768984254242,
1.74701493417668E-11));
#15767=CARTESIAN_POINT('Ctrl Pts',(-7.27603390512272,-105.593984254242,
4.20082013377292));
#15768=CARTESIAN_POINT('Ctrl Pts',(-4.85068927007173,-105.418984254242,
8.40164026752836));
#15769=CARTESIAN_POINT('Ctrl Pts',(1.5129078685785E-11,-105.243984254242,
8.40164026751963));
#15770=CARTESIAN_POINT('Ctrl Pts',(4.85068927010198,-105.068984254242,8.4016402675109));
#15771=CARTESIAN_POINT('Ctrl Pts',(7.27603390513785,-104.893984254242,4.20082013374672));
#15772=CARTESIAN_POINT('Ctrl Pts',(9.70137854017372,-104.718984254242,-1.74689612655491E-11));
#15773=CARTESIAN_POINT('Ctrl Pts',(7.27603390512273,-104.543984254242,-4.20082013377291));
#15774=CARTESIAN_POINT('Ctrl Pts',(4.85068927007173,-104.368984254242,-8.40164026752836));
#15775=CARTESIAN_POINT('Ctrl Pts',(-1.51301075899711E-11,-104.193984254242,
-8.40164026751963));
#15776=CARTESIAN_POINT('Ctrl Pts',(-4.85068927010199,-104.018984254242,
-8.4016402675109));
#15777=CARTESIAN_POINT('Ctrl Pts',(-7.27603390513785,-103.843984254242,
-4.20082013374671));
#15778=CARTESIAN_POINT('Ctrl Pts',(-9.70137854017372,-103.668984254242,
1.74701493417668E-11));
#15779=CARTESIAN_POINT('Ctrl Pts',(-7.27603390512272,-103.493984254242,
4.20082013377292));
#15780=CARTESIAN_POINT('Ctrl Pts',(-4.85068927007173,-103.318984254242,
8.40164026752836));
#15781=CARTESIAN_POINT('Ctrl Pts',(1.5129078685785E-11,-103.143984254242,
8.40164026751963));
#15782=CARTESIAN_POINT('Ctrl Pts',(4.85068927010198,-102.968984254242,8.4016402675109));
#15783=CARTESIAN_POINT('Ctrl Pts',(7.27603390513785,-102.793984254242,4.20082013374672));
#15784=CARTESIAN_POINT('Ctrl Pts',(9.70137854017372,-102.618984254242,-1.74689612655491E-11));
#15785=CARTESIAN_POINT('Ctrl Pts',(7.27603390512273,-102.443984254242,-4.20082013377291));
#15786=CARTESIAN_POINT('Ctrl Pts',(4.85068927007173,-102.268984254242,-8.40164026752836));
#15787=CARTESIAN_POINT('Ctrl Pts',(-1.51301075899711E-11,-102.093984254242,
-8.40164026751963));
#15788=CARTESIAN_POINT('Ctrl Pts',(-4.85068927010199,-101.918984254242,
-8.4016402675109));
#15789=CARTESIAN_POINT('Ctrl Pts',(-7.27603390513785,-101.743984254242,
-4.20082013374671));
#15790=CARTESIAN_POINT('Ctrl Pts',(-9.70137854017372,-101.568984254242,
1.74701493417668E-11));
#15791=CARTESIAN_POINT('Ctrl Pts',(-7.27603390512272,-101.393984254242,
4.20082013377292));
#15792=CARTESIAN_POINT('Ctrl Pts',(-4.85068927007173,-101.218984254242,
8.40164026752836));
#15793=CARTESIAN_POINT('Ctrl Pts',(1.5129078685785E-11,-101.043984254242,
8.40164026751963));
#15794=CARTESIAN_POINT('Ctrl Pts',(4.85068927010198,-100.868984254242,8.4016402675109));
#15795=CARTESIAN_POINT('Ctrl Pts',(7.27603390513785,-100.693984254242,4.20082013374672));
#15796=CARTESIAN_POINT('Ctrl Pts',(9.70137854017372,-100.518984254242,-1.74689612655491E-11));
#15797=CARTESIAN_POINT('Ctrl Pts',(7.27603390512273,-100.343984254242,-4.20082013377291));
#15798=CARTESIAN_POINT('Ctrl Pts',(4.85068927007173,-100.168984254242,-8.40164026752836));
#15799=CARTESIAN_POINT('Ctrl Pts',(-1.51301075899711E-11,-99.9939842542418,
-8.40164026751963));
#15800=CARTESIAN_POINT('Ctrl Pts',(-4.85068927010199,-99.8189842542418,
-8.4016402675109));
#15801=CARTESIAN_POINT('Ctrl Pts',(-7.27603390513785,-99.6439842542417,
-4.20082013374671));
#15802=CARTESIAN_POINT('Ctrl Pts',(-9.70137854017372,-99.4689842542418,
1.74701493417668E-11));
#15803=CARTESIAN_POINT('Ctrl Pts',(-7.27603390512272,-99.2939842542417,
4.20082013377292));
#15804=CARTESIAN_POINT('Ctrl Pts',(-4.85068927007173,-99.1189842542418,
8.40164026752836));
#15805=CARTESIAN_POINT('Ctrl Pts',(1.5129078685785E-11,-98.9439842542418,
8.40164026751963));
#15806=CARTESIAN_POINT('Ctrl Pts',(4.85068927010198,-98.7689842542417,8.4016402675109));
#15807=CARTESIAN_POINT('Ctrl Pts',(7.27603390513785,-98.5939842542417,4.20082013374672));
#15808=CARTESIAN_POINT('Ctrl Pts',(9.70137854017372,-98.4189842542418,-1.74689612655491E-11));
#15809=CARTESIAN_POINT('Ctrl Pts',(7.27603390512273,-98.2439842542418,-4.20082013377291));
#15810=CARTESIAN_POINT('Ctrl Pts',(4.85068927007173,-98.0689842542417,-8.40164026752836));
#15811=CARTESIAN_POINT('Ctrl Pts',(-1.51301075899711E-11,-97.8939842542418,
-8.40164026751963));
#15812=CARTESIAN_POINT('Ctrl Pts',(-4.85068927010199,-97.7189842542418,
-8.4016402675109));
#15813=CARTESIAN_POINT('Ctrl Pts',(-7.27603390513785,-97.5439842542417,
-4.20082013374671));
#15814=CARTESIAN_POINT('Ctrl Pts',(-9.70137854017372,-97.3689842542418,
1.74701493417668E-11));
#15815=CARTESIAN_POINT('Ctrl Pts',(-7.27603390512272,-97.1939842542418,
4.20082013377292));
#15816=CARTESIAN_POINT('Ctrl Pts',(-4.85068927007173,-97.0189842542418,
8.40164026752836));
#15817=CARTESIAN_POINT('Ctrl Pts',(1.5129078685785E-11,-96.8439842542418,
8.40164026751963));
#15818=CARTESIAN_POINT('Ctrl Pts',(4.85068927010198,-96.6689842542418,8.4016402675109));
#15819=CARTESIAN_POINT('Ctrl Pts',(7.27603390513785,-96.4939842542417,4.20082013374672));
#15820=CARTESIAN_POINT('Ctrl Pts',(9.70137854017372,-96.3189842542418,-1.74689612655491E-11));
#15821=CARTESIAN_POINT('Ctrl Pts',(7.27603390512273,-96.1439842542418,-4.20082013377291));
#15822=CARTESIAN_POINT('Ctrl Pts',(4.85068927007173,-95.9689842542417,-8.40164026752836));
#15823=CARTESIAN_POINT('Ctrl Pts',(-1.51301075899711E-11,-95.7939842542418,
-8.40164026751963));
#15824=CARTESIAN_POINT('Ctrl Pts',(-4.85068927010199,-95.6189842542418,
-8.4016402675109));
#15825=CARTESIAN_POINT('Ctrl Pts',(-7.27603390513785,-95.4439842542418,
-4.20082013374671));
#15826=CARTESIAN_POINT('Ctrl Pts',(-9.70137854017372,-95.2689842542418,
1.74701493417668E-11));
#15827=CARTESIAN_POINT('Ctrl Pts',(-7.27603390512272,-95.0939842542418,
4.20082013377292));
#15828=CARTESIAN_POINT('Ctrl Pts',(-4.85068927007173,-94.9189842542418,
8.40164026752836));
#15829=CARTESIAN_POINT('Ctrl Pts',(1.5129078685785E-11,-94.7439842542418,
8.40164026751963));
#15830=CARTESIAN_POINT('Ctrl Pts',(4.85068927010198,-94.5689842542417,8.4016402675109));
#15831=CARTESIAN_POINT('Ctrl Pts',(7.27603390513785,-94.3939842542418,4.20082013374672));
#15832=CARTESIAN_POINT('Ctrl Pts',(9.70137854017372,-94.2189842542417,-1.74689612655491E-11));
#15833=CARTESIAN_POINT('Ctrl Pts',(7.27603390512273,-94.0439842542417,-4.20082013377291));
#15834=CARTESIAN_POINT('Ctrl Pts',(4.85068927007173,-93.8689842542418,-8.40164026752836));
#15835=CARTESIAN_POINT('Ctrl Pts',(-1.51301075899711E-11,-93.6939842542417,
-8.40164026751963));
#15836=CARTESIAN_POINT('Ctrl Pts',(-4.85068927010199,-93.5189842542417,
-8.4016402675109));
#15837=CARTESIAN_POINT('Ctrl Pts',(-7.27603390513785,-93.3439842542418,
-4.20082013374671));
#15838=CARTESIAN_POINT('Ctrl Pts',(-9.70137854017372,-93.1689842542418,
1.74701493417668E-11));
#15839=CARTESIAN_POINT('Ctrl Pts',(-7.27603390512272,-92.9939842542417,
4.20082013377292));
#15840=CARTESIAN_POINT('Ctrl Pts',(-4.85068927007173,-92.8189842542418,
8.40164026752836));
#15841=CARTESIAN_POINT('Ctrl Pts',(1.5129078685785E-11,-92.6439842542418,
8.40164026751963));
#15842=CARTESIAN_POINT('Ctrl Pts',(4.85068927010198,-92.4689842542418,8.4016402675109));
#15843=CARTESIAN_POINT('Ctrl Pts',(7.27603390513785,-92.2939842542418,4.20082013374672));
#15844=CARTESIAN_POINT('Ctrl Pts',(9.70137854017372,-92.1189842542418,-1.74689612655491E-11));
#15845=CARTESIAN_POINT('Ctrl Pts',(7.27603390512273,-91.9439842542417,-4.20082013377291));
#15846=CARTESIAN_POINT('Ctrl Pts',(4.85068927007173,-91.7689842542418,-8.40164026752836));
#15847=CARTESIAN_POINT('Ctrl Pts',(-1.51301075899711E-11,-91.5939842542418,
-8.40164026751963));
#15848=CARTESIAN_POINT('Ctrl Pts',(-4.85068927010199,-91.4189842542417,
-8.4016402675109));
#15849=CARTESIAN_POINT('Ctrl Pts',(-7.27603390513785,-91.2439842542418,
-4.20082013374671));
#15850=CARTESIAN_POINT('Ctrl Pts',(-9.70137854017372,-91.0689842542418,
1.74701493417668E-11));
#15851=CARTESIAN_POINT('Ctrl Pts',(-7.27603390512272,-90.8939842542418,
4.20082013377292));
#15852=CARTESIAN_POINT('Ctrl Pts',(-4.85068927007173,-90.7189842542418,
8.40164026752836));
#15853=CARTESIAN_POINT('Ctrl Pts',(1.5129078685785E-11,-90.5439842542418,
8.40164026751963));
#15854=CARTESIAN_POINT('Ctrl Pts',(4.85068927010198,-90.3689842542418,8.4016402675109));
#15855=CARTESIAN_POINT('Ctrl Pts',(7.27603390513785,-90.1939842542418,4.20082013374672));
#15856=CARTESIAN_POINT('Ctrl Pts',(9.70137854017372,-90.0189842542418,-1.74689612655491E-11));
#15857=CARTESIAN_POINT('Ctrl Pts',(7.27603390512273,-89.8439842542418,-4.20082013377291));
#15858=CARTESIAN_POINT('Ctrl Pts',(4.85068927007173,-89.6689842542418,-8.40164026752836));
#15859=CARTESIAN_POINT('Ctrl Pts',(-1.51301075899711E-11,-89.4939842542418,
-8.40164026751963));
#15860=CARTESIAN_POINT('Ctrl Pts',(-4.85068927010199,-89.3189842542418,
-8.4016402675109));
#15861=CARTESIAN_POINT('Ctrl Pts',(-7.27603390513785,-89.1439842542418,
-4.20082013374671));
#15862=CARTESIAN_POINT('Ctrl Pts',(-9.70137854017372,-88.9689842542418,
1.74701493417668E-11));
#15863=CARTESIAN_POINT('Ctrl Pts',(-7.27603390512272,-88.7939842542418,
4.20082013377292));
#15864=CARTESIAN_POINT('Ctrl Pts',(-4.85068927007173,-88.6189842542418,
8.40164026752836));
#15865=CARTESIAN_POINT('Ctrl Pts',(1.5129078685785E-11,-88.4439842542418,
8.40164026751963));
#15866=CARTESIAN_POINT('Ctrl Pts',(4.85068927010198,-88.2689842542418,8.4016402675109));
#15867=CARTESIAN_POINT('Ctrl Pts',(7.27603390513785,-88.0939842542418,4.20082013374672));
#15868=CARTESIAN_POINT('Ctrl Pts',(9.70137854017372,-87.9189842542418,-1.74689612655491E-11));
#15869=CARTESIAN_POINT('Ctrl Pts',(7.27603390512273,-87.7439842542418,-4.20082013377291));
#15870=CARTESIAN_POINT('Ctrl Pts',(4.85068927007173,-87.5689842542418,-8.40164026752836));
#15871=CARTESIAN_POINT('Ctrl Pts',(-1.51301075899711E-11,-87.3939842542418,
-8.40164026751963));
#15872=CARTESIAN_POINT('Ctrl Pts',(-4.85068927010199,-87.2189842542418,
-8.4016402675109));
#15873=CARTESIAN_POINT('Ctrl Pts',(-7.27603390513785,-87.0439842542418,
-4.20082013374671));
#15874=CARTESIAN_POINT('Ctrl Pts',(-9.70137854017372,-86.8689842542418,
1.74701493417668E-11));
#15875=CARTESIAN_POINT('Ctrl Pts',(-7.27603390512272,-86.6939842542418,
4.20082013377292));
#15876=CARTESIAN_POINT('Ctrl Pts',(-4.85068927007173,-86.5189842542418,
8.40164026752836));
#15877=CARTESIAN_POINT('Ctrl Pts',(1.5129078685785E-11,-86.3439842542418,
8.40164026751963));
#15878=CARTESIAN_POINT('Ctrl Pts',(4.85068927010198,-86.1689842542418,8.4016402675109));
#15879=CARTESIAN_POINT('Ctrl Pts',(7.27603390513785,-85.9939842542418,4.20082013374672));
#15880=CARTESIAN_POINT('Ctrl Pts',(9.70137854017372,-85.8189842542418,-1.74689612655491E-11));
#15881=CARTESIAN_POINT('Ctrl Pts',(7.27603390512273,-85.6439842542418,-4.20082013377291));
#15882=CARTESIAN_POINT('Ctrl Pts',(4.85068927007173,-85.4689842542418,-8.40164026752836));
#15883=CARTESIAN_POINT('Ctrl Pts',(-1.51301075899711E-11,-85.2939842542417,
-8.40164026751963));
#15884=CARTESIAN_POINT('Ctrl Pts',(-4.85068927010199,-85.1189842542418,
-8.4016402675109));
#15885=CARTESIAN_POINT('Ctrl Pts',(-7.27603390513785,-84.9439842542418,
-4.20082013374671));
#15886=CARTESIAN_POINT('Ctrl Pts',(-9.70137854017372,-84.7689842542418,
1.74701493417668E-11));
#15887=CARTESIAN_POINT('Ctrl Pts',(-7.27603390512272,-84.5939842542418,
4.20082013377292));
#15888=CARTESIAN_POINT('Ctrl Pts',(-4.85068927007173,-84.4189842542418,
8.40164026752836));
#15889=CARTESIAN_POINT('Ctrl Pts',(1.5129078685785E-11,-84.2439842542418,
8.40164026751963));
#15890=CARTESIAN_POINT('Ctrl Pts',(4.85068927010198,-84.0689842542418,8.4016402675109));
#15891=CARTESIAN_POINT('Ctrl Pts',(7.27603390513785,-83.8939842542418,4.20082013374672));
#15892=CARTESIAN_POINT('Ctrl Pts',(9.70137854017372,-83.7189842542418,-1.74689612655491E-11));
#15893=CARTESIAN_POINT('Ctrl Pts',(7.27603390512273,-83.5439842542418,-4.20082013377291));
#15894=CARTESIAN_POINT('Ctrl Pts',(4.85068927007173,-83.3689842542418,-8.40164026752836));
#15895=CARTESIAN_POINT('Ctrl Pts',(-1.51301075899711E-11,-83.1939842542418,
-8.40164026751963));
#15896=CARTESIAN_POINT('Ctrl Pts',(-4.85068927010199,-83.0189842542418,
-8.4016402675109));
#15897=CARTESIAN_POINT('Ctrl Pts',(-7.27603390513785,-82.8439842542418,
-4.20082013374671));
#15898=CARTESIAN_POINT('Ctrl Pts',(-9.70137854017372,-82.6689842542418,
1.74701493417668E-11));
#15899=CARTESIAN_POINT('Ctrl Pts',(-7.27603390512272,-82.4939842542418,
4.20082013377292));
#15900=CARTESIAN_POINT('Ctrl Pts',(-4.85068927007173,-82.3189842542418,
8.40164026752836));
#15901=CARTESIAN_POINT('Ctrl Pts',(1.5129078685785E-11,-82.1439842542418,
8.40164026751963));
#15902=CARTESIAN_POINT('Ctrl Pts',(4.85068927010198,-81.9689842542418,8.4016402675109));
#15903=CARTESIAN_POINT('Ctrl Pts',(7.27603390513785,-81.7939842542418,4.20082013374672));
#15904=CARTESIAN_POINT('Ctrl Pts',(9.70137854017372,-81.6189842542418,-1.74689612655491E-11));
#15905=CARTESIAN_POINT('Ctrl Pts',(7.27603390512273,-81.4439842542418,-4.20082013377291));
#15906=CARTESIAN_POINT('Ctrl Pts',(4.85068927007173,-81.2689842542418,-8.40164026752836));
#15907=CARTESIAN_POINT('Ctrl Pts',(-1.51301075899711E-11,-81.0939842542418,
-8.40164026751963));
#15908=CARTESIAN_POINT('Ctrl Pts',(-4.85068927010199,-80.9189842542418,
-8.4016402675109));
#15909=CARTESIAN_POINT('Ctrl Pts',(-7.27603390513785,-80.7439842542418,
-4.20082013374671));
#15910=CARTESIAN_POINT('Ctrl Pts',(-9.70137854017372,-80.5689842542418,
1.74701493417668E-11));
#15911=CARTESIAN_POINT('Ctrl Pts',(-7.27603390512272,-80.3939842542418,
4.20082013377292));
#15912=CARTESIAN_POINT('Ctrl Pts',(-4.85068927007173,-80.2189842542418,
8.40164026752836));
#15913=CARTESIAN_POINT('Ctrl Pts',(1.5129078685785E-11,-80.0439842542418,
8.40164026751963));
#15914=CARTESIAN_POINT('Ctrl Pts',(4.85068927010198,-79.8689842542418,8.4016402675109));
#15915=CARTESIAN_POINT('Ctrl Pts',(7.27603390513785,-79.6939842542418,4.20082013374672));
#15916=CARTESIAN_POINT('Ctrl Pts',(9.70137854017372,-79.5189842542418,-1.74689612655491E-11));
#15917=CARTESIAN_POINT('Ctrl Pts',(7.27603390512273,-79.3439842542418,-4.20082013377291));
#15918=CARTESIAN_POINT('Ctrl Pts',(4.85068927007173,-79.1689842542418,-8.40164026752836));
#15919=CARTESIAN_POINT('Ctrl Pts',(-1.51301075899711E-11,-78.9939842542418,
-8.40164026751963));
#15920=CARTESIAN_POINT('Ctrl Pts',(-4.85068927010199,-78.8189842542418,
-8.4016402675109));
#15921=CARTESIAN_POINT('Ctrl Pts',(-7.27603390513785,-78.6439842542418,
-4.20082013374671));
#15922=CARTESIAN_POINT('Ctrl Pts',(-9.70137854017372,-78.4689842542418,
1.74701493417668E-11));
#15923=CARTESIAN_POINT('Ctrl Pts',(-7.27603390512272,-78.2939842542418,
4.20082013377292));
#15924=CARTESIAN_POINT('Ctrl Pts',(-4.85068927007173,-78.1189842542418,
8.40164026752836));
#15925=CARTESIAN_POINT('Ctrl Pts',(1.5129078685785E-11,-77.9439842542418,
8.40164026751963));
#15926=CARTESIAN_POINT('Ctrl Pts',(4.85068927010198,-77.7689842542418,8.4016402675109));
#15927=CARTESIAN_POINT('Ctrl Pts',(7.27603390513785,-77.5939842542418,4.20082013374672));
#15928=CARTESIAN_POINT('Ctrl Pts',(9.70137854017372,-77.4189842542418,-1.74689612655491E-11));
#15929=CARTESIAN_POINT('Ctrl Pts',(7.27603390512273,-77.2439842542418,-4.20082013377291));
#15930=CARTESIAN_POINT('Ctrl Pts',(4.85068927007173,-77.0689842542418,-8.40164026752836));
#15931=CARTESIAN_POINT('Ctrl Pts',(-1.51301075899711E-11,-76.8939842542418,
-8.40164026751963));
#15932=CARTESIAN_POINT('Ctrl Pts',(-4.85068927010199,-76.7189842542418,
-8.4016402675109));
#15933=CARTESIAN_POINT('Ctrl Pts',(-7.27603390513785,-76.5439842542418,
-4.20082013374671));
#15934=CARTESIAN_POINT('Ctrl Pts',(-9.70137854017372,-76.3689842542418,
1.74701493417668E-11));
#15935=CARTESIAN_POINT('Ctrl Pts',(-7.27603390512272,-76.1939842542418,
4.20082013377292));
#15936=CARTESIAN_POINT('Ctrl Pts',(-4.85068927007173,-76.0189842542418,
8.40164026752836));
#15937=CARTESIAN_POINT('Ctrl Pts',(1.5129078685785E-11,-75.8439842542418,
8.40164026751963));
#15938=CARTESIAN_POINT('Ctrl Pts',(4.85068927010198,-75.6689842542418,8.4016402675109));
#15939=CARTESIAN_POINT('Ctrl Pts',(7.27603390513785,-75.4939842542418,4.20082013374672));
#15940=CARTESIAN_POINT('Ctrl Pts',(9.70137854017372,-75.3189842542418,-1.74689612655491E-11));
#15941=CARTESIAN_POINT('Ctrl Pts',(7.27603390512273,-75.1439842542418,-4.20082013377291));
#15942=CARTESIAN_POINT('Ctrl Pts',(4.85068927007173,-74.9689842542418,-8.40164026752836));
#15943=CARTESIAN_POINT('Ctrl Pts',(-1.51301075899711E-11,-74.7939842542418,
-8.40164026751963));
#15944=CARTESIAN_POINT('Ctrl Pts',(-4.85068927010199,-74.6189842542418,
-8.4016402675109));
#15945=CARTESIAN_POINT('Ctrl Pts',(-7.27603390513785,-74.4439842542418,
-4.20082013374671));
#15946=CARTESIAN_POINT('Ctrl Pts',(-9.70137854017372,-74.2689842542418,
1.74701493417668E-11));
#15947=CARTESIAN_POINT('Ctrl Pts',(-7.27603390512272,-74.0939842542418,
4.20082013377292));
#15948=CARTESIAN_POINT('Ctrl Pts',(-4.85068927007173,-73.9189842542418,
8.40164026752836));
#15949=CARTESIAN_POINT('Ctrl Pts',(1.5129078685785E-11,-73.7439842542418,
8.40164026751963));
#15950=CARTESIAN_POINT('Ctrl Pts',(4.85068927010198,-73.5689842542418,8.4016402675109));
#15951=CARTESIAN_POINT('Ctrl Pts',(7.27603390513785,-73.3939842542418,4.20082013374672));
#15952=CARTESIAN_POINT('Ctrl Pts',(9.70137854017372,-73.2189842542418,-1.74689612655491E-11));
#15953=CARTESIAN_POINT('Ctrl Pts',(7.27603390512273,-73.0439842542418,-4.20082013377291));
#15954=CARTESIAN_POINT('Ctrl Pts',(4.85068927007173,-72.8689842542418,-8.40164026752836));
#15955=CARTESIAN_POINT('Ctrl Pts',(-1.51301075899711E-11,-72.6939842542418,
-8.40164026751963));
#15956=CARTESIAN_POINT('Ctrl Pts',(-4.85068927010199,-72.5189842542418,
-8.4016402675109));
#15957=CARTESIAN_POINT('Ctrl Pts',(-7.27603390513785,-72.3439842542418,
-4.20082013374671));
#15958=CARTESIAN_POINT('Ctrl Pts',(-9.70137854017372,-72.1689842542418,
1.74701493417668E-11));
#15959=CARTESIAN_POINT('Ctrl Pts',(-7.27603390512272,-71.9939842542418,
4.20082013377292));
#15960=CARTESIAN_POINT('Ctrl Pts',(-4.85068927007173,-71.8189842542418,
8.40164026752836));
#15961=CARTESIAN_POINT('Ctrl Pts',(1.5129078685785E-11,-71.6439842542418,
8.40164026751963));
#15962=CARTESIAN_POINT('Ctrl Pts',(4.85068927010198,-71.4689842542418,8.4016402675109));
#15963=CARTESIAN_POINT('Ctrl Pts',(7.27603390513785,-71.2939842542418,4.20082013374672));
#15964=CARTESIAN_POINT('Ctrl Pts',(9.70137854017372,-71.1189842542418,-1.74689612655491E-11));
#15965=CARTESIAN_POINT('Ctrl Pts',(7.27603390512273,-70.9439842542418,-4.20082013377291));
#15966=CARTESIAN_POINT('Ctrl Pts',(4.85068927007173,-70.7689842542418,-8.40164026752836));
#15967=CARTESIAN_POINT('Ctrl Pts',(-1.51301075899711E-11,-70.5939842542418,
-8.40164026751963));
#15968=CARTESIAN_POINT('Ctrl Pts',(-4.85068927010199,-70.4189842542418,
-8.4016402675109));
#15969=CARTESIAN_POINT('Ctrl Pts',(-7.27603390513785,-70.2439842542418,
-4.20082013374671));
#15970=CARTESIAN_POINT('Ctrl Pts',(-9.70137854017372,-70.0689842542418,
1.74701493417668E-11));
#15971=CARTESIAN_POINT('Ctrl Pts',(-7.27603390512272,-69.8939842542418,
4.20082013377292));
#15972=CARTESIAN_POINT('Ctrl Pts',(-4.85068927007173,-69.7189842542418,
8.40164026752836));
#15973=CARTESIAN_POINT('Ctrl Pts',(1.5129078685785E-11,-69.5439842542418,
8.40164026751963));
#15974=CARTESIAN_POINT('Ctrl Pts',(4.85068927010198,-69.3689842542418,8.4016402675109));
#15975=CARTESIAN_POINT('Ctrl Pts',(7.27603390513785,-69.1939842542418,4.20082013374672));
#15976=CARTESIAN_POINT('Ctrl Pts',(9.70137854017372,-69.0189842542418,-1.74689612655491E-11));
#15977=CARTESIAN_POINT('Ctrl Pts',(7.27603390512273,-68.8439842542418,-4.20082013377291));
#15978=CARTESIAN_POINT('Ctrl Pts',(4.85068927007173,-68.6689842542418,-8.40164026752836));
#15979=CARTESIAN_POINT('Ctrl Pts',(-1.51301075899711E-11,-68.4939842542418,
-8.40164026751963));
#15980=CARTESIAN_POINT('Ctrl Pts',(-4.85068927010199,-68.3189842542418,
-8.4016402675109));
#15981=CARTESIAN_POINT('Ctrl Pts',(-7.27603390513785,-68.1439842542418,
-4.20082013374671));
#15982=CARTESIAN_POINT('Ctrl Pts',(-9.70137854017372,-67.9689842542418,
1.74701493417668E-11));
#15983=CARTESIAN_POINT('Ctrl Pts',(-7.27603390512272,-67.7939842542418,
4.20082013377292));
#15984=CARTESIAN_POINT('Ctrl Pts',(-4.85068927007173,-67.6189842542418,
8.40164026752836));
#15985=CARTESIAN_POINT('Ctrl Pts',(1.5129078685785E-11,-67.4439842542418,
8.40164026751963));
#15986=CARTESIAN_POINT('Ctrl Pts',(4.85068927010198,-67.2689842542418,8.4016402675109));
#15987=CARTESIAN_POINT('Ctrl Pts',(7.27603390513785,-67.0939842542418,4.20082013374672));
#15988=CARTESIAN_POINT('Ctrl Pts',(9.70137854017372,-66.9189842542418,-1.74689612655491E-11));
#15989=CARTESIAN_POINT('Ctrl Pts',(7.27603390512273,-66.7439842542418,-4.20082013377291));
#15990=CARTESIAN_POINT('Ctrl Pts',(4.85068927007173,-66.5689842542419,-8.40164026752836));
#15991=CARTESIAN_POINT('Ctrl Pts',(-1.51301075899711E-11,-66.3939842542418,
-8.40164026751963));
#15992=CARTESIAN_POINT('Ctrl Pts',(-4.85068927010199,-66.2189842542418,
-8.4016402675109));
#15993=CARTESIAN_POINT('Ctrl Pts',(-7.27603390513785,-66.0439842542418,
-4.20082013374671));
#15994=CARTESIAN_POINT('Ctrl Pts',(-9.70137854017372,-65.8689842542418,
1.74701493417668E-11));
#15995=CARTESIAN_POINT('Ctrl Pts',(-7.27603390512272,-65.6939842542418,
4.20082013377292));
#15996=CARTESIAN_POINT('Ctrl Pts',(-4.85068927007173,-65.5189842542418,
8.40164026752836));
#15997=CARTESIAN_POINT('Ctrl Pts',(1.5129078685785E-11,-65.3439842542418,
8.40164026751963));
#15998=CARTESIAN_POINT('Ctrl Pts',(4.85068927010198,-65.1689842542418,8.4016402675109));
#15999=CARTESIAN_POINT('Ctrl Pts',(7.27603390513785,-64.9939842542418,4.20082013374672));
#16000=CARTESIAN_POINT('Ctrl Pts',(9.70137854017372,-64.8189842542418,-1.74689612655491E-11));
#16001=CARTESIAN_POINT('Ctrl Pts',(7.27603390512273,-64.6439842542418,-4.20082013377291));
#16002=CARTESIAN_POINT('Ctrl Pts',(4.85068927007173,-64.4689842542418,-8.40164026752836));
#16003=CARTESIAN_POINT('Ctrl Pts',(-1.51301075899711E-11,-64.2939842542418,
-8.40164026751963));
#16004=CARTESIAN_POINT('Ctrl Pts',(-4.85068927010199,-64.1189842542418,
-8.4016402675109));
#16005=CARTESIAN_POINT('Ctrl Pts',(-7.27603390513785,-63.9439842542418,
-4.20082013374671));
#16006=CARTESIAN_POINT('Ctrl Pts',(-9.70137854017372,-63.7689842542418,
1.74701493417668E-11));
#16007=CARTESIAN_POINT('Ctrl Pts',(-7.27603390512272,-63.5939842542418,
4.20082013377292));
#16008=CARTESIAN_POINT('Ctrl Pts',(-4.85068927007173,-63.4189842542418,
8.40164026752836));
#16009=CARTESIAN_POINT('Ctrl Pts',(1.5129078685785E-11,-63.2439842542418,
8.40164026751963));
#16010=CARTESIAN_POINT('Ctrl Pts',(4.85068927010198,-63.0689842542418,8.4016402675109));
#16011=CARTESIAN_POINT('Ctrl Pts',(7.27603390513785,-62.8939842542418,4.20082013374672));
#16012=CARTESIAN_POINT('Ctrl Pts',(9.70137854017372,-62.7189842542418,-1.74689612655491E-11));
#16013=CARTESIAN_POINT('Ctrl Pts',(7.27603390512273,-62.5439842542418,-4.20082013377291));
#16014=CARTESIAN_POINT('Ctrl Pts',(4.85068927007173,-62.3689842542419,-8.40164026752836));
#16015=CARTESIAN_POINT('Ctrl Pts',(-1.51301075899711E-11,-62.1939842542418,
-8.40164026751963));
#16016=CARTESIAN_POINT('Ctrl Pts',(-4.85068927010199,-62.0189842542418,
-8.4016402675109));
#16017=CARTESIAN_POINT('Ctrl Pts',(-7.27603390513785,-61.8439842542418,
-4.20082013374671));
#16018=CARTESIAN_POINT('Ctrl Pts',(-9.70137854017372,-61.6689842542418,
1.74701493417668E-11));
#16019=CARTESIAN_POINT('Ctrl Pts',(-7.27603390512272,-61.4939842542418,
4.20082013377292));
#16020=CARTESIAN_POINT('Ctrl Pts',(-4.85068927007173,-61.3189842542419,
8.40164026752836));
#16021=CARTESIAN_POINT('Ctrl Pts',(1.5129078685785E-11,-61.1439842542418,
8.40164026751963));
#16022=CARTESIAN_POINT('Ctrl Pts',(4.85068927010198,-60.9689842542418,8.4016402675109));
#16023=CARTESIAN_POINT('Ctrl Pts',(7.27603390513785,-60.7939842542418,4.20082013374672));
#16024=CARTESIAN_POINT('Ctrl Pts',(9.70137854017372,-60.6189842542418,-1.74689612655491E-11));
#16025=CARTESIAN_POINT('Ctrl Pts',(7.27603390512273,-60.4439842542418,-4.20082013377291));
#16026=CARTESIAN_POINT('Ctrl Pts',(4.85068927007173,-60.2689842542419,-8.40164026752836));
#16027=CARTESIAN_POINT('Ctrl Pts',(-1.51301075899711E-11,-60.0939842542418,
-8.40164026751963));
#16028=CARTESIAN_POINT('Ctrl Pts',(-4.85068927010199,-59.9189842542418,
-8.4016402675109));
#16029=CARTESIAN_POINT('Ctrl Pts',(-7.27603390513785,-59.7439842542419,
-4.20082013374671));
#16030=CARTESIAN_POINT('Ctrl Pts',(-9.70137854017372,-59.5689842542418,
1.74701493417668E-11));
#16031=CARTESIAN_POINT('Ctrl Pts',(-7.27603390512272,-59.3939842542418,
4.20082013377292));
#16032=CARTESIAN_POINT('Ctrl Pts',(-4.85068927007173,-59.2189842542419,
8.40164026752836));
#16033=CARTESIAN_POINT('Ctrl Pts',(1.5129078685785E-11,-59.0439842542418,
8.40164026751963));
#16034=CARTESIAN_POINT('Ctrl Pts',(4.85068927010198,-58.8689842542419,8.4016402675109));
#16035=CARTESIAN_POINT('Ctrl Pts',(7.27603390513785,-58.6939842542419,4.20082013374672));
#16036=CARTESIAN_POINT('Ctrl Pts',(9.70137854017372,-58.5189842542418,-1.74689612655491E-11));
#16037=CARTESIAN_POINT('Ctrl Pts',(7.27603390512273,-58.3439842542418,-4.20082013377291));
#16038=CARTESIAN_POINT('Ctrl Pts',(4.85068927007173,-58.1689842542419,-8.40164026752836));
#16039=CARTESIAN_POINT('Ctrl Pts',(-1.51301075899711E-11,-57.9939842542418,
-8.40164026751963));
#16040=CARTESIAN_POINT('Ctrl Pts',(-4.85068927010199,-57.8189842542418,
-8.4016402675109));
#16041=CARTESIAN_POINT('Ctrl Pts',(-7.27603390513785,-57.6439842542418,
-4.20082013374671));
#16042=CARTESIAN_POINT('Ctrl Pts',(-9.70137854017372,-57.4689842542418,
1.74701493417668E-11));
#16043=CARTESIAN_POINT('Ctrl Pts',(-7.27603390512272,-57.2939842542418,
4.20082013377292));
#16044=CARTESIAN_POINT('Ctrl Pts',(-4.85068927007173,-57.1189842542418,
8.40164026752836));
#16045=CARTESIAN_POINT('Ctrl Pts',(1.5129078685785E-11,-56.9439842542418,
8.40164026751963));
#16046=CARTESIAN_POINT('Ctrl Pts',(4.85068927010198,-56.7689842542419,8.4016402675109));
#16047=CARTESIAN_POINT('Ctrl Pts',(7.27603390513785,-56.5939842542418,4.20082013374672));
#16048=CARTESIAN_POINT('Ctrl Pts',(9.70137854017372,-56.4189842542418,-1.74689612655491E-11));
#16049=CARTESIAN_POINT('Ctrl Pts',(7.27603390512273,-56.2439842542419,-4.20082013377291));
#16050=CARTESIAN_POINT('Ctrl Pts',(4.85068927007173,-56.0689842542418,-8.40164026752836));
#16051=CARTESIAN_POINT('Ctrl Pts',(-1.51301075899711E-11,-55.8939842542418,
-8.40164026751963));
#16052=CARTESIAN_POINT('Ctrl Pts',(-4.85068927010199,-55.7189842542419,
-8.4016402675109));
#16053=CARTESIAN_POINT('Ctrl Pts',(-7.27603390513785,-55.5439842542418,
-4.20082013374671));
#16054=CARTESIAN_POINT('Ctrl Pts',(-9.70137854017372,-55.3689842542418,
1.74701493417668E-11));
#16055=CARTESIAN_POINT('Ctrl Pts',(-7.27603390512272,-55.1939842542419,
4.20082013377292));
#16056=CARTESIAN_POINT('Ctrl Pts',(-4.85068927007173,-55.0189842542419,
8.40164026752836));
#16057=CARTESIAN_POINT('Ctrl Pts',(1.5129078685785E-11,-54.8439842542419,
8.40164026751963));
#16058=CARTESIAN_POINT('Ctrl Pts',(4.85068927010198,-54.6689842542418,8.4016402675109));
#16059=CARTESIAN_POINT('Ctrl Pts',(7.27603390513785,-54.4939842542419,4.20082013374672));
#16060=CARTESIAN_POINT('Ctrl Pts',(9.70137854017372,-54.3189842542419,-1.74689612655491E-11));
#16061=CARTESIAN_POINT('Ctrl Pts',(7.27603390512273,-54.1439842542419,-4.20082013377291));
#16062=CARTESIAN_POINT('Ctrl Pts',(4.85068927007173,-53.9689842542419,-8.40164026752836));
#16063=CARTESIAN_POINT('Ctrl Pts',(-1.51301075899711E-11,-53.7939842542419,
-8.40164026751963));
#16064=CARTESIAN_POINT('Ctrl Pts',(-4.85068927010199,-53.6189842542419,
-8.4016402675109));
#16065=CARTESIAN_POINT('Ctrl Pts',(-7.27603390513785,-53.4439842542418,
-4.20082013374671));
#16066=CARTESIAN_POINT('Ctrl Pts',(-9.70137854017372,-53.2689842542418,
1.74701493417668E-11));
#16067=CARTESIAN_POINT('Ctrl Pts',(-7.27603390512272,-53.0939842542418,
4.20082013377292));
#16068=CARTESIAN_POINT('Ctrl Pts',(-4.85068927007173,-52.9189842542419,
8.40164026752836));
#16069=CARTESIAN_POINT('Ctrl Pts',(1.5129078685785E-11,-52.7439842542418,
8.40164026751963));
#16070=CARTESIAN_POINT('Ctrl Pts',(4.85068927010198,-52.5689842542419,8.4016402675109));
#16071=CARTESIAN_POINT('Ctrl Pts',(7.27603390513785,-52.3939842542419,4.20082013374672));
#16072=CARTESIAN_POINT('Ctrl Pts',(9.70137854017372,-52.2189842542419,-1.74689612655491E-11));
#16073=CARTESIAN_POINT('Ctrl Pts',(7.27603390512273,-52.0439842542418,-4.20082013377291));
#16074=CARTESIAN_POINT('Ctrl Pts',(4.85068927007173,-51.8689842542419,-8.40164026752836));
#16075=CARTESIAN_POINT('Ctrl Pts',(-1.51301075899711E-11,-51.6939842542418,
-8.40164026751963));
#16076=CARTESIAN_POINT('Ctrl Pts',(-4.85068927010199,-51.5189842542419,
-8.4016402675109));
#16077=CARTESIAN_POINT('Ctrl Pts',(-7.27603390513785,-51.3439842542419,
-4.20082013374671));
#16078=CARTESIAN_POINT('Ctrl Pts',(-9.70137854017372,-51.1689842542419,
1.74701493417668E-11));
#16079=CARTESIAN_POINT('Ctrl Pts',(-7.27603390512272,-50.9939842542419,
4.20082013377292));
#16080=CARTESIAN_POINT('Ctrl Pts',(-4.85068927007173,-50.8189842542419,
8.40164026752836));
#16081=CARTESIAN_POINT('Ctrl Pts',(1.5129078685785E-11,-50.6439842542419,
8.40164026751963));
#16082=CARTESIAN_POINT('Ctrl Pts',(4.85068927010198,-50.4689842542419,8.4016402675109));
#16083=CARTESIAN_POINT('Ctrl Pts',(7.27603390513785,-50.2939842542418,4.20082013374672));
#16084=CARTESIAN_POINT('Ctrl Pts',(9.70137854017372,-50.1189842542419,-1.74689612655491E-11));
#16085=CARTESIAN_POINT('Ctrl Pts',(7.27603390512273,-49.9439842542419,-4.20082013377291));
#16086=CARTESIAN_POINT('Ctrl Pts',(4.85068927007173,-49.7689842542419,-8.40164026752836));
#16087=CARTESIAN_POINT('Ctrl Pts',(-1.51301075899711E-11,-49.5939842542419,
-8.40164026751963));
#16088=CARTESIAN_POINT('Ctrl Pts',(-4.85068927010199,-49.4189842542419,
-8.4016402675109));
#16089=CARTESIAN_POINT('Ctrl Pts',(-7.27603390513785,-49.2439842542419,
-4.20082013374671));
#16090=CARTESIAN_POINT('Ctrl Pts',(-9.70137854017372,-49.0689842542419,
1.74701493417668E-11));
#16091=CARTESIAN_POINT('Ctrl Pts',(-7.27603390512272,-48.8939842542419,
4.20082013377292));
#16092=CARTESIAN_POINT('Ctrl Pts',(-4.85068927007173,-48.7189842542419,
8.40164026752836));
#16093=CARTESIAN_POINT('Ctrl Pts',(1.5129078685785E-11,-48.5439842542419,
8.40164026751963));
#16094=CARTESIAN_POINT('Ctrl Pts',(4.85068927010198,-48.3689842542419,8.4016402675109));
#16095=CARTESIAN_POINT('Ctrl Pts',(7.27603390513785,-48.1939842542419,4.20082013374672));
#16096=CARTESIAN_POINT('Ctrl Pts',(9.70137854017372,-48.0189842542419,-1.74689612655491E-11));
#16097=CARTESIAN_POINT('Ctrl Pts',(7.27603390512273,-47.8439842542419,-4.20082013377291));
#16098=CARTESIAN_POINT('Ctrl Pts',(4.85068927007173,-47.6689842542419,-8.40164026752836));
#16099=CARTESIAN_POINT('Ctrl Pts',(-1.51301075899711E-11,-47.4939842542419,
-8.40164026751963));
#16100=CARTESIAN_POINT('Ctrl Pts',(-4.85068927010199,-47.3189842542419,
-8.4016402675109));
#16101=CARTESIAN_POINT('Ctrl Pts',(-7.27603390513785,-47.1439842542419,
-4.20082013374671));
#16102=CARTESIAN_POINT('Ctrl Pts',(-9.70137854017372,-46.9689842542419,
1.74701493417668E-11));
#16103=CARTESIAN_POINT('Ctrl Pts',(-7.27603390512272,-46.7939842542419,
4.20082013377292));
#16104=CARTESIAN_POINT('Ctrl Pts',(-4.85068927007173,-46.6189842542419,
8.40164026752836));
#16105=CARTESIAN_POINT('Ctrl Pts',(1.5129078685785E-11,-46.4439842542419,
8.40164026751963));
#16106=CARTESIAN_POINT('Ctrl Pts',(4.85068927010198,-46.2689842542419,8.4016402675109));
#16107=CARTESIAN_POINT('Ctrl Pts',(7.27603390513785,-46.0939842542419,4.20082013374672));
#16108=CARTESIAN_POINT('Ctrl Pts',(9.70137854017372,-45.9189842542419,-1.74689612655491E-11));
#16109=CARTESIAN_POINT('Ctrl Pts',(7.27603390512273,-45.7439842542419,-4.20082013377291));
#16110=CARTESIAN_POINT('Ctrl Pts',(4.85068927007173,-45.5689842542419,-8.40164026752836));
#16111=CARTESIAN_POINT('Ctrl Pts',(-1.51301075899711E-11,-45.3939842542419,
-8.40164026751963));
#16112=CARTESIAN_POINT('Ctrl Pts',(-4.85068927010199,-45.2189842542419,
-8.4016402675109));
#16113=CARTESIAN_POINT('Ctrl Pts',(-7.27603390513785,-45.0439842542419,
-4.20082013374671));
#16114=CARTESIAN_POINT('Ctrl Pts',(-9.70137854017372,-44.8689842542419,
1.74701493417668E-11));
#16115=CARTESIAN_POINT('Ctrl Pts',(-7.27603390512272,-44.6939842542419,
4.20082013377292));
#16116=CARTESIAN_POINT('Ctrl Pts',(-4.85068927007173,-44.5189842542419,
8.40164026752836));
#16117=CARTESIAN_POINT('Ctrl Pts',(1.5129078685785E-11,-44.3439842542419,
8.40164026751963));
#16118=CARTESIAN_POINT('Ctrl Pts',(4.85068927010198,-44.1689842542419,8.4016402675109));
#16119=CARTESIAN_POINT('Ctrl Pts',(7.27603390513785,-43.9939842542419,4.20082013374672));
#16120=CARTESIAN_POINT('Ctrl Pts',(9.70137854017372,-43.8189842542419,-1.74689612655491E-11));
#16121=CARTESIAN_POINT('Ctrl Pts',(7.27603390512273,-43.6439842542419,-4.20082013377291));
#16122=CARTESIAN_POINT('Ctrl Pts',(4.85068927007173,-43.4689842542419,-8.40164026752836));
#16123=CARTESIAN_POINT('Ctrl Pts',(-1.51301075899711E-11,-43.2939842542419,
-8.40164026751963));
#16124=CARTESIAN_POINT('Ctrl Pts',(-4.85068927010199,-43.1189842542419,
-8.4016402675109));
#16125=CARTESIAN_POINT('Ctrl Pts',(-7.27603390513785,-42.9439842542419,
-4.20082013374671));
#16126=CARTESIAN_POINT('Ctrl Pts',(-9.70137854017372,-42.7689842542419,
1.74701493417668E-11));
#16127=CARTESIAN_POINT('Ctrl Pts',(-7.27603390512272,-42.5939842542419,
4.20082013377292));
#16128=CARTESIAN_POINT('Ctrl Pts',(-4.85068927007173,-42.4189842542419,
8.40164026752836));
#16129=CARTESIAN_POINT('Ctrl Pts',(1.5129078685785E-11,-42.2439842542419,
8.40164026751963));
#16130=CARTESIAN_POINT('Ctrl Pts',(4.85068927010198,-42.0689842542419,8.4016402675109));
#16131=CARTESIAN_POINT('Ctrl Pts',(7.27603390513785,-41.8939842542419,4.20082013374672));
#16132=CARTESIAN_POINT('Ctrl Pts',(9.70137854017372,-41.7189842542419,-1.74689612655491E-11));
#16133=CARTESIAN_POINT('Ctrl Pts',(7.27603390512273,-41.5439842542419,-4.20082013377291));
#16134=CARTESIAN_POINT('Ctrl Pts',(4.85068927007173,-41.3689842542419,-8.40164026752836));
#16135=CARTESIAN_POINT('Ctrl Pts',(-1.51301075899711E-11,-41.1939842542419,
-8.40164026751963));
#16136=CARTESIAN_POINT('Ctrl Pts',(-4.85068927010199,-41.0189842542419,
-8.4016402675109));
#16137=CARTESIAN_POINT('Ctrl Pts',(-7.27603390513785,-40.8439842542419,
-4.20082013374671));
#16138=CARTESIAN_POINT('Ctrl Pts',(-9.70137854017372,-40.6689842542419,
1.74701493417668E-11));
#16139=CARTESIAN_POINT('Ctrl Pts',(-7.27603390512272,-40.4939842542419,
4.20082013377292));
#16140=CARTESIAN_POINT('Ctrl Pts',(-4.85068927007173,-40.3189842542419,
8.40164026752836));
#16141=CARTESIAN_POINT('Ctrl Pts',(1.5129078685785E-11,-40.1439842542419,
8.40164026751963));
#16142=CARTESIAN_POINT('Ctrl Pts',(4.85068927010198,-39.9689842542419,8.4016402675109));
#16143=CARTESIAN_POINT('Ctrl Pts',(7.27603390513785,-39.7939842542419,4.20082013374672));
#16144=CARTESIAN_POINT('Ctrl Pts',(9.70137854017372,-39.6189842542419,-1.74689612655491E-11));
#16145=CARTESIAN_POINT('Ctrl Pts',(7.27603390512273,-39.4439842542419,-4.20082013377291));
#16146=CARTESIAN_POINT('Ctrl Pts',(4.85068927007173,-39.2689842542419,-8.40164026752836));
#16147=CARTESIAN_POINT('Ctrl Pts',(-1.51301075899711E-11,-39.0939842542419,
-8.40164026751963));
#16148=CARTESIAN_POINT('Ctrl Pts',(-4.85068927010199,-38.9189842542419,
-8.4016402675109));
#16149=CARTESIAN_POINT('Ctrl Pts',(-7.27603390513785,-38.7439842542419,
-4.20082013374671));
#16150=CARTESIAN_POINT('Ctrl Pts',(-9.70137854017372,-38.5689842542419,
1.74701493417668E-11));
#16151=CARTESIAN_POINT('Ctrl Pts',(-7.27603390512272,-38.3939842542419,
4.20082013377292));
#16152=CARTESIAN_POINT('Ctrl Pts',(-4.85068927007173,-38.2189842542419,
8.40164026752836));
#16153=CARTESIAN_POINT('Ctrl Pts',(1.5129078685785E-11,-38.0439842542419,
8.40164026751963));
#16154=CARTESIAN_POINT('Ctrl Pts',(4.85068927010198,-37.8689842542419,8.4016402675109));
#16155=CARTESIAN_POINT('Ctrl Pts',(7.27603390513785,-37.6939842542419,4.20082013374672));
#16156=CARTESIAN_POINT('Ctrl Pts',(9.70137854017372,-37.5189842542419,-1.74689612655491E-11));
#16157=CARTESIAN_POINT('Ctrl Pts',(7.27603390512273,-37.3439842542419,-4.20082013377291));
#16158=CARTESIAN_POINT('Ctrl Pts',(4.85068927007173,-37.1689842542419,-8.40164026752836));
#16159=CARTESIAN_POINT('Ctrl Pts',(-1.51301075899711E-11,-36.9939842542419,
-8.40164026751963));
#16160=CARTESIAN_POINT('Ctrl Pts',(-4.85068927010199,-36.8189842542419,
-8.4016402675109));
#16161=CARTESIAN_POINT('Ctrl Pts',(-7.27603390513785,-36.6439842542419,
-4.20082013374671));
#16162=CARTESIAN_POINT('Ctrl Pts',(-9.70137854017372,-36.4689842542419,
1.74701493417668E-11));
#16163=CARTESIAN_POINT('Ctrl Pts',(-7.27603390512272,-36.2939842542419,
4.20082013377292));
#16164=CARTESIAN_POINT('Ctrl Pts',(-4.85068927007173,-36.1189842542419,
8.40164026752836));
#16165=CARTESIAN_POINT('Ctrl Pts',(1.5129078685785E-11,-35.9439842542419,
8.40164026751963));
#16166=CARTESIAN_POINT('Ctrl Pts',(4.85068927010198,-35.7689842542419,8.4016402675109));
#16167=CARTESIAN_POINT('Ctrl Pts',(7.27603390513785,-35.5939842542419,4.20082013374672));
#16168=CARTESIAN_POINT('Ctrl Pts',(9.70137854017372,-35.4189842542419,-1.74689612655491E-11));
#16169=CARTESIAN_POINT('Ctrl Pts',(7.27603390512273,-35.2439842542419,-4.20082013377291));
#16170=CARTESIAN_POINT('Ctrl Pts',(4.85068927007173,-35.0689842542419,-8.40164026752836));
#16171=CARTESIAN_POINT('Ctrl Pts',(-1.51301075899711E-11,-34.8939842542419,
-8.40164026751963));
#16172=CARTESIAN_POINT('Ctrl Pts',(-4.85068927010199,-34.7189842542419,
-8.4016402675109));
#16173=CARTESIAN_POINT('Ctrl Pts',(-7.27603390513785,-34.5439842542419,
-4.20082013374671));
#16174=CARTESIAN_POINT('Ctrl Pts',(-9.70137854017372,-34.3689842542419,
1.74701493417668E-11));
#16175=CARTESIAN_POINT('Ctrl Pts',(-7.27603390512272,-34.1939842542419,
4.20082013377292));
#16176=CARTESIAN_POINT('Ctrl Pts',(-4.85068927007173,-34.0189842542419,
8.40164026752836));
#16177=CARTESIAN_POINT('Ctrl Pts',(1.5129078685785E-11,-33.8439842542419,
8.40164026751963));
#16178=CARTESIAN_POINT('Ctrl Pts',(4.85068927010198,-33.6689842542419,8.4016402675109));
#16179=CARTESIAN_POINT('Ctrl Pts',(7.27603390513785,-33.4939842542419,4.20082013374672));
#16180=CARTESIAN_POINT('Ctrl Pts',(9.70137854017372,-33.3189842542419,-1.74689612655491E-11));
#16181=CARTESIAN_POINT('Ctrl Pts',(7.27603390512273,-33.1439842542419,-4.20082013377291));
#16182=CARTESIAN_POINT('Ctrl Pts',(4.85068927007173,-32.9689842542419,-8.40164026752836));
#16183=CARTESIAN_POINT('Ctrl Pts',(-1.51301075899711E-11,-32.7939842542419,
-8.40164026751963));
#16184=CARTESIAN_POINT('Ctrl Pts',(-4.85068927010199,-32.6189842542419,
-8.4016402675109));
#16185=CARTESIAN_POINT('Ctrl Pts',(-7.27603390513785,-32.4439842542419,
-4.20082013374671));
#16186=CARTESIAN_POINT('Ctrl Pts',(-9.70137854017372,-32.2689842542419,
1.74701493417668E-11));
#16187=CARTESIAN_POINT('Ctrl Pts',(-7.27603390512272,-32.0939842542419,
4.20082013377292));
#16188=CARTESIAN_POINT('Ctrl Pts',(-4.85068927007173,-31.9189842542419,
8.40164026752836));
#16189=CARTESIAN_POINT('Ctrl Pts',(1.5129078685785E-11,-31.7439842542419,
8.40164026751963));
#16190=CARTESIAN_POINT('Ctrl Pts',(4.85068927010198,-31.5689842542419,8.4016402675109));
#16191=CARTESIAN_POINT('Ctrl Pts',(7.27603390513785,-31.3939842542419,4.20082013374672));
#16192=CARTESIAN_POINT('Ctrl Pts',(9.70137854017372,-31.2189842542419,-1.74689612655491E-11));
#16193=CARTESIAN_POINT('Ctrl Pts',(7.27603390512273,-31.0439842542419,-4.20082013377291));
#16194=CARTESIAN_POINT('Ctrl Pts',(4.85068927007173,-30.8689842542419,-8.40164026752836));
#16195=CARTESIAN_POINT('Ctrl Pts',(-1.51301075899711E-11,-30.6939842542419,
-8.40164026751963));
#16196=CARTESIAN_POINT('Ctrl Pts',(-4.85068927010199,-30.5189842542419,
-8.4016402675109));
#16197=CARTESIAN_POINT('Ctrl Pts',(-7.27603390513785,-30.3439842542419,
-4.20082013374671));
#16198=CARTESIAN_POINT('Ctrl Pts',(-9.70137854017372,-30.1689842542419,
1.74701493417668E-11));
#16199=CARTESIAN_POINT('Ctrl Pts',(-7.27603390512272,-29.9939842542419,
4.20082013377292));
#16200=CARTESIAN_POINT('Ctrl Pts',(-4.85068927007173,-29.8189842542419,
8.40164026752836));
#16201=CARTESIAN_POINT('Ctrl Pts',(1.5129078685785E-11,-29.6439842542419,
8.40164026751963));
#16202=CARTESIAN_POINT('Ctrl Pts',(4.85068927010198,-29.4689842542419,8.4016402675109));
#16203=CARTESIAN_POINT('Ctrl Pts',(7.27603390513785,-29.2939842542419,4.20082013374672));
#16204=CARTESIAN_POINT('Ctrl Pts',(9.70137854017372,-29.1189842542419,-1.74689612655491E-11));
#16205=CARTESIAN_POINT('Ctrl Pts',(7.27603390512273,-28.9439842542419,-4.20082013377291));
#16206=CARTESIAN_POINT('Ctrl Pts',(4.85068927007173,-28.7689842542419,-8.40164026752836));
#16207=CARTESIAN_POINT('Ctrl Pts',(-1.51301075899711E-11,-28.5939842542419,
-8.40164026751963));
#16208=CARTESIAN_POINT('Ctrl Pts',(-4.85068927010199,-28.4189842542419,
-8.4016402675109));
#16209=CARTESIAN_POINT('Ctrl Pts',(-7.27603390513785,-28.2439842542419,
-4.20082013374671));
#16210=CARTESIAN_POINT('Ctrl Pts',(-9.70137854017372,-28.0689842542419,
1.74701493417668E-11));
#16211=CARTESIAN_POINT('Ctrl Pts',(-7.27603390512272,-27.8939842542419,
4.20082013377292));
#16212=CARTESIAN_POINT('Ctrl Pts',(-4.85068927007173,-27.7189842542419,
8.40164026752836));
#16213=CARTESIAN_POINT('Ctrl Pts',(1.5129078685785E-11,-27.5439842542419,
8.40164026751963));
#16214=CARTESIAN_POINT('Ctrl Pts',(4.85068927010198,-27.3689842542419,8.4016402675109));
#16215=CARTESIAN_POINT('Ctrl Pts',(7.27603390513785,-27.1939842542419,4.20082013374672));
#16216=CARTESIAN_POINT('Ctrl Pts',(9.70137854017372,-27.0189842542419,-1.74689612655491E-11));
#16217=CARTESIAN_POINT('Ctrl Pts',(7.27603390512273,-26.8439842542419,-4.20082013377291));
#16218=CARTESIAN_POINT('Ctrl Pts',(4.85068927007173,-26.6689842542419,-8.40164026752836));
#16219=CARTESIAN_POINT('Ctrl Pts',(-1.51301075899711E-11,-26.4939842542419,
-8.40164026751963));
#16220=CARTESIAN_POINT('Ctrl Pts',(-4.85068927010199,-26.3189842542419,
-8.4016402675109));
#16221=CARTESIAN_POINT('Ctrl Pts',(-7.27603390513785,-26.1439842542419,
-4.20082013374671));
#16222=CARTESIAN_POINT('Ctrl Pts',(-9.70137854017372,-25.9689842542419,
1.74701493417668E-11));
#16223=CARTESIAN_POINT('Ctrl Pts',(-7.27603390512272,-25.7939842542419,
4.20082013377292));
#16224=CARTESIAN_POINT('Ctrl Pts',(-4.85068927007173,-25.6189842542419,
8.40164026752836));
#16225=CARTESIAN_POINT('Ctrl Pts',(1.5129078685785E-11,-25.4439842542419,
8.40164026751963));
#16226=CARTESIAN_POINT('Ctrl Pts',(4.85068927010198,-25.2689842542419,8.4016402675109));
#16227=CARTESIAN_POINT('Ctrl Pts',(7.27603390513785,-25.0939842542419,4.20082013374672));
#16228=CARTESIAN_POINT('Ctrl Pts',(9.70137854017372,-24.9189842542419,-1.74689612655491E-11));
#16229=CARTESIAN_POINT('Ctrl Pts',(7.27603390512273,-24.7439842542419,-4.20082013377291));
#16230=CARTESIAN_POINT('Ctrl Pts',(4.85068927007173,-24.5689842542419,-8.40164026752836));
#16231=CARTESIAN_POINT('Ctrl Pts',(-1.51301075899711E-11,-24.3939842542419,
-8.40164026751963));
#16232=CARTESIAN_POINT('Ctrl Pts',(-4.85068927010199,-24.2189842542419,
-8.4016402675109));
#16233=CARTESIAN_POINT('Ctrl Pts',(-7.27603390513785,-24.0439842542419,
-4.20082013374671));
#16234=CARTESIAN_POINT('Ctrl Pts',(-9.70137854017372,-23.8689842542419,
1.74701493417668E-11));
#16235=CARTESIAN_POINT('Ctrl Pts',(-7.27603390512272,-23.6939842542419,
4.20082013377292));
#16236=CARTESIAN_POINT('Ctrl Pts',(-4.85068927007173,-23.5189842542419,
8.40164026752836));
#16237=CARTESIAN_POINT('Ctrl Pts',(1.5129078685785E-11,-23.3439842542419,
8.40164026751963));
#16238=CARTESIAN_POINT('Ctrl Pts',(4.85068927010198,-23.1689842542419,8.4016402675109));
#16239=CARTESIAN_POINT('Ctrl Pts',(7.27603390513785,-22.9939842542419,4.20082013374672));
#16240=CARTESIAN_POINT('Ctrl Pts',(9.70137854017372,-22.8189842542419,-1.74689612655491E-11));
#16241=CARTESIAN_POINT('Ctrl Pts',(7.27603390512273,-22.6439842542419,-4.20082013377291));
#16242=CARTESIAN_POINT('Ctrl Pts',(4.85068927007173,-22.4689842542419,-8.40164026752836));
#16243=CARTESIAN_POINT('Ctrl Pts',(-1.51301075899711E-11,-22.2939842542419,
-8.40164026751963));
#16244=CARTESIAN_POINT('Ctrl Pts',(-4.85068927010199,-22.1189842542419,
-8.4016402675109));
#16245=CARTESIAN_POINT('Ctrl Pts',(-7.27603390513785,-21.9439842542419,
-4.20082013374671));
#16246=CARTESIAN_POINT('Ctrl Pts',(-9.70137854017372,-21.7689842542419,
1.74701493417668E-11));
#16247=CARTESIAN_POINT('Ctrl Pts',(-7.27603390512272,-21.5939842542419,
4.20082013377292));
#16248=CARTESIAN_POINT('Ctrl Pts',(-4.85068927007173,-21.4189842542419,
8.40164026752836));
#16249=CARTESIAN_POINT('Ctrl Pts',(1.5129078685785E-11,-21.2439842542419,
8.40164026751963));
#16250=CARTESIAN_POINT('Ctrl Pts',(4.85068927010198,-21.0689842542419,8.4016402675109));
#16251=CARTESIAN_POINT('Ctrl Pts',(7.27603390513785,-20.8939842542419,4.20082013374672));
#16252=CARTESIAN_POINT('Ctrl Pts',(9.70137854017372,-20.7189842542419,-1.74689612655491E-11));
#16253=CARTESIAN_POINT('Ctrl Pts',(7.27603390512273,-20.5439842542419,-4.20082013377291));
#16254=CARTESIAN_POINT('Ctrl Pts',(4.85068927007173,-20.3689842542419,-8.40164026752836));
#16255=CARTESIAN_POINT('Ctrl Pts',(-1.51301075899711E-11,-20.1939842542419,
-8.40164026751963));
#16256=CARTESIAN_POINT('Ctrl Pts',(-4.85068927010199,-20.0189842542419,
-8.4016402675109));
#16257=CARTESIAN_POINT('Ctrl Pts',(-7.27603390513785,-19.8439842542419,
-4.20082013374671));
#16258=CARTESIAN_POINT('Ctrl Pts',(-9.70137854017372,-19.6689842542419,
1.74701493417668E-11));
#16259=CARTESIAN_POINT('Ctrl Pts',(-7.27603390512272,-19.4939842542419,
4.20082013377292));
#16260=CARTESIAN_POINT('Ctrl Pts',(-4.85068927007173,-19.3189842542419,
8.40164026752836));
#16261=CARTESIAN_POINT('Ctrl Pts',(1.5129078685785E-11,-19.1439842542419,
8.40164026751963));
#16262=CARTESIAN_POINT('Ctrl Pts',(4.85068927010198,-18.9689842542419,8.4016402675109));
#16263=CARTESIAN_POINT('Ctrl Pts',(7.27603390513785,-18.7939842542419,4.20082013374672));
#16264=CARTESIAN_POINT('Ctrl Pts',(9.70137854017372,-18.6189842542419,-1.74689612655491E-11));
#16265=CARTESIAN_POINT('Ctrl Pts',(7.27603390512273,-18.4439842542419,-4.20082013377291));
#16266=CARTESIAN_POINT('Ctrl Pts',(4.85068927007173,-18.2689842542419,-8.40164026752836));
#16267=CARTESIAN_POINT('Ctrl Pts',(-1.51301075899711E-11,-18.0939842542419,
-8.40164026751963));
#16268=CARTESIAN_POINT('Ctrl Pts',(-4.85068927010199,-17.9189842542419,
-8.4016402675109));
#16269=CARTESIAN_POINT('Ctrl Pts',(-7.27603390513785,-17.7439842542419,
-4.20082013374671));
#16270=CARTESIAN_POINT('Ctrl Pts',(-9.70137854017372,-17.5689842542419,
1.74701493417668E-11));
#16271=CARTESIAN_POINT('Ctrl Pts',(-7.27603390512272,-17.3939842542419,
4.20082013377292));
#16272=CARTESIAN_POINT('Ctrl Pts',(-4.85068927007173,-17.2189842542419,
8.40164026752836));
#16273=CARTESIAN_POINT('Ctrl Pts',(1.5129078685785E-11,-17.0439842542419,
8.40164026751963));
#16274=CARTESIAN_POINT('Ctrl Pts',(4.85068927010198,-16.8689842542419,8.4016402675109));
#16275=CARTESIAN_POINT('Ctrl Pts',(7.27603390513785,-16.6939842542419,4.20082013374672));
#16276=CARTESIAN_POINT('Ctrl Pts',(9.70137854017372,-16.518984254242,-1.74689612655491E-11));
#16277=CARTESIAN_POINT('Ctrl Pts',(7.27603390512273,-16.3439842542419,-4.20082013377291));
#16278=CARTESIAN_POINT('Ctrl Pts',(4.85068927007173,-16.1689842542419,-8.40164026752836));
#16279=CARTESIAN_POINT('Ctrl Pts',(-1.51301075899711E-11,-15.9939842542419,
-8.40164026751963));
#16280=CARTESIAN_POINT('Ctrl Pts',(-4.85068927010199,-15.8189842542419,
-8.4016402675109));
#16281=CARTESIAN_POINT('Ctrl Pts',(-7.27603390513785,-15.6439842542419,
-4.20082013374671));
#16282=CARTESIAN_POINT('Ctrl Pts',(-9.70137854017372,-15.4689842542419,
1.74701493417668E-11));
#16283=CARTESIAN_POINT('Ctrl Pts',(-7.27603390512272,-15.2939842542419,
4.20082013377292));
#16284=CARTESIAN_POINT('Ctrl Pts',(-4.85068927007173,-15.1189842542419,
8.40164026752836));
#16285=CARTESIAN_POINT('Ctrl Pts',(1.5129078685785E-11,-14.9439842542419,
8.40164026751963));
#16286=CARTESIAN_POINT('Ctrl Pts',(4.85068927010198,-14.7689842542419,8.4016402675109));
#16287=CARTESIAN_POINT('Ctrl Pts',(7.27603390513785,-14.5939842542419,4.20082013374672));
#16288=CARTESIAN_POINT('Ctrl Pts',(9.70137854017372,-14.4189842542419,-1.74689612655491E-11));
#16289=CARTESIAN_POINT('Ctrl Pts',(7.27603390512273,-14.2439842542419,-4.20082013377291));
#16290=CARTESIAN_POINT('Ctrl Pts',(4.85068927007173,-14.0689842542419,-8.40164026752836));
#16291=CARTESIAN_POINT('Ctrl Pts',(-1.51301075899711E-11,-13.8939842542419,
-8.40164026751963));
#16292=CARTESIAN_POINT('Ctrl Pts',(-4.85068927010199,-13.7189842542419,
-8.4016402675109));
#16293=CARTESIAN_POINT('Ctrl Pts',(-7.27603390513785,-13.5439842542419,
-4.20082013374671));
#16294=CARTESIAN_POINT('Ctrl Pts',(-9.70137854017372,-13.3689842542419,
1.74701493417668E-11));
#16295=CARTESIAN_POINT('Ctrl Pts',(-7.27603390512272,-13.193984254242,4.20082013377292));
#16296=CARTESIAN_POINT('Ctrl Pts',(-4.85068927007173,-13.018984254242,8.40164026752836));
#16297=CARTESIAN_POINT('Ctrl Pts',(1.5129078685785E-11,-12.8439842542419,
8.40164026751963));
#16298=CARTESIAN_POINT('Ctrl Pts',(4.85068927010198,-12.668984254242,8.4016402675109));
#16299=CARTESIAN_POINT('Ctrl Pts',(7.27603390513785,-12.4939842542419,4.20082013374672));
#16300=CARTESIAN_POINT('Ctrl Pts',(9.70137854017372,-12.3189842542419,-1.74689612655491E-11));
#16301=CARTESIAN_POINT('Ctrl Pts',(7.27603390512273,-12.143984254242,-4.20082013377291));
#16302=CARTESIAN_POINT('Ctrl Pts',(4.85068927007173,-11.968984254242,-8.40164026752836));
#16303=CARTESIAN_POINT('Ctrl Pts',(-1.51301075899711E-11,-11.7939842542419,
-8.40164026751963));
#16304=CARTESIAN_POINT('Ctrl Pts',(-4.85068927010199,-11.6189842542419,
-8.4016402675109));
#16305=CARTESIAN_POINT('Ctrl Pts',(-7.27603390513785,-11.443984254242,-4.20082013374671));
#16306=CARTESIAN_POINT('Ctrl Pts',(-9.70137854017372,-11.2689842542419,
1.74701493417668E-11));
#16307=CARTESIAN_POINT('Ctrl Pts',(-7.27603390512272,-11.0939842542419,
4.20082013377292));
#16308=CARTESIAN_POINT('Ctrl Pts',(-4.85068927007173,-10.918984254242,8.40164026752836));
#16309=CARTESIAN_POINT('Ctrl Pts',(1.5129078685785E-11,-10.7439842542419,
8.40164026751963));
#16310=CARTESIAN_POINT('Ctrl Pts',(4.85068927010198,-10.5689842542419,8.4016402675109));
#16311=CARTESIAN_POINT('Ctrl Pts',(7.27603390513785,-10.393984254242,4.20082013374672));
#16312=CARTESIAN_POINT('Ctrl Pts',(9.70137854017372,-10.2189842542419,-1.74689612655491E-11));
#16313=CARTESIAN_POINT('Ctrl Pts',(7.27603390512273,-10.0439842542419,-4.20082013377291));
#16314=CARTESIAN_POINT('Ctrl Pts',(4.85068927007173,-9.86898425424196,-8.40164026752836));
#16315=CARTESIAN_POINT('Ctrl Pts',(-1.51301075899711E-11,-9.69398425424195,
-8.40164026751963));
#16316=CARTESIAN_POINT('Ctrl Pts',(-4.85068927010199,-9.51898425424195,
-8.4016402675109));
#16317=CARTESIAN_POINT('Ctrl Pts',(-7.27603390513785,-9.34398425424196,
-4.20082013374671));
#16318=CARTESIAN_POINT('Ctrl Pts',(-9.70137854017372,-9.16898425424195,
1.74701493417668E-11));
#16319=CARTESIAN_POINT('Ctrl Pts',(-7.27603390512272,-8.99398425424194,
4.20082013377292));
#16320=CARTESIAN_POINT('Ctrl Pts',(-4.85068927007173,-8.81898425424197,
8.40164026752836));
#16321=CARTESIAN_POINT('Ctrl Pts',(1.5129078685785E-11,-8.64398425424195,
8.40164026751963));
#16322=CARTESIAN_POINT('Ctrl Pts',(4.85068927010198,-8.46898425424195,8.4016402675109));
#16323=CARTESIAN_POINT('Ctrl Pts',(7.27603390513785,-8.29398425424196,4.20082013374672));
#16324=CARTESIAN_POINT('Ctrl Pts',(9.70137854017372,-8.11898425424196,-1.74689612655491E-11));
#16325=CARTESIAN_POINT('Ctrl Pts',(7.27603390512273,-7.94398425424195,-4.20082013377291));
#16326=CARTESIAN_POINT('Ctrl Pts',(4.85068927007173,-7.76898425424197,-8.40164026752836));
#16327=CARTESIAN_POINT('Ctrl Pts',(-1.51301075899711E-11,-7.59398425424196,
-8.40164026751963));
#16328=CARTESIAN_POINT('Ctrl Pts',(-4.85068927010199,-7.41898425424196,
-8.4016402675109));
#16329=CARTESIAN_POINT('Ctrl Pts',(-7.27603390513785,-7.24398425424194,
-4.20082013374671));
#16330=CARTESIAN_POINT('Ctrl Pts',(-9.70137854017372,-7.06898425424196,
1.74701493417668E-11));
#16331=CARTESIAN_POINT('Ctrl Pts',(-7.27603390512272,-6.89398425424195,
4.20082013377292));
#16332=CARTESIAN_POINT('Ctrl Pts',(-4.85068927007173,-6.71898425424195,
8.40164026752836));
#16333=CARTESIAN_POINT('Ctrl Pts',(1.5129078685785E-11,-6.54398425424196,
8.40164026751963));
#16334=CARTESIAN_POINT('Ctrl Pts',(4.85068927010198,-6.36898425424197,8.4016402675109));
#16335=CARTESIAN_POINT('Ctrl Pts',(7.27603390513785,-6.19398425424195,4.20082013374672));
#16336=CARTESIAN_POINT('Ctrl Pts',(9.70137854017372,-6.01898425424197,-1.74689612655491E-11));
#16337=CARTESIAN_POINT('Ctrl Pts',(7.27603390512273,-5.84398425424196,-4.20082013377291));
#16338=CARTESIAN_POINT('Ctrl Pts',(4.85068927007173,-5.66898425424195,-8.40164026752836));
#16339=CARTESIAN_POINT('Ctrl Pts',(-1.51301075899711E-11,-5.49398425424197,
-8.40164026751963));
#16340=CARTESIAN_POINT('Ctrl Pts',(-4.85068927010199,-5.31898425424197,
-8.4016402675109));
#16341=CARTESIAN_POINT('Ctrl Pts',(-7.27603390513785,-5.14398425424195,
-4.20082013374671));
#16342=CARTESIAN_POINT('Ctrl Pts',(-9.70137854017372,-4.96898425424197,
1.74701493417668E-11));
#16343=CARTESIAN_POINT('Ctrl Pts',(-7.27603390512272,-4.79398425424196,
4.20082013377292));
#16344=CARTESIAN_POINT('Ctrl Pts',(-4.85068927007173,-4.61898425424196,
8.40164026752836));
#16345=CARTESIAN_POINT('Ctrl Pts',(1.5129078685785E-11,-4.44398425424197,
8.40164026751963));
#16346=CARTESIAN_POINT('Ctrl Pts',(4.85068927010198,-4.26898425424197,8.4016402675109));
#16347=CARTESIAN_POINT('Ctrl Pts',(7.27603390513785,-4.09398425424196,4.20082013374672));
#16348=CARTESIAN_POINT('Ctrl Pts',(9.70137854017372,-3.91898425424198,-1.74689612655491E-11));
#16349=CARTESIAN_POINT('Ctrl Pts',(7.27603390512273,-3.74398425424197,-4.20082013377291));
#16350=CARTESIAN_POINT('Ctrl Pts',(4.85068927007173,-3.56898425424196,-8.40164026752836));
#16351=CARTESIAN_POINT('Ctrl Pts',(-1.51301075899711E-11,-3.39398425424198,
-8.40164026751963));
#16352=CARTESIAN_POINT('Ctrl Pts',(-4.85068927010199,-3.21898425424198,
-8.4016402675109));
#16353=CARTESIAN_POINT('Ctrl Pts',(-7.27603390513785,-3.04398425424196,
-4.20082013374671));
#16354=CARTESIAN_POINT('Ctrl Pts',(-9.70137854017372,-2.86898425424196,
1.74701493417668E-11));
#16355=CARTESIAN_POINT('Ctrl Pts',(-7.27603390512272,-2.69398425424197,
4.20082013377292));
#16356=CARTESIAN_POINT('Ctrl Pts',(-4.85068927007173,-2.51898425424196,
8.40164026752836));
#16357=CARTESIAN_POINT('Ctrl Pts',(1.5129078685785E-11,-2.34398425424195,
8.40164026751963));
#16358=CARTESIAN_POINT('Ctrl Pts',(4.85068927010198,-2.16898425424197,8.4016402675109));
#16359=CARTESIAN_POINT('Ctrl Pts',(7.27603390513785,-1.99398425424197,4.20082013374672));
#16360=CARTESIAN_POINT('Ctrl Pts',(9.70137854017372,-1.81898425424196,-1.74689612655491E-11));
#16361=CARTESIAN_POINT('Ctrl Pts',(7.27603390512273,-1.64398425424198,-4.20082013377291));
#16362=CARTESIAN_POINT('Ctrl Pts',(4.85068927007173,-1.46898425424197,-8.40164026752836));
#16363=CARTESIAN_POINT('Ctrl Pts',(-1.51301075899711E-11,-1.29398425424196,
-8.40164026751963));
#16364=CARTESIAN_POINT('Ctrl Pts',(-4.85068927010199,-1.11898425424198,
-8.4016402675109));
#16365=CARTESIAN_POINT('Ctrl Pts',(-7.27603390513785,-0.94398425424197,
-4.20082013374671));
#16366=CARTESIAN_POINT('Ctrl Pts',(-9.70137854017372,-0.768984254241965,
1.74701493417668E-11));
#16367=CARTESIAN_POINT('Ctrl Pts',(-7.27603390512272,-0.59398425424198,
4.20082013377292));
#16368=CARTESIAN_POINT('Ctrl Pts',(-4.85068927007173,-0.418984254241974,
8.40164026752836));
#16369=CARTESIAN_POINT('Ctrl Pts',(1.5129078685785E-11,-0.243984254241963,
8.40164026751963));
#16370=CARTESIAN_POINT('Ctrl Pts',(4.85068927010198,-0.068984254241984,
8.4016402675109));
#16371=CARTESIAN_POINT('Ctrl Pts',(7.27603390513785,0.106015745758026,4.20082013374672));
#16372=CARTESIAN_POINT('Ctrl Pts',(9.70137854017372,0.28101574575803,-1.74689612655491E-11));
#16373=CARTESIAN_POINT('Ctrl Pts',(7.27603390512273,0.456015745758015,-4.20082013377291));
#16374=CARTESIAN_POINT('Ctrl Pts',(4.85068927007173,0.631015745758021,-8.40164026752836));
#16375=CARTESIAN_POINT('Ctrl Pts',(-1.51301075899711E-11,0.806015745758032,
-8.40164026751963));
#16376=CARTESIAN_POINT('Ctrl Pts',(-4.85068927010199,0.981015745758011,
-8.4016402675109));
#16377=CARTESIAN_POINT('Ctrl Pts',(-7.27603390513785,1.15601574575802,-4.20082013374671));
#16378=CARTESIAN_POINT('Ctrl Pts',(-9.70137854017372,1.33101574575803,1.74701493417668E-11));
#16379=CARTESIAN_POINT('Ctrl Pts',(-7.27603390512272,1.50601574575804,4.20082013377292));
#16380=CARTESIAN_POINT('Ctrl Pts',(-4.85068927007173,1.68101574575802,8.40164026752836));
#16381=CARTESIAN_POINT('Ctrl Pts',(1.5129078685785E-11,1.85601574575803,
8.40164026751963));
#16382=CARTESIAN_POINT('Ctrl Pts',(4.85068927010198,2.03101574575803,8.4016402675109));
#16383=CARTESIAN_POINT('Ctrl Pts',(7.27603390513785,2.20601574575802,4.20082013374672));
#16384=CARTESIAN_POINT('Ctrl Pts',(9.70137854017372,2.38101574575802,-1.74689612655491E-11));
#16385=CARTESIAN_POINT('Ctrl Pts',(7.27603390512273,2.55601574575803,-4.20082013377291));
#16386=CARTESIAN_POINT('Ctrl Pts',(4.85068927007173,2.73101574575801,-8.40164026752836));
#16387=CARTESIAN_POINT('Ctrl Pts',(-1.51301075899711E-11,2.90601574575802,
-8.40164026751963));
#16388=CARTESIAN_POINT('Ctrl Pts',(-4.85068927010199,3.08101574575803,-8.4016402675109));
#16389=CARTESIAN_POINT('Ctrl Pts',(-7.27603390513785,3.25601574575801,-4.20082013374671));
#16390=CARTESIAN_POINT('Ctrl Pts',(-9.70137854017372,3.43101574575802,1.74701493417668E-11));
#16391=CARTESIAN_POINT('Ctrl Pts',(-7.27603390512272,3.60601574575803,4.20082013377292));
#16392=CARTESIAN_POINT('Ctrl Pts',(-4.85068927007173,3.78101574575801,8.40164026752836));
#16393=CARTESIAN_POINT('Ctrl Pts',(1.5129078685785E-11,3.95601574575802,
8.40164026751963));
#16394=CARTESIAN_POINT('Ctrl Pts',(4.85068927010198,4.13101574575802,8.4016402675109));
#16395=CARTESIAN_POINT('Ctrl Pts',(7.27603390513785,4.30601574575801,4.20082013374672));
#16396=CARTESIAN_POINT('Ctrl Pts',(9.70137854017372,4.48101574575801,-1.74689612655491E-11));
#16397=CARTESIAN_POINT('Ctrl Pts',(7.27603390512273,4.65601574575802,-4.20082013377291));
#16398=CARTESIAN_POINT('Ctrl Pts',(4.85068927007173,4.831015745758,-8.40164026752836));
#16399=CARTESIAN_POINT('Ctrl Pts',(-1.51301075899711E-11,5.00601574575801,
-8.40164026751963));
#16400=CARTESIAN_POINT('Ctrl Pts',(-4.85068927010199,5.18101574575802,-8.4016402675109));
#16401=CARTESIAN_POINT('Ctrl Pts',(-7.27603390513785,5.356015745758,-4.20082013374671));
#16402=CARTESIAN_POINT('Ctrl Pts',(-9.70137854017372,5.53101574575801,1.74701493417668E-11));
#16403=CARTESIAN_POINT('Ctrl Pts',(-7.27603390512272,5.70601574575802,4.20082013377292));
#16404=CARTESIAN_POINT('Ctrl Pts',(-4.85068927007173,5.881015745758,8.40164026752836));
#16405=CARTESIAN_POINT('Ctrl Pts',(1.5129078685785E-11,6.05601574575801,
8.40164026751963));
#16406=CARTESIAN_POINT('Ctrl Pts',(4.85068927010198,6.23101574575801,8.4016402675109));
#16407=CARTESIAN_POINT('Ctrl Pts',(7.27603390513785,6.40601574575803,4.20082013374672));
#16408=CARTESIAN_POINT('Ctrl Pts',(9.70137854017372,6.581015745758,-1.74689612655491E-11));
#16409=CARTESIAN_POINT('Ctrl Pts',(7.27603390512273,6.75601574575802,-4.20082013377291));
#16410=CARTESIAN_POINT('Ctrl Pts',(4.85068927007173,6.93101574575802,-8.40164026752836));
#16411=CARTESIAN_POINT('Ctrl Pts',(-1.51301075899711E-11,7.106015745758,
-8.40164026751963));
#16412=CARTESIAN_POINT('Ctrl Pts',(-4.85068927010199,7.28101574575801,-8.4016402675109));
#16413=CARTESIAN_POINT('Ctrl Pts',(-7.27603390513785,7.45601574575802,-4.20082013374671));
#16414=CARTESIAN_POINT('Ctrl Pts',(-9.70137854017372,7.631015745758,1.74701493417668E-11));
#16415=CARTESIAN_POINT('Ctrl Pts',(-7.27603390512272,7.80601574575801,4.20082013377292));
#16416=CARTESIAN_POINT('Ctrl Pts',(-4.85068927007173,7.98101574575801,8.40164026752836));
#16417=CARTESIAN_POINT('Ctrl Pts',(1.5129078685785E-11,8.156015745758,8.40164026751963));
#16418=CARTESIAN_POINT('Ctrl Pts',(4.85068927010198,8.331015745758,8.4016402675109));
#16419=CARTESIAN_POINT('Ctrl Pts',(7.27603390513785,8.50601574575802,4.20082013374672));
#16420=CARTESIAN_POINT('Ctrl Pts',(9.70137854017372,8.68101574575799,-1.74689612655491E-11));
#16421=CARTESIAN_POINT('Ctrl Pts',(7.27603390512273,8.85601574575801,-4.20082013377291));
#16422=CARTESIAN_POINT('Ctrl Pts',(4.85068927007173,9.03101574575801,-8.40164026752836));
#16423=CARTESIAN_POINT('Ctrl Pts',(-1.51301075899711E-11,9.20601574575799,
-8.40164026751963));
#16424=CARTESIAN_POINT('Ctrl Pts',(-4.85068927010199,9.381015745758,-8.4016402675109));
#16425=CARTESIAN_POINT('Ctrl Pts',(-7.27603390513785,9.55601574575801,-4.20082013374671));
#16426=CARTESIAN_POINT('Ctrl Pts',(-9.70137854017372,9.73101574575799,1.74701493417668E-11));
#16427=CARTESIAN_POINT('Ctrl Pts',(-7.27603390512272,9.906015745758,4.20082013377292));
#16428=CARTESIAN_POINT('Ctrl Pts',(-4.85068927007173,10.081015745758,8.40164026752836));
#16429=CARTESIAN_POINT('Ctrl Pts',(1.5129078685785E-11,10.256015745758,
8.40164026751963));
#16430=CARTESIAN_POINT('Ctrl Pts',(4.85068927010198,10.431015745758,8.4016402675109));
#16431=CARTESIAN_POINT('Ctrl Pts',(7.27603390513785,10.606015745758,4.20082013374672));
#16432=CARTESIAN_POINT('Ctrl Pts',(9.70137854017372,10.781015745758,-1.74689612655491E-11));
#16433=CARTESIAN_POINT('Ctrl Pts',(7.27603390512273,10.956015745758,-4.20082013377291));
#16434=CARTESIAN_POINT('Ctrl Pts',(4.85068927007173,11.131015745758,-8.40164026752836));
#16435=CARTESIAN_POINT('Ctrl Pts',(-1.51301075899711E-11,11.306015745758,
-8.40164026751963));
#16436=CARTESIAN_POINT('Ctrl Pts',(-4.85068927010199,11.481015745758,-8.4016402675109));
#16437=CARTESIAN_POINT('Ctrl Pts',(-7.27603390513785,11.656015745758,-4.20082013374671));
#16438=CARTESIAN_POINT('Ctrl Pts',(-9.70137854017372,11.831015745758,1.74701493417668E-11));
#16439=CARTESIAN_POINT('Ctrl Pts',(-7.27603390512272,12.006015745758,4.20082013377292));
#16440=CARTESIAN_POINT('Ctrl Pts',(-4.85068927007173,12.181015745758,8.40164026752836));
#16441=CARTESIAN_POINT('Ctrl Pts',(1.5129078685785E-11,12.356015745758,
8.40164026751963));
#16442=CARTESIAN_POINT('Ctrl Pts',(4.85068927010198,12.531015745758,8.4016402675109));
#16443=CARTESIAN_POINT('Ctrl Pts',(7.27603390513785,12.706015745758,4.20082013374672));
#16444=CARTESIAN_POINT('Ctrl Pts',(9.70137854017372,12.881015745758,-1.74689612655491E-11));
#16445=CARTESIAN_POINT('Ctrl Pts',(7.27603390512273,13.056015745758,-4.20082013377291));
#16446=CARTESIAN_POINT('Ctrl Pts',(4.85068927007173,13.231015745758,-8.40164026752836));
#16447=CARTESIAN_POINT('Ctrl Pts',(-1.51301075899711E-11,13.406015745758,
-8.40164026751963));
#16448=CARTESIAN_POINT('Ctrl Pts',(-4.85068927010199,13.581015745758,-8.4016402675109));
#16449=CARTESIAN_POINT('Ctrl Pts',(-7.27603390513785,13.756015745758,-4.20082013374671));
#16450=CARTESIAN_POINT('Ctrl Pts',(-9.70137854017372,13.931015745758,1.74701493417668E-11));
#16451=CARTESIAN_POINT('Ctrl Pts',(-7.27603390512272,14.106015745758,4.20082013377292));
#16452=CARTESIAN_POINT('Ctrl Pts',(-4.85068927007173,14.281015745758,8.40164026752836));
#16453=CARTESIAN_POINT('Ctrl Pts',(1.5129078685785E-11,14.456015745758,
8.40164026751963));
#16454=CARTESIAN_POINT('Ctrl Pts',(4.85068927010198,14.631015745758,8.4016402675109));
#16455=CARTESIAN_POINT('Ctrl Pts',(7.27603390513785,14.806015745758,4.20082013374672));
#16456=CARTESIAN_POINT('Ctrl Pts',(9.70137854017372,14.981015745758,-1.74689612655491E-11));
#16457=CARTESIAN_POINT('Ctrl Pts',(7.27603390512273,15.156015745758,-4.20082013377291));
#16458=CARTESIAN_POINT('Ctrl Pts',(4.85068927007173,15.331015745758,-8.40164026752836));
#16459=CARTESIAN_POINT('Ctrl Pts',(-1.51301075899711E-11,15.506015745758,
-8.40164026751963));
#16460=CARTESIAN_POINT('Ctrl Pts',(-4.85068927010199,15.681015745758,-8.4016402675109));
#16461=CARTESIAN_POINT('Ctrl Pts',(-7.27603390513785,15.856015745758,-4.20082013374671));
#16462=CARTESIAN_POINT('Ctrl Pts',(-9.70137854017372,16.031015745758,1.74701493417668E-11));
#16463=CARTESIAN_POINT('Ctrl Pts',(-7.27603390512272,16.206015745758,4.20082013377292));
#16464=CARTESIAN_POINT('Ctrl Pts',(-4.85068927007173,16.381015745758,8.40164026752836));
#16465=CARTESIAN_POINT('Ctrl Pts',(1.5129078685785E-11,16.556015745758,
8.40164026751963));
#16466=CARTESIAN_POINT('Ctrl Pts',(4.85068927010198,16.731015745758,8.4016402675109));
#16467=CARTESIAN_POINT('Ctrl Pts',(7.27603390513785,16.906015745758,4.20082013374672));
#16468=CARTESIAN_POINT('Ctrl Pts',(9.70137854017372,17.081015745758,-1.74689612655491E-11));
#16469=CARTESIAN_POINT('Ctrl Pts',(7.27603390512273,17.256015745758,-4.20082013377291));
#16470=CARTESIAN_POINT('Ctrl Pts',(4.85068927007173,17.431015745758,-8.40164026752836));
#16471=CARTESIAN_POINT('Ctrl Pts',(-1.51301075899711E-11,17.606015745758,
-8.40164026751963));
#16472=CARTESIAN_POINT('Ctrl Pts',(-4.85068927010199,17.781015745758,-8.4016402675109));
#16473=CARTESIAN_POINT('Ctrl Pts',(-7.27603390513785,17.956015745758,-4.20082013374671));
#16474=CARTESIAN_POINT('Ctrl Pts',(-9.70137854017372,18.131015745758,1.74701493417668E-11));
#16475=CARTESIAN_POINT('Ctrl Pts',(-7.27603390512272,18.306015745758,4.20082013377292));
#16476=CARTESIAN_POINT('Ctrl Pts',(-4.85068927007173,18.481015745758,8.40164026752836));
#16477=CARTESIAN_POINT('Ctrl Pts',(1.5129078685785E-11,18.656015745758,
8.40164026751963));
#16478=CARTESIAN_POINT('Ctrl Pts',(4.85068927010198,18.831015745758,8.4016402675109));
#16479=CARTESIAN_POINT('Ctrl Pts',(7.27603390513785,19.006015745758,4.20082013374672));
#16480=CARTESIAN_POINT('Ctrl Pts',(9.70137854017372,19.181015745758,-1.74689612655491E-11));
#16481=CARTESIAN_POINT('Ctrl Pts',(7.27603390512273,19.356015745758,-4.20082013377291));
#16482=CARTESIAN_POINT('Ctrl Pts',(4.85068927007173,19.531015745758,-8.40164026752836));
#16483=CARTESIAN_POINT('Ctrl Pts',(-1.51301075899711E-11,19.706015745758,
-8.40164026751963));
#16484=CARTESIAN_POINT('Ctrl Pts',(-4.85068927010199,19.881015745758,-8.4016402675109));
#16485=CARTESIAN_POINT('Ctrl Pts',(-7.27603390513785,20.056015745758,-4.20082013374671));
#16486=CARTESIAN_POINT('Ctrl Pts',(-9.70137854017372,20.231015745758,1.74701493417668E-11));
#16487=CARTESIAN_POINT('Ctrl Pts',(-7.27603390512272,20.406015745758,4.20082013377292));
#16488=CARTESIAN_POINT('Ctrl Pts',(-4.85068927007173,20.581015745758,8.40164026752836));
#16489=CARTESIAN_POINT('Ctrl Pts',(1.5129078685785E-11,20.756015745758,
8.40164026751963));
#16490=CARTESIAN_POINT('Ctrl Pts',(4.85068927010198,20.931015745758,8.4016402675109));
#16491=CARTESIAN_POINT('Ctrl Pts',(7.27603390513785,21.106015745758,4.20082013374672));
#16492=CARTESIAN_POINT('Ctrl Pts',(9.70137854017372,21.281015745758,-1.74689612655491E-11));
#16493=CARTESIAN_POINT('Ctrl Pts',(7.27603390512273,21.456015745758,-4.20082013377291));
#16494=CARTESIAN_POINT('Ctrl Pts',(4.85068927007173,21.631015745758,-8.40164026752836));
#16495=CARTESIAN_POINT('Ctrl Pts',(-1.51301075899711E-11,21.806015745758,
-8.40164026751963));
#16496=CARTESIAN_POINT('Ctrl Pts',(-4.85068927010199,21.981015745758,-8.4016402675109));
#16497=CARTESIAN_POINT('Ctrl Pts',(-7.27603390513785,22.156015745758,-4.20082013374671));
#16498=CARTESIAN_POINT('Ctrl Pts',(-9.70137854017372,22.331015745758,1.74701493417668E-11));
#16499=CARTESIAN_POINT('Ctrl Pts',(-7.27603390512272,22.506015745758,4.20082013377292));
#16500=CARTESIAN_POINT('Ctrl Pts',(-4.85068927007173,22.681015745758,8.40164026752836));
#16501=CARTESIAN_POINT('Ctrl Pts',(1.5129078685785E-11,22.856015745758,
8.40164026751963));
#16502=CARTESIAN_POINT('Ctrl Pts',(4.85068927010198,23.031015745758,8.4016402675109));
#16503=CARTESIAN_POINT('Ctrl Pts',(7.27603390513785,23.206015745758,4.20082013374672));
#16504=CARTESIAN_POINT('Ctrl Pts',(9.70137854017372,23.381015745758,-1.74689612655491E-11));
#16505=CARTESIAN_POINT('Ctrl Pts',(7.27603390512273,23.556015745758,-4.20082013377291));
#16506=CARTESIAN_POINT('Ctrl Pts',(4.85068927007173,23.731015745758,-8.40164026752836));
#16507=CARTESIAN_POINT('Ctrl Pts',(-1.51301075899711E-11,23.906015745758,
-8.40164026751963));
#16508=CARTESIAN_POINT('Ctrl Pts',(-4.85068927010199,24.081015745758,-8.4016402675109));
#16509=CARTESIAN_POINT('Ctrl Pts',(-7.27603390513785,24.256015745758,-4.20082013374671));
#16510=CARTESIAN_POINT('Ctrl Pts',(-9.70137854017372,24.431015745758,1.74701493417668E-11));
#16511=CARTESIAN_POINT('Ctrl Pts',(-7.27603390512272,24.606015745758,4.20082013377292));
#16512=CARTESIAN_POINT('Ctrl Pts',(-4.85068927007173,24.781015745758,8.40164026752836));
#16513=CARTESIAN_POINT('Ctrl Pts',(1.5129078685785E-11,24.956015745758,
8.40164026751963));
#16514=CARTESIAN_POINT('Ctrl Pts',(4.85068927010198,25.131015745758,8.4016402675109));
#16515=CARTESIAN_POINT('Ctrl Pts',(7.27603390513785,25.306015745758,4.20082013374672));
#16516=CARTESIAN_POINT('Ctrl Pts',(9.70137854017372,25.481015745758,-1.74689612655491E-11));
#16517=CARTESIAN_POINT('Ctrl Pts',(7.27603390512273,25.656015745758,-4.20082013377291));
#16518=CARTESIAN_POINT('Ctrl Pts',(4.85068927007173,25.831015745758,-8.40164026752836));
#16519=CARTESIAN_POINT('Ctrl Pts',(-1.51301075899711E-11,26.006015745758,
-8.40164026751963));
#16520=CARTESIAN_POINT('Ctrl Pts',(-1.4702867290402E-11,-143.970483118095,
-8.16439679232146));
#16521=CARTESIAN_POINT('Ctrl Pts',(-4.71371668583241,-143.795483118095,
-8.16439679231297));
#16522=CARTESIAN_POINT('Ctrl Pts',(-7.07057502873392,-143.620483118095,
-4.082198396148));
#16523=CARTESIAN_POINT('Ctrl Pts',(-9.42743337163542,-143.445483118095,
1.69768315121407E-11));
#16524=CARTESIAN_POINT('Ctrl Pts',(-7.07057502871922,-143.270483118095,
4.08219839617346));
#16525=CARTESIAN_POINT('Ctrl Pts',(-4.71371668580301,-143.095483118095,
8.16439679232994));
#16526=CARTESIAN_POINT('Ctrl Pts',(1.47018674401621E-11,-142.920483118095,
8.16439679232146));
#16527=CARTESIAN_POINT('Ctrl Pts',(4.71371668583241,-142.745483118095,8.16439679231297));
#16528=CARTESIAN_POINT('Ctrl Pts',(7.07057502873392,-142.570483118095,4.082198396148));
#16529=CARTESIAN_POINT('Ctrl Pts',(9.42743337163542,-142.395483118095,-1.69756769845304E-11));
#16530=CARTESIAN_POINT('Ctrl Pts',(7.07057502871922,-142.220483118095,-4.08219839617346));
#16531=CARTESIAN_POINT('Ctrl Pts',(4.71371668580301,-142.045483118095,-8.16439679232994));
#16532=CARTESIAN_POINT('Ctrl Pts',(-1.4702867290402E-11,-141.870483118095,
-8.16439679232146));
#16533=CARTESIAN_POINT('Ctrl Pts',(-4.71371668583241,-141.695483118095,
-8.16439679231297));
#16534=CARTESIAN_POINT('Ctrl Pts',(-7.07057502873392,-141.520483118095,
-4.082198396148));
#16535=CARTESIAN_POINT('Ctrl Pts',(-9.42743337163542,-141.345483118095,
1.69768315121407E-11));
#16536=CARTESIAN_POINT('Ctrl Pts',(-7.07057502871922,-141.170483118095,
4.08219839617346));
#16537=CARTESIAN_POINT('Ctrl Pts',(-4.71371668580301,-140.995483118095,
8.16439679232994));
#16538=CARTESIAN_POINT('Ctrl Pts',(1.47018674401621E-11,-140.820483118095,
8.16439679232146));
#16539=CARTESIAN_POINT('Ctrl Pts',(4.71371668583241,-140.645483118095,8.16439679231297));
#16540=CARTESIAN_POINT('Ctrl Pts',(7.07057502873392,-140.470483118095,4.082198396148));
#16541=CARTESIAN_POINT('Ctrl Pts',(9.42743337163542,-140.295483118095,-1.69756769845304E-11));
#16542=CARTESIAN_POINT('Ctrl Pts',(7.07057502871922,-140.120483118095,-4.08219839617346));
#16543=CARTESIAN_POINT('Ctrl Pts',(4.71371668580301,-139.945483118095,-8.16439679232994));
#16544=CARTESIAN_POINT('Ctrl Pts',(-1.4702867290402E-11,-139.770483118095,
-8.16439679232146));
#16545=CARTESIAN_POINT('Ctrl Pts',(-4.71371668583241,-139.595483118095,
-8.16439679231297));
#16546=CARTESIAN_POINT('Ctrl Pts',(-7.07057502873392,-139.420483118095,
-4.082198396148));
#16547=CARTESIAN_POINT('Ctrl Pts',(-9.42743337163542,-139.245483118095,
1.69768315121407E-11));
#16548=CARTESIAN_POINT('Ctrl Pts',(-7.07057502871922,-139.070483118095,
4.08219839617346));
#16549=CARTESIAN_POINT('Ctrl Pts',(-4.71371668580301,-138.895483118095,
8.16439679232994));
#16550=CARTESIAN_POINT('Ctrl Pts',(1.47018674401621E-11,-138.720483118095,
8.16439679232146));
#16551=CARTESIAN_POINT('Ctrl Pts',(4.71371668583241,-138.545483118095,8.16439679231297));
#16552=CARTESIAN_POINT('Ctrl Pts',(7.07057502873392,-138.370483118095,4.082198396148));
#16553=CARTESIAN_POINT('Ctrl Pts',(9.42743337163542,-138.195483118095,-1.69756769845304E-11));
#16554=CARTESIAN_POINT('Ctrl Pts',(7.07057502871922,-138.020483118095,-4.08219839617346));
#16555=CARTESIAN_POINT('Ctrl Pts',(4.71371668580301,-137.845483118095,-8.16439679232994));
#16556=CARTESIAN_POINT('Ctrl Pts',(-1.4702867290402E-11,-137.670483118095,
-8.16439679232146));
#16557=CARTESIAN_POINT('Ctrl Pts',(-4.71371668583241,-137.495483118095,
-8.16439679231297));
#16558=CARTESIAN_POINT('Ctrl Pts',(-7.07057502873392,-137.320483118095,
-4.082198396148));
#16559=CARTESIAN_POINT('Ctrl Pts',(-9.42743337163542,-137.145483118095,
1.69768315121407E-11));
#16560=CARTESIAN_POINT('Ctrl Pts',(-7.07057502871922,-136.970483118095,
4.08219839617346));
#16561=CARTESIAN_POINT('Ctrl Pts',(-4.71371668580301,-136.795483118095,
8.16439679232994));
#16562=CARTESIAN_POINT('Ctrl Pts',(1.47018674401621E-11,-136.620483118095,
8.16439679232146));
#16563=CARTESIAN_POINT('Ctrl Pts',(4.71371668583241,-136.445483118095,8.16439679231297));
#16564=CARTESIAN_POINT('Ctrl Pts',(7.07057502873392,-136.270483118095,4.082198396148));
#16565=CARTESIAN_POINT('Ctrl Pts',(9.42743337163542,-136.095483118095,-1.69756769845304E-11));
#16566=CARTESIAN_POINT('Ctrl Pts',(7.07057502871922,-135.920483118095,-4.08219839617346));
#16567=CARTESIAN_POINT('Ctrl Pts',(4.71371668580301,-135.745483118095,-8.16439679232994));
#16568=CARTESIAN_POINT('Ctrl Pts',(-1.4702867290402E-11,-135.570483118095,
-8.16439679232146));
#16569=CARTESIAN_POINT('Ctrl Pts',(-4.71371668583241,-135.395483118095,
-8.16439679231297));
#16570=CARTESIAN_POINT('Ctrl Pts',(-7.07057502873392,-135.220483118095,
-4.082198396148));
#16571=CARTESIAN_POINT('Ctrl Pts',(-9.42743337163542,-135.045483118095,
1.69768315121407E-11));
#16572=CARTESIAN_POINT('Ctrl Pts',(-7.07057502871922,-134.870483118095,
4.08219839617346));
#16573=CARTESIAN_POINT('Ctrl Pts',(-4.71371668580301,-134.695483118095,
8.16439679232994));
#16574=CARTESIAN_POINT('Ctrl Pts',(1.47018674401621E-11,-134.520483118095,
8.16439679232146));
#16575=CARTESIAN_POINT('Ctrl Pts',(4.71371668583241,-134.345483118095,8.16439679231297));
#16576=CARTESIAN_POINT('Ctrl Pts',(7.07057502873392,-134.170483118095,4.082198396148));
#16577=CARTESIAN_POINT('Ctrl Pts',(9.42743337163542,-133.995483118095,-1.69756769845304E-11));
#16578=CARTESIAN_POINT('Ctrl Pts',(7.07057502871922,-133.820483118095,-4.08219839617346));
#16579=CARTESIAN_POINT('Ctrl Pts',(4.71371668580301,-133.645483118095,-8.16439679232994));
#16580=CARTESIAN_POINT('Ctrl Pts',(-1.4702867290402E-11,-133.470483118095,
-8.16439679232146));
#16581=CARTESIAN_POINT('Ctrl Pts',(-4.71371668583241,-133.295483118095,
-8.16439679231297));
#16582=CARTESIAN_POINT('Ctrl Pts',(-7.07057502873392,-133.120483118095,
-4.082198396148));
#16583=CARTESIAN_POINT('Ctrl Pts',(-9.42743337163542,-132.945483118095,
1.69768315121407E-11));
#16584=CARTESIAN_POINT('Ctrl Pts',(-7.07057502871922,-132.770483118095,
4.08219839617346));
#16585=CARTESIAN_POINT('Ctrl Pts',(-4.71371668580301,-132.595483118095,
8.16439679232994));
#16586=CARTESIAN_POINT('Ctrl Pts',(1.47018674401621E-11,-132.420483118095,
8.16439679232146));
#16587=CARTESIAN_POINT('Ctrl Pts',(4.71371668583241,-132.245483118095,8.16439679231297));
#16588=CARTESIAN_POINT('Ctrl Pts',(7.07057502873392,-132.070483118095,4.082198396148));
#16589=CARTESIAN_POINT('Ctrl Pts',(9.42743337163542,-131.895483118095,-1.69756769845304E-11));
#16590=CARTESIAN_POINT('Ctrl Pts',(7.07057502871922,-131.720483118095,-4.08219839617346));
#16591=CARTESIAN_POINT('Ctrl Pts',(4.71371668580301,-131.545483118095,-8.16439679232994));
#16592=CARTESIAN_POINT('Ctrl Pts',(-1.4702867290402E-11,-131.370483118095,
-8.16439679232146));
#16593=CARTESIAN_POINT('Ctrl Pts',(-4.71371668583241,-131.195483118095,
-8.16439679231297));
#16594=CARTESIAN_POINT('Ctrl Pts',(-7.07057502873392,-131.020483118095,
-4.082198396148));
#16595=CARTESIAN_POINT('Ctrl Pts',(-9.42743337163542,-130.845483118095,
1.69768315121407E-11));
#16596=CARTESIAN_POINT('Ctrl Pts',(-7.07057502871922,-130.670483118095,
4.08219839617346));
#16597=CARTESIAN_POINT('Ctrl Pts',(-4.71371668580301,-130.495483118095,
8.16439679232994));
#16598=CARTESIAN_POINT('Ctrl Pts',(1.47018674401621E-11,-130.320483118095,
8.16439679232146));
#16599=CARTESIAN_POINT('Ctrl Pts',(4.71371668583241,-130.145483118095,8.16439679231297));
#16600=CARTESIAN_POINT('Ctrl Pts',(7.07057502873392,-129.970483118095,4.082198396148));
#16601=CARTESIAN_POINT('Ctrl Pts',(9.42743337163542,-129.795483118095,-1.69756769845304E-11));
#16602=CARTESIAN_POINT('Ctrl Pts',(7.07057502871922,-129.620483118095,-4.08219839617346));
#16603=CARTESIAN_POINT('Ctrl Pts',(4.71371668580301,-129.445483118095,-8.16439679232994));
#16604=CARTESIAN_POINT('Ctrl Pts',(-1.4702867290402E-11,-129.270483118095,
-8.16439679232146));
#16605=CARTESIAN_POINT('Ctrl Pts',(-4.71371668583241,-129.095483118095,
-8.16439679231297));
#16606=CARTESIAN_POINT('Ctrl Pts',(-7.07057502873392,-128.920483118095,
-4.082198396148));
#16607=CARTESIAN_POINT('Ctrl Pts',(-9.42743337163542,-128.745483118095,
1.69768315121407E-11));
#16608=CARTESIAN_POINT('Ctrl Pts',(-7.07057502871922,-128.570483118095,
4.08219839617346));
#16609=CARTESIAN_POINT('Ctrl Pts',(-4.71371668580301,-128.395483118095,
8.16439679232994));
#16610=CARTESIAN_POINT('Ctrl Pts',(1.47018674401621E-11,-128.220483118095,
8.16439679232146));
#16611=CARTESIAN_POINT('Ctrl Pts',(4.71371668583241,-128.045483118095,8.16439679231297));
#16612=CARTESIAN_POINT('Ctrl Pts',(7.07057502873392,-127.870483118095,4.082198396148));
#16613=CARTESIAN_POINT('Ctrl Pts',(9.42743337163542,-127.695483118095,-1.69756769845304E-11));
#16614=CARTESIAN_POINT('Ctrl Pts',(7.07057502871922,-127.520483118095,-4.08219839617346));
#16615=CARTESIAN_POINT('Ctrl Pts',(4.71371668580301,-127.345483118095,-8.16439679232994));
#16616=CARTESIAN_POINT('Ctrl Pts',(-1.4702867290402E-11,-127.170483118095,
-8.16439679232146));
#16617=CARTESIAN_POINT('Ctrl Pts',(-4.71371668583241,-126.995483118095,
-8.16439679231297));
#16618=CARTESIAN_POINT('Ctrl Pts',(-7.07057502873392,-126.820483118095,
-4.082198396148));
#16619=CARTESIAN_POINT('Ctrl Pts',(-9.42743337163542,-126.645483118095,
1.69768315121407E-11));
#16620=CARTESIAN_POINT('Ctrl Pts',(-7.07057502871922,-126.470483118095,
4.08219839617346));
#16621=CARTESIAN_POINT('Ctrl Pts',(-4.71371668580301,-126.295483118095,
8.16439679232994));
#16622=CARTESIAN_POINT('Ctrl Pts',(1.47018674401621E-11,-126.120483118095,
8.16439679232146));
#16623=CARTESIAN_POINT('Ctrl Pts',(4.71371668583241,-125.945483118095,8.16439679231297));
#16624=CARTESIAN_POINT('Ctrl Pts',(7.07057502873392,-125.770483118095,4.082198396148));
#16625=CARTESIAN_POINT('Ctrl Pts',(9.42743337163542,-125.595483118095,-1.69756769845304E-11));
#16626=CARTESIAN_POINT('Ctrl Pts',(7.07057502871922,-125.420483118095,-4.08219839617346));
#16627=CARTESIAN_POINT('Ctrl Pts',(4.71371668580301,-125.245483118095,-8.16439679232994));
#16628=CARTESIAN_POINT('Ctrl Pts',(-1.4702867290402E-11,-125.070483118095,
-8.16439679232146));
#16629=CARTESIAN_POINT('Ctrl Pts',(-4.71371668583241,-124.895483118095,
-8.16439679231297));
#16630=CARTESIAN_POINT('Ctrl Pts',(-7.07057502873392,-124.720483118095,
-4.082198396148));
#16631=CARTESIAN_POINT('Ctrl Pts',(-9.42743337163542,-124.545483118095,
1.69768315121407E-11));
#16632=CARTESIAN_POINT('Ctrl Pts',(-7.07057502871922,-124.370483118095,
4.08219839617346));
#16633=CARTESIAN_POINT('Ctrl Pts',(-4.71371668580301,-124.195483118095,
8.16439679232994));
#16634=CARTESIAN_POINT('Ctrl Pts',(1.47018674401621E-11,-124.020483118095,
8.16439679232146));
#16635=CARTESIAN_POINT('Ctrl Pts',(4.71371668583241,-123.845483118095,8.16439679231297));
#16636=CARTESIAN_POINT('Ctrl Pts',(7.07057502873392,-123.670483118095,4.082198396148));
#16637=CARTESIAN_POINT('Ctrl Pts',(9.42743337163542,-123.495483118095,-1.69756769845304E-11));
#16638=CARTESIAN_POINT('Ctrl Pts',(7.07057502871922,-123.320483118095,-4.08219839617346));
#16639=CARTESIAN_POINT('Ctrl Pts',(4.71371668580301,-123.145483118095,-8.16439679232994));
#16640=CARTESIAN_POINT('Ctrl Pts',(-1.4702867290402E-11,-122.970483118095,
-8.16439679232146));
#16641=CARTESIAN_POINT('Ctrl Pts',(-4.71371668583241,-122.795483118095,
-8.16439679231297));
#16642=CARTESIAN_POINT('Ctrl Pts',(-7.07057502873392,-122.620483118095,
-4.082198396148));
#16643=CARTESIAN_POINT('Ctrl Pts',(-9.42743337163542,-122.445483118095,
1.69768315121407E-11));
#16644=CARTESIAN_POINT('Ctrl Pts',(-7.07057502871922,-122.270483118095,
4.08219839617346));
#16645=CARTESIAN_POINT('Ctrl Pts',(-4.71371668580301,-122.095483118095,
8.16439679232994));
#16646=CARTESIAN_POINT('Ctrl Pts',(1.47018674401621E-11,-121.920483118095,
8.16439679232146));
#16647=CARTESIAN_POINT('Ctrl Pts',(4.71371668583241,-121.745483118095,8.16439679231297));
#16648=CARTESIAN_POINT('Ctrl Pts',(7.07057502873392,-121.570483118095,4.082198396148));
#16649=CARTESIAN_POINT('Ctrl Pts',(9.42743337163542,-121.395483118095,-1.69756769845304E-11));
#16650=CARTESIAN_POINT('Ctrl Pts',(7.07057502871922,-121.220483118095,-4.08219839617346));
#16651=CARTESIAN_POINT('Ctrl Pts',(4.71371668580301,-121.045483118095,-8.16439679232994));
#16652=CARTESIAN_POINT('Ctrl Pts',(-1.4702867290402E-11,-120.870483118095,
-8.16439679232146));
#16653=CARTESIAN_POINT('Ctrl Pts',(-4.71371668583241,-120.695483118095,
-8.16439679231297));
#16654=CARTESIAN_POINT('Ctrl Pts',(-7.07057502873392,-120.520483118095,
-4.082198396148));
#16655=CARTESIAN_POINT('Ctrl Pts',(-9.42743337163542,-120.345483118095,
1.69768315121407E-11));
#16656=CARTESIAN_POINT('Ctrl Pts',(-7.07057502871922,-120.170483118095,
4.08219839617346));
#16657=CARTESIAN_POINT('Ctrl Pts',(-4.71371668580301,-119.995483118095,
8.16439679232994));
#16658=CARTESIAN_POINT('Ctrl Pts',(1.47018674401621E-11,-119.820483118095,
8.16439679232146));
#16659=CARTESIAN_POINT('Ctrl Pts',(4.71371668583241,-119.645483118095,8.16439679231297));
#16660=CARTESIAN_POINT('Ctrl Pts',(7.07057502873392,-119.470483118095,4.082198396148));
#16661=CARTESIAN_POINT('Ctrl Pts',(9.42743337163542,-119.295483118095,-1.69756769845304E-11));
#16662=CARTESIAN_POINT('Ctrl Pts',(7.07057502871922,-119.120483118095,-4.08219839617346));
#16663=CARTESIAN_POINT('Ctrl Pts',(4.71371668580301,-118.945483118095,-8.16439679232994));
#16664=CARTESIAN_POINT('Ctrl Pts',(-1.4702867290402E-11,-118.770483118095,
-8.16439679232146));
#16665=CARTESIAN_POINT('Ctrl Pts',(-4.71371668583241,-118.595483118095,
-8.16439679231297));
#16666=CARTESIAN_POINT('Ctrl Pts',(-7.07057502873392,-118.420483118095,
-4.082198396148));
#16667=CARTESIAN_POINT('Ctrl Pts',(-9.42743337163542,-118.245483118095,
1.69768315121407E-11));
#16668=CARTESIAN_POINT('Ctrl Pts',(-7.07057502871922,-118.070483118095,
4.08219839617346));
#16669=CARTESIAN_POINT('Ctrl Pts',(-4.71371668580301,-117.895483118095,
8.16439679232994));
#16670=CARTESIAN_POINT('Ctrl Pts',(1.47018674401621E-11,-117.720483118095,
8.16439679232146));
#16671=CARTESIAN_POINT('Ctrl Pts',(4.71371668583241,-117.545483118095,8.16439679231297));
#16672=CARTESIAN_POINT('Ctrl Pts',(7.07057502873392,-117.370483118095,4.082198396148));
#16673=CARTESIAN_POINT('Ctrl Pts',(9.42743337163542,-117.195483118095,-1.69756769845304E-11));
#16674=CARTESIAN_POINT('Ctrl Pts',(7.07057502871922,-117.020483118095,-4.08219839617346));
#16675=CARTESIAN_POINT('Ctrl Pts',(4.71371668580301,-116.845483118095,-8.16439679232994));
#16676=CARTESIAN_POINT('Ctrl Pts',(-1.4702867290402E-11,-116.670483118095,
-8.16439679232146));
#16677=CARTESIAN_POINT('Ctrl Pts',(-4.71371668583241,-116.495483118095,
-8.16439679231297));
#16678=CARTESIAN_POINT('Ctrl Pts',(-7.07057502873392,-116.320483118095,
-4.082198396148));
#16679=CARTESIAN_POINT('Ctrl Pts',(-9.42743337163542,-116.145483118095,
1.69768315121407E-11));
#16680=CARTESIAN_POINT('Ctrl Pts',(-7.07057502871922,-115.970483118095,
4.08219839617346));
#16681=CARTESIAN_POINT('Ctrl Pts',(-4.71371668580301,-115.795483118095,
8.16439679232994));
#16682=CARTESIAN_POINT('Ctrl Pts',(1.47018674401621E-11,-115.620483118095,
8.16439679232146));
#16683=CARTESIAN_POINT('Ctrl Pts',(4.71371668583241,-115.445483118095,8.16439679231297));
#16684=CARTESIAN_POINT('Ctrl Pts',(7.07057502873392,-115.270483118095,4.082198396148));
#16685=CARTESIAN_POINT('Ctrl Pts',(9.42743337163542,-115.095483118095,-1.69756769845304E-11));
#16686=CARTESIAN_POINT('Ctrl Pts',(7.07057502871922,-114.920483118095,-4.08219839617346));
#16687=CARTESIAN_POINT('Ctrl Pts',(4.71371668580301,-114.745483118095,-8.16439679232994));
#16688=CARTESIAN_POINT('Ctrl Pts',(-1.4702867290402E-11,-114.570483118095,
-8.16439679232146));
#16689=CARTESIAN_POINT('Ctrl Pts',(-4.71371668583241,-114.395483118095,
-8.16439679231297));
#16690=CARTESIAN_POINT('Ctrl Pts',(-7.07057502873392,-114.220483118095,
-4.082198396148));
#16691=CARTESIAN_POINT('Ctrl Pts',(-9.42743337163542,-114.045483118095,
1.69768315121407E-11));
#16692=CARTESIAN_POINT('Ctrl Pts',(-7.07057502871922,-113.870483118095,
4.08219839617346));
#16693=CARTESIAN_POINT('Ctrl Pts',(-4.71371668580301,-113.695483118095,
8.16439679232994));
#16694=CARTESIAN_POINT('Ctrl Pts',(1.47018674401621E-11,-113.520483118095,
8.16439679232146));
#16695=CARTESIAN_POINT('Ctrl Pts',(4.71371668583241,-113.345483118095,8.16439679231297));
#16696=CARTESIAN_POINT('Ctrl Pts',(7.07057502873392,-113.170483118095,4.082198396148));
#16697=CARTESIAN_POINT('Ctrl Pts',(9.42743337163542,-112.995483118095,-1.69756769845304E-11));
#16698=CARTESIAN_POINT('Ctrl Pts',(7.07057502871922,-112.820483118095,-4.08219839617346));
#16699=CARTESIAN_POINT('Ctrl Pts',(4.71371668580301,-112.645483118095,-8.16439679232994));
#16700=CARTESIAN_POINT('Ctrl Pts',(-1.4702867290402E-11,-112.470483118095,
-8.16439679232146));
#16701=CARTESIAN_POINT('Ctrl Pts',(-4.71371668583241,-112.295483118095,
-8.16439679231297));
#16702=CARTESIAN_POINT('Ctrl Pts',(-7.07057502873392,-112.120483118095,
-4.082198396148));
#16703=CARTESIAN_POINT('Ctrl Pts',(-9.42743337163542,-111.945483118095,
1.69768315121407E-11));
#16704=CARTESIAN_POINT('Ctrl Pts',(-7.07057502871922,-111.770483118095,
4.08219839617346));
#16705=CARTESIAN_POINT('Ctrl Pts',(-4.71371668580301,-111.595483118095,
8.16439679232994));
#16706=CARTESIAN_POINT('Ctrl Pts',(1.47018674401621E-11,-111.420483118095,
8.16439679232146));
#16707=CARTESIAN_POINT('Ctrl Pts',(4.71371668583241,-111.245483118095,8.16439679231297));
#16708=CARTESIAN_POINT('Ctrl Pts',(7.07057502873392,-111.070483118095,4.082198396148));
#16709=CARTESIAN_POINT('Ctrl Pts',(9.42743337163542,-110.895483118095,-1.69756769845304E-11));
#16710=CARTESIAN_POINT('Ctrl Pts',(7.07057502871922,-110.720483118095,-4.08219839617346));
#16711=CARTESIAN_POINT('Ctrl Pts',(4.71371668580301,-110.545483118095,-8.16439679232994));
#16712=CARTESIAN_POINT('Ctrl Pts',(-1.4702867290402E-11,-110.370483118095,
-8.16439679232146));
#16713=CARTESIAN_POINT('Ctrl Pts',(-4.71371668583241,-110.195483118095,
-8.16439679231297));
#16714=CARTESIAN_POINT('Ctrl Pts',(-7.07057502873392,-110.020483118095,
-4.082198396148));
#16715=CARTESIAN_POINT('Ctrl Pts',(-9.42743337163542,-109.845483118095,
1.69768315121407E-11));
#16716=CARTESIAN_POINT('Ctrl Pts',(-7.07057502871922,-109.670483118095,
4.08219839617346));
#16717=CARTESIAN_POINT('Ctrl Pts',(-4.71371668580301,-109.495483118095,
8.16439679232994));
#16718=CARTESIAN_POINT('Ctrl Pts',(1.47018674401621E-11,-109.320483118095,
8.16439679232146));
#16719=CARTESIAN_POINT('Ctrl Pts',(4.71371668583241,-109.145483118095,8.16439679231297));
#16720=CARTESIAN_POINT('Ctrl Pts',(7.07057502873392,-108.970483118095,4.082198396148));
#16721=CARTESIAN_POINT('Ctrl Pts',(9.42743337163542,-108.795483118095,-1.69756769845304E-11));
#16722=CARTESIAN_POINT('Ctrl Pts',(7.07057502871922,-108.620483118095,-4.08219839617346));
#16723=CARTESIAN_POINT('Ctrl Pts',(4.71371668580301,-108.445483118095,-8.16439679232994));
#16724=CARTESIAN_POINT('Ctrl Pts',(-1.4702867290402E-11,-108.270483118095,
-8.16439679232146));
#16725=CARTESIAN_POINT('Ctrl Pts',(-4.71371668583241,-108.095483118095,
-8.16439679231297));
#16726=CARTESIAN_POINT('Ctrl Pts',(-7.07057502873392,-107.920483118095,
-4.082198396148));
#16727=CARTESIAN_POINT('Ctrl Pts',(-9.42743337163542,-107.745483118095,
1.69768315121407E-11));
#16728=CARTESIAN_POINT('Ctrl Pts',(-7.07057502871922,-107.570483118095,
4.08219839617346));
#16729=CARTESIAN_POINT('Ctrl Pts',(-4.71371668580301,-107.395483118095,
8.16439679232994));
#16730=CARTESIAN_POINT('Ctrl Pts',(1.47018674401621E-11,-107.220483118095,
8.16439679232146));
#16731=CARTESIAN_POINT('Ctrl Pts',(4.71371668583241,-107.045483118095,8.16439679231297));
#16732=CARTESIAN_POINT('Ctrl Pts',(7.07057502873392,-106.870483118095,4.082198396148));
#16733=CARTESIAN_POINT('Ctrl Pts',(9.42743337163542,-106.695483118095,-1.69756769845304E-11));
#16734=CARTESIAN_POINT('Ctrl Pts',(7.07057502871922,-106.520483118095,-4.08219839617346));
#16735=CARTESIAN_POINT('Ctrl Pts',(4.71371668580301,-106.345483118095,-8.16439679232994));
#16736=CARTESIAN_POINT('Ctrl Pts',(-1.4702867290402E-11,-106.170483118095,
-8.16439679232146));
#16737=CARTESIAN_POINT('Ctrl Pts',(-4.71371668583241,-105.995483118095,
-8.16439679231297));
#16738=CARTESIAN_POINT('Ctrl Pts',(-7.07057502873392,-105.820483118095,
-4.082198396148));
#16739=CARTESIAN_POINT('Ctrl Pts',(-9.42743337163542,-105.645483118095,
1.69768315121407E-11));
#16740=CARTESIAN_POINT('Ctrl Pts',(-7.07057502871922,-105.470483118095,
4.08219839617346));
#16741=CARTESIAN_POINT('Ctrl Pts',(-4.71371668580301,-105.295483118095,
8.16439679232994));
#16742=CARTESIAN_POINT('Ctrl Pts',(1.47018674401621E-11,-105.120483118095,
8.16439679232146));
#16743=CARTESIAN_POINT('Ctrl Pts',(4.71371668583241,-104.945483118095,8.16439679231297));
#16744=CARTESIAN_POINT('Ctrl Pts',(7.07057502873392,-104.770483118095,4.082198396148));
#16745=CARTESIAN_POINT('Ctrl Pts',(9.42743337163542,-104.595483118095,-1.69756769845304E-11));
#16746=CARTESIAN_POINT('Ctrl Pts',(7.07057502871922,-104.420483118095,-4.08219839617346));
#16747=CARTESIAN_POINT('Ctrl Pts',(4.71371668580301,-104.245483118095,-8.16439679232994));
#16748=CARTESIAN_POINT('Ctrl Pts',(-1.4702867290402E-11,-104.070483118095,
-8.16439679232146));
#16749=CARTESIAN_POINT('Ctrl Pts',(-4.71371668583241,-103.895483118095,
-8.16439679231297));
#16750=CARTESIAN_POINT('Ctrl Pts',(-7.07057502873392,-103.720483118095,
-4.082198396148));
#16751=CARTESIAN_POINT('Ctrl Pts',(-9.42743337163542,-103.545483118095,
1.69768315121407E-11));
#16752=CARTESIAN_POINT('Ctrl Pts',(-7.07057502871922,-103.370483118095,
4.08219839617346));
#16753=CARTESIAN_POINT('Ctrl Pts',(-4.71371668580301,-103.195483118095,
8.16439679232994));
#16754=CARTESIAN_POINT('Ctrl Pts',(1.47018674401621E-11,-103.020483118095,
8.16439679232146));
#16755=CARTESIAN_POINT('Ctrl Pts',(4.71371668583241,-102.845483118095,8.16439679231297));
#16756=CARTESIAN_POINT('Ctrl Pts',(7.07057502873392,-102.670483118095,4.082198396148));
#16757=CARTESIAN_POINT('Ctrl Pts',(9.42743337163542,-102.495483118095,-1.69756769845304E-11));
#16758=CARTESIAN_POINT('Ctrl Pts',(7.07057502871922,-102.320483118095,-4.08219839617346));
#16759=CARTESIAN_POINT('Ctrl Pts',(4.71371668580301,-102.145483118095,-8.16439679232994));
#16760=CARTESIAN_POINT('Ctrl Pts',(-1.4702867290402E-11,-101.970483118095,
-8.16439679232146));
#16761=CARTESIAN_POINT('Ctrl Pts',(-4.71371668583241,-101.795483118095,
-8.16439679231297));
#16762=CARTESIAN_POINT('Ctrl Pts',(-7.07057502873392,-101.620483118095,
-4.082198396148));
#16763=CARTESIAN_POINT('Ctrl Pts',(-9.42743337163542,-101.445483118095,
1.69768315121407E-11));
#16764=CARTESIAN_POINT('Ctrl Pts',(-7.07057502871922,-101.270483118095,
4.08219839617346));
#16765=CARTESIAN_POINT('Ctrl Pts',(-4.71371668580301,-101.095483118095,
8.16439679232994));
#16766=CARTESIAN_POINT('Ctrl Pts',(1.47018674401621E-11,-100.920483118095,
8.16439679232146));
#16767=CARTESIAN_POINT('Ctrl Pts',(4.71371668583241,-100.745483118095,8.16439679231297));
#16768=CARTESIAN_POINT('Ctrl Pts',(7.07057502873392,-100.570483118095,4.082198396148));
#16769=CARTESIAN_POINT('Ctrl Pts',(9.42743337163542,-100.395483118095,-1.69756769845304E-11));
#16770=CARTESIAN_POINT('Ctrl Pts',(7.07057502871922,-100.220483118095,-4.08219839617346));
#16771=CARTESIAN_POINT('Ctrl Pts',(4.71371668580301,-100.045483118095,-8.16439679232994));
#16772=CARTESIAN_POINT('Ctrl Pts',(-1.4702867290402E-11,-99.8704831180952,
-8.16439679232146));
#16773=CARTESIAN_POINT('Ctrl Pts',(-4.71371668583241,-99.6954831180952,
-8.16439679231297));
#16774=CARTESIAN_POINT('Ctrl Pts',(-7.07057502873392,-99.5204831180952,
-4.082198396148));
#16775=CARTESIAN_POINT('Ctrl Pts',(-9.42743337163542,-99.3454831180952,
1.69768315121407E-11));
#16776=CARTESIAN_POINT('Ctrl Pts',(-7.07057502871922,-99.1704831180952,
4.08219839617346));
#16777=CARTESIAN_POINT('Ctrl Pts',(-4.71371668580301,-98.9954831180952,
8.16439679232994));
#16778=CARTESIAN_POINT('Ctrl Pts',(1.47018674401621E-11,-98.8204831180952,
8.16439679232146));
#16779=CARTESIAN_POINT('Ctrl Pts',(4.71371668583241,-98.6454831180952,8.16439679231297));
#16780=CARTESIAN_POINT('Ctrl Pts',(7.07057502873392,-98.4704831180952,4.082198396148));
#16781=CARTESIAN_POINT('Ctrl Pts',(9.42743337163542,-98.2954831180952,-1.69756769845304E-11));
#16782=CARTESIAN_POINT('Ctrl Pts',(7.07057502871922,-98.1204831180952,-4.08219839617346));
#16783=CARTESIAN_POINT('Ctrl Pts',(4.71371668580301,-97.9454831180952,-8.16439679232994));
#16784=CARTESIAN_POINT('Ctrl Pts',(-1.4702867290402E-11,-97.7704831180952,
-8.16439679232146));
#16785=CARTESIAN_POINT('Ctrl Pts',(-4.71371668583241,-97.5954831180952,
-8.16439679231297));
#16786=CARTESIAN_POINT('Ctrl Pts',(-7.07057502873392,-97.4204831180952,
-4.082198396148));
#16787=CARTESIAN_POINT('Ctrl Pts',(-9.42743337163542,-97.2454831180952,
1.69768315121407E-11));
#16788=CARTESIAN_POINT('Ctrl Pts',(-7.07057502871922,-97.0704831180952,
4.08219839617346));
#16789=CARTESIAN_POINT('Ctrl Pts',(-4.71371668580301,-96.8954831180952,
8.16439679232994));
#16790=CARTESIAN_POINT('Ctrl Pts',(1.47018674401621E-11,-96.7204831180952,
8.16439679232146));
#16791=CARTESIAN_POINT('Ctrl Pts',(4.71371668583241,-96.5454831180952,8.16439679231297));
#16792=CARTESIAN_POINT('Ctrl Pts',(7.07057502873392,-96.3704831180952,4.082198396148));
#16793=CARTESIAN_POINT('Ctrl Pts',(9.42743337163542,-96.1954831180952,-1.69756769845304E-11));
#16794=CARTESIAN_POINT('Ctrl Pts',(7.07057502871922,-96.0204831180952,-4.08219839617346));
#16795=CARTESIAN_POINT('Ctrl Pts',(4.71371668580301,-95.8454831180952,-8.16439679232994));
#16796=CARTESIAN_POINT('Ctrl Pts',(-1.4702867290402E-11,-95.6704831180952,
-8.16439679232146));
#16797=CARTESIAN_POINT('Ctrl Pts',(-4.71371668583241,-95.4954831180952,
-8.16439679231297));
#16798=CARTESIAN_POINT('Ctrl Pts',(-7.07057502873392,-95.3204831180952,
-4.082198396148));
#16799=CARTESIAN_POINT('Ctrl Pts',(-9.42743337163542,-95.1454831180952,
1.69768315121407E-11));
#16800=CARTESIAN_POINT('Ctrl Pts',(-7.07057502871922,-94.9704831180952,
4.08219839617346));
#16801=CARTESIAN_POINT('Ctrl Pts',(-4.71371668580301,-94.7954831180952,
8.16439679232994));
#16802=CARTESIAN_POINT('Ctrl Pts',(1.47018674401621E-11,-94.6204831180952,
8.16439679232146));
#16803=CARTESIAN_POINT('Ctrl Pts',(4.71371668583241,-94.4454831180952,8.16439679231297));
#16804=CARTESIAN_POINT('Ctrl Pts',(7.07057502873392,-94.2704831180952,4.082198396148));
#16805=CARTESIAN_POINT('Ctrl Pts',(9.42743337163542,-94.0954831180952,-1.69756769845304E-11));
#16806=CARTESIAN_POINT('Ctrl Pts',(7.07057502871922,-93.9204831180952,-4.08219839617346));
#16807=CARTESIAN_POINT('Ctrl Pts',(4.71371668580301,-93.7454831180952,-8.16439679232994));
#16808=CARTESIAN_POINT('Ctrl Pts',(-1.4702867290402E-11,-93.5704831180952,
-8.16439679232146));
#16809=CARTESIAN_POINT('Ctrl Pts',(-4.71371668583241,-93.3954831180952,
-8.16439679231297));
#16810=CARTESIAN_POINT('Ctrl Pts',(-7.07057502873392,-93.2204831180952,
-4.082198396148));
#16811=CARTESIAN_POINT('Ctrl Pts',(-9.42743337163542,-93.0454831180952,
1.69768315121407E-11));
#16812=CARTESIAN_POINT('Ctrl Pts',(-7.07057502871922,-92.8704831180952,
4.08219839617346));
#16813=CARTESIAN_POINT('Ctrl Pts',(-4.71371668580301,-92.6954831180952,
8.16439679232994));
#16814=CARTESIAN_POINT('Ctrl Pts',(1.47018674401621E-11,-92.5204831180952,
8.16439679232146));
#16815=CARTESIAN_POINT('Ctrl Pts',(4.71371668583241,-92.3454831180952,8.16439679231297));
#16816=CARTESIAN_POINT('Ctrl Pts',(7.07057502873392,-92.1704831180952,4.082198396148));
#16817=CARTESIAN_POINT('Ctrl Pts',(9.42743337163542,-91.9954831180952,-1.69756769845304E-11));
#16818=CARTESIAN_POINT('Ctrl Pts',(7.07057502871922,-91.8204831180952,-4.08219839617346));
#16819=CARTESIAN_POINT('Ctrl Pts',(4.71371668580301,-91.6454831180952,-8.16439679232994));
#16820=CARTESIAN_POINT('Ctrl Pts',(-1.4702867290402E-11,-91.4704831180952,
-8.16439679232146));
#16821=CARTESIAN_POINT('Ctrl Pts',(-4.71371668583241,-91.2954831180952,
-8.16439679231297));
#16822=CARTESIAN_POINT('Ctrl Pts',(-7.07057502873392,-91.1204831180952,
-4.082198396148));
#16823=CARTESIAN_POINT('Ctrl Pts',(-9.42743337163542,-90.9454831180952,
1.69768315121407E-11));
#16824=CARTESIAN_POINT('Ctrl Pts',(-7.07057502871922,-90.7704831180952,
4.08219839617346));
#16825=CARTESIAN_POINT('Ctrl Pts',(-4.71371668580301,-90.5954831180952,
8.16439679232994));
#16826=CARTESIAN_POINT('Ctrl Pts',(1.47018674401621E-11,-90.4204831180952,
8.16439679232146));
#16827=CARTESIAN_POINT('Ctrl Pts',(4.71371668583241,-90.2454831180952,8.16439679231297));
#16828=CARTESIAN_POINT('Ctrl Pts',(7.07057502873392,-90.0704831180952,4.082198396148));
#16829=CARTESIAN_POINT('Ctrl Pts',(9.42743337163542,-89.8954831180952,-1.69756769845304E-11));
#16830=CARTESIAN_POINT('Ctrl Pts',(7.07057502871922,-89.7204831180952,-4.08219839617346));
#16831=CARTESIAN_POINT('Ctrl Pts',(4.71371668580301,-89.5454831180952,-8.16439679232994));
#16832=CARTESIAN_POINT('Ctrl Pts',(-1.4702867290402E-11,-89.3704831180952,
-8.16439679232146));
#16833=CARTESIAN_POINT('Ctrl Pts',(-4.71371668583241,-89.1954831180952,
-8.16439679231297));
#16834=CARTESIAN_POINT('Ctrl Pts',(-7.07057502873392,-89.0204831180952,
-4.082198396148));
#16835=CARTESIAN_POINT('Ctrl Pts',(-9.42743337163542,-88.8454831180952,
1.69768315121407E-11));
#16836=CARTESIAN_POINT('Ctrl Pts',(-7.07057502871922,-88.6704831180952,
4.08219839617346));
#16837=CARTESIAN_POINT('Ctrl Pts',(-4.71371668580301,-88.4954831180952,
8.16439679232994));
#16838=CARTESIAN_POINT('Ctrl Pts',(1.47018674401621E-11,-88.3204831180952,
8.16439679232146));
#16839=CARTESIAN_POINT('Ctrl Pts',(4.71371668583241,-88.1454831180952,8.16439679231297));
#16840=CARTESIAN_POINT('Ctrl Pts',(7.07057502873392,-87.9704831180952,4.082198396148));
#16841=CARTESIAN_POINT('Ctrl Pts',(9.42743337163542,-87.7954831180952,-1.69756769845304E-11));
#16842=CARTESIAN_POINT('Ctrl Pts',(7.07057502871922,-87.6204831180952,-4.08219839617346));
#16843=CARTESIAN_POINT('Ctrl Pts',(4.71371668580301,-87.4454831180952,-8.16439679232994));
#16844=CARTESIAN_POINT('Ctrl Pts',(-1.4702867290402E-11,-87.2704831180952,
-8.16439679232146));
#16845=CARTESIAN_POINT('Ctrl Pts',(-4.71371668583241,-87.0954831180952,
-8.16439679231297));
#16846=CARTESIAN_POINT('Ctrl Pts',(-7.07057502873392,-86.9204831180952,
-4.082198396148));
#16847=CARTESIAN_POINT('Ctrl Pts',(-9.42743337163542,-86.7454831180952,
1.69768315121407E-11));
#16848=CARTESIAN_POINT('Ctrl Pts',(-7.07057502871922,-86.5704831180952,
4.08219839617346));
#16849=CARTESIAN_POINT('Ctrl Pts',(-4.71371668580301,-86.3954831180952,
8.16439679232994));
#16850=CARTESIAN_POINT('Ctrl Pts',(1.47018674401621E-11,-86.2204831180952,
8.16439679232146));
#16851=CARTESIAN_POINT('Ctrl Pts',(4.71371668583241,-86.0454831180952,8.16439679231297));
#16852=CARTESIAN_POINT('Ctrl Pts',(7.07057502873392,-85.8704831180952,4.082198396148));
#16853=CARTESIAN_POINT('Ctrl Pts',(9.42743337163542,-85.6954831180952,-1.69756769845304E-11));
#16854=CARTESIAN_POINT('Ctrl Pts',(7.07057502871922,-85.5204831180952,-4.08219839617346));
#16855=CARTESIAN_POINT('Ctrl Pts',(4.71371668580301,-85.3454831180952,-8.16439679232994));
#16856=CARTESIAN_POINT('Ctrl Pts',(-1.4702867290402E-11,-85.1704831180952,
-8.16439679232146));
#16857=CARTESIAN_POINT('Ctrl Pts',(-4.71371668583241,-84.9954831180952,
-8.16439679231297));
#16858=CARTESIAN_POINT('Ctrl Pts',(-7.07057502873392,-84.8204831180952,
-4.082198396148));
#16859=CARTESIAN_POINT('Ctrl Pts',(-9.42743337163542,-84.6454831180952,
1.69768315121407E-11));
#16860=CARTESIAN_POINT('Ctrl Pts',(-7.07057502871922,-84.4704831180952,
4.08219839617346));
#16861=CARTESIAN_POINT('Ctrl Pts',(-4.71371668580301,-84.2954831180952,
8.16439679232994));
#16862=CARTESIAN_POINT('Ctrl Pts',(1.47018674401621E-11,-84.1204831180952,
8.16439679232146));
#16863=CARTESIAN_POINT('Ctrl Pts',(4.71371668583241,-83.9454831180952,8.16439679231297));
#16864=CARTESIAN_POINT('Ctrl Pts',(7.07057502873392,-83.7704831180952,4.082198396148));
#16865=CARTESIAN_POINT('Ctrl Pts',(9.42743337163542,-83.5954831180952,-1.69756769845304E-11));
#16866=CARTESIAN_POINT('Ctrl Pts',(7.07057502871922,-83.4204831180952,-4.08219839617346));
#16867=CARTESIAN_POINT('Ctrl Pts',(4.71371668580301,-83.2454831180952,-8.16439679232994));
#16868=CARTESIAN_POINT('Ctrl Pts',(-1.4702867290402E-11,-83.0704831180952,
-8.16439679232146));
#16869=CARTESIAN_POINT('Ctrl Pts',(-4.71371668583241,-82.8954831180952,
-8.16439679231297));
#16870=CARTESIAN_POINT('Ctrl Pts',(-7.07057502873392,-82.7204831180952,
-4.082198396148));
#16871=CARTESIAN_POINT('Ctrl Pts',(-9.42743337163542,-82.5454831180952,
1.69768315121407E-11));
#16872=CARTESIAN_POINT('Ctrl Pts',(-7.07057502871922,-82.3704831180952,
4.08219839617346));
#16873=CARTESIAN_POINT('Ctrl Pts',(-4.71371668580301,-82.1954831180952,
8.16439679232994));
#16874=CARTESIAN_POINT('Ctrl Pts',(1.47018674401621E-11,-82.0204831180952,
8.16439679232146));
#16875=CARTESIAN_POINT('Ctrl Pts',(4.71371668583241,-81.8454831180952,8.16439679231297));
#16876=CARTESIAN_POINT('Ctrl Pts',(7.07057502873392,-81.6704831180952,4.082198396148));
#16877=CARTESIAN_POINT('Ctrl Pts',(9.42743337163542,-81.4954831180952,-1.69756769845304E-11));
#16878=CARTESIAN_POINT('Ctrl Pts',(7.07057502871922,-81.3204831180952,-4.08219839617346));
#16879=CARTESIAN_POINT('Ctrl Pts',(4.71371668580301,-81.1454831180953,-8.16439679232994));
#16880=CARTESIAN_POINT('Ctrl Pts',(-1.4702867290402E-11,-80.9704831180952,
-8.16439679232146));
#16881=CARTESIAN_POINT('Ctrl Pts',(-4.71371668583241,-80.7954831180952,
-8.16439679231297));
#16882=CARTESIAN_POINT('Ctrl Pts',(-7.07057502873392,-80.6204831180952,
-4.082198396148));
#16883=CARTESIAN_POINT('Ctrl Pts',(-9.42743337163542,-80.4454831180952,
1.69768315121407E-11));
#16884=CARTESIAN_POINT('Ctrl Pts',(-7.07057502871922,-80.2704831180952,
4.08219839617346));
#16885=CARTESIAN_POINT('Ctrl Pts',(-4.71371668580301,-80.0954831180952,
8.16439679232994));
#16886=CARTESIAN_POINT('Ctrl Pts',(1.47018674401621E-11,-79.9204831180952,
8.16439679232146));
#16887=CARTESIAN_POINT('Ctrl Pts',(4.71371668583241,-79.7454831180953,8.16439679231297));
#16888=CARTESIAN_POINT('Ctrl Pts',(7.07057502873392,-79.5704831180952,4.082198396148));
#16889=CARTESIAN_POINT('Ctrl Pts',(9.42743337163542,-79.3954831180952,-1.69756769845304E-11));
#16890=CARTESIAN_POINT('Ctrl Pts',(7.07057502871922,-79.2204831180952,-4.08219839617346));
#16891=CARTESIAN_POINT('Ctrl Pts',(4.71371668580301,-79.0454831180952,-8.16439679232994));
#16892=CARTESIAN_POINT('Ctrl Pts',(-1.4702867290402E-11,-78.8704831180952,
-8.16439679232146));
#16893=CARTESIAN_POINT('Ctrl Pts',(-4.71371668583241,-78.6954831180953,
-8.16439679231297));
#16894=CARTESIAN_POINT('Ctrl Pts',(-7.07057502873392,-78.5204831180952,
-4.082198396148));
#16895=CARTESIAN_POINT('Ctrl Pts',(-9.42743337163542,-78.3454831180952,
1.69768315121407E-11));
#16896=CARTESIAN_POINT('Ctrl Pts',(-7.07057502871922,-78.1704831180953,
4.08219839617346));
#16897=CARTESIAN_POINT('Ctrl Pts',(-4.71371668580301,-77.9954831180953,
8.16439679232994));
#16898=CARTESIAN_POINT('Ctrl Pts',(1.47018674401621E-11,-77.8204831180952,
8.16439679232146));
#16899=CARTESIAN_POINT('Ctrl Pts',(4.71371668583241,-77.6454831180953,8.16439679231297));
#16900=CARTESIAN_POINT('Ctrl Pts',(7.07057502873392,-77.4704831180952,4.082198396148));
#16901=CARTESIAN_POINT('Ctrl Pts',(9.42743337163542,-77.2954831180952,-1.69756769845304E-11));
#16902=CARTESIAN_POINT('Ctrl Pts',(7.07057502871922,-77.1204831180952,-4.08219839617346));
#16903=CARTESIAN_POINT('Ctrl Pts',(4.71371668580301,-76.9454831180952,-8.16439679232994));
#16904=CARTESIAN_POINT('Ctrl Pts',(-1.4702867290402E-11,-76.7704831180952,
-8.16439679232146));
#16905=CARTESIAN_POINT('Ctrl Pts',(-4.71371668583241,-76.5954831180953,
-8.16439679231297));
#16906=CARTESIAN_POINT('Ctrl Pts',(-7.07057502873392,-76.4204831180952,
-4.082198396148));
#16907=CARTESIAN_POINT('Ctrl Pts',(-9.42743337163542,-76.2454831180952,
1.69768315121407E-11));
#16908=CARTESIAN_POINT('Ctrl Pts',(-7.07057502871922,-76.0704831180952,
4.08219839617346));
#16909=CARTESIAN_POINT('Ctrl Pts',(-4.71371668580301,-75.8954831180952,
8.16439679232994));
#16910=CARTESIAN_POINT('Ctrl Pts',(1.47018674401621E-11,-75.7204831180952,
8.16439679232146));
#16911=CARTESIAN_POINT('Ctrl Pts',(4.71371668583241,-75.5454831180952,8.16439679231297));
#16912=CARTESIAN_POINT('Ctrl Pts',(7.07057502873392,-75.3704831180952,4.082198396148));
#16913=CARTESIAN_POINT('Ctrl Pts',(9.42743337163542,-75.1954831180952,-1.69756769845304E-11));
#16914=CARTESIAN_POINT('Ctrl Pts',(7.07057502871922,-75.0204831180952,-4.08219839617346));
#16915=CARTESIAN_POINT('Ctrl Pts',(4.71371668580301,-74.8454831180952,-8.16439679232994));
#16916=CARTESIAN_POINT('Ctrl Pts',(-1.4702867290402E-11,-74.6704831180952,
-8.16439679232146));
#16917=CARTESIAN_POINT('Ctrl Pts',(-4.71371668583241,-74.4954831180953,
-8.16439679231297));
#16918=CARTESIAN_POINT('Ctrl Pts',(-7.07057502873392,-74.3204831180952,
-4.082198396148));
#16919=CARTESIAN_POINT('Ctrl Pts',(-9.42743337163542,-74.1454831180952,
1.69768315121407E-11));
#16920=CARTESIAN_POINT('Ctrl Pts',(-7.07057502871922,-73.9704831180952,
4.08219839617346));
#16921=CARTESIAN_POINT('Ctrl Pts',(-4.71371668580301,-73.7954831180952,
8.16439679232994));
#16922=CARTESIAN_POINT('Ctrl Pts',(1.47018674401621E-11,-73.6204831180952,
8.16439679232146));
#16923=CARTESIAN_POINT('Ctrl Pts',(4.71371668583241,-73.4454831180953,8.16439679231297));
#16924=CARTESIAN_POINT('Ctrl Pts',(7.07057502873392,-73.2704831180952,4.082198396148));
#16925=CARTESIAN_POINT('Ctrl Pts',(9.42743337163542,-73.0954831180953,-1.69756769845304E-11));
#16926=CARTESIAN_POINT('Ctrl Pts',(7.07057502871922,-72.9204831180952,-4.08219839617346));
#16927=CARTESIAN_POINT('Ctrl Pts',(4.71371668580301,-72.7454831180952,-8.16439679232994));
#16928=CARTESIAN_POINT('Ctrl Pts',(-1.4702867290402E-11,-72.5704831180953,
-8.16439679232146));
#16929=CARTESIAN_POINT('Ctrl Pts',(-4.71371668583241,-72.3954831180953,
-8.16439679231297));
#16930=CARTESIAN_POINT('Ctrl Pts',(-7.07057502873392,-72.2204831180952,
-4.082198396148));
#16931=CARTESIAN_POINT('Ctrl Pts',(-9.42743337163542,-72.0454831180953,
1.69768315121407E-11));
#16932=CARTESIAN_POINT('Ctrl Pts',(-7.07057502871922,-71.8704831180952,
4.08219839617346));
#16933=CARTESIAN_POINT('Ctrl Pts',(-4.71371668580301,-71.6954831180952,
8.16439679232994));
#16934=CARTESIAN_POINT('Ctrl Pts',(1.47018674401621E-11,-71.5204831180953,
8.16439679232146));
#16935=CARTESIAN_POINT('Ctrl Pts',(4.71371668583241,-71.3454831180952,8.16439679231297));
#16936=CARTESIAN_POINT('Ctrl Pts',(7.07057502873392,-71.1704831180952,4.082198396148));
#16937=CARTESIAN_POINT('Ctrl Pts',(9.42743337163542,-70.9954831180953,-1.69756769845304E-11));
#16938=CARTESIAN_POINT('Ctrl Pts',(7.07057502871922,-70.8204831180952,-4.08219839617346));
#16939=CARTESIAN_POINT('Ctrl Pts',(4.71371668580301,-70.6454831180952,-8.16439679232994));
#16940=CARTESIAN_POINT('Ctrl Pts',(-1.4702867290402E-11,-70.4704831180953,
-8.16439679232146));
#16941=CARTESIAN_POINT('Ctrl Pts',(-4.71371668583241,-70.2954831180952,
-8.16439679231297));
#16942=CARTESIAN_POINT('Ctrl Pts',(-7.07057502873392,-70.1204831180952,
-4.082198396148));
#16943=CARTESIAN_POINT('Ctrl Pts',(-9.42743337163542,-69.9454831180953,
1.69768315121407E-11));
#16944=CARTESIAN_POINT('Ctrl Pts',(-7.07057502871922,-69.7704831180953,
4.08219839617346));
#16945=CARTESIAN_POINT('Ctrl Pts',(-4.71371668580301,-69.5954831180952,
8.16439679232994));
#16946=CARTESIAN_POINT('Ctrl Pts',(1.47018674401621E-11,-69.4204831180953,
8.16439679232146));
#16947=CARTESIAN_POINT('Ctrl Pts',(4.71371668583241,-69.2454831180953,8.16439679231297));
#16948=CARTESIAN_POINT('Ctrl Pts',(7.07057502873392,-69.0704831180953,4.082198396148));
#16949=CARTESIAN_POINT('Ctrl Pts',(9.42743337163542,-68.8954831180953,-1.69756769845304E-11));
#16950=CARTESIAN_POINT('Ctrl Pts',(7.07057502871922,-68.7204831180952,-4.08219839617346));
#16951=CARTESIAN_POINT('Ctrl Pts',(4.71371668580301,-68.5454831180952,-8.16439679232994));
#16952=CARTESIAN_POINT('Ctrl Pts',(-1.4702867290402E-11,-68.3704831180953,
-8.16439679232146));
#16953=CARTESIAN_POINT('Ctrl Pts',(-4.71371668583241,-68.1954831180952,
-8.16439679231297));
#16954=CARTESIAN_POINT('Ctrl Pts',(-7.07057502873392,-68.0204831180953,
-4.082198396148));
#16955=CARTESIAN_POINT('Ctrl Pts',(-9.42743337163542,-67.8454831180953,
1.69768315121407E-11));
#16956=CARTESIAN_POINT('Ctrl Pts',(-7.07057502871922,-67.6704831180952,
4.08219839617346));
#16957=CARTESIAN_POINT('Ctrl Pts',(-4.71371668580301,-67.4954831180953,
8.16439679232994));
#16958=CARTESIAN_POINT('Ctrl Pts',(1.47018674401621E-11,-67.3204831180953,
8.16439679232146));
#16959=CARTESIAN_POINT('Ctrl Pts',(4.71371668583241,-67.1454831180952,8.16439679231297));
#16960=CARTESIAN_POINT('Ctrl Pts',(7.07057502873392,-66.9704831180952,4.082198396148));
#16961=CARTESIAN_POINT('Ctrl Pts',(9.42743337163542,-66.7954831180953,-1.69756769845304E-11));
#16962=CARTESIAN_POINT('Ctrl Pts',(7.07057502871922,-66.6204831180952,-4.08219839617346));
#16963=CARTESIAN_POINT('Ctrl Pts',(4.71371668580301,-66.4454831180952,-8.16439679232994));
#16964=CARTESIAN_POINT('Ctrl Pts',(-1.4702867290402E-11,-66.2704831180953,
-8.16439679232146));
#16965=CARTESIAN_POINT('Ctrl Pts',(-4.71371668583241,-66.0954831180952,
-8.16439679231297));
#16966=CARTESIAN_POINT('Ctrl Pts',(-7.07057502873392,-65.9204831180952,
-4.082198396148));
#16967=CARTESIAN_POINT('Ctrl Pts',(-9.42743337163542,-65.7454831180953,
1.69768315121407E-11));
#16968=CARTESIAN_POINT('Ctrl Pts',(-7.07057502871922,-65.5704831180953,
4.08219839617346));
#16969=CARTESIAN_POINT('Ctrl Pts',(-4.71371668580301,-65.3954831180953,
8.16439679232994));
#16970=CARTESIAN_POINT('Ctrl Pts',(1.47018674401621E-11,-65.2204831180952,
8.16439679232146));
#16971=CARTESIAN_POINT('Ctrl Pts',(4.71371668583241,-65.0454831180952,8.16439679231297));
#16972=CARTESIAN_POINT('Ctrl Pts',(7.07057502873392,-64.8704831180953,4.082198396148));
#16973=CARTESIAN_POINT('Ctrl Pts',(9.42743337163542,-64.6954831180953,-1.69756769845304E-11));
#16974=CARTESIAN_POINT('Ctrl Pts',(7.07057502871922,-64.5204831180953,-4.08219839617346));
#16975=CARTESIAN_POINT('Ctrl Pts',(4.71371668580301,-64.3454831180953,-8.16439679232994));
#16976=CARTESIAN_POINT('Ctrl Pts',(-1.4702867290402E-11,-64.1704831180952,
-8.16439679232146));
#16977=CARTESIAN_POINT('Ctrl Pts',(-4.71371668583241,-63.9954831180953,
-8.16439679231297));
#16978=CARTESIAN_POINT('Ctrl Pts',(-7.07057502873392,-63.8204831180953,
-4.082198396148));
#16979=CARTESIAN_POINT('Ctrl Pts',(-9.42743337163542,-63.6454831180953,
1.69768315121407E-11));
#16980=CARTESIAN_POINT('Ctrl Pts',(-7.07057502871922,-63.4704831180953,
4.08219839617346));
#16981=CARTESIAN_POINT('Ctrl Pts',(-4.71371668580301,-63.2954831180953,
8.16439679232994));
#16982=CARTESIAN_POINT('Ctrl Pts',(1.47018674401621E-11,-63.1204831180953,
8.16439679232146));
#16983=CARTESIAN_POINT('Ctrl Pts',(4.71371668583241,-62.9454831180952,8.16439679231297));
#16984=CARTESIAN_POINT('Ctrl Pts',(7.07057502873392,-62.7704831180953,4.082198396148));
#16985=CARTESIAN_POINT('Ctrl Pts',(9.42743337163542,-62.5954831180953,-1.69756769845304E-11));
#16986=CARTESIAN_POINT('Ctrl Pts',(7.07057502871922,-62.4204831180953,-4.08219839617346));
#16987=CARTESIAN_POINT('Ctrl Pts',(4.71371668580301,-62.2454831180953,-8.16439679232994));
#16988=CARTESIAN_POINT('Ctrl Pts',(-1.4702867290402E-11,-62.0704831180953,
-8.16439679232146));
#16989=CARTESIAN_POINT('Ctrl Pts',(-4.71371668583241,-61.8954831180952,
-8.16439679231297));
#16990=CARTESIAN_POINT('Ctrl Pts',(-7.07057502873392,-61.7204831180953,
-4.082198396148));
#16991=CARTESIAN_POINT('Ctrl Pts',(-9.42743337163542,-61.5454831180953,
1.69768315121407E-11));
#16992=CARTESIAN_POINT('Ctrl Pts',(-7.07057502871922,-61.3704831180953,
4.08219839617346));
#16993=CARTESIAN_POINT('Ctrl Pts',(-4.71371668580301,-61.1954831180953,
8.16439679232994));
#16994=CARTESIAN_POINT('Ctrl Pts',(1.47018674401621E-11,-61.0204831180953,
8.16439679232146));
#16995=CARTESIAN_POINT('Ctrl Pts',(4.71371668583241,-60.8454831180953,8.16439679231297));
#16996=CARTESIAN_POINT('Ctrl Pts',(7.07057502873392,-60.6704831180953,4.082198396148));
#16997=CARTESIAN_POINT('Ctrl Pts',(9.42743337163542,-60.4954831180953,-1.69756769845304E-11));
#16998=CARTESIAN_POINT('Ctrl Pts',(7.07057502871922,-60.3204831180953,-4.08219839617346));
#16999=CARTESIAN_POINT('Ctrl Pts',(4.71371668580301,-60.1454831180953,-8.16439679232994));
#17000=CARTESIAN_POINT('Ctrl Pts',(-1.4702867290402E-11,-59.9704831180953,
-8.16439679232146));
#17001=CARTESIAN_POINT('Ctrl Pts',(-4.71371668583241,-59.7954831180953,
-8.16439679231297));
#17002=CARTESIAN_POINT('Ctrl Pts',(-7.07057502873392,-59.6204831180953,
-4.082198396148));
#17003=CARTESIAN_POINT('Ctrl Pts',(-9.42743337163542,-59.4454831180953,
1.69768315121407E-11));
#17004=CARTESIAN_POINT('Ctrl Pts',(-7.07057502871922,-59.2704831180953,
4.08219839617346));
#17005=CARTESIAN_POINT('Ctrl Pts',(-4.71371668580301,-59.0954831180953,
8.16439679232994));
#17006=CARTESIAN_POINT('Ctrl Pts',(1.47018674401621E-11,-58.9204831180953,
8.16439679232146));
#17007=CARTESIAN_POINT('Ctrl Pts',(4.71371668583241,-58.7454831180953,8.16439679231297));
#17008=CARTESIAN_POINT('Ctrl Pts',(7.07057502873392,-58.5704831180953,4.082198396148));
#17009=CARTESIAN_POINT('Ctrl Pts',(9.42743337163542,-58.3954831180953,-1.69756769845304E-11));
#17010=CARTESIAN_POINT('Ctrl Pts',(7.07057502871922,-58.2204831180953,-4.08219839617346));
#17011=CARTESIAN_POINT('Ctrl Pts',(4.71371668580301,-58.0454831180953,-8.16439679232994));
#17012=CARTESIAN_POINT('Ctrl Pts',(-1.4702867290402E-11,-57.8704831180952,
-8.16439679232146));
#17013=CARTESIAN_POINT('Ctrl Pts',(-4.71371668583241,-57.6954831180953,
-8.16439679231297));
#17014=CARTESIAN_POINT('Ctrl Pts',(-7.07057502873392,-57.5204831180953,
-4.082198396148));
#17015=CARTESIAN_POINT('Ctrl Pts',(-9.42743337163542,-57.3454831180953,
1.69768315121407E-11));
#17016=CARTESIAN_POINT('Ctrl Pts',(-7.07057502871922,-57.1704831180953,
4.08219839617346));
#17017=CARTESIAN_POINT('Ctrl Pts',(-4.71371668580301,-56.9954831180953,
8.16439679232994));
#17018=CARTESIAN_POINT('Ctrl Pts',(1.47018674401621E-11,-56.8204831180953,
8.16439679232146));
#17019=CARTESIAN_POINT('Ctrl Pts',(4.71371668583241,-56.6454831180953,8.16439679231297));
#17020=CARTESIAN_POINT('Ctrl Pts',(7.07057502873392,-56.4704831180953,4.082198396148));
#17021=CARTESIAN_POINT('Ctrl Pts',(9.42743337163542,-56.2954831180953,-1.69756769845304E-11));
#17022=CARTESIAN_POINT('Ctrl Pts',(7.07057502871922,-56.1204831180953,-4.08219839617346));
#17023=CARTESIAN_POINT('Ctrl Pts',(4.71371668580301,-55.9454831180953,-8.16439679232994));
#17024=CARTESIAN_POINT('Ctrl Pts',(-1.4702867290402E-11,-55.7704831180953,
-8.16439679232146));
#17025=CARTESIAN_POINT('Ctrl Pts',(-4.71371668583241,-55.5954831180953,
-8.16439679231297));
#17026=CARTESIAN_POINT('Ctrl Pts',(-7.07057502873392,-55.4204831180953,
-4.082198396148));
#17027=CARTESIAN_POINT('Ctrl Pts',(-9.42743337163542,-55.2454831180953,
1.69768315121407E-11));
#17028=CARTESIAN_POINT('Ctrl Pts',(-7.07057502871922,-55.0704831180953,
4.08219839617346));
#17029=CARTESIAN_POINT('Ctrl Pts',(-4.71371668580301,-54.8954831180953,
8.16439679232994));
#17030=CARTESIAN_POINT('Ctrl Pts',(1.47018674401621E-11,-54.7204831180953,
8.16439679232146));
#17031=CARTESIAN_POINT('Ctrl Pts',(4.71371668583241,-54.5454831180953,8.16439679231297));
#17032=CARTESIAN_POINT('Ctrl Pts',(7.07057502873392,-54.3704831180953,4.082198396148));
#17033=CARTESIAN_POINT('Ctrl Pts',(9.42743337163542,-54.1954831180953,-1.69756769845304E-11));
#17034=CARTESIAN_POINT('Ctrl Pts',(7.07057502871922,-54.0204831180953,-4.08219839617346));
#17035=CARTESIAN_POINT('Ctrl Pts',(4.71371668580301,-53.8454831180953,-8.16439679232994));
#17036=CARTESIAN_POINT('Ctrl Pts',(-1.4702867290402E-11,-53.6704831180953,
-8.16439679232146));
#17037=CARTESIAN_POINT('Ctrl Pts',(-4.71371668583241,-53.4954831180953,
-8.16439679231297));
#17038=CARTESIAN_POINT('Ctrl Pts',(-7.07057502873392,-53.3204831180953,
-4.082198396148));
#17039=CARTESIAN_POINT('Ctrl Pts',(-9.42743337163542,-53.1454831180953,
1.69768315121407E-11));
#17040=CARTESIAN_POINT('Ctrl Pts',(-7.07057502871922,-52.9704831180953,
4.08219839617346));
#17041=CARTESIAN_POINT('Ctrl Pts',(-4.71371668580301,-52.7954831180953,
8.16439679232994));
#17042=CARTESIAN_POINT('Ctrl Pts',(1.47018674401621E-11,-52.6204831180953,
8.16439679232146));
#17043=CARTESIAN_POINT('Ctrl Pts',(4.71371668583241,-52.4454831180953,8.16439679231297));
#17044=CARTESIAN_POINT('Ctrl Pts',(7.07057502873392,-52.2704831180953,4.082198396148));
#17045=CARTESIAN_POINT('Ctrl Pts',(9.42743337163542,-52.0954831180953,-1.69756769845304E-11));
#17046=CARTESIAN_POINT('Ctrl Pts',(7.07057502871922,-51.9204831180953,-4.08219839617346));
#17047=CARTESIAN_POINT('Ctrl Pts',(4.71371668580301,-51.7454831180953,-8.16439679232994));
#17048=CARTESIAN_POINT('Ctrl Pts',(-1.4702867290402E-11,-51.5704831180953,
-8.16439679232146));
#17049=CARTESIAN_POINT('Ctrl Pts',(-4.71371668583241,-51.3954831180953,
-8.16439679231297));
#17050=CARTESIAN_POINT('Ctrl Pts',(-7.07057502873392,-51.2204831180953,
-4.082198396148));
#17051=CARTESIAN_POINT('Ctrl Pts',(-9.42743337163542,-51.0454831180953,
1.69768315121407E-11));
#17052=CARTESIAN_POINT('Ctrl Pts',(-7.07057502871922,-50.8704831180953,
4.08219839617346));
#17053=CARTESIAN_POINT('Ctrl Pts',(-4.71371668580301,-50.6954831180953,
8.16439679232994));
#17054=CARTESIAN_POINT('Ctrl Pts',(1.47018674401621E-11,-50.5204831180953,
8.16439679232146));
#17055=CARTESIAN_POINT('Ctrl Pts',(4.71371668583241,-50.3454831180953,8.16439679231297));
#17056=CARTESIAN_POINT('Ctrl Pts',(7.07057502873392,-50.1704831180953,4.082198396148));
#17057=CARTESIAN_POINT('Ctrl Pts',(9.42743337163542,-49.9954831180953,-1.69756769845304E-11));
#17058=CARTESIAN_POINT('Ctrl Pts',(7.07057502871922,-49.8204831180953,-4.08219839617346));
#17059=CARTESIAN_POINT('Ctrl Pts',(4.71371668580301,-49.6454831180953,-8.16439679232994));
#17060=CARTESIAN_POINT('Ctrl Pts',(-1.4702867290402E-11,-49.4704831180953,
-8.16439679232146));
#17061=CARTESIAN_POINT('Ctrl Pts',(-4.71371668583241,-49.2954831180953,
-8.16439679231297));
#17062=CARTESIAN_POINT('Ctrl Pts',(-7.07057502873392,-49.1204831180953,
-4.082198396148));
#17063=CARTESIAN_POINT('Ctrl Pts',(-9.42743337163542,-48.9454831180953,
1.69768315121407E-11));
#17064=CARTESIAN_POINT('Ctrl Pts',(-7.07057502871922,-48.7704831180953,
4.08219839617346));
#17065=CARTESIAN_POINT('Ctrl Pts',(-4.71371668580301,-48.5954831180953,
8.16439679232994));
#17066=CARTESIAN_POINT('Ctrl Pts',(1.47018674401621E-11,-48.4204831180953,
8.16439679232146));
#17067=CARTESIAN_POINT('Ctrl Pts',(4.71371668583241,-48.2454831180953,8.16439679231297));
#17068=CARTESIAN_POINT('Ctrl Pts',(7.07057502873392,-48.0704831180953,4.082198396148));
#17069=CARTESIAN_POINT('Ctrl Pts',(9.42743337163542,-47.8954831180953,-1.69756769845304E-11));
#17070=CARTESIAN_POINT('Ctrl Pts',(7.07057502871922,-47.7204831180953,-4.08219839617346));
#17071=CARTESIAN_POINT('Ctrl Pts',(4.71371668580301,-47.5454831180953,-8.16439679232994));
#17072=CARTESIAN_POINT('Ctrl Pts',(-1.4702867290402E-11,-47.3704831180953,
-8.16439679232146));
#17073=CARTESIAN_POINT('Ctrl Pts',(-4.71371668583241,-47.1954831180953,
-8.16439679231297));
#17074=CARTESIAN_POINT('Ctrl Pts',(-7.07057502873392,-47.0204831180953,
-4.082198396148));
#17075=CARTESIAN_POINT('Ctrl Pts',(-9.42743337163542,-46.8454831180953,
1.69768315121407E-11));
#17076=CARTESIAN_POINT('Ctrl Pts',(-7.07057502871922,-46.6704831180953,
4.08219839617346));
#17077=CARTESIAN_POINT('Ctrl Pts',(-4.71371668580301,-46.4954831180953,
8.16439679232994));
#17078=CARTESIAN_POINT('Ctrl Pts',(1.47018674401621E-11,-46.3204831180953,
8.16439679232146));
#17079=CARTESIAN_POINT('Ctrl Pts',(4.71371668583241,-46.1454831180953,8.16439679231297));
#17080=CARTESIAN_POINT('Ctrl Pts',(7.07057502873392,-45.9704831180953,4.082198396148));
#17081=CARTESIAN_POINT('Ctrl Pts',(9.42743337163542,-45.7954831180953,-1.69756769845304E-11));
#17082=CARTESIAN_POINT('Ctrl Pts',(7.07057502871922,-45.6204831180953,-4.08219839617346));
#17083=CARTESIAN_POINT('Ctrl Pts',(4.71371668580301,-45.4454831180953,-8.16439679232994));
#17084=CARTESIAN_POINT('Ctrl Pts',(-1.4702867290402E-11,-45.2704831180953,
-8.16439679232146));
#17085=CARTESIAN_POINT('Ctrl Pts',(-4.71371668583241,-45.0954831180953,
-8.16439679231297));
#17086=CARTESIAN_POINT('Ctrl Pts',(-7.07057502873392,-44.9204831180953,
-4.082198396148));
#17087=CARTESIAN_POINT('Ctrl Pts',(-9.42743337163542,-44.7454831180953,
1.69768315121407E-11));
#17088=CARTESIAN_POINT('Ctrl Pts',(-7.07057502871922,-44.5704831180953,
4.08219839617346));
#17089=CARTESIAN_POINT('Ctrl Pts',(-4.71371668580301,-44.3954831180953,
8.16439679232994));
#17090=CARTESIAN_POINT('Ctrl Pts',(1.47018674401621E-11,-44.2204831180953,
8.16439679232146));
#17091=CARTESIAN_POINT('Ctrl Pts',(4.71371668583241,-44.0454831180953,8.16439679231297));
#17092=CARTESIAN_POINT('Ctrl Pts',(7.07057502873392,-43.8704831180953,4.082198396148));
#17093=CARTESIAN_POINT('Ctrl Pts',(9.42743337163542,-43.6954831180953,-1.69756769845304E-11));
#17094=CARTESIAN_POINT('Ctrl Pts',(7.07057502871922,-43.5204831180953,-4.08219839617346));
#17095=CARTESIAN_POINT('Ctrl Pts',(4.71371668580301,-43.3454831180953,-8.16439679232994));
#17096=CARTESIAN_POINT('Ctrl Pts',(-1.4702867290402E-11,-43.1704831180953,
-8.16439679232146));
#17097=CARTESIAN_POINT('Ctrl Pts',(-4.71371668583241,-42.9954831180953,
-8.16439679231297));
#17098=CARTESIAN_POINT('Ctrl Pts',(-7.07057502873392,-42.8204831180953,
-4.082198396148));
#17099=CARTESIAN_POINT('Ctrl Pts',(-9.42743337163542,-42.6454831180953,
1.69768315121407E-11));
#17100=CARTESIAN_POINT('Ctrl Pts',(-7.07057502871922,-42.4704831180953,
4.08219839617346));
#17101=CARTESIAN_POINT('Ctrl Pts',(-4.71371668580301,-42.2954831180953,
8.16439679232994));
#17102=CARTESIAN_POINT('Ctrl Pts',(1.47018674401621E-11,-42.1204831180953,
8.16439679232146));
#17103=CARTESIAN_POINT('Ctrl Pts',(4.71371668583241,-41.9454831180953,8.16439679231297));
#17104=CARTESIAN_POINT('Ctrl Pts',(7.07057502873392,-41.7704831180953,4.082198396148));
#17105=CARTESIAN_POINT('Ctrl Pts',(9.42743337163542,-41.5954831180953,-1.69756769845304E-11));
#17106=CARTESIAN_POINT('Ctrl Pts',(7.07057502871922,-41.4204831180953,-4.08219839617346));
#17107=CARTESIAN_POINT('Ctrl Pts',(4.71371668580301,-41.2454831180953,-8.16439679232994));
#17108=CARTESIAN_POINT('Ctrl Pts',(-1.4702867290402E-11,-41.0704831180953,
-8.16439679232146));
#17109=CARTESIAN_POINT('Ctrl Pts',(-4.71371668583241,-40.8954831180953,
-8.16439679231297));
#17110=CARTESIAN_POINT('Ctrl Pts',(-7.07057502873392,-40.7204831180953,
-4.082198396148));
#17111=CARTESIAN_POINT('Ctrl Pts',(-9.42743337163542,-40.5454831180953,
1.69768315121407E-11));
#17112=CARTESIAN_POINT('Ctrl Pts',(-7.07057502871922,-40.3704831180953,
4.08219839617346));
#17113=CARTESIAN_POINT('Ctrl Pts',(-4.71371668580301,-40.1954831180953,
8.16439679232994));
#17114=CARTESIAN_POINT('Ctrl Pts',(1.47018674401621E-11,-40.0204831180953,
8.16439679232146));
#17115=CARTESIAN_POINT('Ctrl Pts',(4.71371668583241,-39.8454831180953,8.16439679231297));
#17116=CARTESIAN_POINT('Ctrl Pts',(7.07057502873392,-39.6704831180953,4.082198396148));
#17117=CARTESIAN_POINT('Ctrl Pts',(9.42743337163542,-39.4954831180953,-1.69756769845304E-11));
#17118=CARTESIAN_POINT('Ctrl Pts',(7.07057502871922,-39.3204831180953,-4.08219839617346));
#17119=CARTESIAN_POINT('Ctrl Pts',(4.71371668580301,-39.1454831180953,-8.16439679232994));
#17120=CARTESIAN_POINT('Ctrl Pts',(-1.4702867290402E-11,-38.9704831180953,
-8.16439679232146));
#17121=CARTESIAN_POINT('Ctrl Pts',(-4.71371668583241,-38.7954831180953,
-8.16439679231297));
#17122=CARTESIAN_POINT('Ctrl Pts',(-7.07057502873392,-38.6204831180953,
-4.082198396148));
#17123=CARTESIAN_POINT('Ctrl Pts',(-9.42743337163542,-38.4454831180953,
1.69768315121407E-11));
#17124=CARTESIAN_POINT('Ctrl Pts',(-7.07057502871922,-38.2704831180953,
4.08219839617346));
#17125=CARTESIAN_POINT('Ctrl Pts',(-4.71371668580301,-38.0954831180953,
8.16439679232994));
#17126=CARTESIAN_POINT('Ctrl Pts',(1.47018674401621E-11,-37.9204831180953,
8.16439679232146));
#17127=CARTESIAN_POINT('Ctrl Pts',(4.71371668583241,-37.7454831180953,8.16439679231297));
#17128=CARTESIAN_POINT('Ctrl Pts',(7.07057502873392,-37.5704831180953,4.082198396148));
#17129=CARTESIAN_POINT('Ctrl Pts',(9.42743337163542,-37.3954831180953,-1.69756769845304E-11));
#17130=CARTESIAN_POINT('Ctrl Pts',(7.07057502871922,-37.2204831180953,-4.08219839617346));
#17131=CARTESIAN_POINT('Ctrl Pts',(4.71371668580301,-37.0454831180953,-8.16439679232994));
#17132=CARTESIAN_POINT('Ctrl Pts',(-1.4702867290402E-11,-36.8704831180953,
-8.16439679232146));
#17133=CARTESIAN_POINT('Ctrl Pts',(-4.71371668583241,-36.6954831180953,
-8.16439679231297));
#17134=CARTESIAN_POINT('Ctrl Pts',(-7.07057502873392,-36.5204831180953,
-4.082198396148));
#17135=CARTESIAN_POINT('Ctrl Pts',(-9.42743337163542,-36.3454831180953,
1.69768315121407E-11));
#17136=CARTESIAN_POINT('Ctrl Pts',(-7.07057502871922,-36.1704831180953,
4.08219839617346));
#17137=CARTESIAN_POINT('Ctrl Pts',(-4.71371668580301,-35.9954831180953,
8.16439679232994));
#17138=CARTESIAN_POINT('Ctrl Pts',(1.47018674401621E-11,-35.8204831180953,
8.16439679232146));
#17139=CARTESIAN_POINT('Ctrl Pts',(4.71371668583241,-35.6454831180953,8.16439679231297));
#17140=CARTESIAN_POINT('Ctrl Pts',(7.07057502873392,-35.4704831180953,4.082198396148));
#17141=CARTESIAN_POINT('Ctrl Pts',(9.42743337163542,-35.2954831180953,-1.69756769845304E-11));
#17142=CARTESIAN_POINT('Ctrl Pts',(7.07057502871922,-35.1204831180953,-4.08219839617346));
#17143=CARTESIAN_POINT('Ctrl Pts',(4.71371668580301,-34.9454831180953,-8.16439679232994));
#17144=CARTESIAN_POINT('Ctrl Pts',(-1.4702867290402E-11,-34.7704831180953,
-8.16439679232146));
#17145=CARTESIAN_POINT('Ctrl Pts',(-4.71371668583241,-34.5954831180953,
-8.16439679231297));
#17146=CARTESIAN_POINT('Ctrl Pts',(-7.07057502873392,-34.4204831180953,
-4.082198396148));
#17147=CARTESIAN_POINT('Ctrl Pts',(-9.42743337163542,-34.2454831180953,
1.69768315121407E-11));
#17148=CARTESIAN_POINT('Ctrl Pts',(-7.07057502871922,-34.0704831180953,
4.08219839617346));
#17149=CARTESIAN_POINT('Ctrl Pts',(-4.71371668580301,-33.8954831180953,
8.16439679232994));
#17150=CARTESIAN_POINT('Ctrl Pts',(1.47018674401621E-11,-33.7204831180953,
8.16439679232146));
#17151=CARTESIAN_POINT('Ctrl Pts',(4.71371668583241,-33.5454831180953,8.16439679231297));
#17152=CARTESIAN_POINT('Ctrl Pts',(7.07057502873392,-33.3704831180953,4.082198396148));
#17153=CARTESIAN_POINT('Ctrl Pts',(9.42743337163542,-33.1954831180953,-1.69756769845304E-11));
#17154=CARTESIAN_POINT('Ctrl Pts',(7.07057502871922,-33.0204831180953,-4.08219839617346));
#17155=CARTESIAN_POINT('Ctrl Pts',(4.71371668580301,-32.8454831180953,-8.16439679232994));
#17156=CARTESIAN_POINT('Ctrl Pts',(-1.4702867290402E-11,-32.6704831180953,
-8.16439679232146));
#17157=CARTESIAN_POINT('Ctrl Pts',(-4.71371668583241,-32.4954831180953,
-8.16439679231297));
#17158=CARTESIAN_POINT('Ctrl Pts',(-7.07057502873392,-32.3204831180953,
-4.082198396148));
#17159=CARTESIAN_POINT('Ctrl Pts',(-9.42743337163542,-32.1454831180953,
1.69768315121407E-11));
#17160=CARTESIAN_POINT('Ctrl Pts',(-7.07057502871922,-31.9704831180953,
4.08219839617346));
#17161=CARTESIAN_POINT('Ctrl Pts',(-4.71371668580301,-31.7954831180953,
8.16439679232994));
#17162=CARTESIAN_POINT('Ctrl Pts',(1.47018674401621E-11,-31.6204831180953,
8.16439679232146));
#17163=CARTESIAN_POINT('Ctrl Pts',(4.71371668583241,-31.4454831180953,8.16439679231297));
#17164=CARTESIAN_POINT('Ctrl Pts',(7.07057502873392,-31.2704831180953,4.082198396148));
#17165=CARTESIAN_POINT('Ctrl Pts',(9.42743337163542,-31.0954831180953,-1.69756769845304E-11));
#17166=CARTESIAN_POINT('Ctrl Pts',(7.07057502871922,-30.9204831180953,-4.08219839617346));
#17167=CARTESIAN_POINT('Ctrl Pts',(4.71371668580301,-30.7454831180953,-8.16439679232994));
#17168=CARTESIAN_POINT('Ctrl Pts',(-1.4702867290402E-11,-30.5704831180953,
-8.16439679232146));
#17169=CARTESIAN_POINT('Ctrl Pts',(-4.71371668583241,-30.3954831180953,
-8.16439679231297));
#17170=CARTESIAN_POINT('Ctrl Pts',(-7.07057502873392,-30.2204831180953,
-4.082198396148));
#17171=CARTESIAN_POINT('Ctrl Pts',(-9.42743337163542,-30.0454831180953,
1.69768315121407E-11));
#17172=CARTESIAN_POINT('Ctrl Pts',(-7.07057502871922,-29.8704831180953,
4.08219839617346));
#17173=CARTESIAN_POINT('Ctrl Pts',(-4.71371668580301,-29.6954831180953,
8.16439679232994));
#17174=CARTESIAN_POINT('Ctrl Pts',(1.47018674401621E-11,-29.5204831180953,
8.16439679232146));
#17175=CARTESIAN_POINT('Ctrl Pts',(4.71371668583241,-29.3454831180953,8.16439679231297));
#17176=CARTESIAN_POINT('Ctrl Pts',(7.07057502873392,-29.1704831180953,4.082198396148));
#17177=CARTESIAN_POINT('Ctrl Pts',(9.42743337163542,-28.9954831180954,-1.69756769845304E-11));
#17178=CARTESIAN_POINT('Ctrl Pts',(7.07057502871922,-28.8204831180953,-4.08219839617346));
#17179=CARTESIAN_POINT('Ctrl Pts',(4.71371668580301,-28.6454831180953,-8.16439679232994));
#17180=CARTESIAN_POINT('Ctrl Pts',(-1.4702867290402E-11,-28.4704831180953,
-8.16439679232146));
#17181=CARTESIAN_POINT('Ctrl Pts',(-4.71371668583241,-28.2954831180953,
-8.16439679231297));
#17182=CARTESIAN_POINT('Ctrl Pts',(-7.07057502873392,-28.1204831180953,
-4.082198396148));
#17183=CARTESIAN_POINT('Ctrl Pts',(-9.42743337163542,-27.9454831180954,
1.69768315121407E-11));
#17184=CARTESIAN_POINT('Ctrl Pts',(-7.07057502871922,-27.7704831180953,
4.08219839617346));
#17185=CARTESIAN_POINT('Ctrl Pts',(-4.71371668580301,-27.5954831180953,
8.16439679232994));
#17186=CARTESIAN_POINT('Ctrl Pts',(1.47018674401621E-11,-27.4204831180953,
8.16439679232146));
#17187=CARTESIAN_POINT('Ctrl Pts',(4.71371668583241,-27.2454831180954,8.16439679231297));
#17188=CARTESIAN_POINT('Ctrl Pts',(7.07057502873392,-27.0704831180953,4.082198396148));
#17189=CARTESIAN_POINT('Ctrl Pts',(9.42743337163542,-26.8954831180954,-1.69756769845304E-11));
#17190=CARTESIAN_POINT('Ctrl Pts',(7.07057502871922,-26.7204831180953,-4.08219839617346));
#17191=CARTESIAN_POINT('Ctrl Pts',(4.71371668580301,-26.5454831180953,-8.16439679232994));
#17192=CARTESIAN_POINT('Ctrl Pts',(-1.4702867290402E-11,-26.3704831180953,
-8.16439679232146));
#17193=CARTESIAN_POINT('Ctrl Pts',(-4.71371668583241,-26.1954831180954,
-8.16439679231297));
#17194=CARTESIAN_POINT('Ctrl Pts',(-7.07057502873392,-26.0204831180953,
-4.082198396148));
#17195=CARTESIAN_POINT('Ctrl Pts',(-9.42743337163542,-25.8454831180953,
1.69768315121407E-11));
#17196=CARTESIAN_POINT('Ctrl Pts',(-7.07057502871922,-25.6704831180953,
4.08219839617346));
#17197=CARTESIAN_POINT('Ctrl Pts',(-4.71371668580301,-25.4954831180954,
8.16439679232994));
#17198=CARTESIAN_POINT('Ctrl Pts',(1.47018674401621E-11,-25.3204831180953,
8.16439679232146));
#17199=CARTESIAN_POINT('Ctrl Pts',(4.71371668583241,-25.1454831180954,8.16439679231297));
#17200=CARTESIAN_POINT('Ctrl Pts',(7.07057502873392,-24.9704831180954,4.082198396148));
#17201=CARTESIAN_POINT('Ctrl Pts',(9.42743337163542,-24.7954831180953,-1.69756769845304E-11));
#17202=CARTESIAN_POINT('Ctrl Pts',(7.07057502871922,-24.6204831180954,-4.08219839617346));
#17203=CARTESIAN_POINT('Ctrl Pts',(4.71371668580301,-24.4454831180954,-8.16439679232994));
#17204=CARTESIAN_POINT('Ctrl Pts',(-1.4702867290402E-11,-24.2704831180953,
-8.16439679232146));
#17205=CARTESIAN_POINT('Ctrl Pts',(-4.71371668583241,-24.0954831180954,
-8.16439679231297));
#17206=CARTESIAN_POINT('Ctrl Pts',(-7.07057502873392,-23.9204831180953,
-4.082198396148));
#17207=CARTESIAN_POINT('Ctrl Pts',(-9.42743337163542,-23.7454831180954,
1.69768315121407E-11));
#17208=CARTESIAN_POINT('Ctrl Pts',(-7.07057502871922,-23.5704831180954,
4.08219839617346));
#17209=CARTESIAN_POINT('Ctrl Pts',(-4.71371668580301,-23.3954831180954,
8.16439679232994));
#17210=CARTESIAN_POINT('Ctrl Pts',(1.47018674401621E-11,-23.2204831180953,
8.16439679232146));
#17211=CARTESIAN_POINT('Ctrl Pts',(4.71371668583241,-23.0454831180954,8.16439679231297));
#17212=CARTESIAN_POINT('Ctrl Pts',(7.07057502873392,-22.8704831180954,4.082198396148));
#17213=CARTESIAN_POINT('Ctrl Pts',(9.42743337163542,-22.6954831180954,-1.69756769845304E-11));
#17214=CARTESIAN_POINT('Ctrl Pts',(7.07057502871922,-22.5204831180954,-4.08219839617346));
#17215=CARTESIAN_POINT('Ctrl Pts',(4.71371668580301,-22.3454831180954,-8.16439679232994));
#17216=CARTESIAN_POINT('Ctrl Pts',(-1.4702867290402E-11,-22.1704831180954,
-8.16439679232146));
#17217=CARTESIAN_POINT('Ctrl Pts',(-4.71371668583241,-21.9954831180954,
-8.16439679231297));
#17218=CARTESIAN_POINT('Ctrl Pts',(-7.07057502873392,-21.8204831180954,
-4.082198396148));
#17219=CARTESIAN_POINT('Ctrl Pts',(-9.42743337163542,-21.6454831180954,
1.69768315121407E-11));
#17220=CARTESIAN_POINT('Ctrl Pts',(-7.07057502871922,-21.4704831180953,
4.08219839617346));
#17221=CARTESIAN_POINT('Ctrl Pts',(-4.71371668580301,-21.2954831180954,
8.16439679232994));
#17222=CARTESIAN_POINT('Ctrl Pts',(1.47018674401621E-11,-21.1204831180954,
8.16439679232146));
#17223=CARTESIAN_POINT('Ctrl Pts',(4.71371668583241,-20.9454831180954,8.16439679231297));
#17224=CARTESIAN_POINT('Ctrl Pts',(7.07057502873392,-20.7704831180954,4.082198396148));
#17225=CARTESIAN_POINT('Ctrl Pts',(9.42743337163542,-20.5954831180954,-1.69756769845304E-11));
#17226=CARTESIAN_POINT('Ctrl Pts',(7.07057502871922,-20.4204831180954,-4.08219839617346));
#17227=CARTESIAN_POINT('Ctrl Pts',(4.71371668580301,-20.2454831180954,-8.16439679232994));
#17228=CARTESIAN_POINT('Ctrl Pts',(-1.4702867290402E-11,-20.0704831180954,
-8.16439679232146));
#17229=CARTESIAN_POINT('Ctrl Pts',(-4.71371668583241,-19.8954831180954,
-8.16439679231297));
#17230=CARTESIAN_POINT('Ctrl Pts',(-7.07057502873392,-19.7204831180954,
-4.082198396148));
#17231=CARTESIAN_POINT('Ctrl Pts',(-9.42743337163542,-19.5454831180954,
1.69768315121407E-11));
#17232=CARTESIAN_POINT('Ctrl Pts',(-7.07057502871922,-19.3704831180954,
4.08219839617346));
#17233=CARTESIAN_POINT('Ctrl Pts',(-4.71371668580301,-19.1954831180954,
8.16439679232994));
#17234=CARTESIAN_POINT('Ctrl Pts',(1.47018674401621E-11,-19.0204831180954,
8.16439679232146));
#17235=CARTESIAN_POINT('Ctrl Pts',(4.71371668583241,-18.8454831180954,8.16439679231297));
#17236=CARTESIAN_POINT('Ctrl Pts',(7.07057502873392,-18.6704831180954,4.082198396148));
#17237=CARTESIAN_POINT('Ctrl Pts',(9.42743337163542,-18.4954831180954,-1.69756769845304E-11));
#17238=CARTESIAN_POINT('Ctrl Pts',(7.07057502871922,-18.3204831180954,-4.08219839617346));
#17239=CARTESIAN_POINT('Ctrl Pts',(4.71371668580301,-18.1454831180954,-8.16439679232994));
#17240=CARTESIAN_POINT('Ctrl Pts',(-1.4702867290402E-11,-17.9704831180954,
-8.16439679232146));
#17241=CARTESIAN_POINT('Ctrl Pts',(-4.71371668583241,-17.7954831180954,
-8.16439679231297));
#17242=CARTESIAN_POINT('Ctrl Pts',(-7.07057502873392,-17.6204831180954,
-4.082198396148));
#17243=CARTESIAN_POINT('Ctrl Pts',(-9.42743337163542,-17.4454831180954,
1.69768315121407E-11));
#17244=CARTESIAN_POINT('Ctrl Pts',(-7.07057502871922,-17.2704831180954,
4.08219839617346));
#17245=CARTESIAN_POINT('Ctrl Pts',(-4.71371668580301,-17.0954831180954,
8.16439679232994));
#17246=CARTESIAN_POINT('Ctrl Pts',(1.47018674401621E-11,-16.9204831180954,
8.16439679232146));
#17247=CARTESIAN_POINT('Ctrl Pts',(4.71371668583241,-16.7454831180954,8.16439679231297));
#17248=CARTESIAN_POINT('Ctrl Pts',(7.07057502873392,-16.5704831180954,4.082198396148));
#17249=CARTESIAN_POINT('Ctrl Pts',(9.42743337163542,-16.3954831180954,-1.69756769845304E-11));
#17250=CARTESIAN_POINT('Ctrl Pts',(7.07057502871922,-16.2204831180954,-4.08219839617346));
#17251=CARTESIAN_POINT('Ctrl Pts',(4.71371668580301,-16.0454831180954,-8.16439679232994));
#17252=CARTESIAN_POINT('Ctrl Pts',(-1.4702867290402E-11,-15.8704831180954,
-8.16439679232146));
#17253=CARTESIAN_POINT('Ctrl Pts',(-4.71371668583241,-15.6954831180954,
-8.16439679231297));
#17254=CARTESIAN_POINT('Ctrl Pts',(-7.07057502873392,-15.5204831180954,
-4.082198396148));
#17255=CARTESIAN_POINT('Ctrl Pts',(-9.42743337163542,-15.3454831180954,
1.69768315121407E-11));
#17256=CARTESIAN_POINT('Ctrl Pts',(-7.07057502871922,-15.1704831180954,
4.08219839617346));
#17257=CARTESIAN_POINT('Ctrl Pts',(-4.71371668580301,-14.9954831180954,
8.16439679232994));
#17258=CARTESIAN_POINT('Ctrl Pts',(1.47018674401621E-11,-14.8204831180954,
8.16439679232146));
#17259=CARTESIAN_POINT('Ctrl Pts',(4.71371668583241,-14.6454831180954,8.16439679231297));
#17260=CARTESIAN_POINT('Ctrl Pts',(7.07057502873392,-14.4704831180954,4.082198396148));
#17261=CARTESIAN_POINT('Ctrl Pts',(9.42743337163542,-14.2954831180954,-1.69756769845304E-11));
#17262=CARTESIAN_POINT('Ctrl Pts',(7.07057502871922,-14.1204831180954,-4.08219839617346));
#17263=CARTESIAN_POINT('Ctrl Pts',(4.71371668580301,-13.9454831180954,-8.16439679232994));
#17264=CARTESIAN_POINT('Ctrl Pts',(-1.4702867290402E-11,-13.7704831180954,
-8.16439679232146));
#17265=CARTESIAN_POINT('Ctrl Pts',(-4.71371668583241,-13.5954831180954,
-8.16439679231297));
#17266=CARTESIAN_POINT('Ctrl Pts',(-7.07057502873392,-13.4204831180954,
-4.082198396148));
#17267=CARTESIAN_POINT('Ctrl Pts',(-9.42743337163542,-13.2454831180954,
1.69768315121407E-11));
#17268=CARTESIAN_POINT('Ctrl Pts',(-7.07057502871922,-13.0704831180954,
4.08219839617346));
#17269=CARTESIAN_POINT('Ctrl Pts',(-4.71371668580301,-12.8954831180954,
8.16439679232994));
#17270=CARTESIAN_POINT('Ctrl Pts',(1.47018674401621E-11,-12.7204831180954,
8.16439679232146));
#17271=CARTESIAN_POINT('Ctrl Pts',(4.71371668583241,-12.5454831180954,8.16439679231297));
#17272=CARTESIAN_POINT('Ctrl Pts',(7.07057502873392,-12.3704831180954,4.082198396148));
#17273=CARTESIAN_POINT('Ctrl Pts',(9.42743337163542,-12.1954831180954,-1.69756769845304E-11));
#17274=CARTESIAN_POINT('Ctrl Pts',(7.07057502871922,-12.0204831180954,-4.08219839617346));
#17275=CARTESIAN_POINT('Ctrl Pts',(4.71371668580301,-11.8454831180954,-8.16439679232994));
#17276=CARTESIAN_POINT('Ctrl Pts',(-1.4702867290402E-11,-11.6704831180954,
-8.16439679232146));
#17277=CARTESIAN_POINT('Ctrl Pts',(-4.71371668583241,-11.4954831180954,
-8.16439679231297));
#17278=CARTESIAN_POINT('Ctrl Pts',(-7.07057502873392,-11.3204831180954,
-4.082198396148));
#17279=CARTESIAN_POINT('Ctrl Pts',(-9.42743337163542,-11.1454831180954,
1.69768315121407E-11));
#17280=CARTESIAN_POINT('Ctrl Pts',(-7.07057502871922,-10.9704831180954,
4.08219839617346));
#17281=CARTESIAN_POINT('Ctrl Pts',(-4.71371668580301,-10.7954831180954,
8.16439679232994));
#17282=CARTESIAN_POINT('Ctrl Pts',(1.47018674401621E-11,-10.6204831180954,
8.16439679232146));
#17283=CARTESIAN_POINT('Ctrl Pts',(4.71371668583241,-10.4454831180954,8.16439679231297));
#17284=CARTESIAN_POINT('Ctrl Pts',(7.07057502873392,-10.2704831180954,4.082198396148));
#17285=CARTESIAN_POINT('Ctrl Pts',(9.42743337163542,-10.0954831180954,-1.69756769845304E-11));
#17286=CARTESIAN_POINT('Ctrl Pts',(7.07057502871922,-9.92048311809537,-4.08219839617346));
#17287=CARTESIAN_POINT('Ctrl Pts',(4.71371668580301,-9.74548311809539,-8.16439679232994));
#17288=CARTESIAN_POINT('Ctrl Pts',(-1.4702867290402E-11,-9.57048311809539,
-8.16439679232146));
#17289=CARTESIAN_POINT('Ctrl Pts',(-4.71371668583241,-9.39548311809538,
-8.16439679231297));
#17290=CARTESIAN_POINT('Ctrl Pts',(-7.07057502873392,-9.22048311809539,
-4.082198396148));
#17291=CARTESIAN_POINT('Ctrl Pts',(-9.42743337163542,-9.04548311809539,
1.69768315121407E-11));
#17292=CARTESIAN_POINT('Ctrl Pts',(-7.07057502871922,-8.87048311809537,
4.08219839617346));
#17293=CARTESIAN_POINT('Ctrl Pts',(-4.71371668580301,-8.6954831180954,8.16439679232994));
#17294=CARTESIAN_POINT('Ctrl Pts',(1.47018674401621E-11,-8.52048311809539,
8.16439679232146));
#17295=CARTESIAN_POINT('Ctrl Pts',(4.71371668583241,-8.34548311809539,8.16439679231297));
#17296=CARTESIAN_POINT('Ctrl Pts',(7.07057502873392,-8.1704831180954,4.082198396148));
#17297=CARTESIAN_POINT('Ctrl Pts',(9.42743337163542,-7.9954831180954,-1.69756769845304E-11));
#17298=CARTESIAN_POINT('Ctrl Pts',(7.07057502871922,-7.82048311809538,-4.08219839617346));
#17299=CARTESIAN_POINT('Ctrl Pts',(4.71371668580301,-7.64548311809541,-8.16439679232994));
#17300=CARTESIAN_POINT('Ctrl Pts',(-1.4702867290402E-11,-7.47048311809539,
-8.16439679232146));
#17301=CARTESIAN_POINT('Ctrl Pts',(-4.71371668583241,-7.29548311809539,
-8.16439679231297));
#17302=CARTESIAN_POINT('Ctrl Pts',(-7.07057502873392,-7.12048311809538,
-4.082198396148));
#17303=CARTESIAN_POINT('Ctrl Pts',(-9.42743337163542,-6.94548311809541,
1.69768315121407E-11));
#17304=CARTESIAN_POINT('Ctrl Pts',(-7.07057502871922,-6.77048311809538,
4.08219839617346));
#17305=CARTESIAN_POINT('Ctrl Pts',(-4.71371668580301,-6.59548311809539,
8.16439679232994));
#17306=CARTESIAN_POINT('Ctrl Pts',(1.47018674401621E-11,-6.4204831180954,
8.16439679232146));
#17307=CARTESIAN_POINT('Ctrl Pts',(4.71371668583241,-6.24548311809539,8.16439679231297));
#17308=CARTESIAN_POINT('Ctrl Pts',(7.07057502873392,-6.07048311809538,4.082198396148));
#17309=CARTESIAN_POINT('Ctrl Pts',(9.42743337163542,-5.89548311809541,-1.69756769845304E-11));
#17310=CARTESIAN_POINT('Ctrl Pts',(7.07057502871922,-5.72048311809538,-4.08219839617346));
#17311=CARTESIAN_POINT('Ctrl Pts',(4.71371668580301,-5.54548311809539,-8.16439679232994));
#17312=CARTESIAN_POINT('Ctrl Pts',(-1.4702867290402E-11,-5.3704831180954,
-8.16439679232146));
#17313=CARTESIAN_POINT('Ctrl Pts',(-4.71371668583241,-5.19548311809541,
-8.16439679231297));
#17314=CARTESIAN_POINT('Ctrl Pts',(-7.07057502873392,-5.02048311809538,
-4.082198396148));
#17315=CARTESIAN_POINT('Ctrl Pts',(-9.42743337163542,-4.84548311809541,
1.69768315121407E-11));
#17316=CARTESIAN_POINT('Ctrl Pts',(-7.07057502871922,-4.6704831180954,4.08219839617346));
#17317=CARTESIAN_POINT('Ctrl Pts',(-4.71371668580301,-4.49548311809539,
8.16439679232994));
#17318=CARTESIAN_POINT('Ctrl Pts',(1.47018674401621E-11,-4.3204831180954,
8.16439679232146));
#17319=CARTESIAN_POINT('Ctrl Pts',(4.71371668583241,-4.14548311809541,8.16439679231297));
#17320=CARTESIAN_POINT('Ctrl Pts',(7.07057502873392,-3.97048311809539,4.082198396148));
#17321=CARTESIAN_POINT('Ctrl Pts',(9.42743337163542,-3.79548311809541,-1.69756769845304E-11));
#17322=CARTESIAN_POINT('Ctrl Pts',(7.07057502871922,-3.6204831180954,-4.08219839617346));
#17323=CARTESIAN_POINT('Ctrl Pts',(4.71371668580301,-3.44548311809539,-8.16439679232994));
#17324=CARTESIAN_POINT('Ctrl Pts',(-1.4702867290402E-11,-3.27048311809541,
-8.16439679232146));
#17325=CARTESIAN_POINT('Ctrl Pts',(-4.71371668583241,-3.09548311809541,
-8.16439679231297));
#17326=CARTESIAN_POINT('Ctrl Pts',(-7.07057502873392,-2.92048311809539,
-4.082198396148));
#17327=CARTESIAN_POINT('Ctrl Pts',(-9.42743337163542,-2.74548311809539,
1.69768315121407E-11));
#17328=CARTESIAN_POINT('Ctrl Pts',(-7.07057502871922,-2.5704831180954,4.08219839617346));
#17329=CARTESIAN_POINT('Ctrl Pts',(-4.71371668580301,-2.3954831180954,8.16439679232994));
#17330=CARTESIAN_POINT('Ctrl Pts',(1.47018674401621E-11,-2.22048311809539,
8.16439679232146));
#17331=CARTESIAN_POINT('Ctrl Pts',(4.71371668583241,-2.04548311809541,8.16439679231297));
#17332=CARTESIAN_POINT('Ctrl Pts',(7.07057502873392,-1.87048311809539,4.082198396148));
#17333=CARTESIAN_POINT('Ctrl Pts',(9.42743337163542,-1.69548311809539,-1.69756769845304E-11));
#17334=CARTESIAN_POINT('Ctrl Pts',(7.07057502871922,-1.52048311809541,-4.08219839617346));
#17335=CARTESIAN_POINT('Ctrl Pts',(4.71371668580301,-1.34548311809541,-8.16439679232994));
#17336=CARTESIAN_POINT('Ctrl Pts',(-1.4702867290402E-11,-1.17048311809539,
-8.16439679232146));
#17337=CARTESIAN_POINT('Ctrl Pts',(-4.71371668583241,-0.995483118095416,
-8.16439679231297));
#17338=CARTESIAN_POINT('Ctrl Pts',(-7.07057502873392,-0.820483118095406,
-4.082198396148));
#17339=CARTESIAN_POINT('Ctrl Pts',(-9.42743337163542,-0.645483118095396,
1.69768315121407E-11));
#17340=CARTESIAN_POINT('Ctrl Pts',(-7.07057502871922,-0.47048311809541,
4.08219839617346));
#17341=CARTESIAN_POINT('Ctrl Pts',(-4.71371668580301,-0.295483118095414,
8.16439679232994));
#17342=CARTESIAN_POINT('Ctrl Pts',(1.47018674401621E-11,-0.120483118095393,
8.16439679232146));
#17343=CARTESIAN_POINT('Ctrl Pts',(4.71371668583241,0.054516881904581,8.16439679231297));
#17344=CARTESIAN_POINT('Ctrl Pts',(7.07057502873392,0.229516881904591,4.082198396148));
#17345=CARTESIAN_POINT('Ctrl Pts',(9.42743337163542,0.404516881904601,-1.69756769845304E-11));
#17346=CARTESIAN_POINT('Ctrl Pts',(7.07057502871922,0.579516881904587,-4.08219839617346));
#17347=CARTESIAN_POINT('Ctrl Pts',(4.71371668580301,0.754516881904583,-8.16439679232994));
#17348=CARTESIAN_POINT('Ctrl Pts',(-1.4702867290402E-11,0.929516881904604,
-8.16439679232146));
#17349=CARTESIAN_POINT('Ctrl Pts',(-4.71371668583241,1.10451688190458,-8.16439679231297));
#17350=CARTESIAN_POINT('Ctrl Pts',(-7.07057502873392,1.27951688190459,-4.082198396148));
#17351=CARTESIAN_POINT('Ctrl Pts',(-9.42743337163542,1.4545168819046,1.69768315121407E-11));
#17352=CARTESIAN_POINT('Ctrl Pts',(-7.07057502871922,1.62951688190461,4.08219839617346));
#17353=CARTESIAN_POINT('Ctrl Pts',(-4.71371668580301,1.80451688190458,8.16439679232994));
#17354=CARTESIAN_POINT('Ctrl Pts',(1.47018674401621E-11,1.9795168819046,
8.16439679232146));
#17355=CARTESIAN_POINT('Ctrl Pts',(4.71371668583241,2.1545168819046,8.16439679231297));
#17356=CARTESIAN_POINT('Ctrl Pts',(7.07057502873392,2.32951688190458,4.082198396148));
#17357=CARTESIAN_POINT('Ctrl Pts',(9.42743337163542,2.50451688190458,-1.69756769845304E-11));
#17358=CARTESIAN_POINT('Ctrl Pts',(7.07057502871922,2.6795168819046,-4.08219839617346));
#17359=CARTESIAN_POINT('Ctrl Pts',(4.71371668580301,2.85451688190458,-8.16439679232994));
#17360=CARTESIAN_POINT('Ctrl Pts',(-1.4702867290402E-11,3.02951688190459,
-8.16439679232146));
#17361=CARTESIAN_POINT('Ctrl Pts',(-4.71371668583241,3.2045168819046,-8.16439679231297));
#17362=CARTESIAN_POINT('Ctrl Pts',(-7.07057502873392,3.37951688190458,-4.082198396148));
#17363=CARTESIAN_POINT('Ctrl Pts',(-9.42743337163542,3.55451688190458,1.69768315121407E-11));
#17364=CARTESIAN_POINT('Ctrl Pts',(-7.07057502871922,3.7295168819046,4.08219839617346));
#17365=CARTESIAN_POINT('Ctrl Pts',(-4.71371668580301,3.90451688190458,8.16439679232994));
#17366=CARTESIAN_POINT('Ctrl Pts',(1.47018674401621E-11,4.07951688190458,
8.16439679232146));
#17367=CARTESIAN_POINT('Ctrl Pts',(4.71371668583241,4.2545168819046,8.16439679231297));
#17368=CARTESIAN_POINT('Ctrl Pts',(7.07057502873392,4.42951688190458,4.082198396148));
#17369=CARTESIAN_POINT('Ctrl Pts',(9.42743337163542,4.60451688190458,-1.69756769845304E-11));
#17370=CARTESIAN_POINT('Ctrl Pts',(7.07057502871922,4.7795168819046,-4.08219839617346));
#17371=CARTESIAN_POINT('Ctrl Pts',(4.71371668580301,4.95451688190457,-8.16439679232994));
#17372=CARTESIAN_POINT('Ctrl Pts',(-1.4702867290402E-11,5.12951688190458,
-8.16439679232146));
#17373=CARTESIAN_POINT('Ctrl Pts',(-4.71371668583241,5.30451688190459,-8.16439679231297));
#17374=CARTESIAN_POINT('Ctrl Pts',(-7.07057502873392,5.47951688190458,-4.082198396148));
#17375=CARTESIAN_POINT('Ctrl Pts',(-9.42743337163542,5.65451688190458,1.69768315121407E-11));
#17376=CARTESIAN_POINT('Ctrl Pts',(-7.07057502871922,5.82951688190459,4.08219839617346));
#17377=CARTESIAN_POINT('Ctrl Pts',(-4.71371668580301,6.00451688190457,8.16439679232994));
#17378=CARTESIAN_POINT('Ctrl Pts',(1.47018674401621E-11,6.17951688190458,
8.16439679232146));
#17379=CARTESIAN_POINT('Ctrl Pts',(4.71371668583241,6.35451688190459,8.16439679231297));
#17380=CARTESIAN_POINT('Ctrl Pts',(7.07057502873392,6.52951688190459,4.082198396148));
#17381=CARTESIAN_POINT('Ctrl Pts',(9.42743337163542,6.70451688190457,-1.69756769845304E-11));
#17382=CARTESIAN_POINT('Ctrl Pts',(7.07057502871922,6.87951688190458,-4.08219839617346));
#17383=CARTESIAN_POINT('Ctrl Pts',(4.71371668580301,7.05451688190459,-8.16439679232994));
#17384=CARTESIAN_POINT('Ctrl Pts',(-1.4702867290402E-11,7.22951688190457,
-8.16439679232146));
#17385=CARTESIAN_POINT('Ctrl Pts',(-4.71371668583241,7.40451688190458,-8.16439679231297));
#17386=CARTESIAN_POINT('Ctrl Pts',(-7.07057502873392,7.57951688190459,-4.082198396148));
#17387=CARTESIAN_POINT('Ctrl Pts',(-9.42743337163542,7.75451688190457,1.69768315121407E-11));
#17388=CARTESIAN_POINT('Ctrl Pts',(-7.07057502871922,7.92951688190458,4.08219839617346));
#17389=CARTESIAN_POINT('Ctrl Pts',(-4.71371668580301,8.10451688190458,8.16439679232994));
#17390=CARTESIAN_POINT('Ctrl Pts',(1.47018674401621E-11,8.27951688190457,
8.16439679232146));
#17391=CARTESIAN_POINT('Ctrl Pts',(4.71371668583241,8.45451688190457,8.16439679231297));
#17392=CARTESIAN_POINT('Ctrl Pts',(7.07057502873392,8.62951688190459,4.082198396148));
#17393=CARTESIAN_POINT('Ctrl Pts',(9.42743337163542,8.80451688190457,-1.69756769845304E-11));
#17394=CARTESIAN_POINT('Ctrl Pts',(7.07057502871922,8.97951688190457,-4.08219839617346));
#17395=CARTESIAN_POINT('Ctrl Pts',(4.71371668580301,9.15451688190458,-8.16439679232994));
#17396=CARTESIAN_POINT('Ctrl Pts',(-1.4702867290402E-11,9.32951688190457,
-8.16439679232146));
#17397=CARTESIAN_POINT('Ctrl Pts',(-4.71371668583241,9.50451688190457,-8.16439679231297));
#17398=CARTESIAN_POINT('Ctrl Pts',(-7.07057502873392,9.67951688190458,-4.082198396148));
#17399=CARTESIAN_POINT('Ctrl Pts',(-9.42743337163542,9.85451688190457,1.69768315121407E-11));
#17400=CARTESIAN_POINT('Ctrl Pts',(-7.07057502871922,10.0295168819046,4.08219839617346));
#17401=CARTESIAN_POINT('Ctrl Pts',(-4.71371668580301,10.2045168819046,8.16439679232994));
#17402=CARTESIAN_POINT('Ctrl Pts',(1.47018674401621E-11,10.3795168819046,
8.16439679232146));
#17403=CARTESIAN_POINT('Ctrl Pts',(4.71371668583241,10.5545168819046,8.16439679231297));
#17404=CARTESIAN_POINT('Ctrl Pts',(7.07057502873392,10.7295168819046,4.082198396148));
#17405=CARTESIAN_POINT('Ctrl Pts',(9.42743337163542,10.9045168819046,-1.69756769845304E-11));
#17406=CARTESIAN_POINT('Ctrl Pts',(7.07057502871922,11.0795168819046,-4.08219839617346));
#17407=CARTESIAN_POINT('Ctrl Pts',(4.71371668580301,11.2545168819046,-8.16439679232994));
#17408=CARTESIAN_POINT('Ctrl Pts',(-1.4702867290402E-11,11.4295168819046,
-8.16439679232146));
#17409=CARTESIAN_POINT('Ctrl Pts',(-4.71371668583241,11.6045168819046,-8.16439679231297));
#17410=CARTESIAN_POINT('Ctrl Pts',(-7.07057502873392,11.7795168819046,-4.082198396148));
#17411=CARTESIAN_POINT('Ctrl Pts',(-9.42743337163542,11.9545168819046,1.69768315121407E-11));
#17412=CARTESIAN_POINT('Ctrl Pts',(-7.07057502871922,12.1295168819046,4.08219839617346));
#17413=CARTESIAN_POINT('Ctrl Pts',(-4.71371668580301,12.3045168819046,8.16439679232994));
#17414=CARTESIAN_POINT('Ctrl Pts',(1.47018674401621E-11,12.4795168819046,
8.16439679232146));
#17415=CARTESIAN_POINT('Ctrl Pts',(4.71371668583241,12.6545168819046,8.16439679231297));
#17416=CARTESIAN_POINT('Ctrl Pts',(7.07057502873392,12.8295168819046,4.082198396148));
#17417=CARTESIAN_POINT('Ctrl Pts',(9.42743337163542,13.0045168819046,-1.69756769845304E-11));
#17418=CARTESIAN_POINT('Ctrl Pts',(7.07057502871922,13.1795168819046,-4.08219839617346));
#17419=CARTESIAN_POINT('Ctrl Pts',(4.71371668580301,13.3545168819046,-8.16439679232994));
#17420=CARTESIAN_POINT('Ctrl Pts',(-1.4702867290402E-11,13.5295168819046,
-8.16439679232146));
#17421=CARTESIAN_POINT('Ctrl Pts',(-4.71371668583241,13.7045168819046,-8.16439679231297));
#17422=CARTESIAN_POINT('Ctrl Pts',(-7.07057502873392,13.8795168819046,-4.082198396148));
#17423=CARTESIAN_POINT('Ctrl Pts',(-9.42743337163542,14.0545168819046,1.69768315121407E-11));
#17424=CARTESIAN_POINT('Ctrl Pts',(-7.07057502871922,14.2295168819046,4.08219839617346));
#17425=CARTESIAN_POINT('Ctrl Pts',(-4.71371668580301,14.4045168819046,8.16439679232994));
#17426=CARTESIAN_POINT('Ctrl Pts',(1.47018674401621E-11,14.5795168819046,
8.16439679232146));
#17427=CARTESIAN_POINT('Ctrl Pts',(4.71371668583241,14.7545168819045,8.16439679231297));
#17428=CARTESIAN_POINT('Ctrl Pts',(7.07057502873392,14.9295168819046,4.082198396148));
#17429=CARTESIAN_POINT('Ctrl Pts',(9.42743337163542,15.1045168819046,-1.69756769845304E-11));
#17430=CARTESIAN_POINT('Ctrl Pts',(7.07057502871922,15.2795168819046,-4.08219839617346));
#17431=CARTESIAN_POINT('Ctrl Pts',(4.71371668580301,15.4545168819046,-8.16439679232994));
#17432=CARTESIAN_POINT('Ctrl Pts',(-1.4702867290402E-11,15.6295168819046,
-8.16439679232146));
#17433=CARTESIAN_POINT('Ctrl Pts',(-4.71371668583241,15.8045168819046,-8.16439679231297));
#17434=CARTESIAN_POINT('Ctrl Pts',(-7.07057502873392,15.9795168819046,-4.082198396148));
#17435=CARTESIAN_POINT('Ctrl Pts',(-9.42743337163542,16.1545168819046,1.69768315121407E-11));
#17436=CARTESIAN_POINT('Ctrl Pts',(-7.07057502871922,16.3295168819046,4.08219839617346));
#17437=CARTESIAN_POINT('Ctrl Pts',(-4.71371668580301,16.5045168819046,8.16439679232994));
#17438=CARTESIAN_POINT('Ctrl Pts',(1.47018674401621E-11,16.6795168819046,
8.16439679232146));
#17439=CARTESIAN_POINT('Ctrl Pts',(4.71371668583241,16.8545168819046,8.16439679231297));
#17440=CARTESIAN_POINT('Ctrl Pts',(7.07057502873392,17.0295168819046,4.082198396148));
#17441=CARTESIAN_POINT('Ctrl Pts',(9.42743337163542,17.2045168819045,-1.69756769845304E-11));
#17442=CARTESIAN_POINT('Ctrl Pts',(7.07057502871922,17.3795168819046,-4.08219839617346));
#17443=CARTESIAN_POINT('Ctrl Pts',(4.71371668580301,17.5545168819045,-8.16439679232994));
#17444=CARTESIAN_POINT('Ctrl Pts',(-1.4702867290402E-11,17.7295168819046,
-8.16439679232146));
#17445=CARTESIAN_POINT('Ctrl Pts',(-4.71371668583241,17.9045168819046,-8.16439679231297));
#17446=CARTESIAN_POINT('Ctrl Pts',(-7.07057502873392,18.0795168819045,-4.082198396148));
#17447=CARTESIAN_POINT('Ctrl Pts',(-9.42743337163542,18.2545168819045,1.69768315121407E-11));
#17448=CARTESIAN_POINT('Ctrl Pts',(-7.07057502871922,18.4295168819046,4.08219839617346));
#17449=CARTESIAN_POINT('Ctrl Pts',(-4.71371668580301,18.6045168819045,8.16439679232994));
#17450=CARTESIAN_POINT('Ctrl Pts',(1.47018674401621E-11,18.7795168819046,
8.16439679232146));
#17451=CARTESIAN_POINT('Ctrl Pts',(4.71371668583241,18.9545168819045,8.16439679231297));
#17452=CARTESIAN_POINT('Ctrl Pts',(7.07057502873392,19.1295168819045,4.082198396148));
#17453=CARTESIAN_POINT('Ctrl Pts',(9.42743337163542,19.3045168819045,-1.69756769845304E-11));
#17454=CARTESIAN_POINT('Ctrl Pts',(7.07057502871922,19.4795168819046,-4.08219839617346));
#17455=CARTESIAN_POINT('Ctrl Pts',(4.71371668580301,19.6545168819046,-8.16439679232994));
#17456=CARTESIAN_POINT('Ctrl Pts',(-1.4702867290402E-11,19.8295168819045,
-8.16439679232146));
#17457=CARTESIAN_POINT('Ctrl Pts',(-4.71371668583241,20.0045168819045,-8.16439679231297));
#17458=CARTESIAN_POINT('Ctrl Pts',(-7.07057502873392,20.1795168819046,-4.082198396148));
#17459=CARTESIAN_POINT('Ctrl Pts',(-9.42743337163542,20.3545168819045,1.69768315121407E-11));
#17460=CARTESIAN_POINT('Ctrl Pts',(-7.07057502871922,20.5295168819046,4.08219839617346));
#17461=CARTESIAN_POINT('Ctrl Pts',(-4.71371668580301,20.7045168819046,8.16439679232994));
#17462=CARTESIAN_POINT('Ctrl Pts',(1.47018674401621E-11,20.8795168819045,
8.16439679232146));
#17463=CARTESIAN_POINT('Ctrl Pts',(4.71371668583241,21.0545168819045,8.16439679231297));
#17464=CARTESIAN_POINT('Ctrl Pts',(7.07057502873392,21.2295168819046,4.082198396148));
#17465=CARTESIAN_POINT('Ctrl Pts',(9.42743337163542,21.4045168819045,-1.69756769845304E-11));
#17466=CARTESIAN_POINT('Ctrl Pts',(7.07057502871922,21.5795168819045,-4.08219839617346));
#17467=CARTESIAN_POINT('Ctrl Pts',(4.71371668580301,21.7545168819045,-8.16439679232994));
#17468=CARTESIAN_POINT('Ctrl Pts',(-1.4702867290402E-11,21.9295168819045,
-8.16439679232146));
#17469=CARTESIAN_POINT('Ctrl Pts',(-4.71371668583241,22.1045168819045,-8.16439679231297));
#17470=CARTESIAN_POINT('Ctrl Pts',(-7.07057502873392,22.2795168819046,-4.082198396148));
#17471=CARTESIAN_POINT('Ctrl Pts',(-9.42743337163542,22.4545168819045,1.69768315121407E-11));
#17472=CARTESIAN_POINT('Ctrl Pts',(-7.07057502871922,22.6295168819045,4.08219839617346));
#17473=CARTESIAN_POINT('Ctrl Pts',(-4.71371668580301,22.8045168819045,8.16439679232994));
#17474=CARTESIAN_POINT('Ctrl Pts',(1.47018674401621E-11,22.9795168819045,
8.16439679232146));
#17475=CARTESIAN_POINT('Ctrl Pts',(4.71371668583241,23.1545168819045,8.16439679231297));
#17476=CARTESIAN_POINT('Ctrl Pts',(7.07057502873392,23.3295168819046,4.082198396148));
#17477=CARTESIAN_POINT('Ctrl Pts',(9.42743337163542,23.5045168819045,-1.69756769845304E-11));
#17478=CARTESIAN_POINT('Ctrl Pts',(7.07057502871922,23.6795168819045,-4.08219839617346));
#17479=CARTESIAN_POINT('Ctrl Pts',(4.71371668580301,23.8545168819045,-8.16439679232994));
#17480=CARTESIAN_POINT('Ctrl Pts',(-1.4702867290402E-11,24.0295168819045,
-8.16439679232146));
#17481=CARTESIAN_POINT('Ctrl Pts',(-4.71371668583241,24.2045168819045,-8.16439679231297));
#17482=CARTESIAN_POINT('Ctrl Pts',(-7.07057502873392,24.3795168819046,-4.082198396148));
#17483=CARTESIAN_POINT('Ctrl Pts',(-9.42743337163542,24.5545168819046,1.69768315121407E-11));
#17484=CARTESIAN_POINT('Ctrl Pts',(-7.07057502871922,24.7295168819045,4.08219839617346));
#17485=CARTESIAN_POINT('Ctrl Pts',(-4.71371668580301,24.9045168819045,8.16439679232994));
#17486=CARTESIAN_POINT('Ctrl Pts',(1.47018674401621E-11,25.0795168819046,
8.16439679232146));
#17487=CARTESIAN_POINT('Ctrl Pts',(4.71371668583241,25.2545168819045,8.16439679231297));
#17488=CARTESIAN_POINT('Ctrl Pts',(7.07057502873392,25.4295168819045,4.082198396148));
#17489=CARTESIAN_POINT('Ctrl Pts',(9.42743337163542,25.6045168819045,-1.69756769845304E-11));
#17490=CARTESIAN_POINT('Ctrl Pts',(7.07057502871922,25.7795168819045,-4.08219839617346));
#17491=CARTESIAN_POINT('Ctrl Pts',(4.71371668580301,25.9545168819045,-8.16439679232994));
#17492=CARTESIAN_POINT('Ctrl Pts',(-1.4702867290402E-11,26.1295168819045,
-8.16439679232146));
#17493=CARTESIAN_POINT('Ctrl Pts',(-1.4702867290402E-11,-143.703019107145,
-8.16439679232146));
#17494=CARTESIAN_POINT('Ctrl Pts',(-4.71371668583241,-143.528019107145,
-8.16439679231297));
#17495=CARTESIAN_POINT('Ctrl Pts',(-7.07057502873392,-143.353019107145,
-4.082198396148));
#17496=CARTESIAN_POINT('Ctrl Pts',(-9.42743337163542,-143.178019107145,
1.69768315121407E-11));
#17497=CARTESIAN_POINT('Ctrl Pts',(-7.07057502871922,-143.003019107145,
4.08219839617346));
#17498=CARTESIAN_POINT('Ctrl Pts',(-4.71371668580301,-142.828019107145,
8.16439679232994));
#17499=CARTESIAN_POINT('Ctrl Pts',(1.47018674401621E-11,-142.653019107145,
8.16439679232146));
#17500=CARTESIAN_POINT('Ctrl Pts',(4.71371668583241,-142.478019107145,8.16439679231297));
#17501=CARTESIAN_POINT('Ctrl Pts',(7.07057502873392,-142.303019107145,4.082198396148));
#17502=CARTESIAN_POINT('Ctrl Pts',(9.42743337163542,-142.128019107145,-1.69756769845304E-11));
#17503=CARTESIAN_POINT('Ctrl Pts',(7.07057502871922,-141.953019107145,-4.08219839617346));
#17504=CARTESIAN_POINT('Ctrl Pts',(4.71371668580301,-141.778019107145,-8.16439679232994));
#17505=CARTESIAN_POINT('Ctrl Pts',(-1.4702867290402E-11,-141.603019107145,
-8.16439679232146));
#17506=CARTESIAN_POINT('Ctrl Pts',(-4.71371668583241,-141.428019107145,
-8.16439679231297));
#17507=CARTESIAN_POINT('Ctrl Pts',(-7.07057502873392,-141.253019107145,
-4.082198396148));
#17508=CARTESIAN_POINT('Ctrl Pts',(-9.42743337163542,-141.078019107145,
1.69768315121407E-11));
#17509=CARTESIAN_POINT('Ctrl Pts',(-7.07057502871922,-140.903019107145,
4.08219839617346));
#17510=CARTESIAN_POINT('Ctrl Pts',(-4.71371668580301,-140.728019107145,
8.16439679232994));
#17511=CARTESIAN_POINT('Ctrl Pts',(1.47018674401621E-11,-140.553019107145,
8.16439679232146));
#17512=CARTESIAN_POINT('Ctrl Pts',(4.71371668583241,-140.378019107145,8.16439679231297));
#17513=CARTESIAN_POINT('Ctrl Pts',(7.07057502873392,-140.203019107145,4.082198396148));
#17514=CARTESIAN_POINT('Ctrl Pts',(9.42743337163542,-140.028019107145,-1.69756769845304E-11));
#17515=CARTESIAN_POINT('Ctrl Pts',(7.07057502871922,-139.853019107145,-4.08219839617346));
#17516=CARTESIAN_POINT('Ctrl Pts',(4.71371668580301,-139.678019107145,-8.16439679232994));
#17517=CARTESIAN_POINT('Ctrl Pts',(-1.4702867290402E-11,-139.503019107145,
-8.16439679232146));
#17518=CARTESIAN_POINT('Ctrl Pts',(-4.71371668583241,-139.328019107145,
-8.16439679231297));
#17519=CARTESIAN_POINT('Ctrl Pts',(-7.07057502873392,-139.153019107145,
-4.082198396148));
#17520=CARTESIAN_POINT('Ctrl Pts',(-9.42743337163542,-138.978019107145,
1.69768315121407E-11));
#17521=CARTESIAN_POINT('Ctrl Pts',(-7.07057502871922,-138.803019107145,
4.08219839617346));
#17522=CARTESIAN_POINT('Ctrl Pts',(-4.71371668580301,-138.628019107145,
8.16439679232994));
#17523=CARTESIAN_POINT('Ctrl Pts',(1.47018674401621E-11,-138.453019107145,
8.16439679232146));
#17524=CARTESIAN_POINT('Ctrl Pts',(4.71371668583241,-138.278019107145,8.16439679231297));
#17525=CARTESIAN_POINT('Ctrl Pts',(7.07057502873392,-138.103019107145,4.082198396148));
#17526=CARTESIAN_POINT('Ctrl Pts',(9.42743337163542,-137.928019107145,-1.69756769845304E-11));
#17527=CARTESIAN_POINT('Ctrl Pts',(7.07057502871922,-137.753019107145,-4.08219839617346));
#17528=CARTESIAN_POINT('Ctrl Pts',(4.71371668580301,-137.578019107145,-8.16439679232994));
#17529=CARTESIAN_POINT('Ctrl Pts',(-1.4702867290402E-11,-137.403019107145,
-8.16439679232146));
#17530=CARTESIAN_POINT('Ctrl Pts',(-4.71371668583241,-137.228019107145,
-8.16439679231297));
#17531=CARTESIAN_POINT('Ctrl Pts',(-7.07057502873392,-137.053019107145,
-4.082198396148));
#17532=CARTESIAN_POINT('Ctrl Pts',(-9.42743337163542,-136.878019107145,
1.69768315121407E-11));
#17533=CARTESIAN_POINT('Ctrl Pts',(-7.07057502871922,-136.703019107145,
4.08219839617346));
#17534=CARTESIAN_POINT('Ctrl Pts',(-4.71371668580301,-136.528019107145,
8.16439679232994));
#17535=CARTESIAN_POINT('Ctrl Pts',(1.47018674401621E-11,-136.353019107145,
8.16439679232146));
#17536=CARTESIAN_POINT('Ctrl Pts',(4.71371668583241,-136.178019107145,8.16439679231297));
#17537=CARTESIAN_POINT('Ctrl Pts',(7.07057502873392,-136.003019107145,4.082198396148));
#17538=CARTESIAN_POINT('Ctrl Pts',(9.42743337163542,-135.828019107145,-1.69756769845304E-11));
#17539=CARTESIAN_POINT('Ctrl Pts',(7.07057502871922,-135.653019107145,-4.08219839617346));
#17540=CARTESIAN_POINT('Ctrl Pts',(4.71371668580301,-135.478019107145,-8.16439679232994));
#17541=CARTESIAN_POINT('Ctrl Pts',(-1.4702867290402E-11,-135.303019107145,
-8.16439679232146));
#17542=CARTESIAN_POINT('Ctrl Pts',(-4.71371668583241,-135.128019107145,
-8.16439679231297));
#17543=CARTESIAN_POINT('Ctrl Pts',(-7.07057502873392,-134.953019107145,
-4.082198396148));
#17544=CARTESIAN_POINT('Ctrl Pts',(-9.42743337163542,-134.778019107145,
1.69768315121407E-11));
#17545=CARTESIAN_POINT('Ctrl Pts',(-7.07057502871922,-134.603019107145,
4.08219839617346));
#17546=CARTESIAN_POINT('Ctrl Pts',(-4.71371668580301,-134.428019107145,
8.16439679232994));
#17547=CARTESIAN_POINT('Ctrl Pts',(1.47018674401621E-11,-134.253019107145,
8.16439679232146));
#17548=CARTESIAN_POINT('Ctrl Pts',(4.71371668583241,-134.078019107145,8.16439679231297));
#17549=CARTESIAN_POINT('Ctrl Pts',(7.07057502873392,-133.903019107145,4.082198396148));
#17550=CARTESIAN_POINT('Ctrl Pts',(9.42743337163542,-133.728019107145,-1.69756769845304E-11));
#17551=CARTESIAN_POINT('Ctrl Pts',(7.07057502871922,-133.553019107145,-4.08219839617346));
#17552=CARTESIAN_POINT('Ctrl Pts',(4.71371668580301,-133.378019107145,-8.16439679232994));
#17553=CARTESIAN_POINT('Ctrl Pts',(-1.4702867290402E-11,-133.203019107145,
-8.16439679232146));
#17554=CARTESIAN_POINT('Ctrl Pts',(-4.71371668583241,-133.028019107145,
-8.16439679231297));
#17555=CARTESIAN_POINT('Ctrl Pts',(-7.07057502873392,-132.853019107145,
-4.082198396148));
#17556=CARTESIAN_POINT('Ctrl Pts',(-9.42743337163542,-132.678019107145,
1.69768315121407E-11));
#17557=CARTESIAN_POINT('Ctrl Pts',(-7.07057502871922,-132.503019107145,
4.08219839617346));
#17558=CARTESIAN_POINT('Ctrl Pts',(-4.71371668580301,-132.328019107145,
8.16439679232994));
#17559=CARTESIAN_POINT('Ctrl Pts',(1.47018674401621E-11,-132.153019107145,
8.16439679232146));
#17560=CARTESIAN_POINT('Ctrl Pts',(4.71371668583241,-131.978019107145,8.16439679231297));
#17561=CARTESIAN_POINT('Ctrl Pts',(7.07057502873392,-131.803019107145,4.082198396148));
#17562=CARTESIAN_POINT('Ctrl Pts',(9.42743337163542,-131.628019107145,-1.69756769845304E-11));
#17563=CARTESIAN_POINT('Ctrl Pts',(7.07057502871922,-131.453019107145,-4.08219839617346));
#17564=CARTESIAN_POINT('Ctrl Pts',(4.71371668580301,-131.278019107145,-8.16439679232994));
#17565=CARTESIAN_POINT('Ctrl Pts',(-1.4702867290402E-11,-131.103019107145,
-8.16439679232146));
#17566=CARTESIAN_POINT('Ctrl Pts',(-4.71371668583241,-130.928019107145,
-8.16439679231297));
#17567=CARTESIAN_POINT('Ctrl Pts',(-7.07057502873392,-130.753019107145,
-4.082198396148));
#17568=CARTESIAN_POINT('Ctrl Pts',(-9.42743337163542,-130.578019107145,
1.69768315121407E-11));
#17569=CARTESIAN_POINT('Ctrl Pts',(-7.07057502871922,-130.403019107145,
4.08219839617346));
#17570=CARTESIAN_POINT('Ctrl Pts',(-4.71371668580301,-130.228019107145,
8.16439679232994));
#17571=CARTESIAN_POINT('Ctrl Pts',(1.47018674401621E-11,-130.053019107145,
8.16439679232146));
#17572=CARTESIAN_POINT('Ctrl Pts',(4.71371668583241,-129.878019107145,8.16439679231297));
#17573=CARTESIAN_POINT('Ctrl Pts',(7.07057502873392,-129.703019107145,4.082198396148));
#17574=CARTESIAN_POINT('Ctrl Pts',(9.42743337163542,-129.528019107145,-1.69756769845304E-11));
#17575=CARTESIAN_POINT('Ctrl Pts',(7.07057502871922,-129.353019107145,-4.08219839617346));
#17576=CARTESIAN_POINT('Ctrl Pts',(4.71371668580301,-129.178019107145,-8.16439679232994));
#17577=CARTESIAN_POINT('Ctrl Pts',(-1.4702867290402E-11,-129.003019107145,
-8.16439679232146));
#17578=CARTESIAN_POINT('Ctrl Pts',(-4.71371668583241,-128.828019107145,
-8.16439679231297));
#17579=CARTESIAN_POINT('Ctrl Pts',(-7.07057502873392,-128.653019107145,
-4.082198396148));
#17580=CARTESIAN_POINT('Ctrl Pts',(-9.42743337163542,-128.478019107145,
1.69768315121407E-11));
#17581=CARTESIAN_POINT('Ctrl Pts',(-7.07057502871922,-128.303019107145,
4.08219839617346));
#17582=CARTESIAN_POINT('Ctrl Pts',(-4.71371668580301,-128.128019107145,
8.16439679232994));
#17583=CARTESIAN_POINT('Ctrl Pts',(1.47018674401621E-11,-127.953019107145,
8.16439679232146));
#17584=CARTESIAN_POINT('Ctrl Pts',(4.71371668583241,-127.778019107145,8.16439679231297));
#17585=CARTESIAN_POINT('Ctrl Pts',(7.07057502873392,-127.603019107145,4.082198396148));
#17586=CARTESIAN_POINT('Ctrl Pts',(9.42743337163542,-127.428019107145,-1.69756769845304E-11));
#17587=CARTESIAN_POINT('Ctrl Pts',(7.07057502871922,-127.253019107145,-4.08219839617346));
#17588=CARTESIAN_POINT('Ctrl Pts',(4.71371668580301,-127.078019107145,-8.16439679232994));
#17589=CARTESIAN_POINT('Ctrl Pts',(-1.4702867290402E-11,-126.903019107145,
-8.16439679232146));
#17590=CARTESIAN_POINT('Ctrl Pts',(-4.71371668583241,-126.728019107145,
-8.16439679231297));
#17591=CARTESIAN_POINT('Ctrl Pts',(-7.07057502873392,-126.553019107145,
-4.082198396148));
#17592=CARTESIAN_POINT('Ctrl Pts',(-9.42743337163542,-126.378019107145,
1.69768315121407E-11));
#17593=CARTESIAN_POINT('Ctrl Pts',(-7.07057502871922,-126.203019107145,
4.08219839617346));
#17594=CARTESIAN_POINT('Ctrl Pts',(-4.71371668580301,-126.028019107145,
8.16439679232994));
#17595=CARTESIAN_POINT('Ctrl Pts',(1.47018674401621E-11,-125.853019107145,
8.16439679232146));
#17596=CARTESIAN_POINT('Ctrl Pts',(4.71371668583241,-125.678019107145,8.16439679231297));
#17597=CARTESIAN_POINT('Ctrl Pts',(7.07057502873392,-125.503019107145,4.082198396148));
#17598=CARTESIAN_POINT('Ctrl Pts',(9.42743337163542,-125.328019107145,-1.69756769845304E-11));
#17599=CARTESIAN_POINT('Ctrl Pts',(7.07057502871922,-125.153019107145,-4.08219839617346));
#17600=CARTESIAN_POINT('Ctrl Pts',(4.71371668580301,-124.978019107145,-8.16439679232994));
#17601=CARTESIAN_POINT('Ctrl Pts',(-1.4702867290402E-11,-124.803019107145,
-8.16439679232146));
#17602=CARTESIAN_POINT('Ctrl Pts',(-4.71371668583241,-124.628019107145,
-8.16439679231297));
#17603=CARTESIAN_POINT('Ctrl Pts',(-7.07057502873392,-124.453019107145,
-4.082198396148));
#17604=CARTESIAN_POINT('Ctrl Pts',(-9.42743337163542,-124.278019107145,
1.69768315121407E-11));
#17605=CARTESIAN_POINT('Ctrl Pts',(-7.07057502871922,-124.103019107145,
4.08219839617346));
#17606=CARTESIAN_POINT('Ctrl Pts',(-4.71371668580301,-123.928019107145,
8.16439679232994));
#17607=CARTESIAN_POINT('Ctrl Pts',(1.47018674401621E-11,-123.753019107145,
8.16439679232146));
#17608=CARTESIAN_POINT('Ctrl Pts',(4.71371668583241,-123.578019107145,8.16439679231297));
#17609=CARTESIAN_POINT('Ctrl Pts',(7.07057502873392,-123.403019107145,4.082198396148));
#17610=CARTESIAN_POINT('Ctrl Pts',(9.42743337163542,-123.228019107145,-1.69756769845304E-11));
#17611=CARTESIAN_POINT('Ctrl Pts',(7.07057502871922,-123.053019107145,-4.08219839617346));
#17612=CARTESIAN_POINT('Ctrl Pts',(4.71371668580301,-122.878019107145,-8.16439679232994));
#17613=CARTESIAN_POINT('Ctrl Pts',(-1.4702867290402E-11,-122.703019107145,
-8.16439679232146));
#17614=CARTESIAN_POINT('Ctrl Pts',(-4.71371668583241,-122.528019107145,
-8.16439679231297));
#17615=CARTESIAN_POINT('Ctrl Pts',(-7.07057502873392,-122.353019107145,
-4.082198396148));
#17616=CARTESIAN_POINT('Ctrl Pts',(-9.42743337163542,-122.178019107145,
1.69768315121407E-11));
#17617=CARTESIAN_POINT('Ctrl Pts',(-7.07057502871922,-122.003019107145,
4.08219839617346));
#17618=CARTESIAN_POINT('Ctrl Pts',(-4.71371668580301,-121.828019107145,
8.16439679232994));
#17619=CARTESIAN_POINT('Ctrl Pts',(1.47018674401621E-11,-121.653019107145,
8.16439679232146));
#17620=CARTESIAN_POINT('Ctrl Pts',(4.71371668583241,-121.478019107145,8.16439679231297));
#17621=CARTESIAN_POINT('Ctrl Pts',(7.07057502873392,-121.303019107145,4.082198396148));
#17622=CARTESIAN_POINT('Ctrl Pts',(9.42743337163542,-121.128019107145,-1.69756769845304E-11));
#17623=CARTESIAN_POINT('Ctrl Pts',(7.07057502871922,-120.953019107145,-4.08219839617346));
#17624=CARTESIAN_POINT('Ctrl Pts',(4.71371668580301,-120.778019107145,-8.16439679232994));
#17625=CARTESIAN_POINT('Ctrl Pts',(-1.4702867290402E-11,-120.603019107145,
-8.16439679232146));
#17626=CARTESIAN_POINT('Ctrl Pts',(-4.71371668583241,-120.428019107145,
-8.16439679231297));
#17627=CARTESIAN_POINT('Ctrl Pts',(-7.07057502873392,-120.253019107145,
-4.082198396148));
#17628=CARTESIAN_POINT('Ctrl Pts',(-9.42743337163542,-120.078019107145,
1.69768315121407E-11));
#17629=CARTESIAN_POINT('Ctrl Pts',(-7.07057502871922,-119.903019107145,
4.08219839617346));
#17630=CARTESIAN_POINT('Ctrl Pts',(-4.71371668580301,-119.728019107145,
8.16439679232994));
#17631=CARTESIAN_POINT('Ctrl Pts',(1.47018674401621E-11,-119.553019107145,
8.16439679232146));
#17632=CARTESIAN_POINT('Ctrl Pts',(4.71371668583241,-119.378019107145,8.16439679231297));
#17633=CARTESIAN_POINT('Ctrl Pts',(7.07057502873392,-119.203019107145,4.082198396148));
#17634=CARTESIAN_POINT('Ctrl Pts',(9.42743337163542,-119.028019107145,-1.69756769845304E-11));
#17635=CARTESIAN_POINT('Ctrl Pts',(7.07057502871922,-118.853019107145,-4.08219839617346));
#17636=CARTESIAN_POINT('Ctrl Pts',(4.71371668580301,-118.678019107145,-8.16439679232994));
#17637=CARTESIAN_POINT('Ctrl Pts',(-1.4702867290402E-11,-118.503019107145,
-8.16439679232146));
#17638=CARTESIAN_POINT('Ctrl Pts',(-4.71371668583241,-118.328019107145,
-8.16439679231297));
#17639=CARTESIAN_POINT('Ctrl Pts',(-7.07057502873392,-118.153019107145,
-4.082198396148));
#17640=CARTESIAN_POINT('Ctrl Pts',(-9.42743337163542,-117.978019107145,
1.69768315121407E-11));
#17641=CARTESIAN_POINT('Ctrl Pts',(-7.07057502871922,-117.803019107145,
4.08219839617346));
#17642=CARTESIAN_POINT('Ctrl Pts',(-4.71371668580301,-117.628019107145,
8.16439679232994));
#17643=CARTESIAN_POINT('Ctrl Pts',(1.47018674401621E-11,-117.453019107145,
8.16439679232146));
#17644=CARTESIAN_POINT('Ctrl Pts',(4.71371668583241,-117.278019107145,8.16439679231297));
#17645=CARTESIAN_POINT('Ctrl Pts',(7.07057502873392,-117.103019107145,4.082198396148));
#17646=CARTESIAN_POINT('Ctrl Pts',(9.42743337163542,-116.928019107145,-1.69756769845304E-11));
#17647=CARTESIAN_POINT('Ctrl Pts',(7.07057502871922,-116.753019107145,-4.08219839617346));
#17648=CARTESIAN_POINT('Ctrl Pts',(4.71371668580301,-116.578019107145,-8.16439679232994));
#17649=CARTESIAN_POINT('Ctrl Pts',(-1.4702867290402E-11,-116.403019107145,
-8.16439679232146));
#17650=CARTESIAN_POINT('Ctrl Pts',(-4.71371668583241,-116.228019107145,
-8.16439679231297));
#17651=CARTESIAN_POINT('Ctrl Pts',(-7.07057502873392,-116.053019107145,
-4.082198396148));
#17652=CARTESIAN_POINT('Ctrl Pts',(-9.42743337163542,-115.878019107145,
1.69768315121407E-11));
#17653=CARTESIAN_POINT('Ctrl Pts',(-7.07057502871922,-115.703019107145,
4.08219839617346));
#17654=CARTESIAN_POINT('Ctrl Pts',(-4.71371668580301,-115.528019107145,
8.16439679232994));
#17655=CARTESIAN_POINT('Ctrl Pts',(1.47018674401621E-11,-115.353019107145,
8.16439679232146));
#17656=CARTESIAN_POINT('Ctrl Pts',(4.71371668583241,-115.178019107145,8.16439679231297));
#17657=CARTESIAN_POINT('Ctrl Pts',(7.07057502873392,-115.003019107145,4.082198396148));
#17658=CARTESIAN_POINT('Ctrl Pts',(9.42743337163542,-114.828019107145,-1.69756769845304E-11));
#17659=CARTESIAN_POINT('Ctrl Pts',(7.07057502871922,-114.653019107145,-4.08219839617346));
#17660=CARTESIAN_POINT('Ctrl Pts',(4.71371668580301,-114.478019107145,-8.16439679232994));
#17661=CARTESIAN_POINT('Ctrl Pts',(-1.4702867290402E-11,-114.303019107145,
-8.16439679232146));
#17662=CARTESIAN_POINT('Ctrl Pts',(-4.71371668583241,-114.128019107145,
-8.16439679231297));
#17663=CARTESIAN_POINT('Ctrl Pts',(-7.07057502873392,-113.953019107145,
-4.082198396148));
#17664=CARTESIAN_POINT('Ctrl Pts',(-9.42743337163542,-113.778019107145,
1.69768315121407E-11));
#17665=CARTESIAN_POINT('Ctrl Pts',(-7.07057502871922,-113.603019107145,
4.08219839617346));
#17666=CARTESIAN_POINT('Ctrl Pts',(-4.71371668580301,-113.428019107145,
8.16439679232994));
#17667=CARTESIAN_POINT('Ctrl Pts',(1.47018674401621E-11,-113.253019107145,
8.16439679232146));
#17668=CARTESIAN_POINT('Ctrl Pts',(4.71371668583241,-113.078019107145,8.16439679231297));
#17669=CARTESIAN_POINT('Ctrl Pts',(7.07057502873392,-112.903019107145,4.082198396148));
#17670=CARTESIAN_POINT('Ctrl Pts',(9.42743337163542,-112.728019107145,-1.69756769845304E-11));
#17671=CARTESIAN_POINT('Ctrl Pts',(7.07057502871922,-112.553019107145,-4.08219839617346));
#17672=CARTESIAN_POINT('Ctrl Pts',(4.71371668580301,-112.378019107145,-8.16439679232994));
#17673=CARTESIAN_POINT('Ctrl Pts',(-1.4702867290402E-11,-112.203019107145,
-8.16439679232146));
#17674=CARTESIAN_POINT('Ctrl Pts',(-4.71371668583241,-112.028019107145,
-8.16439679231297));
#17675=CARTESIAN_POINT('Ctrl Pts',(-7.07057502873392,-111.853019107145,
-4.082198396148));
#17676=CARTESIAN_POINT('Ctrl Pts',(-9.42743337163542,-111.678019107145,
1.69768315121407E-11));
#17677=CARTESIAN_POINT('Ctrl Pts',(-7.07057502871922,-111.503019107145,
4.08219839617346));
#17678=CARTESIAN_POINT('Ctrl Pts',(-4.71371668580301,-111.328019107145,
8.16439679232994));
#17679=CARTESIAN_POINT('Ctrl Pts',(1.47018674401621E-11,-111.153019107145,
8.16439679232146));
#17680=CARTESIAN_POINT('Ctrl Pts',(4.71371668583241,-110.978019107145,8.16439679231297));
#17681=CARTESIAN_POINT('Ctrl Pts',(7.07057502873392,-110.803019107145,4.082198396148));
#17682=CARTESIAN_POINT('Ctrl Pts',(9.42743337163542,-110.628019107145,-1.69756769845304E-11));
#17683=CARTESIAN_POINT('Ctrl Pts',(7.07057502871922,-110.453019107145,-4.08219839617346));
#17684=CARTESIAN_POINT('Ctrl Pts',(4.71371668580301,-110.278019107145,-8.16439679232994));
#17685=CARTESIAN_POINT('Ctrl Pts',(-1.4702867290402E-11,-110.103019107145,
-8.16439679232146));
#17686=CARTESIAN_POINT('Ctrl Pts',(-4.71371668583241,-109.928019107145,
-8.16439679231297));
#17687=CARTESIAN_POINT('Ctrl Pts',(-7.07057502873392,-109.753019107145,
-4.082198396148));
#17688=CARTESIAN_POINT('Ctrl Pts',(-9.42743337163542,-109.578019107145,
1.69768315121407E-11));
#17689=CARTESIAN_POINT('Ctrl Pts',(-7.07057502871922,-109.403019107145,
4.08219839617346));
#17690=CARTESIAN_POINT('Ctrl Pts',(-4.71371668580301,-109.228019107145,
8.16439679232994));
#17691=CARTESIAN_POINT('Ctrl Pts',(1.47018674401621E-11,-109.053019107145,
8.16439679232146));
#17692=CARTESIAN_POINT('Ctrl Pts',(4.71371668583241,-108.878019107145,8.16439679231297));
#17693=CARTESIAN_POINT('Ctrl Pts',(7.07057502873392,-108.703019107145,4.082198396148));
#17694=CARTESIAN_POINT('Ctrl Pts',(9.42743337163542,-108.528019107145,-1.69756769845304E-11));
#17695=CARTESIAN_POINT('Ctrl Pts',(7.07057502871922,-108.353019107145,-4.08219839617346));
#17696=CARTESIAN_POINT('Ctrl Pts',(4.71371668580301,-108.178019107145,-8.16439679232994));
#17697=CARTESIAN_POINT('Ctrl Pts',(-1.4702867290402E-11,-108.003019107145,
-8.16439679232146));
#17698=CARTESIAN_POINT('Ctrl Pts',(-4.71371668583241,-107.828019107145,
-8.16439679231297));
#17699=CARTESIAN_POINT('Ctrl Pts',(-7.07057502873392,-107.653019107145,
-4.082198396148));
#17700=CARTESIAN_POINT('Ctrl Pts',(-9.42743337163542,-107.478019107145,
1.69768315121407E-11));
#17701=CARTESIAN_POINT('Ctrl Pts',(-7.07057502871922,-107.303019107145,
4.08219839617346));
#17702=CARTESIAN_POINT('Ctrl Pts',(-4.71371668580301,-107.128019107145,
8.16439679232994));
#17703=CARTESIAN_POINT('Ctrl Pts',(1.47018674401621E-11,-106.953019107145,
8.16439679232146));
#17704=CARTESIAN_POINT('Ctrl Pts',(4.71371668583241,-106.778019107145,8.16439679231297));
#17705=CARTESIAN_POINT('Ctrl Pts',(7.07057502873392,-106.603019107145,4.082198396148));
#17706=CARTESIAN_POINT('Ctrl Pts',(9.42743337163542,-106.428019107145,-1.69756769845304E-11));
#17707=CARTESIAN_POINT('Ctrl Pts',(7.07057502871922,-106.253019107145,-4.08219839617346));
#17708=CARTESIAN_POINT('Ctrl Pts',(4.71371668580301,-106.078019107145,-8.16439679232994));
#17709=CARTESIAN_POINT('Ctrl Pts',(-1.4702867290402E-11,-105.903019107145,
-8.16439679232146));
#17710=CARTESIAN_POINT('Ctrl Pts',(-4.71371668583241,-105.728019107145,
-8.16439679231297));
#17711=CARTESIAN_POINT('Ctrl Pts',(-7.07057502873392,-105.553019107145,
-4.082198396148));
#17712=CARTESIAN_POINT('Ctrl Pts',(-9.42743337163542,-105.378019107145,
1.69768315121407E-11));
#17713=CARTESIAN_POINT('Ctrl Pts',(-7.07057502871922,-105.203019107145,
4.08219839617346));
#17714=CARTESIAN_POINT('Ctrl Pts',(-4.71371668580301,-105.028019107145,
8.16439679232994));
#17715=CARTESIAN_POINT('Ctrl Pts',(1.47018674401621E-11,-104.853019107145,
8.16439679232146));
#17716=CARTESIAN_POINT('Ctrl Pts',(4.71371668583241,-104.678019107145,8.16439679231297));
#17717=CARTESIAN_POINT('Ctrl Pts',(7.07057502873392,-104.503019107145,4.082198396148));
#17718=CARTESIAN_POINT('Ctrl Pts',(9.42743337163542,-104.328019107145,-1.69756769845304E-11));
#17719=CARTESIAN_POINT('Ctrl Pts',(7.07057502871922,-104.153019107145,-4.08219839617346));
#17720=CARTESIAN_POINT('Ctrl Pts',(4.71371668580301,-103.978019107145,-8.16439679232994));
#17721=CARTESIAN_POINT('Ctrl Pts',(-1.4702867290402E-11,-103.803019107145,
-8.16439679232146));
#17722=CARTESIAN_POINT('Ctrl Pts',(-4.71371668583241,-103.628019107145,
-8.16439679231297));
#17723=CARTESIAN_POINT('Ctrl Pts',(-7.07057502873392,-103.453019107145,
-4.082198396148));
#17724=CARTESIAN_POINT('Ctrl Pts',(-9.42743337163542,-103.278019107145,
1.69768315121407E-11));
#17725=CARTESIAN_POINT('Ctrl Pts',(-7.07057502871922,-103.103019107145,
4.08219839617346));
#17726=CARTESIAN_POINT('Ctrl Pts',(-4.71371668580301,-102.928019107145,
8.16439679232994));
#17727=CARTESIAN_POINT('Ctrl Pts',(1.47018674401621E-11,-102.753019107145,
8.16439679232146));
#17728=CARTESIAN_POINT('Ctrl Pts',(4.71371668583241,-102.578019107145,8.16439679231297));
#17729=CARTESIAN_POINT('Ctrl Pts',(7.07057502873392,-102.403019107145,4.082198396148));
#17730=CARTESIAN_POINT('Ctrl Pts',(9.42743337163542,-102.228019107145,-1.69756769845304E-11));
#17731=CARTESIAN_POINT('Ctrl Pts',(7.07057502871922,-102.053019107145,-4.08219839617346));
#17732=CARTESIAN_POINT('Ctrl Pts',(4.71371668580301,-101.878019107145,-8.16439679232994));
#17733=CARTESIAN_POINT('Ctrl Pts',(-1.4702867290402E-11,-101.703019107145,
-8.16439679232146));
#17734=CARTESIAN_POINT('Ctrl Pts',(-4.71371668583241,-101.528019107145,
-8.16439679231297));
#17735=CARTESIAN_POINT('Ctrl Pts',(-7.07057502873392,-101.353019107145,
-4.082198396148));
#17736=CARTESIAN_POINT('Ctrl Pts',(-9.42743337163542,-101.178019107145,
1.69768315121407E-11));
#17737=CARTESIAN_POINT('Ctrl Pts',(-7.07057502871922,-101.003019107145,
4.08219839617346));
#17738=CARTESIAN_POINT('Ctrl Pts',(-4.71371668580301,-100.828019107145,
8.16439679232994));
#17739=CARTESIAN_POINT('Ctrl Pts',(1.47018674401621E-11,-100.653019107145,
8.16439679232146));
#17740=CARTESIAN_POINT('Ctrl Pts',(4.71371668583241,-100.478019107145,8.16439679231297));
#17741=CARTESIAN_POINT('Ctrl Pts',(7.07057502873392,-100.303019107145,4.082198396148));
#17742=CARTESIAN_POINT('Ctrl Pts',(9.42743337163542,-100.128019107145,-1.69756769845304E-11));
#17743=CARTESIAN_POINT('Ctrl Pts',(7.07057502871922,-99.953019107145,-4.08219839617346));
#17744=CARTESIAN_POINT('Ctrl Pts',(4.71371668580301,-99.7780191071449,-8.16439679232994));
#17745=CARTESIAN_POINT('Ctrl Pts',(-1.4702867290402E-11,-99.6030191071449,
-8.16439679232146));
#17746=CARTESIAN_POINT('Ctrl Pts',(-4.71371668583241,-99.4280191071449,
-8.16439679231297));
#17747=CARTESIAN_POINT('Ctrl Pts',(-7.07057502873392,-99.253019107145,-4.082198396148));
#17748=CARTESIAN_POINT('Ctrl Pts',(-9.42743337163542,-99.078019107145,1.69768315121407E-11));
#17749=CARTESIAN_POINT('Ctrl Pts',(-7.07057502871922,-98.903019107145,4.08219839617346));
#17750=CARTESIAN_POINT('Ctrl Pts',(-4.71371668580301,-98.7280191071449,
8.16439679232994));
#17751=CARTESIAN_POINT('Ctrl Pts',(1.47018674401621E-11,-98.5530191071449,
8.16439679232146));
#17752=CARTESIAN_POINT('Ctrl Pts',(4.71371668583241,-98.378019107145,8.16439679231297));
#17753=CARTESIAN_POINT('Ctrl Pts',(7.07057502873392,-98.2030191071449,4.082198396148));
#17754=CARTESIAN_POINT('Ctrl Pts',(9.42743337163542,-98.0280191071449,-1.69756769845304E-11));
#17755=CARTESIAN_POINT('Ctrl Pts',(7.07057502871922,-97.8530191071449,-4.08219839617346));
#17756=CARTESIAN_POINT('Ctrl Pts',(4.71371668580301,-97.6780191071449,-8.16439679232994));
#17757=CARTESIAN_POINT('Ctrl Pts',(-1.4702867290402E-11,-97.503019107145,
-8.16439679232146));
#17758=CARTESIAN_POINT('Ctrl Pts',(-4.71371668583241,-97.328019107145,-8.16439679231297));
#17759=CARTESIAN_POINT('Ctrl Pts',(-7.07057502873392,-97.153019107145,-4.082198396148));
#17760=CARTESIAN_POINT('Ctrl Pts',(-9.42743337163542,-96.978019107145,1.69768315121407E-11));
#17761=CARTESIAN_POINT('Ctrl Pts',(-7.07057502871922,-96.803019107145,4.08219839617346));
#17762=CARTESIAN_POINT('Ctrl Pts',(-4.71371668580301,-96.6280191071449,
8.16439679232994));
#17763=CARTESIAN_POINT('Ctrl Pts',(1.47018674401621E-11,-96.453019107145,
8.16439679232146));
#17764=CARTESIAN_POINT('Ctrl Pts',(4.71371668583241,-96.278019107145,8.16439679231297));
#17765=CARTESIAN_POINT('Ctrl Pts',(7.07057502873392,-96.103019107145,4.082198396148));
#17766=CARTESIAN_POINT('Ctrl Pts',(9.42743337163542,-95.928019107145,-1.69756769845304E-11));
#17767=CARTESIAN_POINT('Ctrl Pts',(7.07057502871922,-95.753019107145,-4.08219839617346));
#17768=CARTESIAN_POINT('Ctrl Pts',(4.71371668580301,-95.5780191071449,-8.16439679232994));
#17769=CARTESIAN_POINT('Ctrl Pts',(-1.4702867290402E-11,-95.403019107145,
-8.16439679232146));
#17770=CARTESIAN_POINT('Ctrl Pts',(-4.71371668583241,-95.228019107145,-8.16439679231297));
#17771=CARTESIAN_POINT('Ctrl Pts',(-7.07057502873392,-95.053019107145,-4.082198396148));
#17772=CARTESIAN_POINT('Ctrl Pts',(-9.42743337163542,-94.8780191071449,
1.69768315121407E-11));
#17773=CARTESIAN_POINT('Ctrl Pts',(-7.07057502871922,-94.703019107145,4.08219839617346));
#17774=CARTESIAN_POINT('Ctrl Pts',(-4.71371668580301,-94.528019107145,8.16439679232994));
#17775=CARTESIAN_POINT('Ctrl Pts',(1.47018674401621E-11,-94.3530191071449,
8.16439679232146));
#17776=CARTESIAN_POINT('Ctrl Pts',(4.71371668583241,-94.178019107145,8.16439679231297));
#17777=CARTESIAN_POINT('Ctrl Pts',(7.07057502873392,-94.003019107145,4.082198396148));
#17778=CARTESIAN_POINT('Ctrl Pts',(9.42743337163542,-93.8280191071449,-1.69756769845304E-11));
#17779=CARTESIAN_POINT('Ctrl Pts',(7.07057502871922,-93.6530191071449,-4.08219839617346));
#17780=CARTESIAN_POINT('Ctrl Pts',(4.71371668580301,-93.4780191071449,-8.16439679232994));
#17781=CARTESIAN_POINT('Ctrl Pts',(-1.4702867290402E-11,-93.3030191071449,
-8.16439679232146));
#17782=CARTESIAN_POINT('Ctrl Pts',(-4.71371668583241,-93.128019107145,-8.16439679231297));
#17783=CARTESIAN_POINT('Ctrl Pts',(-7.07057502873392,-92.953019107145,-4.082198396148));
#17784=CARTESIAN_POINT('Ctrl Pts',(-9.42743337163542,-92.7780191071449,
1.69768315121407E-11));
#17785=CARTESIAN_POINT('Ctrl Pts',(-7.07057502871922,-92.6030191071449,
4.08219839617346));
#17786=CARTESIAN_POINT('Ctrl Pts',(-4.71371668580301,-92.428019107145,8.16439679232994));
#17787=CARTESIAN_POINT('Ctrl Pts',(1.47018674401621E-11,-92.253019107145,
8.16439679232146));
#17788=CARTESIAN_POINT('Ctrl Pts',(4.71371668583241,-92.0780191071449,8.16439679231297));
#17789=CARTESIAN_POINT('Ctrl Pts',(7.07057502873392,-91.903019107145,4.082198396148));
#17790=CARTESIAN_POINT('Ctrl Pts',(9.42743337163542,-91.728019107145,-1.69756769845304E-11));
#17791=CARTESIAN_POINT('Ctrl Pts',(7.07057502871922,-91.553019107145,-4.08219839617346));
#17792=CARTESIAN_POINT('Ctrl Pts',(4.71371668580301,-91.378019107145,-8.16439679232994));
#17793=CARTESIAN_POINT('Ctrl Pts',(-1.4702867290402E-11,-91.203019107145,
-8.16439679232146));
#17794=CARTESIAN_POINT('Ctrl Pts',(-4.71371668583241,-91.028019107145,-8.16439679231297));
#17795=CARTESIAN_POINT('Ctrl Pts',(-7.07057502873392,-90.853019107145,-4.082198396148));
#17796=CARTESIAN_POINT('Ctrl Pts',(-9.42743337163542,-90.678019107145,1.69768315121407E-11));
#17797=CARTESIAN_POINT('Ctrl Pts',(-7.07057502871922,-90.503019107145,4.08219839617346));
#17798=CARTESIAN_POINT('Ctrl Pts',(-4.71371668580301,-90.328019107145,8.16439679232994));
#17799=CARTESIAN_POINT('Ctrl Pts',(1.47018674401621E-11,-90.153019107145,
8.16439679232146));
#17800=CARTESIAN_POINT('Ctrl Pts',(4.71371668583241,-89.978019107145,8.16439679231297));
#17801=CARTESIAN_POINT('Ctrl Pts',(7.07057502873392,-89.803019107145,4.082198396148));
#17802=CARTESIAN_POINT('Ctrl Pts',(9.42743337163542,-89.628019107145,-1.69756769845304E-11));
#17803=CARTESIAN_POINT('Ctrl Pts',(7.07057502871922,-89.4530191071449,-4.08219839617346));
#17804=CARTESIAN_POINT('Ctrl Pts',(4.71371668580301,-89.278019107145,-8.16439679232994));
#17805=CARTESIAN_POINT('Ctrl Pts',(-1.4702867290402E-11,-89.103019107145,
-8.16439679232146));
#17806=CARTESIAN_POINT('Ctrl Pts',(-4.71371668583241,-88.9280191071449,
-8.16439679231297));
#17807=CARTESIAN_POINT('Ctrl Pts',(-7.07057502873392,-88.753019107145,-4.082198396148));
#17808=CARTESIAN_POINT('Ctrl Pts',(-9.42743337163542,-88.578019107145,1.69768315121407E-11));
#17809=CARTESIAN_POINT('Ctrl Pts',(-7.07057502871922,-88.403019107145,4.08219839617346));
#17810=CARTESIAN_POINT('Ctrl Pts',(-4.71371668580301,-88.228019107145,8.16439679232994));
#17811=CARTESIAN_POINT('Ctrl Pts',(1.47018674401621E-11,-88.053019107145,
8.16439679232146));
#17812=CARTESIAN_POINT('Ctrl Pts',(4.71371668583241,-87.878019107145,8.16439679231297));
#17813=CARTESIAN_POINT('Ctrl Pts',(7.07057502873392,-87.703019107145,4.082198396148));
#17814=CARTESIAN_POINT('Ctrl Pts',(9.42743337163542,-87.528019107145,-1.69756769845304E-11));
#17815=CARTESIAN_POINT('Ctrl Pts',(7.07057502871922,-87.353019107145,-4.08219839617346));
#17816=CARTESIAN_POINT('Ctrl Pts',(4.71371668580301,-87.178019107145,-8.16439679232994));
#17817=CARTESIAN_POINT('Ctrl Pts',(-1.4702867290402E-11,-87.003019107145,
-8.16439679232146));
#17818=CARTESIAN_POINT('Ctrl Pts',(-4.71371668583241,-86.828019107145,-8.16439679231297));
#17819=CARTESIAN_POINT('Ctrl Pts',(-7.07057502873392,-86.653019107145,-4.082198396148));
#17820=CARTESIAN_POINT('Ctrl Pts',(-9.42743337163542,-86.478019107145,1.69768315121407E-11));
#17821=CARTESIAN_POINT('Ctrl Pts',(-7.07057502871922,-86.303019107145,4.08219839617346));
#17822=CARTESIAN_POINT('Ctrl Pts',(-4.71371668580301,-86.128019107145,8.16439679232994));
#17823=CARTESIAN_POINT('Ctrl Pts',(1.47018674401621E-11,-85.953019107145,
8.16439679232146));
#17824=CARTESIAN_POINT('Ctrl Pts',(4.71371668583241,-85.778019107145,8.16439679231297));
#17825=CARTESIAN_POINT('Ctrl Pts',(7.07057502873392,-85.603019107145,4.082198396148));
#17826=CARTESIAN_POINT('Ctrl Pts',(9.42743337163542,-85.428019107145,-1.69756769845304E-11));
#17827=CARTESIAN_POINT('Ctrl Pts',(7.07057502871922,-85.253019107145,-4.08219839617346));
#17828=CARTESIAN_POINT('Ctrl Pts',(4.71371668580301,-85.078019107145,-8.16439679232994));
#17829=CARTESIAN_POINT('Ctrl Pts',(-1.4702867290402E-11,-84.903019107145,
-8.16439679232146));
#17830=CARTESIAN_POINT('Ctrl Pts',(-4.71371668583241,-84.728019107145,-8.16439679231297));
#17831=CARTESIAN_POINT('Ctrl Pts',(-7.07057502873392,-84.553019107145,-4.082198396148));
#17832=CARTESIAN_POINT('Ctrl Pts',(-9.42743337163542,-84.378019107145,1.69768315121407E-11));
#17833=CARTESIAN_POINT('Ctrl Pts',(-7.07057502871922,-84.203019107145,4.08219839617346));
#17834=CARTESIAN_POINT('Ctrl Pts',(-4.71371668580301,-84.028019107145,8.16439679232994));
#17835=CARTESIAN_POINT('Ctrl Pts',(1.47018674401621E-11,-83.853019107145,
8.16439679232146));
#17836=CARTESIAN_POINT('Ctrl Pts',(4.71371668583241,-83.678019107145,8.16439679231297));
#17837=CARTESIAN_POINT('Ctrl Pts',(7.07057502873392,-83.503019107145,4.082198396148));
#17838=CARTESIAN_POINT('Ctrl Pts',(9.42743337163542,-83.328019107145,-1.69756769845304E-11));
#17839=CARTESIAN_POINT('Ctrl Pts',(7.07057502871922,-83.153019107145,-4.08219839617346));
#17840=CARTESIAN_POINT('Ctrl Pts',(4.71371668580301,-82.978019107145,-8.16439679232994));
#17841=CARTESIAN_POINT('Ctrl Pts',(-1.4702867290402E-11,-82.803019107145,
-8.16439679232146));
#17842=CARTESIAN_POINT('Ctrl Pts',(-4.71371668583241,-82.628019107145,-8.16439679231297));
#17843=CARTESIAN_POINT('Ctrl Pts',(-7.07057502873392,-82.453019107145,-4.082198396148));
#17844=CARTESIAN_POINT('Ctrl Pts',(-9.42743337163542,-82.278019107145,1.69768315121407E-11));
#17845=CARTESIAN_POINT('Ctrl Pts',(-7.07057502871922,-82.103019107145,4.08219839617346));
#17846=CARTESIAN_POINT('Ctrl Pts',(-4.71371668580301,-81.928019107145,8.16439679232994));
#17847=CARTESIAN_POINT('Ctrl Pts',(1.47018674401621E-11,-81.753019107145,
8.16439679232146));
#17848=CARTESIAN_POINT('Ctrl Pts',(4.71371668583241,-81.578019107145,8.16439679231297));
#17849=CARTESIAN_POINT('Ctrl Pts',(7.07057502873392,-81.403019107145,4.082198396148));
#17850=CARTESIAN_POINT('Ctrl Pts',(9.42743337163542,-81.228019107145,-1.69756769845304E-11));
#17851=CARTESIAN_POINT('Ctrl Pts',(7.07057502871922,-81.053019107145,-4.08219839617346));
#17852=CARTESIAN_POINT('Ctrl Pts',(4.71371668580301,-80.878019107145,-8.16439679232994));
#17853=CARTESIAN_POINT('Ctrl Pts',(-1.4702867290402E-11,-80.703019107145,
-8.16439679232146));
#17854=CARTESIAN_POINT('Ctrl Pts',(-4.71371668583241,-80.528019107145,-8.16439679231297));
#17855=CARTESIAN_POINT('Ctrl Pts',(-7.07057502873392,-80.353019107145,-4.082198396148));
#17856=CARTESIAN_POINT('Ctrl Pts',(-9.42743337163542,-80.178019107145,1.69768315121407E-11));
#17857=CARTESIAN_POINT('Ctrl Pts',(-7.07057502871922,-80.003019107145,4.08219839617346));
#17858=CARTESIAN_POINT('Ctrl Pts',(-4.71371668580301,-79.828019107145,8.16439679232994));
#17859=CARTESIAN_POINT('Ctrl Pts',(1.47018674401621E-11,-79.653019107145,
8.16439679232146));
#17860=CARTESIAN_POINT('Ctrl Pts',(4.71371668583241,-79.478019107145,8.16439679231297));
#17861=CARTESIAN_POINT('Ctrl Pts',(7.07057502873392,-79.303019107145,4.082198396148));
#17862=CARTESIAN_POINT('Ctrl Pts',(9.42743337163542,-79.128019107145,-1.69756769845304E-11));
#17863=CARTESIAN_POINT('Ctrl Pts',(7.07057502871922,-78.953019107145,-4.08219839617346));
#17864=CARTESIAN_POINT('Ctrl Pts',(4.71371668580301,-78.778019107145,-8.16439679232994));
#17865=CARTESIAN_POINT('Ctrl Pts',(-1.4702867290402E-11,-78.603019107145,
-8.16439679232146));
#17866=CARTESIAN_POINT('Ctrl Pts',(-4.71371668583241,-78.428019107145,-8.16439679231297));
#17867=CARTESIAN_POINT('Ctrl Pts',(-7.07057502873392,-78.253019107145,-4.082198396148));
#17868=CARTESIAN_POINT('Ctrl Pts',(-9.42743337163542,-78.078019107145,1.69768315121407E-11));
#17869=CARTESIAN_POINT('Ctrl Pts',(-7.07057502871922,-77.903019107145,4.08219839617346));
#17870=CARTESIAN_POINT('Ctrl Pts',(-4.71371668580301,-77.728019107145,8.16439679232994));
#17871=CARTESIAN_POINT('Ctrl Pts',(1.47018674401621E-11,-77.553019107145,
8.16439679232146));
#17872=CARTESIAN_POINT('Ctrl Pts',(4.71371668583241,-77.378019107145,8.16439679231297));
#17873=CARTESIAN_POINT('Ctrl Pts',(7.07057502873392,-77.203019107145,4.082198396148));
#17874=CARTESIAN_POINT('Ctrl Pts',(9.42743337163542,-77.028019107145,-1.69756769845304E-11));
#17875=CARTESIAN_POINT('Ctrl Pts',(7.07057502871922,-76.853019107145,-4.08219839617346));
#17876=CARTESIAN_POINT('Ctrl Pts',(4.71371668580301,-76.678019107145,-8.16439679232994));
#17877=CARTESIAN_POINT('Ctrl Pts',(-1.4702867290402E-11,-76.503019107145,
-8.16439679232146));
#17878=CARTESIAN_POINT('Ctrl Pts',(-4.71371668583241,-76.328019107145,-8.16439679231297));
#17879=CARTESIAN_POINT('Ctrl Pts',(-7.07057502873392,-76.153019107145,-4.082198396148));
#17880=CARTESIAN_POINT('Ctrl Pts',(-9.42743337163542,-75.978019107145,1.69768315121407E-11));
#17881=CARTESIAN_POINT('Ctrl Pts',(-7.07057502871922,-75.803019107145,4.08219839617346));
#17882=CARTESIAN_POINT('Ctrl Pts',(-4.71371668580301,-75.628019107145,8.16439679232994));
#17883=CARTESIAN_POINT('Ctrl Pts',(1.47018674401621E-11,-75.453019107145,
8.16439679232146));
#17884=CARTESIAN_POINT('Ctrl Pts',(4.71371668583241,-75.278019107145,8.16439679231297));
#17885=CARTESIAN_POINT('Ctrl Pts',(7.07057502873392,-75.103019107145,4.082198396148));
#17886=CARTESIAN_POINT('Ctrl Pts',(9.42743337163542,-74.928019107145,-1.69756769845304E-11));
#17887=CARTESIAN_POINT('Ctrl Pts',(7.07057502871922,-74.753019107145,-4.08219839617346));
#17888=CARTESIAN_POINT('Ctrl Pts',(4.71371668580301,-74.578019107145,-8.16439679232994));
#17889=CARTESIAN_POINT('Ctrl Pts',(-1.4702867290402E-11,-74.403019107145,
-8.16439679232146));
#17890=CARTESIAN_POINT('Ctrl Pts',(-4.71371668583241,-74.228019107145,-8.16439679231297));
#17891=CARTESIAN_POINT('Ctrl Pts',(-7.07057502873392,-74.053019107145,-4.082198396148));
#17892=CARTESIAN_POINT('Ctrl Pts',(-9.42743337163542,-73.878019107145,1.69768315121407E-11));
#17893=CARTESIAN_POINT('Ctrl Pts',(-7.07057502871922,-73.703019107145,4.08219839617346));
#17894=CARTESIAN_POINT('Ctrl Pts',(-4.71371668580301,-73.528019107145,8.16439679232994));
#17895=CARTESIAN_POINT('Ctrl Pts',(1.47018674401621E-11,-73.353019107145,
8.16439679232146));
#17896=CARTESIAN_POINT('Ctrl Pts',(4.71371668583241,-73.178019107145,8.16439679231297));
#17897=CARTESIAN_POINT('Ctrl Pts',(7.07057502873392,-73.003019107145,4.082198396148));
#17898=CARTESIAN_POINT('Ctrl Pts',(9.42743337163542,-72.828019107145,-1.69756769845304E-11));
#17899=CARTESIAN_POINT('Ctrl Pts',(7.07057502871922,-72.653019107145,-4.08219839617346));
#17900=CARTESIAN_POINT('Ctrl Pts',(4.71371668580301,-72.478019107145,-8.16439679232994));
#17901=CARTESIAN_POINT('Ctrl Pts',(-1.4702867290402E-11,-72.303019107145,
-8.16439679232146));
#17902=CARTESIAN_POINT('Ctrl Pts',(-4.71371668583241,-72.128019107145,-8.16439679231297));
#17903=CARTESIAN_POINT('Ctrl Pts',(-7.07057502873392,-71.953019107145,-4.082198396148));
#17904=CARTESIAN_POINT('Ctrl Pts',(-9.42743337163542,-71.778019107145,1.69768315121407E-11));
#17905=CARTESIAN_POINT('Ctrl Pts',(-7.07057502871922,-71.603019107145,4.08219839617346));
#17906=CARTESIAN_POINT('Ctrl Pts',(-4.71371668580301,-71.428019107145,8.16439679232994));
#17907=CARTESIAN_POINT('Ctrl Pts',(1.47018674401621E-11,-71.253019107145,
8.16439679232146));
#17908=CARTESIAN_POINT('Ctrl Pts',(4.71371668583241,-71.078019107145,8.16439679231297));
#17909=CARTESIAN_POINT('Ctrl Pts',(7.07057502873392,-70.903019107145,4.082198396148));
#17910=CARTESIAN_POINT('Ctrl Pts',(9.42743337163542,-70.728019107145,-1.69756769845304E-11));
#17911=CARTESIAN_POINT('Ctrl Pts',(7.07057502871922,-70.553019107145,-4.08219839617346));
#17912=CARTESIAN_POINT('Ctrl Pts',(4.71371668580301,-70.378019107145,-8.16439679232994));
#17913=CARTESIAN_POINT('Ctrl Pts',(-1.4702867290402E-11,-70.203019107145,
-8.16439679232146));
#17914=CARTESIAN_POINT('Ctrl Pts',(-4.71371668583241,-70.028019107145,-8.16439679231297));
#17915=CARTESIAN_POINT('Ctrl Pts',(-7.07057502873392,-69.853019107145,-4.082198396148));
#17916=CARTESIAN_POINT('Ctrl Pts',(-9.42743337163542,-69.678019107145,1.69768315121407E-11));
#17917=CARTESIAN_POINT('Ctrl Pts',(-7.07057502871922,-69.503019107145,4.08219839617346));
#17918=CARTESIAN_POINT('Ctrl Pts',(-4.71371668580301,-69.328019107145,8.16439679232994));
#17919=CARTESIAN_POINT('Ctrl Pts',(1.47018674401621E-11,-69.153019107145,
8.16439679232146));
#17920=CARTESIAN_POINT('Ctrl Pts',(4.71371668583241,-68.978019107145,8.16439679231297));
#17921=CARTESIAN_POINT('Ctrl Pts',(7.07057502873392,-68.803019107145,4.082198396148));
#17922=CARTESIAN_POINT('Ctrl Pts',(9.42743337163542,-68.6280191071451,-1.69756769845304E-11));
#17923=CARTESIAN_POINT('Ctrl Pts',(7.07057502871922,-68.453019107145,-4.08219839617346));
#17924=CARTESIAN_POINT('Ctrl Pts',(4.71371668580301,-68.278019107145,-8.16439679232994));
#17925=CARTESIAN_POINT('Ctrl Pts',(-1.4702867290402E-11,-68.103019107145,
-8.16439679232146));
#17926=CARTESIAN_POINT('Ctrl Pts',(-4.71371668583241,-67.928019107145,-8.16439679231297));
#17927=CARTESIAN_POINT('Ctrl Pts',(-7.07057502873392,-67.753019107145,-4.082198396148));
#17928=CARTESIAN_POINT('Ctrl Pts',(-9.42743337163542,-67.5780191071451,
1.69768315121407E-11));
#17929=CARTESIAN_POINT('Ctrl Pts',(-7.07057502871922,-67.403019107145,4.08219839617346));
#17930=CARTESIAN_POINT('Ctrl Pts',(-4.71371668580301,-67.228019107145,8.16439679232994));
#17931=CARTESIAN_POINT('Ctrl Pts',(1.47018674401621E-11,-67.053019107145,
8.16439679232146));
#17932=CARTESIAN_POINT('Ctrl Pts',(4.71371668583241,-66.878019107145,8.16439679231297));
#17933=CARTESIAN_POINT('Ctrl Pts',(7.07057502873392,-66.703019107145,4.082198396148));
#17934=CARTESIAN_POINT('Ctrl Pts',(9.42743337163542,-66.5280191071451,-1.69756769845304E-11));
#17935=CARTESIAN_POINT('Ctrl Pts',(7.07057502871922,-66.353019107145,-4.08219839617346));
#17936=CARTESIAN_POINT('Ctrl Pts',(4.71371668580301,-66.178019107145,-8.16439679232994));
#17937=CARTESIAN_POINT('Ctrl Pts',(-1.4702867290402E-11,-66.003019107145,
-8.16439679232146));
#17938=CARTESIAN_POINT('Ctrl Pts',(-4.71371668583241,-65.828019107145,-8.16439679231297));
#17939=CARTESIAN_POINT('Ctrl Pts',(-7.07057502873392,-65.653019107145,-4.082198396148));
#17940=CARTESIAN_POINT('Ctrl Pts',(-9.42743337163542,-65.478019107145,1.69768315121407E-11));
#17941=CARTESIAN_POINT('Ctrl Pts',(-7.07057502871922,-65.303019107145,4.08219839617346));
#17942=CARTESIAN_POINT('Ctrl Pts',(-4.71371668580301,-65.1280191071451,
8.16439679232994));
#17943=CARTESIAN_POINT('Ctrl Pts',(1.47018674401621E-11,-64.953019107145,
8.16439679232146));
#17944=CARTESIAN_POINT('Ctrl Pts',(4.71371668583241,-64.778019107145,8.16439679231297));
#17945=CARTESIAN_POINT('Ctrl Pts',(7.07057502873392,-64.603019107145,4.082198396148));
#17946=CARTESIAN_POINT('Ctrl Pts',(9.42743337163542,-64.428019107145,-1.69756769845304E-11));
#17947=CARTESIAN_POINT('Ctrl Pts',(7.07057502871922,-64.253019107145,-4.08219839617346));
#17948=CARTESIAN_POINT('Ctrl Pts',(4.71371668580301,-64.0780191071451,-8.16439679232994));
#17949=CARTESIAN_POINT('Ctrl Pts',(-1.4702867290402E-11,-63.903019107145,
-8.16439679232146));
#17950=CARTESIAN_POINT('Ctrl Pts',(-4.71371668583241,-63.728019107145,-8.16439679231297));
#17951=CARTESIAN_POINT('Ctrl Pts',(-7.07057502873392,-63.553019107145,-4.082198396148));
#17952=CARTESIAN_POINT('Ctrl Pts',(-9.42743337163542,-63.378019107145,1.69768315121407E-11));
#17953=CARTESIAN_POINT('Ctrl Pts',(-7.07057502871922,-63.203019107145,4.08219839617346));
#17954=CARTESIAN_POINT('Ctrl Pts',(-4.71371668580301,-63.028019107145,8.16439679232994));
#17955=CARTESIAN_POINT('Ctrl Pts',(1.47018674401621E-11,-62.853019107145,
8.16439679232146));
#17956=CARTESIAN_POINT('Ctrl Pts',(4.71371668583241,-62.678019107145,8.16439679231297));
#17957=CARTESIAN_POINT('Ctrl Pts',(7.07057502873392,-62.503019107145,4.082198396148));
#17958=CARTESIAN_POINT('Ctrl Pts',(9.42743337163542,-62.328019107145,-1.69756769845304E-11));
#17959=CARTESIAN_POINT('Ctrl Pts',(7.07057502871922,-62.153019107145,-4.08219839617346));
#17960=CARTESIAN_POINT('Ctrl Pts',(4.71371668580301,-61.978019107145,-8.16439679232994));
#17961=CARTESIAN_POINT('Ctrl Pts',(-1.4702867290402E-11,-61.803019107145,
-8.16439679232146));
#17962=CARTESIAN_POINT('Ctrl Pts',(-4.71371668583241,-61.628019107145,-8.16439679231297));
#17963=CARTESIAN_POINT('Ctrl Pts',(-7.07057502873392,-61.453019107145,-4.082198396148));
#17964=CARTESIAN_POINT('Ctrl Pts',(-9.42743337163542,-61.278019107145,1.69768315121407E-11));
#17965=CARTESIAN_POINT('Ctrl Pts',(-7.07057502871922,-61.103019107145,4.08219839617346));
#17966=CARTESIAN_POINT('Ctrl Pts',(-4.71371668580301,-60.9280191071451,
8.16439679232994));
#17967=CARTESIAN_POINT('Ctrl Pts',(1.47018674401621E-11,-60.753019107145,
8.16439679232146));
#17968=CARTESIAN_POINT('Ctrl Pts',(4.71371668583241,-60.578019107145,8.16439679231297));
#17969=CARTESIAN_POINT('Ctrl Pts',(7.07057502873392,-60.403019107145,4.082198396148));
#17970=CARTESIAN_POINT('Ctrl Pts',(9.42743337163542,-60.228019107145,-1.69756769845304E-11));
#17971=CARTESIAN_POINT('Ctrl Pts',(7.07057502871922,-60.053019107145,-4.08219839617346));
#17972=CARTESIAN_POINT('Ctrl Pts',(4.71371668580301,-59.8780191071451,-8.16439679232994));
#17973=CARTESIAN_POINT('Ctrl Pts',(-1.4702867290402E-11,-59.703019107145,
-8.16439679232146));
#17974=CARTESIAN_POINT('Ctrl Pts',(-4.71371668583241,-59.528019107145,-8.16439679231297));
#17975=CARTESIAN_POINT('Ctrl Pts',(-7.07057502873392,-59.3530191071451,
-4.082198396148));
#17976=CARTESIAN_POINT('Ctrl Pts',(-9.42743337163542,-59.178019107145,1.69768315121407E-11));
#17977=CARTESIAN_POINT('Ctrl Pts',(-7.07057502871922,-59.003019107145,4.08219839617346));
#17978=CARTESIAN_POINT('Ctrl Pts',(-4.71371668580301,-58.8280191071451,
8.16439679232994));
#17979=CARTESIAN_POINT('Ctrl Pts',(1.47018674401621E-11,-58.653019107145,
8.16439679232146));
#17980=CARTESIAN_POINT('Ctrl Pts',(4.71371668583241,-58.478019107145,8.16439679231297));
#17981=CARTESIAN_POINT('Ctrl Pts',(7.07057502873392,-58.303019107145,4.082198396148));
#17982=CARTESIAN_POINT('Ctrl Pts',(9.42743337163542,-58.128019107145,-1.69756769845304E-11));
#17983=CARTESIAN_POINT('Ctrl Pts',(7.07057502871922,-57.953019107145,-4.08219839617346));
#17984=CARTESIAN_POINT('Ctrl Pts',(4.71371668580301,-57.7780191071451,-8.16439679232994));
#17985=CARTESIAN_POINT('Ctrl Pts',(-1.4702867290402E-11,-57.603019107145,
-8.16439679232146));
#17986=CARTESIAN_POINT('Ctrl Pts',(-4.71371668583241,-57.428019107145,-8.16439679231297));
#17987=CARTESIAN_POINT('Ctrl Pts',(-7.07057502873392,-57.253019107145,-4.082198396148));
#17988=CARTESIAN_POINT('Ctrl Pts',(-9.42743337163542,-57.078019107145,1.69768315121407E-11));
#17989=CARTESIAN_POINT('Ctrl Pts',(-7.07057502871922,-56.903019107145,4.08219839617346));
#17990=CARTESIAN_POINT('Ctrl Pts',(-4.71371668580301,-56.728019107145,8.16439679232994));
#17991=CARTESIAN_POINT('Ctrl Pts',(1.47018674401621E-11,-56.553019107145,
8.16439679232146));
#17992=CARTESIAN_POINT('Ctrl Pts',(4.71371668583241,-56.3780191071451,8.16439679231297));
#17993=CARTESIAN_POINT('Ctrl Pts',(7.07057502873392,-56.203019107145,4.082198396148));
#17994=CARTESIAN_POINT('Ctrl Pts',(9.42743337163542,-56.028019107145,-1.69756769845304E-11));
#17995=CARTESIAN_POINT('Ctrl Pts',(7.07057502871922,-55.8530191071451,-4.08219839617346));
#17996=CARTESIAN_POINT('Ctrl Pts',(4.71371668580301,-55.678019107145,-8.16439679232994));
#17997=CARTESIAN_POINT('Ctrl Pts',(-1.4702867290402E-11,-55.503019107145,
-8.16439679232146));
#17998=CARTESIAN_POINT('Ctrl Pts',(-4.71371668583241,-55.3280191071451,
-8.16439679231297));
#17999=CARTESIAN_POINT('Ctrl Pts',(-7.07057502873392,-55.153019107145,-4.082198396148));
#18000=CARTESIAN_POINT('Ctrl Pts',(-9.42743337163542,-54.9780191071451,
1.69768315121407E-11));
#18001=CARTESIAN_POINT('Ctrl Pts',(-7.07057502871922,-54.8030191071451,
4.08219839617346));
#18002=CARTESIAN_POINT('Ctrl Pts',(-4.71371668580301,-54.628019107145,8.16439679232994));
#18003=CARTESIAN_POINT('Ctrl Pts',(1.47018674401621E-11,-54.453019107145,
8.16439679232146));
#18004=CARTESIAN_POINT('Ctrl Pts',(4.71371668583241,-54.278019107145,8.16439679231297));
#18005=CARTESIAN_POINT('Ctrl Pts',(7.07057502873392,-54.1030191071451,4.082198396148));
#18006=CARTESIAN_POINT('Ctrl Pts',(9.42743337163542,-53.9280191071451,-1.69756769845304E-11));
#18007=CARTESIAN_POINT('Ctrl Pts',(7.07057502871922,-53.7530191071451,-4.08219839617346));
#18008=CARTESIAN_POINT('Ctrl Pts',(4.71371668580301,-53.5780191071451,-8.16439679232994));
#18009=CARTESIAN_POINT('Ctrl Pts',(-1.4702867290402E-11,-53.403019107145,
-8.16439679232146));
#18010=CARTESIAN_POINT('Ctrl Pts',(-4.71371668583241,-53.228019107145,-8.16439679231297));
#18011=CARTESIAN_POINT('Ctrl Pts',(-7.07057502873392,-53.0530191071451,
-4.082198396148));
#18012=CARTESIAN_POINT('Ctrl Pts',(-9.42743337163542,-52.878019107145,1.69768315121407E-11));
#18013=CARTESIAN_POINT('Ctrl Pts',(-7.07057502871922,-52.703019107145,4.08219839617346));
#18014=CARTESIAN_POINT('Ctrl Pts',(-4.71371668580301,-52.528019107145,8.16439679232994));
#18015=CARTESIAN_POINT('Ctrl Pts',(1.47018674401621E-11,-52.3530191071451,
8.16439679232146));
#18016=CARTESIAN_POINT('Ctrl Pts',(4.71371668583241,-52.178019107145,8.16439679231297));
#18017=CARTESIAN_POINT('Ctrl Pts',(7.07057502873392,-52.0030191071451,4.082198396148));
#18018=CARTESIAN_POINT('Ctrl Pts',(9.42743337163542,-51.828019107145,-1.69756769845304E-11));
#18019=CARTESIAN_POINT('Ctrl Pts',(7.07057502871922,-51.6530191071451,-4.08219839617346));
#18020=CARTESIAN_POINT('Ctrl Pts',(4.71371668580301,-51.4780191071451,-8.16439679232994));
#18021=CARTESIAN_POINT('Ctrl Pts',(-1.4702867290402E-11,-51.303019107145,
-8.16439679232146));
#18022=CARTESIAN_POINT('Ctrl Pts',(-4.71371668583241,-51.1280191071451,
-8.16439679231297));
#18023=CARTESIAN_POINT('Ctrl Pts',(-7.07057502873392,-50.9530191071451,
-4.082198396148));
#18024=CARTESIAN_POINT('Ctrl Pts',(-9.42743337163542,-50.778019107145,1.69768315121407E-11));
#18025=CARTESIAN_POINT('Ctrl Pts',(-7.07057502871922,-50.6030191071451,
4.08219839617346));
#18026=CARTESIAN_POINT('Ctrl Pts',(-4.71371668580301,-50.4280191071451,
8.16439679232994));
#18027=CARTESIAN_POINT('Ctrl Pts',(1.47018674401621E-11,-50.253019107145,
8.16439679232146));
#18028=CARTESIAN_POINT('Ctrl Pts',(4.71371668583241,-50.0780191071451,8.16439679231297));
#18029=CARTESIAN_POINT('Ctrl Pts',(7.07057502873392,-49.9030191071451,4.082198396148));
#18030=CARTESIAN_POINT('Ctrl Pts',(9.42743337163542,-49.728019107145,-1.69756769845304E-11));
#18031=CARTESIAN_POINT('Ctrl Pts',(7.07057502871922,-49.5530191071451,-4.08219839617346));
#18032=CARTESIAN_POINT('Ctrl Pts',(4.71371668580301,-49.3780191071451,-8.16439679232994));
#18033=CARTESIAN_POINT('Ctrl Pts',(-1.4702867290402E-11,-49.2030191071451,
-8.16439679232146));
#18034=CARTESIAN_POINT('Ctrl Pts',(-4.71371668583241,-49.028019107145,-8.16439679231297));
#18035=CARTESIAN_POINT('Ctrl Pts',(-7.07057502873392,-48.853019107145,-4.082198396148));
#18036=CARTESIAN_POINT('Ctrl Pts',(-9.42743337163542,-48.6780191071451,
1.69768315121407E-11));
#18037=CARTESIAN_POINT('Ctrl Pts',(-7.07057502871922,-48.5030191071451,
4.08219839617346));
#18038=CARTESIAN_POINT('Ctrl Pts',(-4.71371668580301,-48.3280191071451,
8.16439679232994));
#18039=CARTESIAN_POINT('Ctrl Pts',(1.47018674401621E-11,-48.1530191071451,
8.16439679232146));
#18040=CARTESIAN_POINT('Ctrl Pts',(4.71371668583241,-47.9780191071451,8.16439679231297));
#18041=CARTESIAN_POINT('Ctrl Pts',(7.07057502873392,-47.8030191071451,4.082198396148));
#18042=CARTESIAN_POINT('Ctrl Pts',(9.42743337163542,-47.6280191071451,-1.69756769845304E-11));
#18043=CARTESIAN_POINT('Ctrl Pts',(7.07057502871922,-47.4530191071451,-4.08219839617346));
#18044=CARTESIAN_POINT('Ctrl Pts',(4.71371668580301,-47.2780191071451,-8.16439679232994));
#18045=CARTESIAN_POINT('Ctrl Pts',(-1.4702867290402E-11,-47.1030191071451,
-8.16439679232146));
#18046=CARTESIAN_POINT('Ctrl Pts',(-4.71371668583241,-46.9280191071451,
-8.16439679231297));
#18047=CARTESIAN_POINT('Ctrl Pts',(-7.07057502873392,-46.7530191071451,
-4.082198396148));
#18048=CARTESIAN_POINT('Ctrl Pts',(-9.42743337163542,-46.5780191071451,
1.69768315121407E-11));
#18049=CARTESIAN_POINT('Ctrl Pts',(-7.07057502871922,-46.4030191071451,
4.08219839617346));
#18050=CARTESIAN_POINT('Ctrl Pts',(-4.71371668580301,-46.2280191071451,
8.16439679232994));
#18051=CARTESIAN_POINT('Ctrl Pts',(1.47018674401621E-11,-46.0530191071451,
8.16439679232146));
#18052=CARTESIAN_POINT('Ctrl Pts',(4.71371668583241,-45.8780191071451,8.16439679231297));
#18053=CARTESIAN_POINT('Ctrl Pts',(7.07057502873392,-45.7030191071451,4.082198396148));
#18054=CARTESIAN_POINT('Ctrl Pts',(9.42743337163542,-45.5280191071451,-1.69756769845304E-11));
#18055=CARTESIAN_POINT('Ctrl Pts',(7.07057502871922,-45.3530191071451,-4.08219839617346));
#18056=CARTESIAN_POINT('Ctrl Pts',(4.71371668580301,-45.1780191071451,-8.16439679232994));
#18057=CARTESIAN_POINT('Ctrl Pts',(-1.4702867290402E-11,-45.0030191071451,
-8.16439679232146));
#18058=CARTESIAN_POINT('Ctrl Pts',(-4.71371668583241,-44.8280191071451,
-8.16439679231297));
#18059=CARTESIAN_POINT('Ctrl Pts',(-7.07057502873392,-44.6530191071451,
-4.082198396148));
#18060=CARTESIAN_POINT('Ctrl Pts',(-9.42743337163542,-44.4780191071451,
1.69768315121407E-11));
#18061=CARTESIAN_POINT('Ctrl Pts',(-7.07057502871922,-44.3030191071451,
4.08219839617346));
#18062=CARTESIAN_POINT('Ctrl Pts',(-4.71371668580301,-44.1280191071451,
8.16439679232994));
#18063=CARTESIAN_POINT('Ctrl Pts',(1.47018674401621E-11,-43.9530191071451,
8.16439679232146));
#18064=CARTESIAN_POINT('Ctrl Pts',(4.71371668583241,-43.7780191071451,8.16439679231297));
#18065=CARTESIAN_POINT('Ctrl Pts',(7.07057502873392,-43.6030191071451,4.082198396148));
#18066=CARTESIAN_POINT('Ctrl Pts',(9.42743337163542,-43.4280191071451,-1.69756769845304E-11));
#18067=CARTESIAN_POINT('Ctrl Pts',(7.07057502871922,-43.2530191071451,-4.08219839617346));
#18068=CARTESIAN_POINT('Ctrl Pts',(4.71371668580301,-43.0780191071451,-8.16439679232994));
#18069=CARTESIAN_POINT('Ctrl Pts',(-1.4702867290402E-11,-42.9030191071451,
-8.16439679232146));
#18070=CARTESIAN_POINT('Ctrl Pts',(-4.71371668583241,-42.7280191071451,
-8.16439679231297));
#18071=CARTESIAN_POINT('Ctrl Pts',(-7.07057502873392,-42.5530191071451,
-4.082198396148));
#18072=CARTESIAN_POINT('Ctrl Pts',(-9.42743337163542,-42.3780191071451,
1.69768315121407E-11));
#18073=CARTESIAN_POINT('Ctrl Pts',(-7.07057502871922,-42.2030191071451,
4.08219839617346));
#18074=CARTESIAN_POINT('Ctrl Pts',(-4.71371668580301,-42.0280191071451,
8.16439679232994));
#18075=CARTESIAN_POINT('Ctrl Pts',(1.47018674401621E-11,-41.8530191071451,
8.16439679232146));
#18076=CARTESIAN_POINT('Ctrl Pts',(4.71371668583241,-41.6780191071451,8.16439679231297));
#18077=CARTESIAN_POINT('Ctrl Pts',(7.07057502873392,-41.5030191071451,4.082198396148));
#18078=CARTESIAN_POINT('Ctrl Pts',(9.42743337163542,-41.3280191071451,-1.69756769845304E-11));
#18079=CARTESIAN_POINT('Ctrl Pts',(7.07057502871922,-41.1530191071451,-4.08219839617346));
#18080=CARTESIAN_POINT('Ctrl Pts',(4.71371668580301,-40.9780191071451,-8.16439679232994));
#18081=CARTESIAN_POINT('Ctrl Pts',(-1.4702867290402E-11,-40.8030191071451,
-8.16439679232146));
#18082=CARTESIAN_POINT('Ctrl Pts',(-4.71371668583241,-40.6280191071451,
-8.16439679231297));
#18083=CARTESIAN_POINT('Ctrl Pts',(-7.07057502873392,-40.4530191071451,
-4.082198396148));
#18084=CARTESIAN_POINT('Ctrl Pts',(-9.42743337163542,-40.2780191071451,
1.69768315121407E-11));
#18085=CARTESIAN_POINT('Ctrl Pts',(-7.07057502871922,-40.1030191071451,
4.08219839617346));
#18086=CARTESIAN_POINT('Ctrl Pts',(-4.71371668580301,-39.9280191071451,
8.16439679232994));
#18087=CARTESIAN_POINT('Ctrl Pts',(1.47018674401621E-11,-39.7530191071451,
8.16439679232146));
#18088=CARTESIAN_POINT('Ctrl Pts',(4.71371668583241,-39.5780191071451,8.16439679231297));
#18089=CARTESIAN_POINT('Ctrl Pts',(7.07057502873392,-39.4030191071451,4.082198396148));
#18090=CARTESIAN_POINT('Ctrl Pts',(9.42743337163542,-39.2280191071451,-1.69756769845304E-11));
#18091=CARTESIAN_POINT('Ctrl Pts',(7.07057502871922,-39.0530191071451,-4.08219839617346));
#18092=CARTESIAN_POINT('Ctrl Pts',(4.71371668580301,-38.8780191071451,-8.16439679232994));
#18093=CARTESIAN_POINT('Ctrl Pts',(-1.4702867290402E-11,-38.7030191071451,
-8.16439679232146));
#18094=CARTESIAN_POINT('Ctrl Pts',(-4.71371668583241,-38.5280191071451,
-8.16439679231297));
#18095=CARTESIAN_POINT('Ctrl Pts',(-7.07057502873392,-38.3530191071451,
-4.082198396148));
#18096=CARTESIAN_POINT('Ctrl Pts',(-9.42743337163542,-38.1780191071451,
1.69768315121407E-11));
#18097=CARTESIAN_POINT('Ctrl Pts',(-7.07057502871922,-38.0030191071451,
4.08219839617346));
#18098=CARTESIAN_POINT('Ctrl Pts',(-4.71371668580301,-37.8280191071451,
8.16439679232994));
#18099=CARTESIAN_POINT('Ctrl Pts',(1.47018674401621E-11,-37.6530191071451,
8.16439679232146));
#18100=CARTESIAN_POINT('Ctrl Pts',(4.71371668583241,-37.4780191071451,8.16439679231297));
#18101=CARTESIAN_POINT('Ctrl Pts',(7.07057502873392,-37.3030191071451,4.082198396148));
#18102=CARTESIAN_POINT('Ctrl Pts',(9.42743337163542,-37.1280191071451,-1.69756769845304E-11));
#18103=CARTESIAN_POINT('Ctrl Pts',(7.07057502871922,-36.9530191071451,-4.08219839617346));
#18104=CARTESIAN_POINT('Ctrl Pts',(4.71371668580301,-36.7780191071451,-8.16439679232994));
#18105=CARTESIAN_POINT('Ctrl Pts',(-1.4702867290402E-11,-36.6030191071451,
-8.16439679232146));
#18106=CARTESIAN_POINT('Ctrl Pts',(-4.71371668583241,-36.4280191071451,
-8.16439679231297));
#18107=CARTESIAN_POINT('Ctrl Pts',(-7.07057502873392,-36.2530191071451,
-4.082198396148));
#18108=CARTESIAN_POINT('Ctrl Pts',(-9.42743337163542,-36.0780191071451,
1.69768315121407E-11));
#18109=CARTESIAN_POINT('Ctrl Pts',(-7.07057502871922,-35.9030191071451,
4.08219839617346));
#18110=CARTESIAN_POINT('Ctrl Pts',(-4.71371668580301,-35.7280191071451,
8.16439679232994));
#18111=CARTESIAN_POINT('Ctrl Pts',(1.47018674401621E-11,-35.5530191071451,
8.16439679232146));
#18112=CARTESIAN_POINT('Ctrl Pts',(4.71371668583241,-35.3780191071451,8.16439679231297));
#18113=CARTESIAN_POINT('Ctrl Pts',(7.07057502873392,-35.2030191071451,4.082198396148));
#18114=CARTESIAN_POINT('Ctrl Pts',(9.42743337163542,-35.0280191071451,-1.69756769845304E-11));
#18115=CARTESIAN_POINT('Ctrl Pts',(7.07057502871922,-34.8530191071451,-4.08219839617346));
#18116=CARTESIAN_POINT('Ctrl Pts',(4.71371668580301,-34.6780191071451,-8.16439679232994));
#18117=CARTESIAN_POINT('Ctrl Pts',(-1.4702867290402E-11,-34.5030191071451,
-8.16439679232146));
#18118=CARTESIAN_POINT('Ctrl Pts',(-4.71371668583241,-34.3280191071451,
-8.16439679231297));
#18119=CARTESIAN_POINT('Ctrl Pts',(-7.07057502873392,-34.1530191071451,
-4.082198396148));
#18120=CARTESIAN_POINT('Ctrl Pts',(-9.42743337163542,-33.9780191071451,
1.69768315121407E-11));
#18121=CARTESIAN_POINT('Ctrl Pts',(-7.07057502871922,-33.8030191071451,
4.08219839617346));
#18122=CARTESIAN_POINT('Ctrl Pts',(-4.71371668580301,-33.6280191071451,
8.16439679232994));
#18123=CARTESIAN_POINT('Ctrl Pts',(1.47018674401621E-11,-33.4530191071451,
8.16439679232146));
#18124=CARTESIAN_POINT('Ctrl Pts',(4.71371668583241,-33.2780191071451,8.16439679231297));
#18125=CARTESIAN_POINT('Ctrl Pts',(7.07057502873392,-33.1030191071451,4.082198396148));
#18126=CARTESIAN_POINT('Ctrl Pts',(9.42743337163542,-32.9280191071451,-1.69756769845304E-11));
#18127=CARTESIAN_POINT('Ctrl Pts',(7.07057502871922,-32.7530191071451,-4.08219839617346));
#18128=CARTESIAN_POINT('Ctrl Pts',(4.71371668580301,-32.5780191071451,-8.16439679232994));
#18129=CARTESIAN_POINT('Ctrl Pts',(-1.4702867290402E-11,-32.4030191071451,
-8.16439679232146));
#18130=CARTESIAN_POINT('Ctrl Pts',(-4.71371668583241,-32.2280191071451,
-8.16439679231297));
#18131=CARTESIAN_POINT('Ctrl Pts',(-7.07057502873392,-32.0530191071451,
-4.082198396148));
#18132=CARTESIAN_POINT('Ctrl Pts',(-9.42743337163542,-31.8780191071451,
1.69768315121407E-11));
#18133=CARTESIAN_POINT('Ctrl Pts',(-7.07057502871922,-31.7030191071451,
4.08219839617346));
#18134=CARTESIAN_POINT('Ctrl Pts',(-4.71371668580301,-31.5280191071451,
8.16439679232994));
#18135=CARTESIAN_POINT('Ctrl Pts',(1.47018674401621E-11,-31.3530191071451,
8.16439679232146));
#18136=CARTESIAN_POINT('Ctrl Pts',(4.71371668583241,-31.1780191071451,8.16439679231297));
#18137=CARTESIAN_POINT('Ctrl Pts',(7.07057502873392,-31.0030191071451,4.082198396148));
#18138=CARTESIAN_POINT('Ctrl Pts',(9.42743337163542,-30.8280191071451,-1.69756769845304E-11));
#18139=CARTESIAN_POINT('Ctrl Pts',(7.07057502871922,-30.6530191071451,-4.08219839617346));
#18140=CARTESIAN_POINT('Ctrl Pts',(4.71371668580301,-30.4780191071451,-8.16439679232994));
#18141=CARTESIAN_POINT('Ctrl Pts',(-1.4702867290402E-11,-30.3030191071451,
-8.16439679232146));
#18142=CARTESIAN_POINT('Ctrl Pts',(-4.71371668583241,-30.1280191071451,
-8.16439679231297));
#18143=CARTESIAN_POINT('Ctrl Pts',(-7.07057502873392,-29.9530191071451,
-4.082198396148));
#18144=CARTESIAN_POINT('Ctrl Pts',(-9.42743337163542,-29.7780191071451,
1.69768315121407E-11));
#18145=CARTESIAN_POINT('Ctrl Pts',(-7.07057502871922,-29.6030191071451,
4.08219839617346));
#18146=CARTESIAN_POINT('Ctrl Pts',(-4.71371668580301,-29.4280191071451,
8.16439679232994));
#18147=CARTESIAN_POINT('Ctrl Pts',(1.47018674401621E-11,-29.2530191071451,
8.16439679232146));
#18148=CARTESIAN_POINT('Ctrl Pts',(4.71371668583241,-29.0780191071451,8.16439679231297));
#18149=CARTESIAN_POINT('Ctrl Pts',(7.07057502873392,-28.9030191071451,4.082198396148));
#18150=CARTESIAN_POINT('Ctrl Pts',(9.42743337163542,-28.7280191071451,-1.69756769845304E-11));
#18151=CARTESIAN_POINT('Ctrl Pts',(7.07057502871922,-28.5530191071451,-4.08219839617346));
#18152=CARTESIAN_POINT('Ctrl Pts',(4.71371668580301,-28.3780191071451,-8.16439679232994));
#18153=CARTESIAN_POINT('Ctrl Pts',(-1.4702867290402E-11,-28.2030191071451,
-8.16439679232146));
#18154=CARTESIAN_POINT('Ctrl Pts',(-4.71371668583241,-28.0280191071451,
-8.16439679231297));
#18155=CARTESIAN_POINT('Ctrl Pts',(-7.07057502873392,-27.8530191071451,
-4.082198396148));
#18156=CARTESIAN_POINT('Ctrl Pts',(-9.42743337163542,-27.6780191071451,
1.69768315121407E-11));
#18157=CARTESIAN_POINT('Ctrl Pts',(-7.07057502871922,-27.5030191071451,
4.08219839617346));
#18158=CARTESIAN_POINT('Ctrl Pts',(-4.71371668580301,-27.3280191071451,
8.16439679232994));
#18159=CARTESIAN_POINT('Ctrl Pts',(1.47018674401621E-11,-27.1530191071451,
8.16439679232146));
#18160=CARTESIAN_POINT('Ctrl Pts',(4.71371668583241,-26.9780191071451,8.16439679231297));
#18161=CARTESIAN_POINT('Ctrl Pts',(7.07057502873392,-26.8030191071451,4.082198396148));
#18162=CARTESIAN_POINT('Ctrl Pts',(9.42743337163542,-26.6280191071451,-1.69756769845304E-11));
#18163=CARTESIAN_POINT('Ctrl Pts',(7.07057502871922,-26.4530191071451,-4.08219839617346));
#18164=CARTESIAN_POINT('Ctrl Pts',(4.71371668580301,-26.2780191071451,-8.16439679232994));
#18165=CARTESIAN_POINT('Ctrl Pts',(-1.4702867290402E-11,-26.1030191071451,
-8.16439679232146));
#18166=CARTESIAN_POINT('Ctrl Pts',(-4.71371668583241,-25.9280191071451,
-8.16439679231297));
#18167=CARTESIAN_POINT('Ctrl Pts',(-7.07057502873392,-25.7530191071451,
-4.082198396148));
#18168=CARTESIAN_POINT('Ctrl Pts',(-9.42743337163542,-25.5780191071451,
1.69768315121407E-11));
#18169=CARTESIAN_POINT('Ctrl Pts',(-7.07057502871922,-25.4030191071451,
4.08219839617346));
#18170=CARTESIAN_POINT('Ctrl Pts',(-4.71371668580301,-25.2280191071451,
8.16439679232994));
#18171=CARTESIAN_POINT('Ctrl Pts',(1.47018674401621E-11,-25.0530191071451,
8.16439679232146));
#18172=CARTESIAN_POINT('Ctrl Pts',(4.71371668583241,-24.8780191071451,8.16439679231297));
#18173=CARTESIAN_POINT('Ctrl Pts',(7.07057502873392,-24.7030191071451,4.082198396148));
#18174=CARTESIAN_POINT('Ctrl Pts',(9.42743337163542,-24.5280191071451,-1.69756769845304E-11));
#18175=CARTESIAN_POINT('Ctrl Pts',(7.07057502871922,-24.3530191071451,-4.08219839617346));
#18176=CARTESIAN_POINT('Ctrl Pts',(4.71371668580301,-24.1780191071451,-8.16439679232994));
#18177=CARTESIAN_POINT('Ctrl Pts',(-1.4702867290402E-11,-24.0030191071451,
-8.16439679232146));
#18178=CARTESIAN_POINT('Ctrl Pts',(-4.71371668583241,-23.8280191071451,
-8.16439679231297));
#18179=CARTESIAN_POINT('Ctrl Pts',(-7.07057502873392,-23.6530191071451,
-4.082198396148));
#18180=CARTESIAN_POINT('Ctrl Pts',(-9.42743337163542,-23.4780191071451,
1.69768315121407E-11));
#18181=CARTESIAN_POINT('Ctrl Pts',(-7.07057502871922,-23.3030191071451,
4.08219839617346));
#18182=CARTESIAN_POINT('Ctrl Pts',(-4.71371668580301,-23.1280191071451,
8.16439679232994));
#18183=CARTESIAN_POINT('Ctrl Pts',(1.47018674401621E-11,-22.9530191071451,
8.16439679232146));
#18184=CARTESIAN_POINT('Ctrl Pts',(4.71371668583241,-22.7780191071451,8.16439679231297));
#18185=CARTESIAN_POINT('Ctrl Pts',(7.07057502873392,-22.6030191071451,4.082198396148));
#18186=CARTESIAN_POINT('Ctrl Pts',(9.42743337163542,-22.4280191071451,-1.69756769845304E-11));
#18187=CARTESIAN_POINT('Ctrl Pts',(7.07057502871922,-22.2530191071451,-4.08219839617346));
#18188=CARTESIAN_POINT('Ctrl Pts',(4.71371668580301,-22.0780191071451,-8.16439679232994));
#18189=CARTESIAN_POINT('Ctrl Pts',(-1.4702867290402E-11,-21.9030191071451,
-8.16439679232146));
#18190=CARTESIAN_POINT('Ctrl Pts',(-4.71371668583241,-21.7280191071451,
-8.16439679231297));
#18191=CARTESIAN_POINT('Ctrl Pts',(-7.07057502873392,-21.5530191071451,
-4.082198396148));
#18192=CARTESIAN_POINT('Ctrl Pts',(-9.42743337163542,-21.3780191071451,
1.69768315121407E-11));
#18193=CARTESIAN_POINT('Ctrl Pts',(-7.07057502871922,-21.2030191071451,
4.08219839617346));
#18194=CARTESIAN_POINT('Ctrl Pts',(-4.71371668580301,-21.0280191071451,
8.16439679232994));
#18195=CARTESIAN_POINT('Ctrl Pts',(1.47018674401621E-11,-20.8530191071451,
8.16439679232146));
#18196=CARTESIAN_POINT('Ctrl Pts',(4.71371668583241,-20.6780191071451,8.16439679231297));
#18197=CARTESIAN_POINT('Ctrl Pts',(7.07057502873392,-20.5030191071451,4.082198396148));
#18198=CARTESIAN_POINT('Ctrl Pts',(9.42743337163542,-20.3280191071451,-1.69756769845304E-11));
#18199=CARTESIAN_POINT('Ctrl Pts',(7.07057502871922,-20.1530191071451,-4.08219839617346));
#18200=CARTESIAN_POINT('Ctrl Pts',(4.71371668580301,-19.9780191071451,-8.16439679232994));
#18201=CARTESIAN_POINT('Ctrl Pts',(-1.4702867290402E-11,-19.8030191071451,
-8.16439679232146));
#18202=CARTESIAN_POINT('Ctrl Pts',(-4.71371668583241,-19.6280191071451,
-8.16439679231297));
#18203=CARTESIAN_POINT('Ctrl Pts',(-7.07057502873392,-19.4530191071451,
-4.082198396148));
#18204=CARTESIAN_POINT('Ctrl Pts',(-9.42743337163542,-19.2780191071451,
1.69768315121407E-11));
#18205=CARTESIAN_POINT('Ctrl Pts',(-7.07057502871922,-19.1030191071451,
4.08219839617346));
#18206=CARTESIAN_POINT('Ctrl Pts',(-4.71371668580301,-18.9280191071451,
8.16439679232994));
#18207=CARTESIAN_POINT('Ctrl Pts',(1.47018674401621E-11,-18.7530191071451,
8.16439679232146));
#18208=CARTESIAN_POINT('Ctrl Pts',(4.71371668583241,-18.5780191071451,8.16439679231297));
#18209=CARTESIAN_POINT('Ctrl Pts',(7.07057502873392,-18.4030191071451,4.082198396148));
#18210=CARTESIAN_POINT('Ctrl Pts',(9.42743337163542,-18.2280191071451,-1.69756769845304E-11));
#18211=CARTESIAN_POINT('Ctrl Pts',(7.07057502871922,-18.0530191071451,-4.08219839617346));
#18212=CARTESIAN_POINT('Ctrl Pts',(4.71371668580301,-17.8780191071451,-8.16439679232994));
#18213=CARTESIAN_POINT('Ctrl Pts',(-1.4702867290402E-11,-17.7030191071451,
-8.16439679232146));
#18214=CARTESIAN_POINT('Ctrl Pts',(-4.71371668583241,-17.5280191071451,
-8.16439679231297));
#18215=CARTESIAN_POINT('Ctrl Pts',(-7.07057502873392,-17.3530191071451,
-4.082198396148));
#18216=CARTESIAN_POINT('Ctrl Pts',(-9.42743337163542,-17.1780191071451,
1.69768315121407E-11));
#18217=CARTESIAN_POINT('Ctrl Pts',(-7.07057502871922,-17.0030191071451,
4.08219839617346));
#18218=CARTESIAN_POINT('Ctrl Pts',(-4.71371668580301,-16.8280191071451,
8.16439679232994));
#18219=CARTESIAN_POINT('Ctrl Pts',(1.47018674401621E-11,-16.6530191071451,
8.16439679232146));
#18220=CARTESIAN_POINT('Ctrl Pts',(4.71371668583241,-16.4780191071451,8.16439679231297));
#18221=CARTESIAN_POINT('Ctrl Pts',(7.07057502873392,-16.3030191071451,4.082198396148));
#18222=CARTESIAN_POINT('Ctrl Pts',(9.42743337163542,-16.1280191071451,-1.69756769845304E-11));
#18223=CARTESIAN_POINT('Ctrl Pts',(7.07057502871922,-15.9530191071451,-4.08219839617346));
#18224=CARTESIAN_POINT('Ctrl Pts',(4.71371668580301,-15.7780191071451,-8.16439679232994));
#18225=CARTESIAN_POINT('Ctrl Pts',(-1.4702867290402E-11,-15.6030191071451,
-8.16439679232146));
#18226=CARTESIAN_POINT('Ctrl Pts',(-4.71371668583241,-15.4280191071451,
-8.16439679231297));
#18227=CARTESIAN_POINT('Ctrl Pts',(-7.07057502873392,-15.2530191071451,
-4.082198396148));
#18228=CARTESIAN_POINT('Ctrl Pts',(-9.42743337163542,-15.0780191071451,
1.69768315121407E-11));
#18229=CARTESIAN_POINT('Ctrl Pts',(-7.07057502871922,-14.9030191071451,
4.08219839617346));
#18230=CARTESIAN_POINT('Ctrl Pts',(-4.71371668580301,-14.7280191071451,
8.16439679232994));
#18231=CARTESIAN_POINT('Ctrl Pts',(1.47018674401621E-11,-14.5530191071451,
8.16439679232146));
#18232=CARTESIAN_POINT('Ctrl Pts',(4.71371668583241,-14.3780191071451,8.16439679231297));
#18233=CARTESIAN_POINT('Ctrl Pts',(7.07057502873392,-14.2030191071451,4.082198396148));
#18234=CARTESIAN_POINT('Ctrl Pts',(9.42743337163542,-14.0280191071451,-1.69756769845304E-11));
#18235=CARTESIAN_POINT('Ctrl Pts',(7.07057502871922,-13.8530191071451,-4.08219839617346));
#18236=CARTESIAN_POINT('Ctrl Pts',(4.71371668580301,-13.6780191071451,-8.16439679232994));
#18237=CARTESIAN_POINT('Ctrl Pts',(-1.4702867290402E-11,-13.5030191071451,
-8.16439679232146));
#18238=CARTESIAN_POINT('Ctrl Pts',(-4.71371668583241,-13.3280191071452,
-8.16439679231297));
#18239=CARTESIAN_POINT('Ctrl Pts',(-7.07057502873392,-13.1530191071451,
-4.082198396148));
#18240=CARTESIAN_POINT('Ctrl Pts',(-9.42743337163542,-12.9780191071451,
1.69768315121407E-11));
#18241=CARTESIAN_POINT('Ctrl Pts',(-7.07057502871922,-12.8030191071452,
4.08219839617346));
#18242=CARTESIAN_POINT('Ctrl Pts',(-4.71371668580301,-12.6280191071451,
8.16439679232994));
#18243=CARTESIAN_POINT('Ctrl Pts',(1.47018674401621E-11,-12.4530191071451,
8.16439679232146));
#18244=CARTESIAN_POINT('Ctrl Pts',(4.71371668583241,-12.2780191071452,8.16439679231297));
#18245=CARTESIAN_POINT('Ctrl Pts',(7.07057502873392,-12.1030191071451,4.082198396148));
#18246=CARTESIAN_POINT('Ctrl Pts',(9.42743337163542,-11.9280191071451,-1.69756769845304E-11));
#18247=CARTESIAN_POINT('Ctrl Pts',(7.07057502871922,-11.7530191071452,-4.08219839617346));
#18248=CARTESIAN_POINT('Ctrl Pts',(4.71371668580301,-11.5780191071452,-8.16439679232994));
#18249=CARTESIAN_POINT('Ctrl Pts',(-1.4702867290402E-11,-11.4030191071451,
-8.16439679232146));
#18250=CARTESIAN_POINT('Ctrl Pts',(-4.71371668583241,-11.2280191071451,
-8.16439679231297));
#18251=CARTESIAN_POINT('Ctrl Pts',(-7.07057502873392,-11.0530191071452,
-4.082198396148));
#18252=CARTESIAN_POINT('Ctrl Pts',(-9.42743337163542,-10.8780191071451,
1.69768315121407E-11));
#18253=CARTESIAN_POINT('Ctrl Pts',(-7.07057502871922,-10.7030191071451,
4.08219839617346));
#18254=CARTESIAN_POINT('Ctrl Pts',(-4.71371668580301,-10.5280191071452,
8.16439679232994));
#18255=CARTESIAN_POINT('Ctrl Pts',(1.47018674401621E-11,-10.3530191071451,
8.16439679232146));
#18256=CARTESIAN_POINT('Ctrl Pts',(4.71371668583241,-10.1780191071451,8.16439679231297));
#18257=CARTESIAN_POINT('Ctrl Pts',(7.07057502873392,-10.0030191071452,4.082198396148));
#18258=CARTESIAN_POINT('Ctrl Pts',(9.42743337163542,-9.82801910714514,-1.69756769845304E-11));
#18259=CARTESIAN_POINT('Ctrl Pts',(7.07057502871922,-9.65301910714514,-4.08219839617346));
#18260=CARTESIAN_POINT('Ctrl Pts',(4.71371668580301,-9.47801910714516,-8.16439679232994));
#18261=CARTESIAN_POINT('Ctrl Pts',(-1.4702867290402E-11,-9.30301910714514,
-8.16439679232146));
#18262=CARTESIAN_POINT('Ctrl Pts',(-4.71371668583241,-9.12801910714515,
-8.16439679231297));
#18263=CARTESIAN_POINT('Ctrl Pts',(-7.07057502873392,-8.95301910714516,
-4.082198396148));
#18264=CARTESIAN_POINT('Ctrl Pts',(-9.42743337163542,-8.77801910714516,
1.69768315121407E-11));
#18265=CARTESIAN_POINT('Ctrl Pts',(-7.07057502871922,-8.60301910714514,
4.08219839617346));
#18266=CARTESIAN_POINT('Ctrl Pts',(-4.71371668580301,-8.42801910714516,
8.16439679232994));
#18267=CARTESIAN_POINT('Ctrl Pts',(1.47018674401621E-11,-8.25301910714516,
8.16439679232146));
#18268=CARTESIAN_POINT('Ctrl Pts',(4.71371668583241,-8.07801910714515,8.16439679231297));
#18269=CARTESIAN_POINT('Ctrl Pts',(7.07057502873392,-7.90301910714516,4.082198396148));
#18270=CARTESIAN_POINT('Ctrl Pts',(9.42743337163542,-7.72801910714516,-1.69756769845304E-11));
#18271=CARTESIAN_POINT('Ctrl Pts',(7.07057502871922,-7.55301910714514,-4.08219839617346));
#18272=CARTESIAN_POINT('Ctrl Pts',(4.71371668580301,-7.37801910714516,-8.16439679232994));
#18273=CARTESIAN_POINT('Ctrl Pts',(-1.4702867290402E-11,-7.20301910714516,
-8.16439679232146));
#18274=CARTESIAN_POINT('Ctrl Pts',(-4.71371668583241,-7.02801910714516,
-8.16439679231297));
#18275=CARTESIAN_POINT('Ctrl Pts',(-7.07057502873392,-6.85301910714514,
-4.082198396148));
#18276=CARTESIAN_POINT('Ctrl Pts',(-9.42743337163542,-6.67801910714516,
1.69768315121407E-11));
#18277=CARTESIAN_POINT('Ctrl Pts',(-7.07057502871922,-6.50301910714514,
4.08219839617346));
#18278=CARTESIAN_POINT('Ctrl Pts',(-4.71371668580301,-6.32801910714515,
8.16439679232994));
#18279=CARTESIAN_POINT('Ctrl Pts',(1.47018674401621E-11,-6.15301910714516,
8.16439679232146));
#18280=CARTESIAN_POINT('Ctrl Pts',(4.71371668583241,-5.97801910714516,8.16439679231297));
#18281=CARTESIAN_POINT('Ctrl Pts',(7.07057502873392,-5.80301910714515,4.082198396148));
#18282=CARTESIAN_POINT('Ctrl Pts',(9.42743337163542,-5.62801910714516,-1.69756769845304E-11));
#18283=CARTESIAN_POINT('Ctrl Pts',(7.07057502871922,-5.45301910714515,-4.08219839617346));
#18284=CARTESIAN_POINT('Ctrl Pts',(4.71371668580301,-5.27801910714516,-8.16439679232994));
#18285=CARTESIAN_POINT('Ctrl Pts',(-1.4702867290402E-11,-5.10301910714516,
-8.16439679232146));
#18286=CARTESIAN_POINT('Ctrl Pts',(-4.71371668583241,-4.92801910714516,
-8.16439679231297));
#18287=CARTESIAN_POINT('Ctrl Pts',(-7.07057502873392,-4.75301910714515,
-4.082198396148));
#18288=CARTESIAN_POINT('Ctrl Pts',(-9.42743337163542,-4.57801910714517,
1.69768315121407E-11));
#18289=CARTESIAN_POINT('Ctrl Pts',(-7.07057502871922,-4.40301910714516,
4.08219839617346));
#18290=CARTESIAN_POINT('Ctrl Pts',(-4.71371668580301,-4.22801910714516,
8.16439679232994));
#18291=CARTESIAN_POINT('Ctrl Pts',(1.47018674401621E-11,-4.05301910714517,
8.16439679232146));
#18292=CARTESIAN_POINT('Ctrl Pts',(4.71371668583241,-3.87801910714518,8.16439679231297));
#18293=CARTESIAN_POINT('Ctrl Pts',(7.07057502873392,-3.70301910714515,4.082198396148));
#18294=CARTESIAN_POINT('Ctrl Pts',(9.42743337163542,-3.52801910714518,-1.69756769845304E-11));
#18295=CARTESIAN_POINT('Ctrl Pts',(7.07057502871922,-3.35301910714517,-4.08219839617346));
#18296=CARTESIAN_POINT('Ctrl Pts',(4.71371668580301,-3.17801910714516,-8.16439679232994));
#18297=CARTESIAN_POINT('Ctrl Pts',(-1.4702867290402E-11,-3.00301910714517,
-8.16439679232146));
#18298=CARTESIAN_POINT('Ctrl Pts',(-4.71371668583241,-2.82801910714518,
-8.16439679231297));
#18299=CARTESIAN_POINT('Ctrl Pts',(-7.07057502873392,-2.65301910714515,
-4.082198396148));
#18300=CARTESIAN_POINT('Ctrl Pts',(-9.42743337163542,-2.47801910714516,
1.69768315121407E-11));
#18301=CARTESIAN_POINT('Ctrl Pts',(-7.07057502871922,-2.30301910714517,
4.08219839617346));
#18302=CARTESIAN_POINT('Ctrl Pts',(-4.71371668580301,-2.12801910714516,
8.16439679232994));
#18303=CARTESIAN_POINT('Ctrl Pts',(1.47018674401621E-11,-1.95301910714515,
8.16439679232146));
#18304=CARTESIAN_POINT('Ctrl Pts',(4.71371668583241,-1.77801910714518,8.16439679231297));
#18305=CARTESIAN_POINT('Ctrl Pts',(7.07057502873392,-1.60301910714516,4.082198396148));
#18306=CARTESIAN_POINT('Ctrl Pts',(9.42743337163542,-1.42801910714516,-1.69756769845304E-11));
#18307=CARTESIAN_POINT('Ctrl Pts',(7.07057502871922,-1.25301910714517,-4.08219839617346));
#18308=CARTESIAN_POINT('Ctrl Pts',(4.71371668580301,-1.07801910714517,-8.16439679232994));
#18309=CARTESIAN_POINT('Ctrl Pts',(-1.4702867290402E-11,-0.903019107145155,
-8.16439679232146));
#18310=CARTESIAN_POINT('Ctrl Pts',(-4.71371668583241,-0.728019107145183,
-8.16439679231297));
#18311=CARTESIAN_POINT('Ctrl Pts',(-7.07057502873392,-0.553019107145171,
-4.082198396148));
#18312=CARTESIAN_POINT('Ctrl Pts',(-9.42743337163542,-0.378019107145163,
1.69768315121407E-11));
#18313=CARTESIAN_POINT('Ctrl Pts',(-7.07057502871922,-0.203019107145175,
4.08219839617346));
#18314=CARTESIAN_POINT('Ctrl Pts',(-4.71371668580301,-0.0280191071451809,
8.16439679232994));
#18315=CARTESIAN_POINT('Ctrl Pts',(1.47018674401621E-11,0.146980892854842,
8.16439679232146));
#18316=CARTESIAN_POINT('Ctrl Pts',(4.71371668583241,0.321980892854814,8.16439679231297));
#18317=CARTESIAN_POINT('Ctrl Pts',(7.07057502873392,0.496980892854826,4.082198396148));
#18318=CARTESIAN_POINT('Ctrl Pts',(9.42743337163542,0.671980892854834,-1.69756769845304E-11));
#18319=CARTESIAN_POINT('Ctrl Pts',(7.07057502871922,0.846980892854822,-4.08219839617346));
#18320=CARTESIAN_POINT('Ctrl Pts',(4.71371668580301,1.02198089285482,-8.16439679232994));
#18321=CARTESIAN_POINT('Ctrl Pts',(-1.4702867290402E-11,1.19698089285484,
-8.16439679232146));
#18322=CARTESIAN_POINT('Ctrl Pts',(-4.71371668583241,1.37198089285481,-8.16439679231297));
#18323=CARTESIAN_POINT('Ctrl Pts',(-7.07057502873392,1.54698089285482,-4.082198396148));
#18324=CARTESIAN_POINT('Ctrl Pts',(-9.42743337163542,1.72198089285483,1.69768315121407E-11));
#18325=CARTESIAN_POINT('Ctrl Pts',(-7.07057502871922,1.89698089285484,4.08219839617346));
#18326=CARTESIAN_POINT('Ctrl Pts',(-4.71371668580301,2.07198089285481,8.16439679232994));
#18327=CARTESIAN_POINT('Ctrl Pts',(1.47018674401621E-11,2.24698089285484,
8.16439679232146));
#18328=CARTESIAN_POINT('Ctrl Pts',(4.71371668583241,2.42198089285483,8.16439679231297));
#18329=CARTESIAN_POINT('Ctrl Pts',(7.07057502873392,2.59698089285482,4.082198396148));
#18330=CARTESIAN_POINT('Ctrl Pts',(9.42743337163542,2.77198089285483,-1.69756769845304E-11));
#18331=CARTESIAN_POINT('Ctrl Pts',(7.07057502871922,2.94698089285484,-4.08219839617346));
#18332=CARTESIAN_POINT('Ctrl Pts',(4.71371668580301,3.12198089285481,-8.16439679232994));
#18333=CARTESIAN_POINT('Ctrl Pts',(-1.4702867290402E-11,3.29698089285482,
-8.16439679232146));
#18334=CARTESIAN_POINT('Ctrl Pts',(-4.71371668583241,3.47198089285483,-8.16439679231297));
#18335=CARTESIAN_POINT('Ctrl Pts',(-7.07057502873392,3.64698089285482,-4.082198396148));
#18336=CARTESIAN_POINT('Ctrl Pts',(-9.42743337163542,3.82198089285481,1.69768315121407E-11));
#18337=CARTESIAN_POINT('Ctrl Pts',(-7.07057502871922,3.99698089285483,4.08219839617346));
#18338=CARTESIAN_POINT('Ctrl Pts',(-4.71371668580301,4.17198089285481,8.16439679232994));
#18339=CARTESIAN_POINT('Ctrl Pts',(1.47018674401621E-11,4.34698089285482,
8.16439679232146));
#18340=CARTESIAN_POINT('Ctrl Pts',(4.71371668583241,4.52198089285483,8.16439679231297));
#18341=CARTESIAN_POINT('Ctrl Pts',(7.07057502873392,4.69698089285481,4.082198396148));
#18342=CARTESIAN_POINT('Ctrl Pts',(9.42743337163542,4.87198089285481,-1.69756769845304E-11));
#18343=CARTESIAN_POINT('Ctrl Pts',(7.07057502871922,5.04698089285483,-4.08219839617346));
#18344=CARTESIAN_POINT('Ctrl Pts',(4.71371668580301,5.22198089285481,-8.16439679232994));
#18345=CARTESIAN_POINT('Ctrl Pts',(-1.4702867290402E-11,5.39698089285482,
-8.16439679232146));
#18346=CARTESIAN_POINT('Ctrl Pts',(-4.71371668583241,5.57198089285483,-8.16439679231297));
#18347=CARTESIAN_POINT('Ctrl Pts',(-7.07057502873392,5.74698089285481,-4.082198396148));
#18348=CARTESIAN_POINT('Ctrl Pts',(-9.42743337163542,5.92198089285481,1.69768315121407E-11));
#18349=CARTESIAN_POINT('Ctrl Pts',(-7.07057502871922,6.09698089285483,4.08219839617346));
#18350=CARTESIAN_POINT('Ctrl Pts',(-4.71371668580301,6.2719808928548,8.16439679232994));
#18351=CARTESIAN_POINT('Ctrl Pts',(1.47018674401621E-11,6.44698089285481,
8.16439679232146));
#18352=CARTESIAN_POINT('Ctrl Pts',(4.71371668583241,6.62198089285482,8.16439679231297));
#18353=CARTESIAN_POINT('Ctrl Pts',(7.07057502873392,6.79698089285483,4.082198396148));
#18354=CARTESIAN_POINT('Ctrl Pts',(9.42743337163542,6.97198089285481,-1.69756769845304E-11));
#18355=CARTESIAN_POINT('Ctrl Pts',(7.07057502871922,7.14698089285482,-4.08219839617346));
#18356=CARTESIAN_POINT('Ctrl Pts',(4.71371668580301,7.32198089285482,-8.16439679232994));
#18357=CARTESIAN_POINT('Ctrl Pts',(-1.4702867290402E-11,7.49698089285481,
-8.16439679232146));
#18358=CARTESIAN_POINT('Ctrl Pts',(-4.71371668583241,7.67198089285481,-8.16439679231297));
#18359=CARTESIAN_POINT('Ctrl Pts',(-7.07057502873392,7.84698089285483,-4.082198396148));
#18360=CARTESIAN_POINT('Ctrl Pts',(-9.42743337163542,8.0219808928548,1.69768315121407E-11));
#18361=CARTESIAN_POINT('Ctrl Pts',(-7.07057502871922,8.19698089285481,4.08219839617346));
#18362=CARTESIAN_POINT('Ctrl Pts',(-4.71371668580301,8.37198089285483,8.16439679232994));
#18363=CARTESIAN_POINT('Ctrl Pts',(1.47018674401621E-11,8.54698089285481,
8.16439679232146));
#18364=CARTESIAN_POINT('Ctrl Pts',(4.71371668583241,8.72198089285481,8.16439679231297));
#18365=CARTESIAN_POINT('Ctrl Pts',(7.07057502873392,8.89698089285482,4.082198396148));
#18366=CARTESIAN_POINT('Ctrl Pts',(9.42743337163542,9.0719808928548,-1.69756769845304E-11));
#18367=CARTESIAN_POINT('Ctrl Pts',(7.07057502871922,9.24698089285481,-4.08219839617346));
#18368=CARTESIAN_POINT('Ctrl Pts',(4.71371668580301,9.42198089285482,-8.16439679232994));
#18369=CARTESIAN_POINT('Ctrl Pts',(-1.4702867290402E-11,9.5969808928548,
-8.16439679232146));
#18370=CARTESIAN_POINT('Ctrl Pts',(-4.71371668583241,9.7719808928548,-8.16439679231297));
#18371=CARTESIAN_POINT('Ctrl Pts',(-7.07057502873392,9.94698089285482,-4.082198396148));
#18372=CARTESIAN_POINT('Ctrl Pts',(-9.42743337163542,10.1219808928548,1.69768315121407E-11));
#18373=CARTESIAN_POINT('Ctrl Pts',(-7.07057502871922,10.2969808928548,4.08219839617346));
#18374=CARTESIAN_POINT('Ctrl Pts',(-4.71371668580301,10.4719808928548,8.16439679232994));
#18375=CARTESIAN_POINT('Ctrl Pts',(1.47018674401621E-11,10.6469808928548,
8.16439679232146));
#18376=CARTESIAN_POINT('Ctrl Pts',(4.71371668583241,10.8219808928548,8.16439679231297));
#18377=CARTESIAN_POINT('Ctrl Pts',(7.07057502873392,10.9969808928548,4.082198396148));
#18378=CARTESIAN_POINT('Ctrl Pts',(9.42743337163542,11.1719808928548,-1.69756769845304E-11));
#18379=CARTESIAN_POINT('Ctrl Pts',(7.07057502871922,11.3469808928548,-4.08219839617346));
#18380=CARTESIAN_POINT('Ctrl Pts',(4.71371668580301,11.5219808928548,-8.16439679232994));
#18381=CARTESIAN_POINT('Ctrl Pts',(-1.4702867290402E-11,11.6969808928548,
-8.16439679232146));
#18382=CARTESIAN_POINT('Ctrl Pts',(-4.71371668583241,11.8719808928548,-8.16439679231297));
#18383=CARTESIAN_POINT('Ctrl Pts',(-7.07057502873392,12.0469808928548,-4.082198396148));
#18384=CARTESIAN_POINT('Ctrl Pts',(-9.42743337163542,12.2219808928548,1.69768315121407E-11));
#18385=CARTESIAN_POINT('Ctrl Pts',(-7.07057502871922,12.3969808928548,4.08219839617346));
#18386=CARTESIAN_POINT('Ctrl Pts',(-4.71371668580301,12.5719808928548,8.16439679232994));
#18387=CARTESIAN_POINT('Ctrl Pts',(1.47018674401621E-11,12.7469808928548,
8.16439679232146));
#18388=CARTESIAN_POINT('Ctrl Pts',(4.71371668583241,12.9219808928548,8.16439679231297));
#18389=CARTESIAN_POINT('Ctrl Pts',(7.07057502873392,13.0969808928548,4.082198396148));
#18390=CARTESIAN_POINT('Ctrl Pts',(9.42743337163542,13.2719808928548,-1.69756769845304E-11));
#18391=CARTESIAN_POINT('Ctrl Pts',(7.07057502871922,13.4469808928548,-4.08219839617346));
#18392=CARTESIAN_POINT('Ctrl Pts',(4.71371668580301,13.6219808928548,-8.16439679232994));
#18393=CARTESIAN_POINT('Ctrl Pts',(-1.4702867290402E-11,13.7969808928548,
-8.16439679232146));
#18394=CARTESIAN_POINT('Ctrl Pts',(-4.71371668583241,13.9719808928548,-8.16439679231297));
#18395=CARTESIAN_POINT('Ctrl Pts',(-7.07057502873392,14.1469808928548,-4.082198396148));
#18396=CARTESIAN_POINT('Ctrl Pts',(-9.42743337163542,14.3219808928548,1.69768315121407E-11));
#18397=CARTESIAN_POINT('Ctrl Pts',(-7.07057502871922,14.4969808928548,4.08219839617346));
#18398=CARTESIAN_POINT('Ctrl Pts',(-4.71371668580301,14.6719808928548,8.16439679232994));
#18399=CARTESIAN_POINT('Ctrl Pts',(1.47018674401621E-11,14.8469808928548,
8.16439679232146));
#18400=CARTESIAN_POINT('Ctrl Pts',(4.71371668583241,15.0219808928548,8.16439679231297));
#18401=CARTESIAN_POINT('Ctrl Pts',(7.07057502873392,15.1969808928548,4.082198396148));
#18402=CARTESIAN_POINT('Ctrl Pts',(9.42743337163542,15.3719808928548,-1.69756769845304E-11));
#18403=CARTESIAN_POINT('Ctrl Pts',(7.07057502871922,15.5469808928548,-4.08219839617346));
#18404=CARTESIAN_POINT('Ctrl Pts',(4.71371668580301,15.7219808928548,-8.16439679232994));
#18405=CARTESIAN_POINT('Ctrl Pts',(-1.4702867290402E-11,15.8969808928548,
-8.16439679232146));
#18406=CARTESIAN_POINT('Ctrl Pts',(-4.71371668583241,16.0719808928548,-8.16439679231297));
#18407=CARTESIAN_POINT('Ctrl Pts',(-7.07057502873392,16.2469808928548,-4.082198396148));
#18408=CARTESIAN_POINT('Ctrl Pts',(-9.42743337163542,16.4219808928548,1.69768315121407E-11));
#18409=CARTESIAN_POINT('Ctrl Pts',(-7.07057502871922,16.5969808928548,4.08219839617346));
#18410=CARTESIAN_POINT('Ctrl Pts',(-4.71371668580301,16.7719808928548,8.16439679232994));
#18411=CARTESIAN_POINT('Ctrl Pts',(1.47018674401621E-11,16.9469808928548,
8.16439679232146));
#18412=CARTESIAN_POINT('Ctrl Pts',(4.71371668583241,17.1219808928548,8.16439679231297));
#18413=CARTESIAN_POINT('Ctrl Pts',(7.07057502873392,17.2969808928548,4.082198396148));
#18414=CARTESIAN_POINT('Ctrl Pts',(9.42743337163542,17.4719808928548,-1.69756769845304E-11));
#18415=CARTESIAN_POINT('Ctrl Pts',(7.07057502871922,17.6469808928548,-4.08219839617346));
#18416=CARTESIAN_POINT('Ctrl Pts',(4.71371668580301,17.8219808928548,-8.16439679232994));
#18417=CARTESIAN_POINT('Ctrl Pts',(-1.4702867290402E-11,17.9969808928548,
-8.16439679232146));
#18418=CARTESIAN_POINT('Ctrl Pts',(-4.71371668583241,18.1719808928548,-8.16439679231297));
#18419=CARTESIAN_POINT('Ctrl Pts',(-7.07057502873392,18.3469808928548,-4.082198396148));
#18420=CARTESIAN_POINT('Ctrl Pts',(-9.42743337163542,18.5219808928548,1.69768315121407E-11));
#18421=CARTESIAN_POINT('Ctrl Pts',(-7.07057502871922,18.6969808928548,4.08219839617346));
#18422=CARTESIAN_POINT('Ctrl Pts',(-4.71371668580301,18.8719808928548,8.16439679232994));
#18423=CARTESIAN_POINT('Ctrl Pts',(1.47018674401621E-11,19.0469808928548,
8.16439679232146));
#18424=CARTESIAN_POINT('Ctrl Pts',(4.71371668583241,19.2219808928548,8.16439679231297));
#18425=CARTESIAN_POINT('Ctrl Pts',(7.07057502873392,19.3969808928548,4.082198396148));
#18426=CARTESIAN_POINT('Ctrl Pts',(9.42743337163542,19.5719808928548,-1.69756769845304E-11));
#18427=CARTESIAN_POINT('Ctrl Pts',(7.07057502871922,19.7469808928548,-4.08219839617346));
#18428=CARTESIAN_POINT('Ctrl Pts',(4.71371668580301,19.9219808928548,-8.16439679232994));
#18429=CARTESIAN_POINT('Ctrl Pts',(-1.4702867290402E-11,20.0969808928548,
-8.16439679232146));
#18430=CARTESIAN_POINT('Ctrl Pts',(-4.71371668583241,20.2719808928548,-8.16439679231297));
#18431=CARTESIAN_POINT('Ctrl Pts',(-7.07057502873392,20.4469808928548,-4.082198396148));
#18432=CARTESIAN_POINT('Ctrl Pts',(-9.42743337163542,20.6219808928548,1.69768315121407E-11));
#18433=CARTESIAN_POINT('Ctrl Pts',(-7.07057502871922,20.7969808928548,4.08219839617346));
#18434=CARTESIAN_POINT('Ctrl Pts',(-4.71371668580301,20.9719808928548,8.16439679232994));
#18435=CARTESIAN_POINT('Ctrl Pts',(1.47018674401621E-11,21.1469808928548,
8.16439679232146));
#18436=CARTESIAN_POINT('Ctrl Pts',(4.71371668583241,21.3219808928548,8.16439679231297));
#18437=CARTESIAN_POINT('Ctrl Pts',(7.07057502873392,21.4969808928548,4.082198396148));
#18438=CARTESIAN_POINT('Ctrl Pts',(9.42743337163542,21.6719808928548,-1.69756769845304E-11));
#18439=CARTESIAN_POINT('Ctrl Pts',(7.07057502871922,21.8469808928548,-4.08219839617346));
#18440=CARTESIAN_POINT('Ctrl Pts',(4.71371668580301,22.0219808928548,-8.16439679232994));
#18441=CARTESIAN_POINT('Ctrl Pts',(-1.4702867290402E-11,22.1969808928548,
-8.16439679232146));
#18442=CARTESIAN_POINT('Ctrl Pts',(-4.71371668583241,22.3719808928548,-8.16439679231297));
#18443=CARTESIAN_POINT('Ctrl Pts',(-7.07057502873392,22.5469808928548,-4.082198396148));
#18444=CARTESIAN_POINT('Ctrl Pts',(-9.42743337163542,22.7219808928548,1.69768315121407E-11));
#18445=CARTESIAN_POINT('Ctrl Pts',(-7.07057502871922,22.8969808928548,4.08219839617346));
#18446=CARTESIAN_POINT('Ctrl Pts',(-4.71371668580301,23.0719808928548,8.16439679232994));
#18447=CARTESIAN_POINT('Ctrl Pts',(1.47018674401621E-11,23.2469808928548,
8.16439679232146));
#18448=CARTESIAN_POINT('Ctrl Pts',(4.71371668583241,23.4219808928548,8.16439679231297));
#18449=CARTESIAN_POINT('Ctrl Pts',(7.07057502873392,23.5969808928548,4.082198396148));
#18450=CARTESIAN_POINT('Ctrl Pts',(9.42743337163542,23.7719808928548,-1.69756769845304E-11));
#18451=CARTESIAN_POINT('Ctrl Pts',(7.07057502871922,23.9469808928548,-4.08219839617346));
#18452=CARTESIAN_POINT('Ctrl Pts',(4.71371668580301,24.1219808928548,-8.16439679232994));
#18453=CARTESIAN_POINT('Ctrl Pts',(-1.4702867290402E-11,24.2969808928548,
-8.16439679232146));
#18454=CARTESIAN_POINT('Ctrl Pts',(-4.71371668583241,24.4719808928548,-8.16439679231297));
#18455=CARTESIAN_POINT('Ctrl Pts',(-7.07057502873392,24.6469808928548,-4.082198396148));
#18456=CARTESIAN_POINT('Ctrl Pts',(-9.42743337163542,24.8219808928548,1.69768315121407E-11));
#18457=CARTESIAN_POINT('Ctrl Pts',(-7.07057502871922,24.9969808928548,4.08219839617346));
#18458=CARTESIAN_POINT('Ctrl Pts',(-4.71371668580301,25.1719808928548,8.16439679232994));
#18459=CARTESIAN_POINT('Ctrl Pts',(1.47018674401621E-11,25.3469808928548,
8.16439679232146));
#18460=CARTESIAN_POINT('Ctrl Pts',(4.71371668583241,25.5219808928548,8.16439679231297));
#18461=CARTESIAN_POINT('Ctrl Pts',(7.07057502873392,25.6969808928548,4.082198396148));
#18462=CARTESIAN_POINT('Ctrl Pts',(9.42743337163542,25.8719808928548,-1.69756769845304E-11));
#18463=CARTESIAN_POINT('Ctrl Pts',(7.07057502871922,26.0469808928548,-4.08219839617346));
#18464=CARTESIAN_POINT('Ctrl Pts',(4.71371668580301,26.2219808928548,-8.16439679232994));
#18465=CARTESIAN_POINT('Ctrl Pts',(-1.4702867290402E-11,26.3969808928548,
-8.16439679232146));
#18466=CARTESIAN_POINT('Ctrl Pts',(-1.51301075899711E-11,-143.579517970998,
-8.40164026751963));
#18467=CARTESIAN_POINT('Ctrl Pts',(-4.85068927010199,-143.404517970998,
-8.4016402675109));
#18468=CARTESIAN_POINT('Ctrl Pts',(-7.27603390513785,-143.229517970998,
-4.20082013374671));
#18469=CARTESIAN_POINT('Ctrl Pts',(-9.70137854017372,-143.054517970998,
1.74701493417668E-11));
#18470=CARTESIAN_POINT('Ctrl Pts',(-7.27603390512272,-142.879517970998,
4.20082013377292));
#18471=CARTESIAN_POINT('Ctrl Pts',(-4.85068927007173,-142.704517970998,
8.40164026752836));
#18472=CARTESIAN_POINT('Ctrl Pts',(1.5129078685785E-11,-142.529517970998,
8.40164026751963));
#18473=CARTESIAN_POINT('Ctrl Pts',(4.85068927010198,-142.354517970998,8.4016402675109));
#18474=CARTESIAN_POINT('Ctrl Pts',(7.27603390513785,-142.179517970998,4.20082013374672));
#18475=CARTESIAN_POINT('Ctrl Pts',(9.70137854017372,-142.004517970998,-1.74689612655491E-11));
#18476=CARTESIAN_POINT('Ctrl Pts',(7.27603390512273,-141.829517970998,-4.20082013377291));
#18477=CARTESIAN_POINT('Ctrl Pts',(4.85068927007173,-141.654517970998,-8.40164026752836));
#18478=CARTESIAN_POINT('Ctrl Pts',(-1.51301075899711E-11,-141.479517970998,
-8.40164026751963));
#18479=CARTESIAN_POINT('Ctrl Pts',(-4.85068927010199,-141.304517970998,
-8.4016402675109));
#18480=CARTESIAN_POINT('Ctrl Pts',(-7.27603390513785,-141.129517970998,
-4.20082013374671));
#18481=CARTESIAN_POINT('Ctrl Pts',(-9.70137854017372,-140.954517970998,
1.74701493417668E-11));
#18482=CARTESIAN_POINT('Ctrl Pts',(-7.27603390512272,-140.779517970998,
4.20082013377292));
#18483=CARTESIAN_POINT('Ctrl Pts',(-4.85068927007173,-140.604517970998,
8.40164026752836));
#18484=CARTESIAN_POINT('Ctrl Pts',(1.5129078685785E-11,-140.429517970998,
8.40164026751963));
#18485=CARTESIAN_POINT('Ctrl Pts',(4.85068927010198,-140.254517970998,8.4016402675109));
#18486=CARTESIAN_POINT('Ctrl Pts',(7.27603390513785,-140.079517970998,4.20082013374672));
#18487=CARTESIAN_POINT('Ctrl Pts',(9.70137854017372,-139.904517970998,-1.74689612655491E-11));
#18488=CARTESIAN_POINT('Ctrl Pts',(7.27603390512273,-139.729517970998,-4.20082013377291));
#18489=CARTESIAN_POINT('Ctrl Pts',(4.85068927007173,-139.554517970998,-8.40164026752836));
#18490=CARTESIAN_POINT('Ctrl Pts',(-1.51301075899711E-11,-139.379517970998,
-8.40164026751963));
#18491=CARTESIAN_POINT('Ctrl Pts',(-4.85068927010199,-139.204517970998,
-8.4016402675109));
#18492=CARTESIAN_POINT('Ctrl Pts',(-7.27603390513785,-139.029517970998,
-4.20082013374671));
#18493=CARTESIAN_POINT('Ctrl Pts',(-9.70137854017372,-138.854517970998,
1.74701493417668E-11));
#18494=CARTESIAN_POINT('Ctrl Pts',(-7.27603390512272,-138.679517970998,
4.20082013377292));
#18495=CARTESIAN_POINT('Ctrl Pts',(-4.85068927007173,-138.504517970998,
8.40164026752836));
#18496=CARTESIAN_POINT('Ctrl Pts',(1.5129078685785E-11,-138.329517970998,
8.40164026751963));
#18497=CARTESIAN_POINT('Ctrl Pts',(4.85068927010198,-138.154517970998,8.4016402675109));
#18498=CARTESIAN_POINT('Ctrl Pts',(7.27603390513785,-137.979517970998,4.20082013374672));
#18499=CARTESIAN_POINT('Ctrl Pts',(9.70137854017372,-137.804517970998,-1.74689612655491E-11));
#18500=CARTESIAN_POINT('Ctrl Pts',(7.27603390512273,-137.629517970998,-4.20082013377291));
#18501=CARTESIAN_POINT('Ctrl Pts',(4.85068927007173,-137.454517970998,-8.40164026752836));
#18502=CARTESIAN_POINT('Ctrl Pts',(-1.51301075899711E-11,-137.279517970998,
-8.40164026751963));
#18503=CARTESIAN_POINT('Ctrl Pts',(-4.85068927010199,-137.104517970998,
-8.4016402675109));
#18504=CARTESIAN_POINT('Ctrl Pts',(-7.27603390513785,-136.929517970998,
-4.20082013374671));
#18505=CARTESIAN_POINT('Ctrl Pts',(-9.70137854017372,-136.754517970998,
1.74701493417668E-11));
#18506=CARTESIAN_POINT('Ctrl Pts',(-7.27603390512272,-136.579517970998,
4.20082013377292));
#18507=CARTESIAN_POINT('Ctrl Pts',(-4.85068927007173,-136.404517970998,
8.40164026752836));
#18508=CARTESIAN_POINT('Ctrl Pts',(1.5129078685785E-11,-136.229517970998,
8.40164026751963));
#18509=CARTESIAN_POINT('Ctrl Pts',(4.85068927010198,-136.054517970998,8.4016402675109));
#18510=CARTESIAN_POINT('Ctrl Pts',(7.27603390513785,-135.879517970998,4.20082013374672));
#18511=CARTESIAN_POINT('Ctrl Pts',(9.70137854017372,-135.704517970998,-1.74689612655491E-11));
#18512=CARTESIAN_POINT('Ctrl Pts',(7.27603390512273,-135.529517970998,-4.20082013377291));
#18513=CARTESIAN_POINT('Ctrl Pts',(4.85068927007173,-135.354517970998,-8.40164026752836));
#18514=CARTESIAN_POINT('Ctrl Pts',(-1.51301075899711E-11,-135.179517970998,
-8.40164026751963));
#18515=CARTESIAN_POINT('Ctrl Pts',(-4.85068927010199,-135.004517970998,
-8.4016402675109));
#18516=CARTESIAN_POINT('Ctrl Pts',(-7.27603390513785,-134.829517970998,
-4.20082013374671));
#18517=CARTESIAN_POINT('Ctrl Pts',(-9.70137854017372,-134.654517970998,
1.74701493417668E-11));
#18518=CARTESIAN_POINT('Ctrl Pts',(-7.27603390512272,-134.479517970998,
4.20082013377292));
#18519=CARTESIAN_POINT('Ctrl Pts',(-4.85068927007173,-134.304517970998,
8.40164026752836));
#18520=CARTESIAN_POINT('Ctrl Pts',(1.5129078685785E-11,-134.129517970998,
8.40164026751963));
#18521=CARTESIAN_POINT('Ctrl Pts',(4.85068927010198,-133.954517970998,8.4016402675109));
#18522=CARTESIAN_POINT('Ctrl Pts',(7.27603390513785,-133.779517970998,4.20082013374672));
#18523=CARTESIAN_POINT('Ctrl Pts',(9.70137854017372,-133.604517970998,-1.74689612655491E-11));
#18524=CARTESIAN_POINT('Ctrl Pts',(7.27603390512273,-133.429517970998,-4.20082013377291));
#18525=CARTESIAN_POINT('Ctrl Pts',(4.85068927007173,-133.254517970998,-8.40164026752836));
#18526=CARTESIAN_POINT('Ctrl Pts',(-1.51301075899711E-11,-133.079517970998,
-8.40164026751963));
#18527=CARTESIAN_POINT('Ctrl Pts',(-4.85068927010199,-132.904517970998,
-8.4016402675109));
#18528=CARTESIAN_POINT('Ctrl Pts',(-7.27603390513785,-132.729517970998,
-4.20082013374671));
#18529=CARTESIAN_POINT('Ctrl Pts',(-9.70137854017372,-132.554517970998,
1.74701493417668E-11));
#18530=CARTESIAN_POINT('Ctrl Pts',(-7.27603390512272,-132.379517970998,
4.20082013377292));
#18531=CARTESIAN_POINT('Ctrl Pts',(-4.85068927007173,-132.204517970998,
8.40164026752836));
#18532=CARTESIAN_POINT('Ctrl Pts',(1.5129078685785E-11,-132.029517970998,
8.40164026751963));
#18533=CARTESIAN_POINT('Ctrl Pts',(4.85068927010198,-131.854517970998,8.4016402675109));
#18534=CARTESIAN_POINT('Ctrl Pts',(7.27603390513785,-131.679517970998,4.20082013374672));
#18535=CARTESIAN_POINT('Ctrl Pts',(9.70137854017372,-131.504517970998,-1.74689612655491E-11));
#18536=CARTESIAN_POINT('Ctrl Pts',(7.27603390512273,-131.329517970998,-4.20082013377291));
#18537=CARTESIAN_POINT('Ctrl Pts',(4.85068927007173,-131.154517970998,-8.40164026752836));
#18538=CARTESIAN_POINT('Ctrl Pts',(-1.51301075899711E-11,-130.979517970998,
-8.40164026751963));
#18539=CARTESIAN_POINT('Ctrl Pts',(-4.85068927010199,-130.804517970998,
-8.4016402675109));
#18540=CARTESIAN_POINT('Ctrl Pts',(-7.27603390513785,-130.629517970998,
-4.20082013374671));
#18541=CARTESIAN_POINT('Ctrl Pts',(-9.70137854017372,-130.454517970998,
1.74701493417668E-11));
#18542=CARTESIAN_POINT('Ctrl Pts',(-7.27603390512272,-130.279517970998,
4.20082013377292));
#18543=CARTESIAN_POINT('Ctrl Pts',(-4.85068927007173,-130.104517970998,
8.40164026752836));
#18544=CARTESIAN_POINT('Ctrl Pts',(1.5129078685785E-11,-129.929517970998,
8.40164026751963));
#18545=CARTESIAN_POINT('Ctrl Pts',(4.85068927010198,-129.754517970998,8.4016402675109));
#18546=CARTESIAN_POINT('Ctrl Pts',(7.27603390513785,-129.579517970998,4.20082013374672));
#18547=CARTESIAN_POINT('Ctrl Pts',(9.70137854017372,-129.404517970998,-1.74689612655491E-11));
#18548=CARTESIAN_POINT('Ctrl Pts',(7.27603390512273,-129.229517970998,-4.20082013377291));
#18549=CARTESIAN_POINT('Ctrl Pts',(4.85068927007173,-129.054517970998,-8.40164026752836));
#18550=CARTESIAN_POINT('Ctrl Pts',(-1.51301075899711E-11,-128.879517970998,
-8.40164026751963));
#18551=CARTESIAN_POINT('Ctrl Pts',(-4.85068927010199,-128.704517970998,
-8.4016402675109));
#18552=CARTESIAN_POINT('Ctrl Pts',(-7.27603390513785,-128.529517970998,
-4.20082013374671));
#18553=CARTESIAN_POINT('Ctrl Pts',(-9.70137854017372,-128.354517970998,
1.74701493417668E-11));
#18554=CARTESIAN_POINT('Ctrl Pts',(-7.27603390512272,-128.179517970998,
4.20082013377292));
#18555=CARTESIAN_POINT('Ctrl Pts',(-4.85068927007173,-128.004517970998,
8.40164026752836));
#18556=CARTESIAN_POINT('Ctrl Pts',(1.5129078685785E-11,-127.829517970998,
8.40164026751963));
#18557=CARTESIAN_POINT('Ctrl Pts',(4.85068927010198,-127.654517970998,8.4016402675109));
#18558=CARTESIAN_POINT('Ctrl Pts',(7.27603390513785,-127.479517970998,4.20082013374672));
#18559=CARTESIAN_POINT('Ctrl Pts',(9.70137854017372,-127.304517970998,-1.74689612655491E-11));
#18560=CARTESIAN_POINT('Ctrl Pts',(7.27603390512273,-127.129517970998,-4.20082013377291));
#18561=CARTESIAN_POINT('Ctrl Pts',(4.85068927007173,-126.954517970998,-8.40164026752836));
#18562=CARTESIAN_POINT('Ctrl Pts',(-1.51301075899711E-11,-126.779517970998,
-8.40164026751963));
#18563=CARTESIAN_POINT('Ctrl Pts',(-4.85068927010199,-126.604517970998,
-8.4016402675109));
#18564=CARTESIAN_POINT('Ctrl Pts',(-7.27603390513785,-126.429517970998,
-4.20082013374671));
#18565=CARTESIAN_POINT('Ctrl Pts',(-9.70137854017372,-126.254517970998,
1.74701493417668E-11));
#18566=CARTESIAN_POINT('Ctrl Pts',(-7.27603390512272,-126.079517970998,
4.20082013377292));
#18567=CARTESIAN_POINT('Ctrl Pts',(-4.85068927007173,-125.904517970998,
8.40164026752836));
#18568=CARTESIAN_POINT('Ctrl Pts',(1.5129078685785E-11,-125.729517970998,
8.40164026751963));
#18569=CARTESIAN_POINT('Ctrl Pts',(4.85068927010198,-125.554517970998,8.4016402675109));
#18570=CARTESIAN_POINT('Ctrl Pts',(7.27603390513785,-125.379517970998,4.20082013374672));
#18571=CARTESIAN_POINT('Ctrl Pts',(9.70137854017372,-125.204517970998,-1.74689612655491E-11));
#18572=CARTESIAN_POINT('Ctrl Pts',(7.27603390512273,-125.029517970998,-4.20082013377291));
#18573=CARTESIAN_POINT('Ctrl Pts',(4.85068927007173,-124.854517970998,-8.40164026752836));
#18574=CARTESIAN_POINT('Ctrl Pts',(-1.51301075899711E-11,-124.679517970998,
-8.40164026751963));
#18575=CARTESIAN_POINT('Ctrl Pts',(-4.85068927010199,-124.504517970998,
-8.4016402675109));
#18576=CARTESIAN_POINT('Ctrl Pts',(-7.27603390513785,-124.329517970998,
-4.20082013374671));
#18577=CARTESIAN_POINT('Ctrl Pts',(-9.70137854017372,-124.154517970998,
1.74701493417668E-11));
#18578=CARTESIAN_POINT('Ctrl Pts',(-7.27603390512272,-123.979517970998,
4.20082013377292));
#18579=CARTESIAN_POINT('Ctrl Pts',(-4.85068927007173,-123.804517970998,
8.40164026752836));
#18580=CARTESIAN_POINT('Ctrl Pts',(1.5129078685785E-11,-123.629517970998,
8.40164026751963));
#18581=CARTESIAN_POINT('Ctrl Pts',(4.85068927010198,-123.454517970998,8.4016402675109));
#18582=CARTESIAN_POINT('Ctrl Pts',(7.27603390513785,-123.279517970998,4.20082013374672));
#18583=CARTESIAN_POINT('Ctrl Pts',(9.70137854017372,-123.104517970998,-1.74689612655491E-11));
#18584=CARTESIAN_POINT('Ctrl Pts',(7.27603390512273,-122.929517970998,-4.20082013377291));
#18585=CARTESIAN_POINT('Ctrl Pts',(4.85068927007173,-122.754517970998,-8.40164026752836));
#18586=CARTESIAN_POINT('Ctrl Pts',(-1.51301075899711E-11,-122.579517970998,
-8.40164026751963));
#18587=CARTESIAN_POINT('Ctrl Pts',(-4.85068927010199,-122.404517970998,
-8.4016402675109));
#18588=CARTESIAN_POINT('Ctrl Pts',(-7.27603390513785,-122.229517970998,
-4.20082013374671));
#18589=CARTESIAN_POINT('Ctrl Pts',(-9.70137854017372,-122.054517970998,
1.74701493417668E-11));
#18590=CARTESIAN_POINT('Ctrl Pts',(-7.27603390512272,-121.879517970998,
4.20082013377292));
#18591=CARTESIAN_POINT('Ctrl Pts',(-4.85068927007173,-121.704517970998,
8.40164026752836));
#18592=CARTESIAN_POINT('Ctrl Pts',(1.5129078685785E-11,-121.529517970998,
8.40164026751963));
#18593=CARTESIAN_POINT('Ctrl Pts',(4.85068927010198,-121.354517970998,8.4016402675109));
#18594=CARTESIAN_POINT('Ctrl Pts',(7.27603390513785,-121.179517970998,4.20082013374672));
#18595=CARTESIAN_POINT('Ctrl Pts',(9.70137854017372,-121.004517970998,-1.74689612655491E-11));
#18596=CARTESIAN_POINT('Ctrl Pts',(7.27603390512273,-120.829517970998,-4.20082013377291));
#18597=CARTESIAN_POINT('Ctrl Pts',(4.85068927007173,-120.654517970998,-8.40164026752836));
#18598=CARTESIAN_POINT('Ctrl Pts',(-1.51301075899711E-11,-120.479517970998,
-8.40164026751963));
#18599=CARTESIAN_POINT('Ctrl Pts',(-4.85068927010199,-120.304517970998,
-8.4016402675109));
#18600=CARTESIAN_POINT('Ctrl Pts',(-7.27603390513785,-120.129517970998,
-4.20082013374671));
#18601=CARTESIAN_POINT('Ctrl Pts',(-9.70137854017372,-119.954517970998,
1.74701493417668E-11));
#18602=CARTESIAN_POINT('Ctrl Pts',(-7.27603390512272,-119.779517970998,
4.20082013377292));
#18603=CARTESIAN_POINT('Ctrl Pts',(-4.85068927007173,-119.604517970998,
8.40164026752836));
#18604=CARTESIAN_POINT('Ctrl Pts',(1.5129078685785E-11,-119.429517970998,
8.40164026751963));
#18605=CARTESIAN_POINT('Ctrl Pts',(4.85068927010198,-119.254517970998,8.4016402675109));
#18606=CARTESIAN_POINT('Ctrl Pts',(7.27603390513785,-119.079517970998,4.20082013374672));
#18607=CARTESIAN_POINT('Ctrl Pts',(9.70137854017372,-118.904517970998,-1.74689612655491E-11));
#18608=CARTESIAN_POINT('Ctrl Pts',(7.27603390512273,-118.729517970998,-4.20082013377291));
#18609=CARTESIAN_POINT('Ctrl Pts',(4.85068927007173,-118.554517970998,-8.40164026752836));
#18610=CARTESIAN_POINT('Ctrl Pts',(-1.51301075899711E-11,-118.379517970998,
-8.40164026751963));
#18611=CARTESIAN_POINT('Ctrl Pts',(-4.85068927010199,-118.204517970998,
-8.4016402675109));
#18612=CARTESIAN_POINT('Ctrl Pts',(-7.27603390513785,-118.029517970998,
-4.20082013374671));
#18613=CARTESIAN_POINT('Ctrl Pts',(-9.70137854017372,-117.854517970998,
1.74701493417668E-11));
#18614=CARTESIAN_POINT('Ctrl Pts',(-7.27603390512272,-117.679517970998,
4.20082013377292));
#18615=CARTESIAN_POINT('Ctrl Pts',(-4.85068927007173,-117.504517970998,
8.40164026752836));
#18616=CARTESIAN_POINT('Ctrl Pts',(1.5129078685785E-11,-117.329517970998,
8.40164026751963));
#18617=CARTESIAN_POINT('Ctrl Pts',(4.85068927010198,-117.154517970998,8.4016402675109));
#18618=CARTESIAN_POINT('Ctrl Pts',(7.27603390513785,-116.979517970998,4.20082013374672));
#18619=CARTESIAN_POINT('Ctrl Pts',(9.70137854017372,-116.804517970998,-1.74689612655491E-11));
#18620=CARTESIAN_POINT('Ctrl Pts',(7.27603390512273,-116.629517970998,-4.20082013377291));
#18621=CARTESIAN_POINT('Ctrl Pts',(4.85068927007173,-116.454517970998,-8.40164026752836));
#18622=CARTESIAN_POINT('Ctrl Pts',(-1.51301075899711E-11,-116.279517970998,
-8.40164026751963));
#18623=CARTESIAN_POINT('Ctrl Pts',(-4.85068927010199,-116.104517970998,
-8.4016402675109));
#18624=CARTESIAN_POINT('Ctrl Pts',(-7.27603390513785,-115.929517970998,
-4.20082013374671));
#18625=CARTESIAN_POINT('Ctrl Pts',(-9.70137854017372,-115.754517970998,
1.74701493417668E-11));
#18626=CARTESIAN_POINT('Ctrl Pts',(-7.27603390512272,-115.579517970998,
4.20082013377292));
#18627=CARTESIAN_POINT('Ctrl Pts',(-4.85068927007173,-115.404517970998,
8.40164026752836));
#18628=CARTESIAN_POINT('Ctrl Pts',(1.5129078685785E-11,-115.229517970998,
8.40164026751963));
#18629=CARTESIAN_POINT('Ctrl Pts',(4.85068927010198,-115.054517970998,8.4016402675109));
#18630=CARTESIAN_POINT('Ctrl Pts',(7.27603390513785,-114.879517970998,4.20082013374672));
#18631=CARTESIAN_POINT('Ctrl Pts',(9.70137854017372,-114.704517970998,-1.74689612655491E-11));
#18632=CARTESIAN_POINT('Ctrl Pts',(7.27603390512273,-114.529517970998,-4.20082013377291));
#18633=CARTESIAN_POINT('Ctrl Pts',(4.85068927007173,-114.354517970998,-8.40164026752836));
#18634=CARTESIAN_POINT('Ctrl Pts',(-1.51301075899711E-11,-114.179517970998,
-8.40164026751963));
#18635=CARTESIAN_POINT('Ctrl Pts',(-4.85068927010199,-114.004517970998,
-8.4016402675109));
#18636=CARTESIAN_POINT('Ctrl Pts',(-7.27603390513785,-113.829517970998,
-4.20082013374671));
#18637=CARTESIAN_POINT('Ctrl Pts',(-9.70137854017372,-113.654517970998,
1.74701493417668E-11));
#18638=CARTESIAN_POINT('Ctrl Pts',(-7.27603390512272,-113.479517970998,
4.20082013377292));
#18639=CARTESIAN_POINT('Ctrl Pts',(-4.85068927007173,-113.304517970998,
8.40164026752836));
#18640=CARTESIAN_POINT('Ctrl Pts',(1.5129078685785E-11,-113.129517970998,
8.40164026751963));
#18641=CARTESIAN_POINT('Ctrl Pts',(4.85068927010198,-112.954517970998,8.4016402675109));
#18642=CARTESIAN_POINT('Ctrl Pts',(7.27603390513785,-112.779517970998,4.20082013374672));
#18643=CARTESIAN_POINT('Ctrl Pts',(9.70137854017372,-112.604517970998,-1.74689612655491E-11));
#18644=CARTESIAN_POINT('Ctrl Pts',(7.27603390512273,-112.429517970998,-4.20082013377291));
#18645=CARTESIAN_POINT('Ctrl Pts',(4.85068927007173,-112.254517970998,-8.40164026752836));
#18646=CARTESIAN_POINT('Ctrl Pts',(-1.51301075899711E-11,-112.079517970998,
-8.40164026751963));
#18647=CARTESIAN_POINT('Ctrl Pts',(-4.85068927010199,-111.904517970998,
-8.4016402675109));
#18648=CARTESIAN_POINT('Ctrl Pts',(-7.27603390513785,-111.729517970998,
-4.20082013374671));
#18649=CARTESIAN_POINT('Ctrl Pts',(-9.70137854017372,-111.554517970998,
1.74701493417668E-11));
#18650=CARTESIAN_POINT('Ctrl Pts',(-7.27603390512272,-111.379517970998,
4.20082013377292));
#18651=CARTESIAN_POINT('Ctrl Pts',(-4.85068927007173,-111.204517970998,
8.40164026752836));
#18652=CARTESIAN_POINT('Ctrl Pts',(1.5129078685785E-11,-111.029517970998,
8.40164026751963));
#18653=CARTESIAN_POINT('Ctrl Pts',(4.85068927010198,-110.854517970998,8.4016402675109));
#18654=CARTESIAN_POINT('Ctrl Pts',(7.27603390513785,-110.679517970998,4.20082013374672));
#18655=CARTESIAN_POINT('Ctrl Pts',(9.70137854017372,-110.504517970998,-1.74689612655491E-11));
#18656=CARTESIAN_POINT('Ctrl Pts',(7.27603390512273,-110.329517970998,-4.20082013377291));
#18657=CARTESIAN_POINT('Ctrl Pts',(4.85068927007173,-110.154517970998,-8.40164026752836));
#18658=CARTESIAN_POINT('Ctrl Pts',(-1.51301075899711E-11,-109.979517970998,
-8.40164026751963));
#18659=CARTESIAN_POINT('Ctrl Pts',(-4.85068927010199,-109.804517970998,
-8.4016402675109));
#18660=CARTESIAN_POINT('Ctrl Pts',(-7.27603390513785,-109.629517970998,
-4.20082013374671));
#18661=CARTESIAN_POINT('Ctrl Pts',(-9.70137854017372,-109.454517970998,
1.74701493417668E-11));
#18662=CARTESIAN_POINT('Ctrl Pts',(-7.27603390512272,-109.279517970998,
4.20082013377292));
#18663=CARTESIAN_POINT('Ctrl Pts',(-4.85068927007173,-109.104517970998,
8.40164026752836));
#18664=CARTESIAN_POINT('Ctrl Pts',(1.5129078685785E-11,-108.929517970998,
8.40164026751963));
#18665=CARTESIAN_POINT('Ctrl Pts',(4.85068927010198,-108.754517970998,8.4016402675109));
#18666=CARTESIAN_POINT('Ctrl Pts',(7.27603390513785,-108.579517970998,4.20082013374672));
#18667=CARTESIAN_POINT('Ctrl Pts',(9.70137854017372,-108.404517970998,-1.74689612655491E-11));
#18668=CARTESIAN_POINT('Ctrl Pts',(7.27603390512273,-108.229517970998,-4.20082013377291));
#18669=CARTESIAN_POINT('Ctrl Pts',(4.85068927007173,-108.054517970998,-8.40164026752836));
#18670=CARTESIAN_POINT('Ctrl Pts',(-1.51301075899711E-11,-107.879517970998,
-8.40164026751963));
#18671=CARTESIAN_POINT('Ctrl Pts',(-4.85068927010199,-107.704517970998,
-8.4016402675109));
#18672=CARTESIAN_POINT('Ctrl Pts',(-7.27603390513785,-107.529517970998,
-4.20082013374671));
#18673=CARTESIAN_POINT('Ctrl Pts',(-9.70137854017372,-107.354517970998,
1.74701493417668E-11));
#18674=CARTESIAN_POINT('Ctrl Pts',(-7.27603390512272,-107.179517970998,
4.20082013377292));
#18675=CARTESIAN_POINT('Ctrl Pts',(-4.85068927007173,-107.004517970998,
8.40164026752836));
#18676=CARTESIAN_POINT('Ctrl Pts',(1.5129078685785E-11,-106.829517970998,
8.40164026751963));
#18677=CARTESIAN_POINT('Ctrl Pts',(4.85068927010198,-106.654517970998,8.4016402675109));
#18678=CARTESIAN_POINT('Ctrl Pts',(7.27603390513785,-106.479517970998,4.20082013374672));
#18679=CARTESIAN_POINT('Ctrl Pts',(9.70137854017372,-106.304517970998,-1.74689612655491E-11));
#18680=CARTESIAN_POINT('Ctrl Pts',(7.27603390512273,-106.129517970998,-4.20082013377291));
#18681=CARTESIAN_POINT('Ctrl Pts',(4.85068927007173,-105.954517970998,-8.40164026752836));
#18682=CARTESIAN_POINT('Ctrl Pts',(-1.51301075899711E-11,-105.779517970998,
-8.40164026751963));
#18683=CARTESIAN_POINT('Ctrl Pts',(-4.85068927010199,-105.604517970998,
-8.4016402675109));
#18684=CARTESIAN_POINT('Ctrl Pts',(-7.27603390513785,-105.429517970998,
-4.20082013374671));
#18685=CARTESIAN_POINT('Ctrl Pts',(-9.70137854017372,-105.254517970998,
1.74701493417668E-11));
#18686=CARTESIAN_POINT('Ctrl Pts',(-7.27603390512272,-105.079517970998,
4.20082013377292));
#18687=CARTESIAN_POINT('Ctrl Pts',(-4.85068927007173,-104.904517970998,
8.40164026752836));
#18688=CARTESIAN_POINT('Ctrl Pts',(1.5129078685785E-11,-104.729517970998,
8.40164026751963));
#18689=CARTESIAN_POINT('Ctrl Pts',(4.85068927010198,-104.554517970998,8.4016402675109));
#18690=CARTESIAN_POINT('Ctrl Pts',(7.27603390513785,-104.379517970998,4.20082013374672));
#18691=CARTESIAN_POINT('Ctrl Pts',(9.70137854017372,-104.204517970998,-1.74689612655491E-11));
#18692=CARTESIAN_POINT('Ctrl Pts',(7.27603390512273,-104.029517970998,-4.20082013377291));
#18693=CARTESIAN_POINT('Ctrl Pts',(4.85068927007173,-103.854517970998,-8.40164026752836));
#18694=CARTESIAN_POINT('Ctrl Pts',(-1.51301075899711E-11,-103.679517970998,
-8.40164026751963));
#18695=CARTESIAN_POINT('Ctrl Pts',(-4.85068927010199,-103.504517970998,
-8.4016402675109));
#18696=CARTESIAN_POINT('Ctrl Pts',(-7.27603390513785,-103.329517970998,
-4.20082013374671));
#18697=CARTESIAN_POINT('Ctrl Pts',(-9.70137854017372,-103.154517970998,
1.74701493417668E-11));
#18698=CARTESIAN_POINT('Ctrl Pts',(-7.27603390512272,-102.979517970998,
4.20082013377292));
#18699=CARTESIAN_POINT('Ctrl Pts',(-4.85068927007173,-102.804517970998,
8.40164026752836));
#18700=CARTESIAN_POINT('Ctrl Pts',(1.5129078685785E-11,-102.629517970998,
8.40164026751963));
#18701=CARTESIAN_POINT('Ctrl Pts',(4.85068927010198,-102.454517970998,8.4016402675109));
#18702=CARTESIAN_POINT('Ctrl Pts',(7.27603390513785,-102.279517970998,4.20082013374672));
#18703=CARTESIAN_POINT('Ctrl Pts',(9.70137854017372,-102.104517970998,-1.74689612655491E-11));
#18704=CARTESIAN_POINT('Ctrl Pts',(7.27603390512273,-101.929517970998,-4.20082013377291));
#18705=CARTESIAN_POINT('Ctrl Pts',(4.85068927007173,-101.754517970998,-8.40164026752836));
#18706=CARTESIAN_POINT('Ctrl Pts',(-1.51301075899711E-11,-101.579517970998,
-8.40164026751963));
#18707=CARTESIAN_POINT('Ctrl Pts',(-4.85068927010199,-101.404517970998,
-8.4016402675109));
#18708=CARTESIAN_POINT('Ctrl Pts',(-7.27603390513785,-101.229517970998,
-4.20082013374671));
#18709=CARTESIAN_POINT('Ctrl Pts',(-9.70137854017372,-101.054517970998,
1.74701493417668E-11));
#18710=CARTESIAN_POINT('Ctrl Pts',(-7.27603390512272,-100.879517970998,
4.20082013377292));
#18711=CARTESIAN_POINT('Ctrl Pts',(-4.85068927007173,-100.704517970998,
8.40164026752836));
#18712=CARTESIAN_POINT('Ctrl Pts',(1.5129078685785E-11,-100.529517970998,
8.40164026751963));
#18713=CARTESIAN_POINT('Ctrl Pts',(4.85068927010198,-100.354517970998,8.4016402675109));
#18714=CARTESIAN_POINT('Ctrl Pts',(7.27603390513785,-100.179517970998,4.20082013374672));
#18715=CARTESIAN_POINT('Ctrl Pts',(9.70137854017372,-100.004517970998,-1.74689612655491E-11));
#18716=CARTESIAN_POINT('Ctrl Pts',(7.27603390512273,-99.8295179709984,-4.20082013377291));
#18717=CARTESIAN_POINT('Ctrl Pts',(4.85068927007173,-99.6545179709984,-8.40164026752836));
#18718=CARTESIAN_POINT('Ctrl Pts',(-1.51301075899711E-11,-99.4795179709984,
-8.40164026751963));
#18719=CARTESIAN_POINT('Ctrl Pts',(-4.85068927010199,-99.3045179709984,
-8.4016402675109));
#18720=CARTESIAN_POINT('Ctrl Pts',(-7.27603390513785,-99.1295179709984,
-4.20082013374671));
#18721=CARTESIAN_POINT('Ctrl Pts',(-9.70137854017372,-98.9545179709984,
1.74701493417668E-11));
#18722=CARTESIAN_POINT('Ctrl Pts',(-7.27603390512272,-98.7795179709984,
4.20082013377292));
#18723=CARTESIAN_POINT('Ctrl Pts',(-4.85068927007173,-98.6045179709984,
8.40164026752836));
#18724=CARTESIAN_POINT('Ctrl Pts',(1.5129078685785E-11,-98.4295179709984,
8.40164026751963));
#18725=CARTESIAN_POINT('Ctrl Pts',(4.85068927010198,-98.2545179709984,8.4016402675109));
#18726=CARTESIAN_POINT('Ctrl Pts',(7.27603390513785,-98.0795179709984,4.20082013374672));
#18727=CARTESIAN_POINT('Ctrl Pts',(9.70137854017372,-97.9045179709984,-1.74689612655491E-11));
#18728=CARTESIAN_POINT('Ctrl Pts',(7.27603390512273,-97.7295179709984,-4.20082013377291));
#18729=CARTESIAN_POINT('Ctrl Pts',(4.85068927007173,-97.5545179709984,-8.40164026752836));
#18730=CARTESIAN_POINT('Ctrl Pts',(-1.51301075899711E-11,-97.3795179709984,
-8.40164026751963));
#18731=CARTESIAN_POINT('Ctrl Pts',(-4.85068927010199,-97.2045179709984,
-8.4016402675109));
#18732=CARTESIAN_POINT('Ctrl Pts',(-7.27603390513785,-97.0295179709984,
-4.20082013374671));
#18733=CARTESIAN_POINT('Ctrl Pts',(-9.70137854017372,-96.8545179709984,
1.74701493417668E-11));
#18734=CARTESIAN_POINT('Ctrl Pts',(-7.27603390512272,-96.6795179709984,
4.20082013377292));
#18735=CARTESIAN_POINT('Ctrl Pts',(-4.85068927007173,-96.5045179709984,
8.40164026752836));
#18736=CARTESIAN_POINT('Ctrl Pts',(1.5129078685785E-11,-96.3295179709984,
8.40164026751963));
#18737=CARTESIAN_POINT('Ctrl Pts',(4.85068927010198,-96.1545179709984,8.4016402675109));
#18738=CARTESIAN_POINT('Ctrl Pts',(7.27603390513785,-95.9795179709984,4.20082013374672));
#18739=CARTESIAN_POINT('Ctrl Pts',(9.70137854017372,-95.8045179709984,-1.74689612655491E-11));
#18740=CARTESIAN_POINT('Ctrl Pts',(7.27603390512273,-95.6295179709984,-4.20082013377291));
#18741=CARTESIAN_POINT('Ctrl Pts',(4.85068927007173,-95.4545179709984,-8.40164026752836));
#18742=CARTESIAN_POINT('Ctrl Pts',(-1.51301075899711E-11,-95.2795179709984,
-8.40164026751963));
#18743=CARTESIAN_POINT('Ctrl Pts',(-4.85068927010199,-95.1045179709984,
-8.4016402675109));
#18744=CARTESIAN_POINT('Ctrl Pts',(-7.27603390513785,-94.9295179709984,
-4.20082013374671));
#18745=CARTESIAN_POINT('Ctrl Pts',(-9.70137854017372,-94.7545179709984,
1.74701493417668E-11));
#18746=CARTESIAN_POINT('Ctrl Pts',(-7.27603390512272,-94.5795179709984,
4.20082013377292));
#18747=CARTESIAN_POINT('Ctrl Pts',(-4.85068927007173,-94.4045179709984,
8.40164026752836));
#18748=CARTESIAN_POINT('Ctrl Pts',(1.5129078685785E-11,-94.2295179709984,
8.40164026751963));
#18749=CARTESIAN_POINT('Ctrl Pts',(4.85068927010198,-94.0545179709984,8.4016402675109));
#18750=CARTESIAN_POINT('Ctrl Pts',(7.27603390513785,-93.8795179709984,4.20082013374672));
#18751=CARTESIAN_POINT('Ctrl Pts',(9.70137854017372,-93.7045179709984,-1.74689612655491E-11));
#18752=CARTESIAN_POINT('Ctrl Pts',(7.27603390512273,-93.5295179709984,-4.20082013377291));
#18753=CARTESIAN_POINT('Ctrl Pts',(4.85068927007173,-93.3545179709984,-8.40164026752836));
#18754=CARTESIAN_POINT('Ctrl Pts',(-1.51301075899711E-11,-93.1795179709984,
-8.40164026751963));
#18755=CARTESIAN_POINT('Ctrl Pts',(-4.85068927010199,-93.0045179709984,
-8.4016402675109));
#18756=CARTESIAN_POINT('Ctrl Pts',(-7.27603390513785,-92.8295179709984,
-4.20082013374671));
#18757=CARTESIAN_POINT('Ctrl Pts',(-9.70137854017372,-92.6545179709984,
1.74701493417668E-11));
#18758=CARTESIAN_POINT('Ctrl Pts',(-7.27603390512272,-92.4795179709984,
4.20082013377292));
#18759=CARTESIAN_POINT('Ctrl Pts',(-4.85068927007173,-92.3045179709984,
8.40164026752836));
#18760=CARTESIAN_POINT('Ctrl Pts',(1.5129078685785E-11,-92.1295179709984,
8.40164026751963));
#18761=CARTESIAN_POINT('Ctrl Pts',(4.85068927010198,-91.9545179709984,8.4016402675109));
#18762=CARTESIAN_POINT('Ctrl Pts',(7.27603390513785,-91.7795179709984,4.20082013374672));
#18763=CARTESIAN_POINT('Ctrl Pts',(9.70137854017372,-91.6045179709984,-1.74689612655491E-11));
#18764=CARTESIAN_POINT('Ctrl Pts',(7.27603390512273,-91.4295179709984,-4.20082013377291));
#18765=CARTESIAN_POINT('Ctrl Pts',(4.85068927007173,-91.2545179709984,-8.40164026752836));
#18766=CARTESIAN_POINT('Ctrl Pts',(-1.51301075899711E-11,-91.0795179709984,
-8.40164026751963));
#18767=CARTESIAN_POINT('Ctrl Pts',(-4.85068927010199,-90.9045179709984,
-8.4016402675109));
#18768=CARTESIAN_POINT('Ctrl Pts',(-7.27603390513785,-90.7295179709984,
-4.20082013374671));
#18769=CARTESIAN_POINT('Ctrl Pts',(-9.70137854017372,-90.5545179709984,
1.74701493417668E-11));
#18770=CARTESIAN_POINT('Ctrl Pts',(-7.27603390512272,-90.3795179709984,
4.20082013377292));
#18771=CARTESIAN_POINT('Ctrl Pts',(-4.85068927007173,-90.2045179709984,
8.40164026752836));
#18772=CARTESIAN_POINT('Ctrl Pts',(1.5129078685785E-11,-90.0295179709984,
8.40164026751963));
#18773=CARTESIAN_POINT('Ctrl Pts',(4.85068927010198,-89.8545179709984,8.4016402675109));
#18774=CARTESIAN_POINT('Ctrl Pts',(7.27603390513785,-89.6795179709984,4.20082013374672));
#18775=CARTESIAN_POINT('Ctrl Pts',(9.70137854017372,-89.5045179709984,-1.74689612655491E-11));
#18776=CARTESIAN_POINT('Ctrl Pts',(7.27603390512273,-89.3295179709984,-4.20082013377291));
#18777=CARTESIAN_POINT('Ctrl Pts',(4.85068927007173,-89.1545179709984,-8.40164026752836));
#18778=CARTESIAN_POINT('Ctrl Pts',(-1.51301075899711E-11,-88.9795179709984,
-8.40164026751963));
#18779=CARTESIAN_POINT('Ctrl Pts',(-4.85068927010199,-88.8045179709984,
-8.4016402675109));
#18780=CARTESIAN_POINT('Ctrl Pts',(-7.27603390513785,-88.6295179709984,
-4.20082013374671));
#18781=CARTESIAN_POINT('Ctrl Pts',(-9.70137854017372,-88.4545179709984,
1.74701493417668E-11));
#18782=CARTESIAN_POINT('Ctrl Pts',(-7.27603390512272,-88.2795179709984,
4.20082013377292));
#18783=CARTESIAN_POINT('Ctrl Pts',(-4.85068927007173,-88.1045179709984,
8.40164026752836));
#18784=CARTESIAN_POINT('Ctrl Pts',(1.5129078685785E-11,-87.9295179709984,
8.40164026751963));
#18785=CARTESIAN_POINT('Ctrl Pts',(4.85068927010198,-87.7545179709984,8.4016402675109));
#18786=CARTESIAN_POINT('Ctrl Pts',(7.27603390513785,-87.5795179709984,4.20082013374672));
#18787=CARTESIAN_POINT('Ctrl Pts',(9.70137854017372,-87.4045179709984,-1.74689612655491E-11));
#18788=CARTESIAN_POINT('Ctrl Pts',(7.27603390512273,-87.2295179709984,-4.20082013377291));
#18789=CARTESIAN_POINT('Ctrl Pts',(4.85068927007173,-87.0545179709984,-8.40164026752836));
#18790=CARTESIAN_POINT('Ctrl Pts',(-1.51301075899711E-11,-86.8795179709984,
-8.40164026751963));
#18791=CARTESIAN_POINT('Ctrl Pts',(-4.85068927010199,-86.7045179709984,
-8.4016402675109));
#18792=CARTESIAN_POINT('Ctrl Pts',(-7.27603390513785,-86.5295179709984,
-4.20082013374671));
#18793=CARTESIAN_POINT('Ctrl Pts',(-9.70137854017372,-86.3545179709984,
1.74701493417668E-11));
#18794=CARTESIAN_POINT('Ctrl Pts',(-7.27603390512272,-86.1795179709984,
4.20082013377292));
#18795=CARTESIAN_POINT('Ctrl Pts',(-4.85068927007173,-86.0045179709984,
8.40164026752836));
#18796=CARTESIAN_POINT('Ctrl Pts',(1.5129078685785E-11,-85.8295179709984,
8.40164026751963));
#18797=CARTESIAN_POINT('Ctrl Pts',(4.85068927010198,-85.6545179709984,8.4016402675109));
#18798=CARTESIAN_POINT('Ctrl Pts',(7.27603390513785,-85.4795179709984,4.20082013374672));
#18799=CARTESIAN_POINT('Ctrl Pts',(9.70137854017372,-85.3045179709984,-1.74689612655491E-11));
#18800=CARTESIAN_POINT('Ctrl Pts',(7.27603390512273,-85.1295179709984,-4.20082013377291));
#18801=CARTESIAN_POINT('Ctrl Pts',(4.85068927007173,-84.9545179709984,-8.40164026752836));
#18802=CARTESIAN_POINT('Ctrl Pts',(-1.51301075899711E-11,-84.7795179709984,
-8.40164026751963));
#18803=CARTESIAN_POINT('Ctrl Pts',(-4.85068927010199,-84.6045179709984,
-8.4016402675109));
#18804=CARTESIAN_POINT('Ctrl Pts',(-7.27603390513785,-84.4295179709984,
-4.20082013374671));
#18805=CARTESIAN_POINT('Ctrl Pts',(-9.70137854017372,-84.2545179709984,
1.74701493417668E-11));
#18806=CARTESIAN_POINT('Ctrl Pts',(-7.27603390512272,-84.0795179709984,
4.20082013377292));
#18807=CARTESIAN_POINT('Ctrl Pts',(-4.85068927007173,-83.9045179709984,
8.40164026752836));
#18808=CARTESIAN_POINT('Ctrl Pts',(1.5129078685785E-11,-83.7295179709984,
8.40164026751963));
#18809=CARTESIAN_POINT('Ctrl Pts',(4.85068927010198,-83.5545179709984,8.4016402675109));
#18810=CARTESIAN_POINT('Ctrl Pts',(7.27603390513785,-83.3795179709984,4.20082013374672));
#18811=CARTESIAN_POINT('Ctrl Pts',(9.70137854017372,-83.2045179709984,-1.74689612655491E-11));
#18812=CARTESIAN_POINT('Ctrl Pts',(7.27603390512273,-83.0295179709984,-4.20082013377291));
#18813=CARTESIAN_POINT('Ctrl Pts',(4.85068927007173,-82.8545179709984,-8.40164026752836));
#18814=CARTESIAN_POINT('Ctrl Pts',(-1.51301075899711E-11,-82.6795179709984,
-8.40164026751963));
#18815=CARTESIAN_POINT('Ctrl Pts',(-4.85068927010199,-82.5045179709984,
-8.4016402675109));
#18816=CARTESIAN_POINT('Ctrl Pts',(-7.27603390513785,-82.3295179709984,
-4.20082013374671));
#18817=CARTESIAN_POINT('Ctrl Pts',(-9.70137854017372,-82.1545179709984,
1.74701493417668E-11));
#18818=CARTESIAN_POINT('Ctrl Pts',(-7.27603390512272,-81.9795179709984,
4.20082013377292));
#18819=CARTESIAN_POINT('Ctrl Pts',(-4.85068927007173,-81.8045179709984,
8.40164026752836));
#18820=CARTESIAN_POINT('Ctrl Pts',(1.5129078685785E-11,-81.6295179709984,
8.40164026751963));
#18821=CARTESIAN_POINT('Ctrl Pts',(4.85068927010198,-81.4545179709984,8.4016402675109));
#18822=CARTESIAN_POINT('Ctrl Pts',(7.27603390513785,-81.2795179709984,4.20082013374672));
#18823=CARTESIAN_POINT('Ctrl Pts',(9.70137854017372,-81.1045179709984,-1.74689612655491E-11));
#18824=CARTESIAN_POINT('Ctrl Pts',(7.27603390512273,-80.9295179709984,-4.20082013377291));
#18825=CARTESIAN_POINT('Ctrl Pts',(4.85068927007173,-80.7545179709984,-8.40164026752836));
#18826=CARTESIAN_POINT('Ctrl Pts',(-1.51301075899711E-11,-80.5795179709984,
-8.40164026751963));
#18827=CARTESIAN_POINT('Ctrl Pts',(-4.85068927010199,-80.4045179709985,
-8.4016402675109));
#18828=CARTESIAN_POINT('Ctrl Pts',(-7.27603390513785,-80.2295179709984,
-4.20082013374671));
#18829=CARTESIAN_POINT('Ctrl Pts',(-9.70137854017372,-80.0545179709984,
1.74701493417668E-11));
#18830=CARTESIAN_POINT('Ctrl Pts',(-7.27603390512272,-79.8795179709984,
4.20082013377292));
#18831=CARTESIAN_POINT('Ctrl Pts',(-4.85068927007173,-79.7045179709984,
8.40164026752836));
#18832=CARTESIAN_POINT('Ctrl Pts',(1.5129078685785E-11,-79.5295179709984,
8.40164026751963));
#18833=CARTESIAN_POINT('Ctrl Pts',(4.85068927010198,-79.3545179709984,8.4016402675109));
#18834=CARTESIAN_POINT('Ctrl Pts',(7.27603390513785,-79.1795179709984,4.20082013374672));
#18835=CARTESIAN_POINT('Ctrl Pts',(9.70137854017372,-79.0045179709984,-1.74689612655491E-11));
#18836=CARTESIAN_POINT('Ctrl Pts',(7.27603390512273,-78.8295179709984,-4.20082013377291));
#18837=CARTESIAN_POINT('Ctrl Pts',(4.85068927007173,-78.6545179709984,-8.40164026752836));
#18838=CARTESIAN_POINT('Ctrl Pts',(-1.51301075899711E-11,-78.4795179709984,
-8.40164026751963));
#18839=CARTESIAN_POINT('Ctrl Pts',(-4.85068927010199,-78.3045179709985,
-8.4016402675109));
#18840=CARTESIAN_POINT('Ctrl Pts',(-7.27603390513785,-78.1295179709984,
-4.20082013374671));
#18841=CARTESIAN_POINT('Ctrl Pts',(-9.70137854017372,-77.9545179709984,
1.74701493417668E-11));
#18842=CARTESIAN_POINT('Ctrl Pts',(-7.27603390512272,-77.7795179709984,
4.20082013377292));
#18843=CARTESIAN_POINT('Ctrl Pts',(-4.85068927007173,-77.6045179709984,
8.40164026752836));
#18844=CARTESIAN_POINT('Ctrl Pts',(1.5129078685785E-11,-77.4295179709984,
8.40164026751963));
#18845=CARTESIAN_POINT('Ctrl Pts',(4.85068927010198,-77.2545179709984,8.4016402675109));
#18846=CARTESIAN_POINT('Ctrl Pts',(7.27603390513785,-77.0795179709984,4.20082013374672));
#18847=CARTESIAN_POINT('Ctrl Pts',(9.70137854017372,-76.9045179709984,-1.74689612655491E-11));
#18848=CARTESIAN_POINT('Ctrl Pts',(7.27603390512273,-76.7295179709984,-4.20082013377291));
#18849=CARTESIAN_POINT('Ctrl Pts',(4.85068927007173,-76.5545179709984,-8.40164026752836));
#18850=CARTESIAN_POINT('Ctrl Pts',(-1.51301075899711E-11,-76.3795179709984,
-8.40164026751963));
#18851=CARTESIAN_POINT('Ctrl Pts',(-4.85068927010199,-76.2045179709985,
-8.4016402675109));
#18852=CARTESIAN_POINT('Ctrl Pts',(-7.27603390513785,-76.0295179709984,
-4.20082013374671));
#18853=CARTESIAN_POINT('Ctrl Pts',(-9.70137854017372,-75.8545179709985,
1.74701493417668E-11));
#18854=CARTESIAN_POINT('Ctrl Pts',(-7.27603390512272,-75.6795179709984,
4.20082013377292));
#18855=CARTESIAN_POINT('Ctrl Pts',(-4.85068927007173,-75.5045179709984,
8.40164026752836));
#18856=CARTESIAN_POINT('Ctrl Pts',(1.5129078685785E-11,-75.3295179709984,
8.40164026751963));
#18857=CARTESIAN_POINT('Ctrl Pts',(4.85068927010198,-75.1545179709984,8.4016402675109));
#18858=CARTESIAN_POINT('Ctrl Pts',(7.27603390513785,-74.9795179709984,4.20082013374672));
#18859=CARTESIAN_POINT('Ctrl Pts',(9.70137854017372,-74.8045179709984,-1.74689612655491E-11));
#18860=CARTESIAN_POINT('Ctrl Pts',(7.27603390512273,-74.6295179709984,-4.20082013377291));
#18861=CARTESIAN_POINT('Ctrl Pts',(4.85068927007173,-74.4545179709984,-8.40164026752836));
#18862=CARTESIAN_POINT('Ctrl Pts',(-1.51301075899711E-11,-74.2795179709984,
-8.40164026751963));
#18863=CARTESIAN_POINT('Ctrl Pts',(-4.85068927010199,-74.1045179709984,
-8.4016402675109));
#18864=CARTESIAN_POINT('Ctrl Pts',(-7.27603390513785,-73.9295179709984,
-4.20082013374671));
#18865=CARTESIAN_POINT('Ctrl Pts',(-9.70137854017372,-73.7545179709984,
1.74701493417668E-11));
#18866=CARTESIAN_POINT('Ctrl Pts',(-7.27603390512272,-73.5795179709984,
4.20082013377292));
#18867=CARTESIAN_POINT('Ctrl Pts',(-4.85068927007173,-73.4045179709984,
8.40164026752836));
#18868=CARTESIAN_POINT('Ctrl Pts',(1.5129078685785E-11,-73.2295179709984,
8.40164026751963));
#18869=CARTESIAN_POINT('Ctrl Pts',(4.85068927010198,-73.0545179709984,8.4016402675109));
#18870=CARTESIAN_POINT('Ctrl Pts',(7.27603390513785,-72.8795179709984,4.20082013374672));
#18871=CARTESIAN_POINT('Ctrl Pts',(9.70137854017372,-72.7045179709984,-1.74689612655491E-11));
#18872=CARTESIAN_POINT('Ctrl Pts',(7.27603390512273,-72.5295179709984,-4.20082013377291));
#18873=CARTESIAN_POINT('Ctrl Pts',(4.85068927007173,-72.3545179709984,-8.40164026752836));
#18874=CARTESIAN_POINT('Ctrl Pts',(-1.51301075899711E-11,-72.1795179709984,
-8.40164026751963));
#18875=CARTESIAN_POINT('Ctrl Pts',(-4.85068927010199,-72.0045179709984,
-8.4016402675109));
#18876=CARTESIAN_POINT('Ctrl Pts',(-7.27603390513785,-71.8295179709984,
-4.20082013374671));
#18877=CARTESIAN_POINT('Ctrl Pts',(-9.70137854017372,-71.6545179709985,
1.74701493417668E-11));
#18878=CARTESIAN_POINT('Ctrl Pts',(-7.27603390512272,-71.4795179709984,
4.20082013377292));
#18879=CARTESIAN_POINT('Ctrl Pts',(-4.85068927007173,-71.3045179709984,
8.40164026752836));
#18880=CARTESIAN_POINT('Ctrl Pts',(1.5129078685785E-11,-71.1295179709984,
8.40164026751963));
#18881=CARTESIAN_POINT('Ctrl Pts',(4.85068927010198,-70.9545179709984,8.4016402675109));
#18882=CARTESIAN_POINT('Ctrl Pts',(7.27603390513785,-70.7795179709984,4.20082013374672));
#18883=CARTESIAN_POINT('Ctrl Pts',(9.70137854017372,-70.6045179709985,-1.74689612655491E-11));
#18884=CARTESIAN_POINT('Ctrl Pts',(7.27603390512273,-70.4295179709984,-4.20082013377291));
#18885=CARTESIAN_POINT('Ctrl Pts',(4.85068927007173,-70.2545179709984,-8.40164026752836));
#18886=CARTESIAN_POINT('Ctrl Pts',(-1.51301075899711E-11,-70.0795179709985,
-8.40164026751963));
#18887=CARTESIAN_POINT('Ctrl Pts',(-4.85068927010199,-69.9045179709984,
-8.4016402675109));
#18888=CARTESIAN_POINT('Ctrl Pts',(-7.27603390513785,-69.7295179709984,
-4.20082013374671));
#18889=CARTESIAN_POINT('Ctrl Pts',(-9.70137854017372,-69.5545179709985,
1.74701493417668E-11));
#18890=CARTESIAN_POINT('Ctrl Pts',(-7.27603390512272,-69.3795179709984,
4.20082013377292));
#18891=CARTESIAN_POINT('Ctrl Pts',(-4.85068927007173,-69.2045179709985,
8.40164026752836));
#18892=CARTESIAN_POINT('Ctrl Pts',(1.5129078685785E-11,-69.0295179709985,
8.40164026751963));
#18893=CARTESIAN_POINT('Ctrl Pts',(4.85068927010198,-68.8545179709984,8.4016402675109));
#18894=CARTESIAN_POINT('Ctrl Pts',(7.27603390513785,-68.6795179709985,4.20082013374672));
#18895=CARTESIAN_POINT('Ctrl Pts',(9.70137854017372,-68.5045179709985,-1.74689612655491E-11));
#18896=CARTESIAN_POINT('Ctrl Pts',(7.27603390512273,-68.3295179709984,-4.20082013377291));
#18897=CARTESIAN_POINT('Ctrl Pts',(4.85068927007173,-68.1545179709985,-8.40164026752836));
#18898=CARTESIAN_POINT('Ctrl Pts',(-1.51301075899711E-11,-67.9795179709985,
-8.40164026751963));
#18899=CARTESIAN_POINT('Ctrl Pts',(-4.85068927010199,-67.8045179709984,
-8.4016402675109));
#18900=CARTESIAN_POINT('Ctrl Pts',(-7.27603390513785,-67.6295179709984,
-4.20082013374671));
#18901=CARTESIAN_POINT('Ctrl Pts',(-9.70137854017372,-67.4545179709985,
1.74701493417668E-11));
#18902=CARTESIAN_POINT('Ctrl Pts',(-7.27603390512272,-67.2795179709984,
4.20082013377292));
#18903=CARTESIAN_POINT('Ctrl Pts',(-4.85068927007173,-67.1045179709985,
8.40164026752836));
#18904=CARTESIAN_POINT('Ctrl Pts',(1.5129078685785E-11,-66.9295179709985,
8.40164026751963));
#18905=CARTESIAN_POINT('Ctrl Pts',(4.85068927010198,-66.7545179709984,8.4016402675109));
#18906=CARTESIAN_POINT('Ctrl Pts',(7.27603390513785,-66.5795179709985,4.20082013374672));
#18907=CARTESIAN_POINT('Ctrl Pts',(9.70137854017372,-66.4045179709985,-1.74689612655491E-11));
#18908=CARTESIAN_POINT('Ctrl Pts',(7.27603390512273,-66.2295179709984,-4.20082013377291));
#18909=CARTESIAN_POINT('Ctrl Pts',(4.85068927007173,-66.0545179709985,-8.40164026752836));
#18910=CARTESIAN_POINT('Ctrl Pts',(-1.51301075899711E-11,-65.8795179709984,
-8.40164026751963));
#18911=CARTESIAN_POINT('Ctrl Pts',(-4.85068927010199,-65.7045179709985,
-8.4016402675109));
#18912=CARTESIAN_POINT('Ctrl Pts',(-7.27603390513785,-65.5295179709985,
-4.20082013374671));
#18913=CARTESIAN_POINT('Ctrl Pts',(-9.70137854017372,-65.3545179709984,
1.74701493417668E-11));
#18914=CARTESIAN_POINT('Ctrl Pts',(-7.27603390512272,-65.1795179709984,
4.20082013377292));
#18915=CARTESIAN_POINT('Ctrl Pts',(-4.85068927007173,-65.0045179709985,
8.40164026752836));
#18916=CARTESIAN_POINT('Ctrl Pts',(1.5129078685785E-11,-64.8295179709985,
8.40164026751963));
#18917=CARTESIAN_POINT('Ctrl Pts',(4.85068927010198,-64.6545179709985,8.4016402675109));
#18918=CARTESIAN_POINT('Ctrl Pts',(7.27603390513785,-64.4795179709985,4.20082013374672));
#18919=CARTESIAN_POINT('Ctrl Pts',(9.70137854017372,-64.3045179709985,-1.74689612655491E-11));
#18920=CARTESIAN_POINT('Ctrl Pts',(7.27603390512273,-64.1295179709984,-4.20082013377291));
#18921=CARTESIAN_POINT('Ctrl Pts',(4.85068927007173,-63.9545179709985,-8.40164026752836));
#18922=CARTESIAN_POINT('Ctrl Pts',(-1.51301075899711E-11,-63.7795179709985,
-8.40164026751963));
#18923=CARTESIAN_POINT('Ctrl Pts',(-4.85068927010199,-63.6045179709985,
-8.4016402675109));
#18924=CARTESIAN_POINT('Ctrl Pts',(-7.27603390513785,-63.4295179709985,
-4.20082013374671));
#18925=CARTESIAN_POINT('Ctrl Pts',(-9.70137854017372,-63.2545179709985,
1.74701493417668E-11));
#18926=CARTESIAN_POINT('Ctrl Pts',(-7.27603390512272,-63.0795179709985,
4.20082013377292));
#18927=CARTESIAN_POINT('Ctrl Pts',(-4.85068927007173,-62.9045179709985,
8.40164026752836));
#18928=CARTESIAN_POINT('Ctrl Pts',(1.5129078685785E-11,-62.7295179709985,
8.40164026751963));
#18929=CARTESIAN_POINT('Ctrl Pts',(4.85068927010198,-62.5545179709985,8.4016402675109));
#18930=CARTESIAN_POINT('Ctrl Pts',(7.27603390513785,-62.3795179709985,4.20082013374672));
#18931=CARTESIAN_POINT('Ctrl Pts',(9.70137854017372,-62.2045179709985,-1.74689612655491E-11));
#18932=CARTESIAN_POINT('Ctrl Pts',(7.27603390512273,-62.0295179709985,-4.20082013377291));
#18933=CARTESIAN_POINT('Ctrl Pts',(4.85068927007173,-61.8545179709985,-8.40164026752836));
#18934=CARTESIAN_POINT('Ctrl Pts',(-1.51301075899711E-11,-61.6795179709985,
-8.40164026751963));
#18935=CARTESIAN_POINT('Ctrl Pts',(-4.85068927010199,-61.5045179709985,
-8.4016402675109));
#18936=CARTESIAN_POINT('Ctrl Pts',(-7.27603390513785,-61.3295179709985,
-4.20082013374671));
#18937=CARTESIAN_POINT('Ctrl Pts',(-9.70137854017372,-61.1545179709985,
1.74701493417668E-11));
#18938=CARTESIAN_POINT('Ctrl Pts',(-7.27603390512272,-60.9795179709985,
4.20082013377292));
#18939=CARTESIAN_POINT('Ctrl Pts',(-4.85068927007173,-60.8045179709985,
8.40164026752836));
#18940=CARTESIAN_POINT('Ctrl Pts',(1.5129078685785E-11,-60.6295179709985,
8.40164026751963));
#18941=CARTESIAN_POINT('Ctrl Pts',(4.85068927010198,-60.4545179709985,8.4016402675109));
#18942=CARTESIAN_POINT('Ctrl Pts',(7.27603390513785,-60.2795179709985,4.20082013374672));
#18943=CARTESIAN_POINT('Ctrl Pts',(9.70137854017372,-60.1045179709985,-1.74689612655491E-11));
#18944=CARTESIAN_POINT('Ctrl Pts',(7.27603390512273,-59.9295179709985,-4.20082013377291));
#18945=CARTESIAN_POINT('Ctrl Pts',(4.85068927007173,-59.7545179709985,-8.40164026752836));
#18946=CARTESIAN_POINT('Ctrl Pts',(-1.51301075899711E-11,-59.5795179709985,
-8.40164026751963));
#18947=CARTESIAN_POINT('Ctrl Pts',(-4.85068927010199,-59.4045179709985,
-8.4016402675109));
#18948=CARTESIAN_POINT('Ctrl Pts',(-7.27603390513785,-59.2295179709985,
-4.20082013374671));
#18949=CARTESIAN_POINT('Ctrl Pts',(-9.70137854017372,-59.0545179709985,
1.74701493417668E-11));
#18950=CARTESIAN_POINT('Ctrl Pts',(-7.27603390512272,-58.8795179709985,
4.20082013377292));
#18951=CARTESIAN_POINT('Ctrl Pts',(-4.85068927007173,-58.7045179709985,
8.40164026752836));
#18952=CARTESIAN_POINT('Ctrl Pts',(1.5129078685785E-11,-58.5295179709984,
8.40164026751963));
#18953=CARTESIAN_POINT('Ctrl Pts',(4.85068927010198,-58.3545179709985,8.4016402675109));
#18954=CARTESIAN_POINT('Ctrl Pts',(7.27603390513785,-58.1795179709985,4.20082013374672));
#18955=CARTESIAN_POINT('Ctrl Pts',(9.70137854017372,-58.0045179709985,-1.74689612655491E-11));
#18956=CARTESIAN_POINT('Ctrl Pts',(7.27603390512273,-57.8295179709985,-4.20082013377291));
#18957=CARTESIAN_POINT('Ctrl Pts',(4.85068927007173,-57.6545179709985,-8.40164026752836));
#18958=CARTESIAN_POINT('Ctrl Pts',(-1.51301075899711E-11,-57.4795179709985,
-8.40164026751963));
#18959=CARTESIAN_POINT('Ctrl Pts',(-4.85068927010199,-57.3045179709985,
-8.4016402675109));
#18960=CARTESIAN_POINT('Ctrl Pts',(-7.27603390513785,-57.1295179709985,
-4.20082013374671));
#18961=CARTESIAN_POINT('Ctrl Pts',(-9.70137854017372,-56.9545179709985,
1.74701493417668E-11));
#18962=CARTESIAN_POINT('Ctrl Pts',(-7.27603390512272,-56.7795179709985,
4.20082013377292));
#18963=CARTESIAN_POINT('Ctrl Pts',(-4.85068927007173,-56.6045179709985,
8.40164026752836));
#18964=CARTESIAN_POINT('Ctrl Pts',(1.5129078685785E-11,-56.4295179709985,
8.40164026751963));
#18965=CARTESIAN_POINT('Ctrl Pts',(4.85068927010198,-56.2545179709985,8.4016402675109));
#18966=CARTESIAN_POINT('Ctrl Pts',(7.27603390513785,-56.0795179709985,4.20082013374672));
#18967=CARTESIAN_POINT('Ctrl Pts',(9.70137854017372,-55.9045179709985,-1.74689612655491E-11));
#18968=CARTESIAN_POINT('Ctrl Pts',(7.27603390512273,-55.7295179709985,-4.20082013377291));
#18969=CARTESIAN_POINT('Ctrl Pts',(4.85068927007173,-55.5545179709985,-8.40164026752836));
#18970=CARTESIAN_POINT('Ctrl Pts',(-1.51301075899711E-11,-55.3795179709985,
-8.40164026751963));
#18971=CARTESIAN_POINT('Ctrl Pts',(-4.85068927010199,-55.2045179709985,
-8.4016402675109));
#18972=CARTESIAN_POINT('Ctrl Pts',(-7.27603390513785,-55.0295179709985,
-4.20082013374671));
#18973=CARTESIAN_POINT('Ctrl Pts',(-9.70137854017372,-54.8545179709985,
1.74701493417668E-11));
#18974=CARTESIAN_POINT('Ctrl Pts',(-7.27603390512272,-54.6795179709985,
4.20082013377292));
#18975=CARTESIAN_POINT('Ctrl Pts',(-4.85068927007173,-54.5045179709985,
8.40164026752836));
#18976=CARTESIAN_POINT('Ctrl Pts',(1.5129078685785E-11,-54.3295179709985,
8.40164026751963));
#18977=CARTESIAN_POINT('Ctrl Pts',(4.85068927010198,-54.1545179709985,8.4016402675109));
#18978=CARTESIAN_POINT('Ctrl Pts',(7.27603390513785,-53.9795179709985,4.20082013374672));
#18979=CARTESIAN_POINT('Ctrl Pts',(9.70137854017372,-53.8045179709985,-1.74689612655491E-11));
#18980=CARTESIAN_POINT('Ctrl Pts',(7.27603390512273,-53.6295179709985,-4.20082013377291));
#18981=CARTESIAN_POINT('Ctrl Pts',(4.85068927007173,-53.4545179709985,-8.40164026752836));
#18982=CARTESIAN_POINT('Ctrl Pts',(-1.51301075899711E-11,-53.2795179709985,
-8.40164026751963));
#18983=CARTESIAN_POINT('Ctrl Pts',(-4.85068927010199,-53.1045179709985,
-8.4016402675109));
#18984=CARTESIAN_POINT('Ctrl Pts',(-7.27603390513785,-52.9295179709985,
-4.20082013374671));
#18985=CARTESIAN_POINT('Ctrl Pts',(-9.70137854017372,-52.7545179709985,
1.74701493417668E-11));
#18986=CARTESIAN_POINT('Ctrl Pts',(-7.27603390512272,-52.5795179709985,
4.20082013377292));
#18987=CARTESIAN_POINT('Ctrl Pts',(-4.85068927007173,-52.4045179709985,
8.40164026752836));
#18988=CARTESIAN_POINT('Ctrl Pts',(1.5129078685785E-11,-52.2295179709985,
8.40164026751963));
#18989=CARTESIAN_POINT('Ctrl Pts',(4.85068927010198,-52.0545179709985,8.4016402675109));
#18990=CARTESIAN_POINT('Ctrl Pts',(7.27603390513785,-51.8795179709985,4.20082013374672));
#18991=CARTESIAN_POINT('Ctrl Pts',(9.70137854017372,-51.7045179709985,-1.74689612655491E-11));
#18992=CARTESIAN_POINT('Ctrl Pts',(7.27603390512273,-51.5295179709985,-4.20082013377291));
#18993=CARTESIAN_POINT('Ctrl Pts',(4.85068927007173,-51.3545179709985,-8.40164026752836));
#18994=CARTESIAN_POINT('Ctrl Pts',(-1.51301075899711E-11,-51.1795179709985,
-8.40164026751963));
#18995=CARTESIAN_POINT('Ctrl Pts',(-4.85068927010199,-51.0045179709985,
-8.4016402675109));
#18996=CARTESIAN_POINT('Ctrl Pts',(-7.27603390513785,-50.8295179709985,
-4.20082013374671));
#18997=CARTESIAN_POINT('Ctrl Pts',(-9.70137854017372,-50.6545179709985,
1.74701493417668E-11));
#18998=CARTESIAN_POINT('Ctrl Pts',(-7.27603390512272,-50.4795179709985,
4.20082013377292));
#18999=CARTESIAN_POINT('Ctrl Pts',(-4.85068927007173,-50.3045179709985,
8.40164026752836));
#19000=CARTESIAN_POINT('Ctrl Pts',(1.5129078685785E-11,-50.1295179709985,
8.40164026751963));
#19001=CARTESIAN_POINT('Ctrl Pts',(4.85068927010198,-49.9545179709985,8.4016402675109));
#19002=CARTESIAN_POINT('Ctrl Pts',(7.27603390513785,-49.7795179709985,4.20082013374672));
#19003=CARTESIAN_POINT('Ctrl Pts',(9.70137854017372,-49.6045179709985,-1.74689612655491E-11));
#19004=CARTESIAN_POINT('Ctrl Pts',(7.27603390512273,-49.4295179709985,-4.20082013377291));
#19005=CARTESIAN_POINT('Ctrl Pts',(4.85068927007173,-49.2545179709985,-8.40164026752836));
#19006=CARTESIAN_POINT('Ctrl Pts',(-1.51301075899711E-11,-49.0795179709985,
-8.40164026751963));
#19007=CARTESIAN_POINT('Ctrl Pts',(-4.85068927010199,-48.9045179709985,
-8.4016402675109));
#19008=CARTESIAN_POINT('Ctrl Pts',(-7.27603390513785,-48.7295179709985,
-4.20082013374671));
#19009=CARTESIAN_POINT('Ctrl Pts',(-9.70137854017372,-48.5545179709985,
1.74701493417668E-11));
#19010=CARTESIAN_POINT('Ctrl Pts',(-7.27603390512272,-48.3795179709985,
4.20082013377292));
#19011=CARTESIAN_POINT('Ctrl Pts',(-4.85068927007173,-48.2045179709985,
8.40164026752836));
#19012=CARTESIAN_POINT('Ctrl Pts',(1.5129078685785E-11,-48.0295179709985,
8.40164026751963));
#19013=CARTESIAN_POINT('Ctrl Pts',(4.85068927010198,-47.8545179709985,8.4016402675109));
#19014=CARTESIAN_POINT('Ctrl Pts',(7.27603390513785,-47.6795179709985,4.20082013374672));
#19015=CARTESIAN_POINT('Ctrl Pts',(9.70137854017372,-47.5045179709985,-1.74689612655491E-11));
#19016=CARTESIAN_POINT('Ctrl Pts',(7.27603390512273,-47.3295179709985,-4.20082013377291));
#19017=CARTESIAN_POINT('Ctrl Pts',(4.85068927007173,-47.1545179709985,-8.40164026752836));
#19018=CARTESIAN_POINT('Ctrl Pts',(-1.51301075899711E-11,-46.9795179709985,
-8.40164026751963));
#19019=CARTESIAN_POINT('Ctrl Pts',(-4.85068927010199,-46.8045179709985,
-8.4016402675109));
#19020=CARTESIAN_POINT('Ctrl Pts',(-7.27603390513785,-46.6295179709985,
-4.20082013374671));
#19021=CARTESIAN_POINT('Ctrl Pts',(-9.70137854017372,-46.4545179709985,
1.74701493417668E-11));
#19022=CARTESIAN_POINT('Ctrl Pts',(-7.27603390512272,-46.2795179709985,
4.20082013377292));
#19023=CARTESIAN_POINT('Ctrl Pts',(-4.85068927007173,-46.1045179709985,
8.40164026752836));
#19024=CARTESIAN_POINT('Ctrl Pts',(1.5129078685785E-11,-45.9295179709985,
8.40164026751963));
#19025=CARTESIAN_POINT('Ctrl Pts',(4.85068927010198,-45.7545179709985,8.4016402675109));
#19026=CARTESIAN_POINT('Ctrl Pts',(7.27603390513785,-45.5795179709985,4.20082013374672));
#19027=CARTESIAN_POINT('Ctrl Pts',(9.70137854017372,-45.4045179709985,-1.74689612655491E-11));
#19028=CARTESIAN_POINT('Ctrl Pts',(7.27603390512273,-45.2295179709985,-4.20082013377291));
#19029=CARTESIAN_POINT('Ctrl Pts',(4.85068927007173,-45.0545179709985,-8.40164026752836));
#19030=CARTESIAN_POINT('Ctrl Pts',(-1.51301075899711E-11,-44.8795179709985,
-8.40164026751963));
#19031=CARTESIAN_POINT('Ctrl Pts',(-4.85068927010199,-44.7045179709985,
-8.4016402675109));
#19032=CARTESIAN_POINT('Ctrl Pts',(-7.27603390513785,-44.5295179709985,
-4.20082013374671));
#19033=CARTESIAN_POINT('Ctrl Pts',(-9.70137854017372,-44.3545179709985,
1.74701493417668E-11));
#19034=CARTESIAN_POINT('Ctrl Pts',(-7.27603390512272,-44.1795179709985,
4.20082013377292));
#19035=CARTESIAN_POINT('Ctrl Pts',(-4.85068927007173,-44.0045179709985,
8.40164026752836));
#19036=CARTESIAN_POINT('Ctrl Pts',(1.5129078685785E-11,-43.8295179709985,
8.40164026751963));
#19037=CARTESIAN_POINT('Ctrl Pts',(4.85068927010198,-43.6545179709985,8.4016402675109));
#19038=CARTESIAN_POINT('Ctrl Pts',(7.27603390513785,-43.4795179709985,4.20082013374672));
#19039=CARTESIAN_POINT('Ctrl Pts',(9.70137854017372,-43.3045179709985,-1.74689612655491E-11));
#19040=CARTESIAN_POINT('Ctrl Pts',(7.27603390512273,-43.1295179709985,-4.20082013377291));
#19041=CARTESIAN_POINT('Ctrl Pts',(4.85068927007173,-42.9545179709985,-8.40164026752836));
#19042=CARTESIAN_POINT('Ctrl Pts',(-1.51301075899711E-11,-42.7795179709985,
-8.40164026751963));
#19043=CARTESIAN_POINT('Ctrl Pts',(-4.85068927010199,-42.6045179709985,
-8.4016402675109));
#19044=CARTESIAN_POINT('Ctrl Pts',(-7.27603390513785,-42.4295179709985,
-4.20082013374671));
#19045=CARTESIAN_POINT('Ctrl Pts',(-9.70137854017372,-42.2545179709985,
1.74701493417668E-11));
#19046=CARTESIAN_POINT('Ctrl Pts',(-7.27603390512272,-42.0795179709985,
4.20082013377292));
#19047=CARTESIAN_POINT('Ctrl Pts',(-4.85068927007173,-41.9045179709985,
8.40164026752836));
#19048=CARTESIAN_POINT('Ctrl Pts',(1.5129078685785E-11,-41.7295179709985,
8.40164026751963));
#19049=CARTESIAN_POINT('Ctrl Pts',(4.85068927010198,-41.5545179709985,8.4016402675109));
#19050=CARTESIAN_POINT('Ctrl Pts',(7.27603390513785,-41.3795179709985,4.20082013374672));
#19051=CARTESIAN_POINT('Ctrl Pts',(9.70137854017372,-41.2045179709985,-1.74689612655491E-11));
#19052=CARTESIAN_POINT('Ctrl Pts',(7.27603390512273,-41.0295179709985,-4.20082013377291));
#19053=CARTESIAN_POINT('Ctrl Pts',(4.85068927007173,-40.8545179709985,-8.40164026752836));
#19054=CARTESIAN_POINT('Ctrl Pts',(-1.51301075899711E-11,-40.6795179709985,
-8.40164026751963));
#19055=CARTESIAN_POINT('Ctrl Pts',(-4.85068927010199,-40.5045179709985,
-8.4016402675109));
#19056=CARTESIAN_POINT('Ctrl Pts',(-7.27603390513785,-40.3295179709985,
-4.20082013374671));
#19057=CARTESIAN_POINT('Ctrl Pts',(-9.70137854017372,-40.1545179709985,
1.74701493417668E-11));
#19058=CARTESIAN_POINT('Ctrl Pts',(-7.27603390512272,-39.9795179709985,
4.20082013377292));
#19059=CARTESIAN_POINT('Ctrl Pts',(-4.85068927007173,-39.8045179709985,
8.40164026752836));
#19060=CARTESIAN_POINT('Ctrl Pts',(1.5129078685785E-11,-39.6295179709985,
8.40164026751963));
#19061=CARTESIAN_POINT('Ctrl Pts',(4.85068927010198,-39.4545179709985,8.4016402675109));
#19062=CARTESIAN_POINT('Ctrl Pts',(7.27603390513785,-39.2795179709985,4.20082013374672));
#19063=CARTESIAN_POINT('Ctrl Pts',(9.70137854017372,-39.1045179709985,-1.74689612655491E-11));
#19064=CARTESIAN_POINT('Ctrl Pts',(7.27603390512273,-38.9295179709985,-4.20082013377291));
#19065=CARTESIAN_POINT('Ctrl Pts',(4.85068927007173,-38.7545179709985,-8.40164026752836));
#19066=CARTESIAN_POINT('Ctrl Pts',(-1.51301075899711E-11,-38.5795179709985,
-8.40164026751963));
#19067=CARTESIAN_POINT('Ctrl Pts',(-4.85068927010199,-38.4045179709985,
-8.4016402675109));
#19068=CARTESIAN_POINT('Ctrl Pts',(-7.27603390513785,-38.2295179709985,
-4.20082013374671));
#19069=CARTESIAN_POINT('Ctrl Pts',(-9.70137854017372,-38.0545179709985,
1.74701493417668E-11));
#19070=CARTESIAN_POINT('Ctrl Pts',(-7.27603390512272,-37.8795179709985,
4.20082013377292));
#19071=CARTESIAN_POINT('Ctrl Pts',(-4.85068927007173,-37.7045179709985,
8.40164026752836));
#19072=CARTESIAN_POINT('Ctrl Pts',(1.5129078685785E-11,-37.5295179709985,
8.40164026751963));
#19073=CARTESIAN_POINT('Ctrl Pts',(4.85068927010198,-37.3545179709985,8.4016402675109));
#19074=CARTESIAN_POINT('Ctrl Pts',(7.27603390513785,-37.1795179709985,4.20082013374672));
#19075=CARTESIAN_POINT('Ctrl Pts',(9.70137854017372,-37.0045179709985,-1.74689612655491E-11));
#19076=CARTESIAN_POINT('Ctrl Pts',(7.27603390512273,-36.8295179709985,-4.20082013377291));
#19077=CARTESIAN_POINT('Ctrl Pts',(4.85068927007173,-36.6545179709985,-8.40164026752836));
#19078=CARTESIAN_POINT('Ctrl Pts',(-1.51301075899711E-11,-36.4795179709985,
-8.40164026751963));
#19079=CARTESIAN_POINT('Ctrl Pts',(-4.85068927010199,-36.3045179709985,
-8.4016402675109));
#19080=CARTESIAN_POINT('Ctrl Pts',(-7.27603390513785,-36.1295179709985,
-4.20082013374671));
#19081=CARTESIAN_POINT('Ctrl Pts',(-9.70137854017372,-35.9545179709985,
1.74701493417668E-11));
#19082=CARTESIAN_POINT('Ctrl Pts',(-7.27603390512272,-35.7795179709985,
4.20082013377292));
#19083=CARTESIAN_POINT('Ctrl Pts',(-4.85068927007173,-35.6045179709985,
8.40164026752836));
#19084=CARTESIAN_POINT('Ctrl Pts',(1.5129078685785E-11,-35.4295179709985,
8.40164026751963));
#19085=CARTESIAN_POINT('Ctrl Pts',(4.85068927010198,-35.2545179709985,8.4016402675109));
#19086=CARTESIAN_POINT('Ctrl Pts',(7.27603390513785,-35.0795179709985,4.20082013374672));
#19087=CARTESIAN_POINT('Ctrl Pts',(9.70137854017372,-34.9045179709985,-1.74689612655491E-11));
#19088=CARTESIAN_POINT('Ctrl Pts',(7.27603390512273,-34.7295179709985,-4.20082013377291));
#19089=CARTESIAN_POINT('Ctrl Pts',(4.85068927007173,-34.5545179709985,-8.40164026752836));
#19090=CARTESIAN_POINT('Ctrl Pts',(-1.51301075899711E-11,-34.3795179709985,
-8.40164026751963));
#19091=CARTESIAN_POINT('Ctrl Pts',(-4.85068927010199,-34.2045179709985,
-8.4016402675109));
#19092=CARTESIAN_POINT('Ctrl Pts',(-7.27603390513785,-34.0295179709985,
-4.20082013374671));
#19093=CARTESIAN_POINT('Ctrl Pts',(-9.70137854017372,-33.8545179709985,
1.74701493417668E-11));
#19094=CARTESIAN_POINT('Ctrl Pts',(-7.27603390512272,-33.6795179709985,
4.20082013377292));
#19095=CARTESIAN_POINT('Ctrl Pts',(-4.85068927007173,-33.5045179709985,
8.40164026752836));
#19096=CARTESIAN_POINT('Ctrl Pts',(1.5129078685785E-11,-33.3295179709985,
8.40164026751963));
#19097=CARTESIAN_POINT('Ctrl Pts',(4.85068927010198,-33.1545179709985,8.4016402675109));
#19098=CARTESIAN_POINT('Ctrl Pts',(7.27603390513785,-32.9795179709985,4.20082013374672));
#19099=CARTESIAN_POINT('Ctrl Pts',(9.70137854017372,-32.8045179709985,-1.74689612655491E-11));
#19100=CARTESIAN_POINT('Ctrl Pts',(7.27603390512273,-32.6295179709985,-4.20082013377291));
#19101=CARTESIAN_POINT('Ctrl Pts',(4.85068927007173,-32.4545179709985,-8.40164026752836));
#19102=CARTESIAN_POINT('Ctrl Pts',(-1.51301075899711E-11,-32.2795179709985,
-8.40164026751963));
#19103=CARTESIAN_POINT('Ctrl Pts',(-4.85068927010199,-32.1045179709985,
-8.4016402675109));
#19104=CARTESIAN_POINT('Ctrl Pts',(-7.27603390513785,-31.9295179709985,
-4.20082013374671));
#19105=CARTESIAN_POINT('Ctrl Pts',(-9.70137854017372,-31.7545179709985,
1.74701493417668E-11));
#19106=CARTESIAN_POINT('Ctrl Pts',(-7.27603390512272,-31.5795179709985,
4.20082013377292));
#19107=CARTESIAN_POINT('Ctrl Pts',(-4.85068927007173,-31.4045179709985,
8.40164026752836));
#19108=CARTESIAN_POINT('Ctrl Pts',(1.5129078685785E-11,-31.2295179709985,
8.40164026751963));
#19109=CARTESIAN_POINT('Ctrl Pts',(4.85068927010198,-31.0545179709985,8.4016402675109));
#19110=CARTESIAN_POINT('Ctrl Pts',(7.27603390513785,-30.8795179709985,4.20082013374672));
#19111=CARTESIAN_POINT('Ctrl Pts',(9.70137854017372,-30.7045179709985,-1.74689612655491E-11));
#19112=CARTESIAN_POINT('Ctrl Pts',(7.27603390512273,-30.5295179709985,-4.20082013377291));
#19113=CARTESIAN_POINT('Ctrl Pts',(4.85068927007173,-30.3545179709985,-8.40164026752836));
#19114=CARTESIAN_POINT('Ctrl Pts',(-1.51301075899711E-11,-30.1795179709985,
-8.40164026751963));
#19115=CARTESIAN_POINT('Ctrl Pts',(-4.85068927010199,-30.0045179709985,
-8.4016402675109));
#19116=CARTESIAN_POINT('Ctrl Pts',(-7.27603390513785,-29.8295179709985,
-4.20082013374671));
#19117=CARTESIAN_POINT('Ctrl Pts',(-9.70137854017372,-29.6545179709985,
1.74701493417668E-11));
#19118=CARTESIAN_POINT('Ctrl Pts',(-7.27603390512272,-29.4795179709985,
4.20082013377292));
#19119=CARTESIAN_POINT('Ctrl Pts',(-4.85068927007173,-29.3045179709985,
8.40164026752836));
#19120=CARTESIAN_POINT('Ctrl Pts',(1.5129078685785E-11,-29.1295179709985,
8.40164026751963));
#19121=CARTESIAN_POINT('Ctrl Pts',(4.85068927010198,-28.9545179709986,8.4016402675109));
#19122=CARTESIAN_POINT('Ctrl Pts',(7.27603390513785,-28.7795179709985,4.20082013374672));
#19123=CARTESIAN_POINT('Ctrl Pts',(9.70137854017372,-28.6045179709986,-1.74689612655491E-11));
#19124=CARTESIAN_POINT('Ctrl Pts',(7.27603390512273,-28.4295179709985,-4.20082013377291));
#19125=CARTESIAN_POINT('Ctrl Pts',(4.85068927007173,-28.2545179709985,-8.40164026752836));
#19126=CARTESIAN_POINT('Ctrl Pts',(-1.51301075899711E-11,-28.0795179709985,
-8.40164026751963));
#19127=CARTESIAN_POINT('Ctrl Pts',(-4.85068927010199,-27.9045179709985,
-8.4016402675109));
#19128=CARTESIAN_POINT('Ctrl Pts',(-7.27603390513785,-27.7295179709985,
-4.20082013374671));
#19129=CARTESIAN_POINT('Ctrl Pts',(-9.70137854017372,-27.5545179709986,
1.74701493417668E-11));
#19130=CARTESIAN_POINT('Ctrl Pts',(-7.27603390512272,-27.3795179709985,
4.20082013377292));
#19131=CARTESIAN_POINT('Ctrl Pts',(-4.85068927007173,-27.2045179709986,
8.40164026752836));
#19132=CARTESIAN_POINT('Ctrl Pts',(1.5129078685785E-11,-27.0295179709986,
8.40164026751963));
#19133=CARTESIAN_POINT('Ctrl Pts',(4.85068927010198,-26.8545179709985,8.4016402675109));
#19134=CARTESIAN_POINT('Ctrl Pts',(7.27603390513785,-26.6795179709985,4.20082013374672));
#19135=CARTESIAN_POINT('Ctrl Pts',(9.70137854017372,-26.5045179709986,-1.74689612655491E-11));
#19136=CARTESIAN_POINT('Ctrl Pts',(7.27603390512273,-26.3295179709985,-4.20082013377291));
#19137=CARTESIAN_POINT('Ctrl Pts',(4.85068927007173,-26.1545179709986,-8.40164026752836));
#19138=CARTESIAN_POINT('Ctrl Pts',(-1.51301075899711E-11,-25.9795179709985,
-8.40164026751963));
#19139=CARTESIAN_POINT('Ctrl Pts',(-4.85068927010199,-25.8045179709985,
-8.4016402675109));
#19140=CARTESIAN_POINT('Ctrl Pts',(-7.27603390513785,-25.6295179709985,
-4.20082013374671));
#19141=CARTESIAN_POINT('Ctrl Pts',(-9.70137854017372,-25.4545179709985,
1.74701493417668E-11));
#19142=CARTESIAN_POINT('Ctrl Pts',(-7.27603390512272,-25.2795179709985,
4.20082013377292));
#19143=CARTESIAN_POINT('Ctrl Pts',(-4.85068927007173,-25.1045179709986,
8.40164026752836));
#19144=CARTESIAN_POINT('Ctrl Pts',(1.5129078685785E-11,-24.9295179709985,
8.40164026751963));
#19145=CARTESIAN_POINT('Ctrl Pts',(4.85068927010198,-24.7545179709985,8.4016402675109));
#19146=CARTESIAN_POINT('Ctrl Pts',(7.27603390513785,-24.5795179709986,4.20082013374672));
#19147=CARTESIAN_POINT('Ctrl Pts',(9.70137854017372,-24.4045179709986,-1.74689612655491E-11));
#19148=CARTESIAN_POINT('Ctrl Pts',(7.27603390512273,-24.2295179709986,-4.20082013377291));
#19149=CARTESIAN_POINT('Ctrl Pts',(4.85068927007173,-24.0545179709986,-8.40164026752836));
#19150=CARTESIAN_POINT('Ctrl Pts',(-1.51301075899711E-11,-23.8795179709986,
-8.40164026751963));
#19151=CARTESIAN_POINT('Ctrl Pts',(-4.85068927010199,-23.7045179709986,
-8.4016402675109));
#19152=CARTESIAN_POINT('Ctrl Pts',(-7.27603390513785,-23.5295179709985,
-4.20082013374671));
#19153=CARTESIAN_POINT('Ctrl Pts',(-9.70137854017372,-23.3545179709986,
1.74701493417668E-11));
#19154=CARTESIAN_POINT('Ctrl Pts',(-7.27603390512272,-23.1795179709986,
4.20082013377292));
#19155=CARTESIAN_POINT('Ctrl Pts',(-4.85068927007173,-23.0045179709986,
8.40164026752836));
#19156=CARTESIAN_POINT('Ctrl Pts',(1.5129078685785E-11,-22.8295179709986,
8.40164026751963));
#19157=CARTESIAN_POINT('Ctrl Pts',(4.85068927010198,-22.6545179709986,8.4016402675109));
#19158=CARTESIAN_POINT('Ctrl Pts',(7.27603390513785,-22.4795179709986,4.20082013374672));
#19159=CARTESIAN_POINT('Ctrl Pts',(9.70137854017372,-22.3045179709986,-1.74689612655491E-11));
#19160=CARTESIAN_POINT('Ctrl Pts',(7.27603390512273,-22.1295179709986,-4.20082013377291));
#19161=CARTESIAN_POINT('Ctrl Pts',(4.85068927007173,-21.9545179709986,-8.40164026752836));
#19162=CARTESIAN_POINT('Ctrl Pts',(-1.51301075899711E-11,-21.7795179709986,
-8.40164026751963));
#19163=CARTESIAN_POINT('Ctrl Pts',(-4.85068927010199,-21.6045179709986,
-8.4016402675109));
#19164=CARTESIAN_POINT('Ctrl Pts',(-7.27603390513785,-21.4295179709986,
-4.20082013374671));
#19165=CARTESIAN_POINT('Ctrl Pts',(-9.70137854017372,-21.2545179709986,
1.74701493417668E-11));
#19166=CARTESIAN_POINT('Ctrl Pts',(-7.27603390512272,-21.0795179709986,
4.20082013377292));
#19167=CARTESIAN_POINT('Ctrl Pts',(-4.85068927007173,-20.9045179709986,
8.40164026752836));
#19168=CARTESIAN_POINT('Ctrl Pts',(1.5129078685785E-11,-20.7295179709986,
8.40164026751963));
#19169=CARTESIAN_POINT('Ctrl Pts',(4.85068927010198,-20.5545179709986,8.4016402675109));
#19170=CARTESIAN_POINT('Ctrl Pts',(7.27603390513785,-20.3795179709986,4.20082013374672));
#19171=CARTESIAN_POINT('Ctrl Pts',(9.70137854017372,-20.2045179709986,-1.74689612655491E-11));
#19172=CARTESIAN_POINT('Ctrl Pts',(7.27603390512273,-20.0295179709986,-4.20082013377291));
#19173=CARTESIAN_POINT('Ctrl Pts',(4.85068927007173,-19.8545179709986,-8.40164026752836));
#19174=CARTESIAN_POINT('Ctrl Pts',(-1.51301075899711E-11,-19.6795179709986,
-8.40164026751963));
#19175=CARTESIAN_POINT('Ctrl Pts',(-4.85068927010199,-19.5045179709986,
-8.4016402675109));
#19176=CARTESIAN_POINT('Ctrl Pts',(-7.27603390513785,-19.3295179709986,
-4.20082013374671));
#19177=CARTESIAN_POINT('Ctrl Pts',(-9.70137854017372,-19.1545179709986,
1.74701493417668E-11));
#19178=CARTESIAN_POINT('Ctrl Pts',(-7.27603390512272,-18.9795179709986,
4.20082013377292));
#19179=CARTESIAN_POINT('Ctrl Pts',(-4.85068927007173,-18.8045179709986,
8.40164026752836));
#19180=CARTESIAN_POINT('Ctrl Pts',(1.5129078685785E-11,-18.6295179709986,
8.40164026751963));
#19181=CARTESIAN_POINT('Ctrl Pts',(4.85068927010198,-18.4545179709986,8.4016402675109));
#19182=CARTESIAN_POINT('Ctrl Pts',(7.27603390513785,-18.2795179709986,4.20082013374672));
#19183=CARTESIAN_POINT('Ctrl Pts',(9.70137854017372,-18.1045179709986,-1.74689612655491E-11));
#19184=CARTESIAN_POINT('Ctrl Pts',(7.27603390512273,-17.9295179709986,-4.20082013377291));
#19185=CARTESIAN_POINT('Ctrl Pts',(4.85068927007173,-17.7545179709986,-8.40164026752836));
#19186=CARTESIAN_POINT('Ctrl Pts',(-1.51301075899711E-11,-17.5795179709986,
-8.40164026751963));
#19187=CARTESIAN_POINT('Ctrl Pts',(-4.85068927010199,-17.4045179709986,
-8.4016402675109));
#19188=CARTESIAN_POINT('Ctrl Pts',(-7.27603390513785,-17.2295179709986,
-4.20082013374671));
#19189=CARTESIAN_POINT('Ctrl Pts',(-9.70137854017372,-17.0545179709986,
1.74701493417668E-11));
#19190=CARTESIAN_POINT('Ctrl Pts',(-7.27603390512272,-16.8795179709986,
4.20082013377292));
#19191=CARTESIAN_POINT('Ctrl Pts',(-4.85068927007173,-16.7045179709986,
8.40164026752836));
#19192=CARTESIAN_POINT('Ctrl Pts',(1.5129078685785E-11,-16.5295179709986,
8.40164026751963));
#19193=CARTESIAN_POINT('Ctrl Pts',(4.85068927010198,-16.3545179709986,8.4016402675109));
#19194=CARTESIAN_POINT('Ctrl Pts',(7.27603390513785,-16.1795179709986,4.20082013374672));
#19195=CARTESIAN_POINT('Ctrl Pts',(9.70137854017372,-16.0045179709986,-1.74689612655491E-11));
#19196=CARTESIAN_POINT('Ctrl Pts',(7.27603390512273,-15.8295179709986,-4.20082013377291));
#19197=CARTESIAN_POINT('Ctrl Pts',(4.85068927007173,-15.6545179709986,-8.40164026752836));
#19198=CARTESIAN_POINT('Ctrl Pts',(-1.51301075899711E-11,-15.4795179709986,
-8.40164026751963));
#19199=CARTESIAN_POINT('Ctrl Pts',(-4.85068927010199,-15.3045179709986,
-8.4016402675109));
#19200=CARTESIAN_POINT('Ctrl Pts',(-7.27603390513785,-15.1295179709986,
-4.20082013374671));
#19201=CARTESIAN_POINT('Ctrl Pts',(-9.70137854017372,-14.9545179709986,
1.74701493417668E-11));
#19202=CARTESIAN_POINT('Ctrl Pts',(-7.27603390512272,-14.7795179709986,
4.20082013377292));
#19203=CARTESIAN_POINT('Ctrl Pts',(-4.85068927007173,-14.6045179709986,
8.40164026752836));
#19204=CARTESIAN_POINT('Ctrl Pts',(1.5129078685785E-11,-14.4295179709986,
8.40164026751963));
#19205=CARTESIAN_POINT('Ctrl Pts',(4.85068927010198,-14.2545179709986,8.4016402675109));
#19206=CARTESIAN_POINT('Ctrl Pts',(7.27603390513785,-14.0795179709986,4.20082013374672));
#19207=CARTESIAN_POINT('Ctrl Pts',(9.70137854017372,-13.9045179709986,-1.74689612655491E-11));
#19208=CARTESIAN_POINT('Ctrl Pts',(7.27603390512273,-13.7295179709986,-4.20082013377291));
#19209=CARTESIAN_POINT('Ctrl Pts',(4.85068927007173,-13.5545179709986,-8.40164026752836));
#19210=CARTESIAN_POINT('Ctrl Pts',(-1.51301075899711E-11,-13.3795179709986,
-8.40164026751963));
#19211=CARTESIAN_POINT('Ctrl Pts',(-4.85068927010199,-13.2045179709986,
-8.4016402675109));
#19212=CARTESIAN_POINT('Ctrl Pts',(-7.27603390513785,-13.0295179709986,
-4.20082013374671));
#19213=CARTESIAN_POINT('Ctrl Pts',(-9.70137854017372,-12.8545179709986,
1.74701493417668E-11));
#19214=CARTESIAN_POINT('Ctrl Pts',(-7.27603390512272,-12.6795179709986,
4.20082013377292));
#19215=CARTESIAN_POINT('Ctrl Pts',(-4.85068927007173,-12.5045179709986,
8.40164026752836));
#19216=CARTESIAN_POINT('Ctrl Pts',(1.5129078685785E-11,-12.3295179709986,
8.40164026751963));
#19217=CARTESIAN_POINT('Ctrl Pts',(4.85068927010198,-12.1545179709986,8.4016402675109));
#19218=CARTESIAN_POINT('Ctrl Pts',(7.27603390513785,-11.9795179709986,4.20082013374672));
#19219=CARTESIAN_POINT('Ctrl Pts',(9.70137854017372,-11.8045179709986,-1.74689612655491E-11));
#19220=CARTESIAN_POINT('Ctrl Pts',(7.27603390512273,-11.6295179709986,-4.20082013377291));
#19221=CARTESIAN_POINT('Ctrl Pts',(4.85068927007173,-11.4545179709986,-8.40164026752836));
#19222=CARTESIAN_POINT('Ctrl Pts',(-1.51301075899711E-11,-11.2795179709986,
-8.40164026751963));
#19223=CARTESIAN_POINT('Ctrl Pts',(-4.85068927010199,-11.1045179709986,
-8.4016402675109));
#19224=CARTESIAN_POINT('Ctrl Pts',(-7.27603390513785,-10.9295179709986,
-4.20082013374671));
#19225=CARTESIAN_POINT('Ctrl Pts',(-9.70137854017372,-10.7545179709986,
1.74701493417668E-11));
#19226=CARTESIAN_POINT('Ctrl Pts',(-7.27603390512272,-10.5795179709986,
4.20082013377292));
#19227=CARTESIAN_POINT('Ctrl Pts',(-4.85068927007173,-10.4045179709986,
8.40164026752836));
#19228=CARTESIAN_POINT('Ctrl Pts',(1.5129078685785E-11,-10.2295179709986,
8.40164026751963));
#19229=CARTESIAN_POINT('Ctrl Pts',(4.85068927010198,-10.0545179709986,8.4016402675109));
#19230=CARTESIAN_POINT('Ctrl Pts',(7.27603390513785,-9.87951797099859,4.20082013374672));
#19231=CARTESIAN_POINT('Ctrl Pts',(9.70137854017372,-9.70451797099858,-1.74689612655491E-11));
#19232=CARTESIAN_POINT('Ctrl Pts',(7.27603390512273,-9.52951797099857,-4.20082013377291));
#19233=CARTESIAN_POINT('Ctrl Pts',(4.85068927007173,-9.3545179709986,-8.40164026752836));
#19234=CARTESIAN_POINT('Ctrl Pts',(-1.51301075899711E-11,-9.17951797099859,
-8.40164026751963));
#19235=CARTESIAN_POINT('Ctrl Pts',(-4.85068927010199,-9.00451797099858,
-8.4016402675109));
#19236=CARTESIAN_POINT('Ctrl Pts',(-7.27603390513785,-8.8295179709986,-4.20082013374671));
#19237=CARTESIAN_POINT('Ctrl Pts',(-9.70137854017372,-8.65451797099859,
1.74701493417668E-11));
#19238=CARTESIAN_POINT('Ctrl Pts',(-7.27603390512272,-8.47951797099858,
4.20082013377292));
#19239=CARTESIAN_POINT('Ctrl Pts',(-4.85068927007173,-8.3045179709986,8.40164026752836));
#19240=CARTESIAN_POINT('Ctrl Pts',(1.5129078685785E-11,-8.12951797099859,
8.40164026751963));
#19241=CARTESIAN_POINT('Ctrl Pts',(4.85068927010198,-7.95451797099859,8.4016402675109));
#19242=CARTESIAN_POINT('Ctrl Pts',(7.27603390513785,-7.7795179709986,4.20082013374672));
#19243=CARTESIAN_POINT('Ctrl Pts',(9.70137854017372,-7.60451797099859,-1.74689612655491E-11));
#19244=CARTESIAN_POINT('Ctrl Pts',(7.27603390512273,-7.42951797099858,-4.20082013377291));
#19245=CARTESIAN_POINT('Ctrl Pts',(4.85068927007173,-7.25451797099861,-8.40164026752836));
#19246=CARTESIAN_POINT('Ctrl Pts',(-1.51301075899711E-11,-7.07951797099859,
-8.40164026751963));
#19247=CARTESIAN_POINT('Ctrl Pts',(-4.85068927010199,-6.90451797099859,
-8.4016402675109));
#19248=CARTESIAN_POINT('Ctrl Pts',(-7.27603390513785,-6.72951797099858,
-4.20082013374671));
#19249=CARTESIAN_POINT('Ctrl Pts',(-9.70137854017372,-6.5545179709986,1.74701493417668E-11));
#19250=CARTESIAN_POINT('Ctrl Pts',(-7.27603390512272,-6.37951797099859,
4.20082013377292));
#19251=CARTESIAN_POINT('Ctrl Pts',(-4.85068927007173,-6.20451797099858,
8.40164026752836));
#19252=CARTESIAN_POINT('Ctrl Pts',(1.5129078685785E-11,-6.0295179709986,
8.40164026751963));
#19253=CARTESIAN_POINT('Ctrl Pts',(4.85068927010198,-5.8545179709986,8.4016402675109));
#19254=CARTESIAN_POINT('Ctrl Pts',(7.27603390513785,-5.67951797099858,4.20082013374672));
#19255=CARTESIAN_POINT('Ctrl Pts',(9.70137854017372,-5.5045179709986,-1.74689612655491E-11));
#19256=CARTESIAN_POINT('Ctrl Pts',(7.27603390512273,-5.32951797099859,-4.20082013377291));
#19257=CARTESIAN_POINT('Ctrl Pts',(4.85068927007173,-5.15451797099859,-8.40164026752836));
#19258=CARTESIAN_POINT('Ctrl Pts',(-1.51301075899711E-11,-4.9795179709986,
-8.40164026751963));
#19259=CARTESIAN_POINT('Ctrl Pts',(-4.85068927010199,-4.8045179709986,-8.4016402675109));
#19260=CARTESIAN_POINT('Ctrl Pts',(-7.27603390513785,-4.62951797099859,
-4.20082013374671));
#19261=CARTESIAN_POINT('Ctrl Pts',(-9.70137854017372,-4.45451797099861,
1.74701493417668E-11));
#19262=CARTESIAN_POINT('Ctrl Pts',(-7.27603390512272,-4.2795179709986,4.20082013377292));
#19263=CARTESIAN_POINT('Ctrl Pts',(-4.85068927007173,-4.10451797099859,
8.40164026752836));
#19264=CARTESIAN_POINT('Ctrl Pts',(1.5129078685785E-11,-3.92951797099861,
8.40164026751963));
#19265=CARTESIAN_POINT('Ctrl Pts',(4.85068927010198,-3.75451797099861,8.4016402675109));
#19266=CARTESIAN_POINT('Ctrl Pts',(7.27603390513785,-3.57951797099859,4.20082013374672));
#19267=CARTESIAN_POINT('Ctrl Pts',(9.70137854017372,-3.40451797099861,-1.74689612655491E-11));
#19268=CARTESIAN_POINT('Ctrl Pts',(7.27603390512273,-3.2295179709986,-4.20082013377291));
#19269=CARTESIAN_POINT('Ctrl Pts',(4.85068927007173,-3.0545179709986,-8.40164026752836));
#19270=CARTESIAN_POINT('Ctrl Pts',(-1.51301075899711E-11,-2.87951797099861,
-8.40164026751963));
#19271=CARTESIAN_POINT('Ctrl Pts',(-4.85068927010199,-2.70451797099861,
-8.4016402675109));
#19272=CARTESIAN_POINT('Ctrl Pts',(-7.27603390513785,-2.5295179709986,-4.20082013374671));
#19273=CARTESIAN_POINT('Ctrl Pts',(-9.70137854017372,-2.3545179709986,1.74701493417668E-11));
#19274=CARTESIAN_POINT('Ctrl Pts',(-7.27603390512272,-2.17951797099861,
4.20082013377292));
#19275=CARTESIAN_POINT('Ctrl Pts',(-4.85068927007173,-2.0045179709986,8.40164026752836));
#19276=CARTESIAN_POINT('Ctrl Pts',(1.5129078685785E-11,-1.82951797099859,
8.40164026751963));
#19277=CARTESIAN_POINT('Ctrl Pts',(4.85068927010198,-1.65451797099861,8.4016402675109));
#19278=CARTESIAN_POINT('Ctrl Pts',(7.27603390513785,-1.4795179709986,4.20082013374672));
#19279=CARTESIAN_POINT('Ctrl Pts',(9.70137854017372,-1.3045179709986,-1.74689612655491E-11));
#19280=CARTESIAN_POINT('Ctrl Pts',(7.27603390512273,-1.12951797099861,-4.20082013377291));
#19281=CARTESIAN_POINT('Ctrl Pts',(4.85068927007173,-0.954517970998605,
-8.40164026752836));
#19282=CARTESIAN_POINT('Ctrl Pts',(-1.51301075899711E-11,-0.779517970998594,
-8.40164026751963));
#19283=CARTESIAN_POINT('Ctrl Pts',(-4.85068927010199,-0.604517970998614,
-8.4016402675109));
#19284=CARTESIAN_POINT('Ctrl Pts',(-7.27603390513785,-0.429517970998605,
-4.20082013374671));
#19285=CARTESIAN_POINT('Ctrl Pts',(-9.70137854017372,-0.2545179709986,1.74701493417668E-11));
#19286=CARTESIAN_POINT('Ctrl Pts',(-7.27603390512272,-0.079517970998616,
4.20082013377292));
#19287=CARTESIAN_POINT('Ctrl Pts',(-4.85068927007173,0.0954820290013905,
8.40164026752836));
#19288=CARTESIAN_POINT('Ctrl Pts',(1.5129078685785E-11,0.270482029001401,
8.40164026751963));
#19289=CARTESIAN_POINT('Ctrl Pts',(4.85068927010198,0.445482029001381,8.4016402675109));
#19290=CARTESIAN_POINT('Ctrl Pts',(7.27603390513785,0.62048202900139,4.20082013374672));
#19291=CARTESIAN_POINT('Ctrl Pts',(9.70137854017372,0.795482029001395,-1.74689612655491E-11));
#19292=CARTESIAN_POINT('Ctrl Pts',(7.27603390512273,0.970482029001379,-4.20082013377291));
#19293=CARTESIAN_POINT('Ctrl Pts',(4.85068927007173,1.14548202900139,-8.40164026752836));
#19294=CARTESIAN_POINT('Ctrl Pts',(-1.51301075899711E-11,1.3204820290014,
-8.40164026751963));
#19295=CARTESIAN_POINT('Ctrl Pts',(-4.85068927010199,1.49548202900138,-8.4016402675109));
#19296=CARTESIAN_POINT('Ctrl Pts',(-7.27603390513785,1.67048202900139,-4.20082013374671));
#19297=CARTESIAN_POINT('Ctrl Pts',(-9.70137854017372,1.84548202900139,1.74701493417668E-11));
#19298=CARTESIAN_POINT('Ctrl Pts',(-7.27603390512272,2.0204820290014,4.20082013377292));
#19299=CARTESIAN_POINT('Ctrl Pts',(-4.85068927007173,2.19548202900138,8.40164026752836));
#19300=CARTESIAN_POINT('Ctrl Pts',(1.5129078685785E-11,2.37048202900139,
8.40164026751963));
#19301=CARTESIAN_POINT('Ctrl Pts',(4.85068927010198,2.5454820290014,8.4016402675109));
#19302=CARTESIAN_POINT('Ctrl Pts',(7.27603390513785,2.72048202900138,4.20082013374672));
#19303=CARTESIAN_POINT('Ctrl Pts',(9.70137854017372,2.89548202900139,-1.74689612655491E-11));
#19304=CARTESIAN_POINT('Ctrl Pts',(7.27603390512273,3.0704820290014,-4.20082013377291));
#19305=CARTESIAN_POINT('Ctrl Pts',(4.85068927007173,3.24548202900138,-8.40164026752836));
#19306=CARTESIAN_POINT('Ctrl Pts',(-1.51301075899711E-11,3.42048202900139,
-8.40164026751963));
#19307=CARTESIAN_POINT('Ctrl Pts',(-4.85068927010199,3.59548202900139,-8.4016402675109));
#19308=CARTESIAN_POINT('Ctrl Pts',(-7.27603390513785,3.77048202900138,-4.20082013374671));
#19309=CARTESIAN_POINT('Ctrl Pts',(-9.70137854017372,3.94548202900138,1.74701493417668E-11));
#19310=CARTESIAN_POINT('Ctrl Pts',(-7.27603390512272,4.12048202900139,4.20082013377292));
#19311=CARTESIAN_POINT('Ctrl Pts',(-4.85068927007173,4.29548202900137,8.40164026752836));
#19312=CARTESIAN_POINT('Ctrl Pts',(1.5129078685785E-11,4.47048202900138,
8.40164026751963));
#19313=CARTESIAN_POINT('Ctrl Pts',(4.85068927010198,4.64548202900139,8.4016402675109));
#19314=CARTESIAN_POINT('Ctrl Pts',(7.27603390513785,4.82048202900137,4.20082013374672));
#19315=CARTESIAN_POINT('Ctrl Pts',(9.70137854017372,4.99548202900138,-1.74689612655491E-11));
#19316=CARTESIAN_POINT('Ctrl Pts',(7.27603390512273,5.17048202900139,-4.20082013377291));
#19317=CARTESIAN_POINT('Ctrl Pts',(4.85068927007173,5.34548202900137,-8.40164026752836));
#19318=CARTESIAN_POINT('Ctrl Pts',(-1.51301075899711E-11,5.52048202900138,
-8.40164026751963));
#19319=CARTESIAN_POINT('Ctrl Pts',(-4.85068927010199,5.69548202900138,-8.4016402675109));
#19320=CARTESIAN_POINT('Ctrl Pts',(-7.27603390513785,5.87048202900137,-4.20082013374671));
#19321=CARTESIAN_POINT('Ctrl Pts',(-9.70137854017372,6.04548202900137,1.74701493417668E-11));
#19322=CARTESIAN_POINT('Ctrl Pts',(-7.27603390512272,6.22048202900138,4.20082013377292));
#19323=CARTESIAN_POINT('Ctrl Pts',(-4.85068927007173,6.39548202900136,8.40164026752836));
#19324=CARTESIAN_POINT('Ctrl Pts',(1.5129078685785E-11,6.57048202900137,
8.40164026751963));
#19325=CARTESIAN_POINT('Ctrl Pts',(4.85068927010198,6.74548202900138,8.4016402675109));
#19326=CARTESIAN_POINT('Ctrl Pts',(7.27603390513785,6.92048202900139,4.20082013374672));
#19327=CARTESIAN_POINT('Ctrl Pts',(9.70137854017372,7.09548202900137,-1.74689612655491E-11));
#19328=CARTESIAN_POINT('Ctrl Pts',(7.27603390512273,7.27048202900138,-4.20082013377291));
#19329=CARTESIAN_POINT('Ctrl Pts',(4.85068927007173,7.44548202900138,-8.40164026752836));
#19330=CARTESIAN_POINT('Ctrl Pts',(-1.51301075899711E-11,7.62048202900137,
-8.40164026751963));
#19331=CARTESIAN_POINT('Ctrl Pts',(-4.85068927010199,7.79548202900137,-8.4016402675109));
#19332=CARTESIAN_POINT('Ctrl Pts',(-7.27603390513785,7.97048202900139,-4.20082013374671));
#19333=CARTESIAN_POINT('Ctrl Pts',(-9.70137854017372,8.14548202900136,1.74701493417668E-11));
#19334=CARTESIAN_POINT('Ctrl Pts',(-7.27603390512272,8.32048202900138,4.20082013377292));
#19335=CARTESIAN_POINT('Ctrl Pts',(-4.85068927007173,8.49548202900138,8.40164026752836));
#19336=CARTESIAN_POINT('Ctrl Pts',(1.5129078685785E-11,8.67048202900136,
8.40164026751963));
#19337=CARTESIAN_POINT('Ctrl Pts',(4.85068927010198,8.84548202900137,8.4016402675109));
#19338=CARTESIAN_POINT('Ctrl Pts',(7.27603390513785,9.02048202900138,4.20082013374672));
#19339=CARTESIAN_POINT('Ctrl Pts',(9.70137854017372,9.19548202900136,-1.74689612655491E-11));
#19340=CARTESIAN_POINT('Ctrl Pts',(7.27603390512273,9.37048202900137,-4.20082013377291));
#19341=CARTESIAN_POINT('Ctrl Pts',(4.85068927007173,9.54548202900137,-8.40164026752836));
#19342=CARTESIAN_POINT('Ctrl Pts',(-1.51301075899711E-11,9.72048202900136,
-8.40164026751963));
#19343=CARTESIAN_POINT('Ctrl Pts',(-4.85068927010199,9.89548202900136,-8.4016402675109));
#19344=CARTESIAN_POINT('Ctrl Pts',(-7.27603390513785,10.0704820290014,-4.20082013374671));
#19345=CARTESIAN_POINT('Ctrl Pts',(-9.70137854017372,10.2454820290014,1.74701493417668E-11));
#19346=CARTESIAN_POINT('Ctrl Pts',(-7.27603390512272,10.4204820290014,4.20082013377292));
#19347=CARTESIAN_POINT('Ctrl Pts',(-4.85068927007173,10.5954820290014,8.40164026752836));
#19348=CARTESIAN_POINT('Ctrl Pts',(1.5129078685785E-11,10.7704820290014,
8.40164026751963));
#19349=CARTESIAN_POINT('Ctrl Pts',(4.85068927010198,10.9454820290014,8.4016402675109));
#19350=CARTESIAN_POINT('Ctrl Pts',(7.27603390513785,11.1204820290014,4.20082013374672));
#19351=CARTESIAN_POINT('Ctrl Pts',(9.70137854017372,11.2954820290014,-1.74689612655491E-11));
#19352=CARTESIAN_POINT('Ctrl Pts',(7.27603390512273,11.4704820290014,-4.20082013377291));
#19353=CARTESIAN_POINT('Ctrl Pts',(4.85068927007173,11.6454820290014,-8.40164026752836));
#19354=CARTESIAN_POINT('Ctrl Pts',(-1.51301075899711E-11,11.8204820290014,
-8.40164026751963));
#19355=CARTESIAN_POINT('Ctrl Pts',(-4.85068927010199,11.9954820290014,-8.4016402675109));
#19356=CARTESIAN_POINT('Ctrl Pts',(-7.27603390513785,12.1704820290014,-4.20082013374671));
#19357=CARTESIAN_POINT('Ctrl Pts',(-9.70137854017372,12.3454820290014,1.74701493417668E-11));
#19358=CARTESIAN_POINT('Ctrl Pts',(-7.27603390512272,12.5204820290014,4.20082013377292));
#19359=CARTESIAN_POINT('Ctrl Pts',(-4.85068927007173,12.6954820290014,8.40164026752836));
#19360=CARTESIAN_POINT('Ctrl Pts',(1.5129078685785E-11,12.8704820290014,
8.40164026751963));
#19361=CARTESIAN_POINT('Ctrl Pts',(4.85068927010198,13.0454820290013,8.4016402675109));
#19362=CARTESIAN_POINT('Ctrl Pts',(7.27603390513785,13.2204820290014,4.20082013374672));
#19363=CARTESIAN_POINT('Ctrl Pts',(9.70137854017372,13.3954820290014,-1.74689612655491E-11));
#19364=CARTESIAN_POINT('Ctrl Pts',(7.27603390512273,13.5704820290014,-4.20082013377291));
#19365=CARTESIAN_POINT('Ctrl Pts',(4.85068927007173,13.7454820290014,-8.40164026752836));
#19366=CARTESIAN_POINT('Ctrl Pts',(-1.51301075899711E-11,13.9204820290014,
-8.40164026751963));
#19367=CARTESIAN_POINT('Ctrl Pts',(-4.85068927010199,14.0954820290013,-8.4016402675109));
#19368=CARTESIAN_POINT('Ctrl Pts',(-7.27603390513785,14.2704820290014,-4.20082013374671));
#19369=CARTESIAN_POINT('Ctrl Pts',(-9.70137854017372,14.4454820290014,1.74701493417668E-11));
#19370=CARTESIAN_POINT('Ctrl Pts',(-7.27603390512272,14.6204820290013,4.20082013377292));
#19371=CARTESIAN_POINT('Ctrl Pts',(-4.85068927007173,14.7954820290014,8.40164026752836));
#19372=CARTESIAN_POINT('Ctrl Pts',(1.5129078685785E-11,14.9704820290014,
8.40164026751963));
#19373=CARTESIAN_POINT('Ctrl Pts',(4.85068927010198,15.1454820290013,8.4016402675109));
#19374=CARTESIAN_POINT('Ctrl Pts',(7.27603390513785,15.3204820290014,4.20082013374672));
#19375=CARTESIAN_POINT('Ctrl Pts',(9.70137854017372,15.4954820290014,-1.74689612655491E-11));
#19376=CARTESIAN_POINT('Ctrl Pts',(7.27603390512273,15.6704820290014,-4.20082013377291));
#19377=CARTESIAN_POINT('Ctrl Pts',(4.85068927007173,15.8454820290013,-8.40164026752836));
#19378=CARTESIAN_POINT('Ctrl Pts',(-1.51301075899711E-11,16.0204820290014,
-8.40164026751963));
#19379=CARTESIAN_POINT('Ctrl Pts',(-4.85068927010199,16.1954820290014,-8.4016402675109));
#19380=CARTESIAN_POINT('Ctrl Pts',(-7.27603390513785,16.3704820290014,-4.20082013374671));
#19381=CARTESIAN_POINT('Ctrl Pts',(-9.70137854017372,16.5454820290013,1.74701493417668E-11));
#19382=CARTESIAN_POINT('Ctrl Pts',(-7.27603390512272,16.7204820290014,4.20082013377292));
#19383=CARTESIAN_POINT('Ctrl Pts',(-4.85068927007173,16.8954820290013,8.40164026752836));
#19384=CARTESIAN_POINT('Ctrl Pts',(1.5129078685785E-11,17.0704820290014,
8.40164026751963));
#19385=CARTESIAN_POINT('Ctrl Pts',(4.85068927010198,17.2454820290014,8.4016402675109));
#19386=CARTESIAN_POINT('Ctrl Pts',(7.27603390513785,17.4204820290013,4.20082013374672));
#19387=CARTESIAN_POINT('Ctrl Pts',(9.70137854017372,17.5954820290013,-1.74689612655491E-11));
#19388=CARTESIAN_POINT('Ctrl Pts',(7.27603390512273,17.7704820290014,-4.20082013377291));
#19389=CARTESIAN_POINT('Ctrl Pts',(4.85068927007173,17.9454820290013,-8.40164026752836));
#19390=CARTESIAN_POINT('Ctrl Pts',(-1.51301075899711E-11,18.1204820290014,
-8.40164026751963));
#19391=CARTESIAN_POINT('Ctrl Pts',(-4.85068927010199,18.2954820290014,-8.4016402675109));
#19392=CARTESIAN_POINT('Ctrl Pts',(-7.27603390513785,18.4704820290013,-4.20082013374671));
#19393=CARTESIAN_POINT('Ctrl Pts',(-9.70137854017372,18.6454820290013,1.74701493417668E-11));
#19394=CARTESIAN_POINT('Ctrl Pts',(-7.27603390512272,18.8204820290014,4.20082013377292));
#19395=CARTESIAN_POINT('Ctrl Pts',(-4.85068927007173,18.9954820290013,8.40164026752836));
#19396=CARTESIAN_POINT('Ctrl Pts',(1.5129078685785E-11,19.1704820290013,
8.40164026751963));
#19397=CARTESIAN_POINT('Ctrl Pts',(4.85068927010198,19.3454820290014,8.4016402675109));
#19398=CARTESIAN_POINT('Ctrl Pts',(7.27603390513785,19.5204820290013,4.20082013374672));
#19399=CARTESIAN_POINT('Ctrl Pts',(9.70137854017372,19.6954820290013,-1.74689612655491E-11));
#19400=CARTESIAN_POINT('Ctrl Pts',(7.27603390512273,19.8704820290014,-4.20082013377291));
#19401=CARTESIAN_POINT('Ctrl Pts',(4.85068927007173,20.0454820290014,-8.40164026752836));
#19402=CARTESIAN_POINT('Ctrl Pts',(-1.51301075899711E-11,20.2204820290013,
-8.40164026751963));
#19403=CARTESIAN_POINT('Ctrl Pts',(-4.85068927010199,20.3954820290014,-8.4016402675109));
#19404=CARTESIAN_POINT('Ctrl Pts',(-7.27603390513785,20.5704820290014,-4.20082013374671));
#19405=CARTESIAN_POINT('Ctrl Pts',(-9.70137854017372,20.7454820290013,1.74701493417668E-11));
#19406=CARTESIAN_POINT('Ctrl Pts',(-7.27603390512272,20.9204820290013,4.20082013377292));
#19407=CARTESIAN_POINT('Ctrl Pts',(-4.85068927007173,21.0954820290014,8.40164026752836));
#19408=CARTESIAN_POINT('Ctrl Pts',(1.5129078685785E-11,21.2704820290013,
8.40164026751963));
#19409=CARTESIAN_POINT('Ctrl Pts',(4.85068927010198,21.4454820290013,8.4016402675109));
#19410=CARTESIAN_POINT('Ctrl Pts',(7.27603390513785,21.6204820290014,4.20082013374672));
#19411=CARTESIAN_POINT('Ctrl Pts',(9.70137854017372,21.7954820290013,-1.74689612655491E-11));
#19412=CARTESIAN_POINT('Ctrl Pts',(7.27603390512273,21.9704820290013,-4.20082013377291));
#19413=CARTESIAN_POINT('Ctrl Pts',(4.85068927007173,22.1454820290013,-8.40164026752836));
#19414=CARTESIAN_POINT('Ctrl Pts',(-1.51301075899711E-11,22.3204820290013,
-8.40164026751963));
#19415=CARTESIAN_POINT('Ctrl Pts',(-4.85068927010199,22.4954820290013,-8.4016402675109));
#19416=CARTESIAN_POINT('Ctrl Pts',(-7.27603390513785,22.6704820290013,-4.20082013374671));
#19417=CARTESIAN_POINT('Ctrl Pts',(-9.70137854017372,22.8454820290013,1.74701493417668E-11));
#19418=CARTESIAN_POINT('Ctrl Pts',(-7.27603390512272,23.0204820290013,4.20082013377292));
#19419=CARTESIAN_POINT('Ctrl Pts',(-4.85068927007173,23.1954820290013,8.40164026752836));
#19420=CARTESIAN_POINT('Ctrl Pts',(1.5129078685785E-11,23.3704820290013,
8.40164026751963));
#19421=CARTESIAN_POINT('Ctrl Pts',(4.85068927010198,23.5454820290013,8.4016402675109));
#19422=CARTESIAN_POINT('Ctrl Pts',(7.27603390513785,23.7204820290013,4.20082013374672));
#19423=CARTESIAN_POINT('Ctrl Pts',(9.70137854017372,23.8954820290013,-1.74689612655491E-11));
#19424=CARTESIAN_POINT('Ctrl Pts',(7.27603390512273,24.0704820290013,-4.20082013377291));
#19425=CARTESIAN_POINT('Ctrl Pts',(4.85068927007173,24.2454820290013,-8.40164026752836));
#19426=CARTESIAN_POINT('Ctrl Pts',(-1.51301075899711E-11,24.4204820290013,
-8.40164026751963));
#19427=CARTESIAN_POINT('Ctrl Pts',(-4.85068927010199,24.5954820290013,-8.4016402675109));
#19428=CARTESIAN_POINT('Ctrl Pts',(-7.27603390513785,24.7704820290013,-4.20082013374671));
#19429=CARTESIAN_POINT('Ctrl Pts',(-9.70137854017372,24.9454820290013,1.74701493417668E-11));
#19430=CARTESIAN_POINT('Ctrl Pts',(-7.27603390512272,25.1204820290013,4.20082013377292));
#19431=CARTESIAN_POINT('Ctrl Pts',(-4.85068927007173,25.2954820290013,8.40164026752836));
#19432=CARTESIAN_POINT('Ctrl Pts',(1.5129078685785E-11,25.4704820290013,
8.40164026751963));
#19433=CARTESIAN_POINT('Ctrl Pts',(4.85068927010198,25.6454820290013,8.4016402675109));
#19434=CARTESIAN_POINT('Ctrl Pts',(7.27603390513785,25.8204820290013,4.20082013374672));
#19435=CARTESIAN_POINT('Ctrl Pts',(9.70137854017372,25.9954820290013,-1.74689612655491E-11));
#19436=CARTESIAN_POINT('Ctrl Pts',(7.27603390512273,26.1704820290013,-4.20082013377291));
#19437=CARTESIAN_POINT('Ctrl Pts',(4.85068927007173,26.3454820290013,-8.40164026752836));
#19438=CARTESIAN_POINT('Ctrl Pts',(-1.51301075899711E-11,26.5204820290013,
-8.40164026751963));
#19439=CARTESIAN_POINT('Ctrl Pts',(-1.51301029103127E-11,-143.579519323734,
-8.40163766893887));
#19440=CARTESIAN_POINT('Ctrl Pts',(-4.85068776981069,-143.404519323734,
-8.40163766893014));
#19441=CARTESIAN_POINT('Ctrl Pts',(-7.2760316547009,-143.229519323734,-4.20081883445633));
#19442=CARTESIAN_POINT('Ctrl Pts',(-9.70137553959111,-143.054519323734,
1.74701439383464E-11));
#19443=CARTESIAN_POINT('Ctrl Pts',(-7.27603165468577,-142.879519323734,
4.20081883448254));
#19444=CARTESIAN_POINT('Ctrl Pts',(-4.85068776978043,-142.704519323734,
8.40163766894761));
#19445=CARTESIAN_POINT('Ctrl Pts',(1.51290740064448E-11,-142.529519323734,
8.40163766893887));
#19446=CARTESIAN_POINT('Ctrl Pts',(4.85068776981068,-142.354519323734,8.40163766893014));
#19447=CARTESIAN_POINT('Ctrl Pts',(7.2760316547009,-142.179519323734,4.20081883445634));
#19448=CARTESIAN_POINT('Ctrl Pts',(9.70137553959111,-142.004519323734,-1.74689558624962E-11));
#19449=CARTESIAN_POINT('Ctrl Pts',(7.27603165468577,-141.829519323734,-4.20081883448253));
#19450=CARTESIAN_POINT('Ctrl Pts',(4.85068776978043,-141.654519323734,-8.4016376689476));
#19451=CARTESIAN_POINT('Ctrl Pts',(-1.51301029103127E-11,-141.479519323734,
-8.40163766893887));
#19452=CARTESIAN_POINT('Ctrl Pts',(-4.85068776981069,-141.304519323734,
-8.40163766893014));
#19453=CARTESIAN_POINT('Ctrl Pts',(-7.2760316547009,-141.129519323734,-4.20081883445633));
#19454=CARTESIAN_POINT('Ctrl Pts',(-9.70137553959111,-140.954519323734,
1.74701439383464E-11));
#19455=CARTESIAN_POINT('Ctrl Pts',(-7.27603165468577,-140.779519323734,
4.20081883448254));
#19456=CARTESIAN_POINT('Ctrl Pts',(-4.85068776978043,-140.604519323734,
8.40163766894761));
#19457=CARTESIAN_POINT('Ctrl Pts',(1.51290740064448E-11,-140.429519323734,
8.40163766893887));
#19458=CARTESIAN_POINT('Ctrl Pts',(4.85068776981068,-140.254519323734,8.40163766893014));
#19459=CARTESIAN_POINT('Ctrl Pts',(7.2760316547009,-140.079519323734,4.20081883445634));
#19460=CARTESIAN_POINT('Ctrl Pts',(9.70137553959111,-139.904519323734,-1.74689558624962E-11));
#19461=CARTESIAN_POINT('Ctrl Pts',(7.27603165468577,-139.729519323734,-4.20081883448253));
#19462=CARTESIAN_POINT('Ctrl Pts',(4.85068776978043,-139.554519323734,-8.4016376689476));
#19463=CARTESIAN_POINT('Ctrl Pts',(-1.51301029103127E-11,-139.379519323734,
-8.40163766893887));
#19464=CARTESIAN_POINT('Ctrl Pts',(-4.85068776981069,-139.204519323734,
-8.40163766893014));
#19465=CARTESIAN_POINT('Ctrl Pts',(-7.2760316547009,-139.029519323734,-4.20081883445633));
#19466=CARTESIAN_POINT('Ctrl Pts',(-9.70137553959111,-138.854519323734,
1.74701439383464E-11));
#19467=CARTESIAN_POINT('Ctrl Pts',(-7.27603165468577,-138.679519323734,
4.20081883448254));
#19468=CARTESIAN_POINT('Ctrl Pts',(-4.85068776978043,-138.504519323734,
8.40163766894761));
#19469=CARTESIAN_POINT('Ctrl Pts',(1.51290740064448E-11,-138.329519323734,
8.40163766893887));
#19470=CARTESIAN_POINT('Ctrl Pts',(4.85068776981068,-138.154519323734,8.40163766893014));
#19471=CARTESIAN_POINT('Ctrl Pts',(7.2760316547009,-137.979519323734,4.20081883445634));
#19472=CARTESIAN_POINT('Ctrl Pts',(9.70137553959111,-137.804519323734,-1.74689558624962E-11));
#19473=CARTESIAN_POINT('Ctrl Pts',(7.27603165468577,-137.629519323734,-4.20081883448253));
#19474=CARTESIAN_POINT('Ctrl Pts',(4.85068776978043,-137.454519323734,-8.4016376689476));
#19475=CARTESIAN_POINT('Ctrl Pts',(-1.51301029103127E-11,-137.279519323734,
-8.40163766893887));
#19476=CARTESIAN_POINT('Ctrl Pts',(-4.85068776981069,-137.104519323734,
-8.40163766893014));
#19477=CARTESIAN_POINT('Ctrl Pts',(-7.2760316547009,-136.929519323734,-4.20081883445633));
#19478=CARTESIAN_POINT('Ctrl Pts',(-9.70137553959111,-136.754519323734,
1.74701439383464E-11));
#19479=CARTESIAN_POINT('Ctrl Pts',(-7.27603165468577,-136.579519323734,
4.20081883448254));
#19480=CARTESIAN_POINT('Ctrl Pts',(-4.85068776978043,-136.404519323734,
8.40163766894761));
#19481=CARTESIAN_POINT('Ctrl Pts',(1.51290740064448E-11,-136.229519323734,
8.40163766893887));
#19482=CARTESIAN_POINT('Ctrl Pts',(4.85068776981068,-136.054519323734,8.40163766893014));
#19483=CARTESIAN_POINT('Ctrl Pts',(7.2760316547009,-135.879519323734,4.20081883445634));
#19484=CARTESIAN_POINT('Ctrl Pts',(9.70137553959111,-135.704519323734,-1.74689558624962E-11));
#19485=CARTESIAN_POINT('Ctrl Pts',(7.27603165468577,-135.529519323734,-4.20081883448253));
#19486=CARTESIAN_POINT('Ctrl Pts',(4.85068776978043,-135.354519323734,-8.4016376689476));
#19487=CARTESIAN_POINT('Ctrl Pts',(-1.51301029103127E-11,-135.179519323734,
-8.40163766893887));
#19488=CARTESIAN_POINT('Ctrl Pts',(-4.85068776981069,-135.004519323734,
-8.40163766893014));
#19489=CARTESIAN_POINT('Ctrl Pts',(-7.2760316547009,-134.829519323734,-4.20081883445633));
#19490=CARTESIAN_POINT('Ctrl Pts',(-9.70137553959111,-134.654519323734,
1.74701439383464E-11));
#19491=CARTESIAN_POINT('Ctrl Pts',(-7.27603165468577,-134.479519323734,
4.20081883448254));
#19492=CARTESIAN_POINT('Ctrl Pts',(-4.85068776978043,-134.304519323734,
8.40163766894761));
#19493=CARTESIAN_POINT('Ctrl Pts',(1.51290740064448E-11,-134.129519323734,
8.40163766893887));
#19494=CARTESIAN_POINT('Ctrl Pts',(4.85068776981068,-133.954519323734,8.40163766893014));
#19495=CARTESIAN_POINT('Ctrl Pts',(7.2760316547009,-133.779519323734,4.20081883445634));
#19496=CARTESIAN_POINT('Ctrl Pts',(9.70137553959111,-133.604519323734,-1.74689558624962E-11));
#19497=CARTESIAN_POINT('Ctrl Pts',(7.27603165468577,-133.429519323734,-4.20081883448253));
#19498=CARTESIAN_POINT('Ctrl Pts',(4.85068776978043,-133.254519323734,-8.4016376689476));
#19499=CARTESIAN_POINT('Ctrl Pts',(-1.51301029103127E-11,-133.079519323734,
-8.40163766893887));
#19500=CARTESIAN_POINT('Ctrl Pts',(-4.85068776981069,-132.904519323734,
-8.40163766893014));
#19501=CARTESIAN_POINT('Ctrl Pts',(-7.2760316547009,-132.729519323734,-4.20081883445633));
#19502=CARTESIAN_POINT('Ctrl Pts',(-9.70137553959111,-132.554519323734,
1.74701439383464E-11));
#19503=CARTESIAN_POINT('Ctrl Pts',(-7.27603165468577,-132.379519323734,
4.20081883448254));
#19504=CARTESIAN_POINT('Ctrl Pts',(-4.85068776978043,-132.204519323734,
8.40163766894761));
#19505=CARTESIAN_POINT('Ctrl Pts',(1.51290740064448E-11,-132.029519323734,
8.40163766893887));
#19506=CARTESIAN_POINT('Ctrl Pts',(4.85068776981068,-131.854519323734,8.40163766893014));
#19507=CARTESIAN_POINT('Ctrl Pts',(7.2760316547009,-131.679519323734,4.20081883445634));
#19508=CARTESIAN_POINT('Ctrl Pts',(9.70137553959111,-131.504519323734,-1.74689558624962E-11));
#19509=CARTESIAN_POINT('Ctrl Pts',(7.27603165468577,-131.329519323734,-4.20081883448253));
#19510=CARTESIAN_POINT('Ctrl Pts',(4.85068776978043,-131.154519323734,-8.4016376689476));
#19511=CARTESIAN_POINT('Ctrl Pts',(-1.51301029103127E-11,-130.979519323734,
-8.40163766893887));
#19512=CARTESIAN_POINT('Ctrl Pts',(-4.85068776981069,-130.804519323734,
-8.40163766893014));
#19513=CARTESIAN_POINT('Ctrl Pts',(-7.2760316547009,-130.629519323734,-4.20081883445633));
#19514=CARTESIAN_POINT('Ctrl Pts',(-9.70137553959111,-130.454519323734,
1.74701439383464E-11));
#19515=CARTESIAN_POINT('Ctrl Pts',(-7.27603165468577,-130.279519323734,
4.20081883448254));
#19516=CARTESIAN_POINT('Ctrl Pts',(-4.85068776978043,-130.104519323734,
8.40163766894761));
#19517=CARTESIAN_POINT('Ctrl Pts',(1.51290740064448E-11,-129.929519323734,
8.40163766893887));
#19518=CARTESIAN_POINT('Ctrl Pts',(4.85068776981068,-129.754519323734,8.40163766893014));
#19519=CARTESIAN_POINT('Ctrl Pts',(7.2760316547009,-129.579519323734,4.20081883445634));
#19520=CARTESIAN_POINT('Ctrl Pts',(9.70137553959111,-129.404519323734,-1.74689558624962E-11));
#19521=CARTESIAN_POINT('Ctrl Pts',(7.27603165468577,-129.229519323734,-4.20081883448253));
#19522=CARTESIAN_POINT('Ctrl Pts',(4.85068776978043,-129.054519323734,-8.4016376689476));
#19523=CARTESIAN_POINT('Ctrl Pts',(-1.51301029103127E-11,-128.879519323734,
-8.40163766893887));
#19524=CARTESIAN_POINT('Ctrl Pts',(-4.85068776981069,-128.704519323734,
-8.40163766893014));
#19525=CARTESIAN_POINT('Ctrl Pts',(-7.2760316547009,-128.529519323734,-4.20081883445633));
#19526=CARTESIAN_POINT('Ctrl Pts',(-9.70137553959111,-128.354519323734,
1.74701439383464E-11));
#19527=CARTESIAN_POINT('Ctrl Pts',(-7.27603165468577,-128.179519323734,
4.20081883448254));
#19528=CARTESIAN_POINT('Ctrl Pts',(-4.85068776978043,-128.004519323734,
8.40163766894761));
#19529=CARTESIAN_POINT('Ctrl Pts',(1.51290740064448E-11,-127.829519323734,
8.40163766893887));
#19530=CARTESIAN_POINT('Ctrl Pts',(4.85068776981068,-127.654519323734,8.40163766893014));
#19531=CARTESIAN_POINT('Ctrl Pts',(7.2760316547009,-127.479519323734,4.20081883445634));
#19532=CARTESIAN_POINT('Ctrl Pts',(9.70137553959111,-127.304519323734,-1.74689558624962E-11));
#19533=CARTESIAN_POINT('Ctrl Pts',(7.27603165468577,-127.129519323734,-4.20081883448253));
#19534=CARTESIAN_POINT('Ctrl Pts',(4.85068776978043,-126.954519323734,-8.4016376689476));
#19535=CARTESIAN_POINT('Ctrl Pts',(-1.51301029103127E-11,-126.779519323734,
-8.40163766893887));
#19536=CARTESIAN_POINT('Ctrl Pts',(-4.85068776981069,-126.604519323734,
-8.40163766893014));
#19537=CARTESIAN_POINT('Ctrl Pts',(-7.2760316547009,-126.429519323734,-4.20081883445633));
#19538=CARTESIAN_POINT('Ctrl Pts',(-9.70137553959111,-126.254519323734,
1.74701439383464E-11));
#19539=CARTESIAN_POINT('Ctrl Pts',(-7.27603165468577,-126.079519323734,
4.20081883448254));
#19540=CARTESIAN_POINT('Ctrl Pts',(-4.85068776978043,-125.904519323734,
8.40163766894761));
#19541=CARTESIAN_POINT('Ctrl Pts',(1.51290740064448E-11,-125.729519323734,
8.40163766893887));
#19542=CARTESIAN_POINT('Ctrl Pts',(4.85068776981068,-125.554519323734,8.40163766893014));
#19543=CARTESIAN_POINT('Ctrl Pts',(7.2760316547009,-125.379519323734,4.20081883445634));
#19544=CARTESIAN_POINT('Ctrl Pts',(9.70137553959111,-125.204519323734,-1.74689558624962E-11));
#19545=CARTESIAN_POINT('Ctrl Pts',(7.27603165468577,-125.029519323734,-4.20081883448253));
#19546=CARTESIAN_POINT('Ctrl Pts',(4.85068776978043,-124.854519323734,-8.4016376689476));
#19547=CARTESIAN_POINT('Ctrl Pts',(-1.51301029103127E-11,-124.679519323734,
-8.40163766893887));
#19548=CARTESIAN_POINT('Ctrl Pts',(-4.85068776981069,-124.504519323734,
-8.40163766893014));
#19549=CARTESIAN_POINT('Ctrl Pts',(-7.2760316547009,-124.329519323734,-4.20081883445633));
#19550=CARTESIAN_POINT('Ctrl Pts',(-9.70137553959111,-124.154519323734,
1.74701439383464E-11));
#19551=CARTESIAN_POINT('Ctrl Pts',(-7.27603165468577,-123.979519323734,
4.20081883448254));
#19552=CARTESIAN_POINT('Ctrl Pts',(-4.85068776978043,-123.804519323734,
8.40163766894761));
#19553=CARTESIAN_POINT('Ctrl Pts',(1.51290740064448E-11,-123.629519323734,
8.40163766893887));
#19554=CARTESIAN_POINT('Ctrl Pts',(4.85068776981068,-123.454519323734,8.40163766893014));
#19555=CARTESIAN_POINT('Ctrl Pts',(7.2760316547009,-123.279519323734,4.20081883445634));
#19556=CARTESIAN_POINT('Ctrl Pts',(9.70137553959111,-123.104519323734,-1.74689558624962E-11));
#19557=CARTESIAN_POINT('Ctrl Pts',(7.27603165468577,-122.929519323734,-4.20081883448253));
#19558=CARTESIAN_POINT('Ctrl Pts',(4.85068776978043,-122.754519323734,-8.4016376689476));
#19559=CARTESIAN_POINT('Ctrl Pts',(-1.51301029103127E-11,-122.579519323734,
-8.40163766893887));
#19560=CARTESIAN_POINT('Ctrl Pts',(-4.85068776981069,-122.404519323734,
-8.40163766893014));
#19561=CARTESIAN_POINT('Ctrl Pts',(-7.2760316547009,-122.229519323734,-4.20081883445633));
#19562=CARTESIAN_POINT('Ctrl Pts',(-9.70137553959111,-122.054519323734,
1.74701439383464E-11));
#19563=CARTESIAN_POINT('Ctrl Pts',(-7.27603165468577,-121.879519323734,
4.20081883448254));
#19564=CARTESIAN_POINT('Ctrl Pts',(-4.85068776978043,-121.704519323734,
8.40163766894761));
#19565=CARTESIAN_POINT('Ctrl Pts',(1.51290740064448E-11,-121.529519323734,
8.40163766893887));
#19566=CARTESIAN_POINT('Ctrl Pts',(4.85068776981068,-121.354519323734,8.40163766893014));
#19567=CARTESIAN_POINT('Ctrl Pts',(7.2760316547009,-121.179519323734,4.20081883445634));
#19568=CARTESIAN_POINT('Ctrl Pts',(9.70137553959111,-121.004519323734,-1.74689558624962E-11));
#19569=CARTESIAN_POINT('Ctrl Pts',(7.27603165468577,-120.829519323734,-4.20081883448253));
#19570=CARTESIAN_POINT('Ctrl Pts',(4.85068776978043,-120.654519323734,-8.4016376689476));
#19571=CARTESIAN_POINT('Ctrl Pts',(-1.51301029103127E-11,-120.479519323734,
-8.40163766893887));
#19572=CARTESIAN_POINT('Ctrl Pts',(-4.85068776981069,-120.304519323734,
-8.40163766893014));
#19573=CARTESIAN_POINT('Ctrl Pts',(-7.2760316547009,-120.129519323734,-4.20081883445633));
#19574=CARTESIAN_POINT('Ctrl Pts',(-9.70137553959111,-119.954519323734,
1.74701439383464E-11));
#19575=CARTESIAN_POINT('Ctrl Pts',(-7.27603165468577,-119.779519323734,
4.20081883448254));
#19576=CARTESIAN_POINT('Ctrl Pts',(-4.85068776978043,-119.604519323734,
8.40163766894761));
#19577=CARTESIAN_POINT('Ctrl Pts',(1.51290740064448E-11,-119.429519323734,
8.40163766893887));
#19578=CARTESIAN_POINT('Ctrl Pts',(4.85068776981068,-119.254519323734,8.40163766893014));
#19579=CARTESIAN_POINT('Ctrl Pts',(7.2760316547009,-119.079519323734,4.20081883445634));
#19580=CARTESIAN_POINT('Ctrl Pts',(9.70137553959111,-118.904519323734,-1.74689558624962E-11));
#19581=CARTESIAN_POINT('Ctrl Pts',(7.27603165468577,-118.729519323734,-4.20081883448253));
#19582=CARTESIAN_POINT('Ctrl Pts',(4.85068776978043,-118.554519323734,-8.4016376689476));
#19583=CARTESIAN_POINT('Ctrl Pts',(-1.51301029103127E-11,-118.379519323734,
-8.40163766893887));
#19584=CARTESIAN_POINT('Ctrl Pts',(-4.85068776981069,-118.204519323734,
-8.40163766893014));
#19585=CARTESIAN_POINT('Ctrl Pts',(-7.2760316547009,-118.029519323734,-4.20081883445633));
#19586=CARTESIAN_POINT('Ctrl Pts',(-9.70137553959111,-117.854519323734,
1.74701439383464E-11));
#19587=CARTESIAN_POINT('Ctrl Pts',(-7.27603165468577,-117.679519323734,
4.20081883448254));
#19588=CARTESIAN_POINT('Ctrl Pts',(-4.85068776978043,-117.504519323734,
8.40163766894761));
#19589=CARTESIAN_POINT('Ctrl Pts',(1.51290740064448E-11,-117.329519323734,
8.40163766893887));
#19590=CARTESIAN_POINT('Ctrl Pts',(4.85068776981068,-117.154519323734,8.40163766893014));
#19591=CARTESIAN_POINT('Ctrl Pts',(7.2760316547009,-116.979519323734,4.20081883445634));
#19592=CARTESIAN_POINT('Ctrl Pts',(9.70137553959111,-116.804519323734,-1.74689558624962E-11));
#19593=CARTESIAN_POINT('Ctrl Pts',(7.27603165468577,-116.629519323734,-4.20081883448253));
#19594=CARTESIAN_POINT('Ctrl Pts',(4.85068776978043,-116.454519323734,-8.4016376689476));
#19595=CARTESIAN_POINT('Ctrl Pts',(-1.51301029103127E-11,-116.279519323734,
-8.40163766893887));
#19596=CARTESIAN_POINT('Ctrl Pts',(-4.85068776981069,-116.104519323734,
-8.40163766893014));
#19597=CARTESIAN_POINT('Ctrl Pts',(-7.2760316547009,-115.929519323734,-4.20081883445633));
#19598=CARTESIAN_POINT('Ctrl Pts',(-9.70137553959111,-115.754519323734,
1.74701439383464E-11));
#19599=CARTESIAN_POINT('Ctrl Pts',(-7.27603165468577,-115.579519323734,
4.20081883448254));
#19600=CARTESIAN_POINT('Ctrl Pts',(-4.85068776978043,-115.404519323734,
8.40163766894761));
#19601=CARTESIAN_POINT('Ctrl Pts',(1.51290740064448E-11,-115.229519323734,
8.40163766893887));
#19602=CARTESIAN_POINT('Ctrl Pts',(4.85068776981068,-115.054519323734,8.40163766893014));
#19603=CARTESIAN_POINT('Ctrl Pts',(7.2760316547009,-114.879519323734,4.20081883445634));
#19604=CARTESIAN_POINT('Ctrl Pts',(9.70137553959111,-114.704519323734,-1.74689558624962E-11));
#19605=CARTESIAN_POINT('Ctrl Pts',(7.27603165468577,-114.529519323734,-4.20081883448253));
#19606=CARTESIAN_POINT('Ctrl Pts',(4.85068776978043,-114.354519323734,-8.4016376689476));
#19607=CARTESIAN_POINT('Ctrl Pts',(-1.51301029103127E-11,-114.179519323734,
-8.40163766893887));
#19608=CARTESIAN_POINT('Ctrl Pts',(-4.85068776981069,-114.004519323734,
-8.40163766893014));
#19609=CARTESIAN_POINT('Ctrl Pts',(-7.2760316547009,-113.829519323734,-4.20081883445633));
#19610=CARTESIAN_POINT('Ctrl Pts',(-9.70137553959111,-113.654519323734,
1.74701439383464E-11));
#19611=CARTESIAN_POINT('Ctrl Pts',(-7.27603165468577,-113.479519323734,
4.20081883448254));
#19612=CARTESIAN_POINT('Ctrl Pts',(-4.85068776978043,-113.304519323734,
8.40163766894761));
#19613=CARTESIAN_POINT('Ctrl Pts',(1.51290740064448E-11,-113.129519323734,
8.40163766893887));
#19614=CARTESIAN_POINT('Ctrl Pts',(4.85068776981068,-112.954519323734,8.40163766893014));
#19615=CARTESIAN_POINT('Ctrl Pts',(7.2760316547009,-112.779519323734,4.20081883445634));
#19616=CARTESIAN_POINT('Ctrl Pts',(9.70137553959111,-112.604519323734,-1.74689558624962E-11));
#19617=CARTESIAN_POINT('Ctrl Pts',(7.27603165468577,-112.429519323734,-4.20081883448253));
#19618=CARTESIAN_POINT('Ctrl Pts',(4.85068776978043,-112.254519323734,-8.4016376689476));
#19619=CARTESIAN_POINT('Ctrl Pts',(-1.51301029103127E-11,-112.079519323734,
-8.40163766893887));
#19620=CARTESIAN_POINT('Ctrl Pts',(-4.85068776981069,-111.904519323734,
-8.40163766893014));
#19621=CARTESIAN_POINT('Ctrl Pts',(-7.2760316547009,-111.729519323734,-4.20081883445633));
#19622=CARTESIAN_POINT('Ctrl Pts',(-9.70137553959111,-111.554519323734,
1.74701439383464E-11));
#19623=CARTESIAN_POINT('Ctrl Pts',(-7.27603165468577,-111.379519323734,
4.20081883448254));
#19624=CARTESIAN_POINT('Ctrl Pts',(-4.85068776978043,-111.204519323734,
8.40163766894761));
#19625=CARTESIAN_POINT('Ctrl Pts',(1.51290740064448E-11,-111.029519323734,
8.40163766893887));
#19626=CARTESIAN_POINT('Ctrl Pts',(4.85068776981068,-110.854519323734,8.40163766893014));
#19627=CARTESIAN_POINT('Ctrl Pts',(7.2760316547009,-110.679519323734,4.20081883445634));
#19628=CARTESIAN_POINT('Ctrl Pts',(9.70137553959111,-110.504519323734,-1.74689558624962E-11));
#19629=CARTESIAN_POINT('Ctrl Pts',(7.27603165468577,-110.329519323734,-4.20081883448253));
#19630=CARTESIAN_POINT('Ctrl Pts',(4.85068776978043,-110.154519323734,-8.4016376689476));
#19631=CARTESIAN_POINT('Ctrl Pts',(-1.51301029103127E-11,-109.979519323734,
-8.40163766893887));
#19632=CARTESIAN_POINT('Ctrl Pts',(-4.85068776981069,-109.804519323734,
-8.40163766893014));
#19633=CARTESIAN_POINT('Ctrl Pts',(-7.2760316547009,-109.629519323734,-4.20081883445633));
#19634=CARTESIAN_POINT('Ctrl Pts',(-9.70137553959111,-109.454519323734,
1.74701439383464E-11));
#19635=CARTESIAN_POINT('Ctrl Pts',(-7.27603165468577,-109.279519323734,
4.20081883448254));
#19636=CARTESIAN_POINT('Ctrl Pts',(-4.85068776978043,-109.104519323734,
8.40163766894761));
#19637=CARTESIAN_POINT('Ctrl Pts',(1.51290740064448E-11,-108.929519323734,
8.40163766893887));
#19638=CARTESIAN_POINT('Ctrl Pts',(4.85068776981068,-108.754519323734,8.40163766893014));
#19639=CARTESIAN_POINT('Ctrl Pts',(7.2760316547009,-108.579519323734,4.20081883445634));
#19640=CARTESIAN_POINT('Ctrl Pts',(9.70137553959111,-108.404519323734,-1.74689558624962E-11));
#19641=CARTESIAN_POINT('Ctrl Pts',(7.27603165468577,-108.229519323734,-4.20081883448253));
#19642=CARTESIAN_POINT('Ctrl Pts',(4.85068776978043,-108.054519323734,-8.4016376689476));
#19643=CARTESIAN_POINT('Ctrl Pts',(-1.51301029103127E-11,-107.879519323734,
-8.40163766893887));
#19644=CARTESIAN_POINT('Ctrl Pts',(-4.85068776981069,-107.704519323734,
-8.40163766893014));
#19645=CARTESIAN_POINT('Ctrl Pts',(-7.2760316547009,-107.529519323734,-4.20081883445633));
#19646=CARTESIAN_POINT('Ctrl Pts',(-9.70137553959111,-107.354519323734,
1.74701439383464E-11));
#19647=CARTESIAN_POINT('Ctrl Pts',(-7.27603165468577,-107.179519323734,
4.20081883448254));
#19648=CARTESIAN_POINT('Ctrl Pts',(-4.85068776978043,-107.004519323734,
8.40163766894761));
#19649=CARTESIAN_POINT('Ctrl Pts',(1.51290740064448E-11,-106.829519323734,
8.40163766893887));
#19650=CARTESIAN_POINT('Ctrl Pts',(4.85068776981068,-106.654519323734,8.40163766893014));
#19651=CARTESIAN_POINT('Ctrl Pts',(7.2760316547009,-106.479519323734,4.20081883445634));
#19652=CARTESIAN_POINT('Ctrl Pts',(9.70137553959111,-106.304519323734,-1.74689558624962E-11));
#19653=CARTESIAN_POINT('Ctrl Pts',(7.27603165468577,-106.129519323734,-4.20081883448253));
#19654=CARTESIAN_POINT('Ctrl Pts',(4.85068776978043,-105.954519323734,-8.4016376689476));
#19655=CARTESIAN_POINT('Ctrl Pts',(-1.51301029103127E-11,-105.779519323734,
-8.40163766893887));
#19656=CARTESIAN_POINT('Ctrl Pts',(-4.85068776981069,-105.604519323734,
-8.40163766893014));
#19657=CARTESIAN_POINT('Ctrl Pts',(-7.2760316547009,-105.429519323734,-4.20081883445633));
#19658=CARTESIAN_POINT('Ctrl Pts',(-9.70137553959111,-105.254519323734,
1.74701439383464E-11));
#19659=CARTESIAN_POINT('Ctrl Pts',(-7.27603165468577,-105.079519323734,
4.20081883448254));
#19660=CARTESIAN_POINT('Ctrl Pts',(-4.85068776978043,-104.904519323734,
8.40163766894761));
#19661=CARTESIAN_POINT('Ctrl Pts',(1.51290740064448E-11,-104.729519323734,
8.40163766893887));
#19662=CARTESIAN_POINT('Ctrl Pts',(4.85068776981068,-104.554519323734,8.40163766893014));
#19663=CARTESIAN_POINT('Ctrl Pts',(7.2760316547009,-104.379519323734,4.20081883445634));
#19664=CARTESIAN_POINT('Ctrl Pts',(9.70137553959111,-104.204519323734,-1.74689558624962E-11));
#19665=CARTESIAN_POINT('Ctrl Pts',(7.27603165468577,-104.029519323734,-4.20081883448253));
#19666=CARTESIAN_POINT('Ctrl Pts',(4.85068776978043,-103.854519323734,-8.4016376689476));
#19667=CARTESIAN_POINT('Ctrl Pts',(-1.51301029103127E-11,-103.679519323734,
-8.40163766893887));
#19668=CARTESIAN_POINT('Ctrl Pts',(-4.85068776981069,-103.504519323734,
-8.40163766893014));
#19669=CARTESIAN_POINT('Ctrl Pts',(-7.2760316547009,-103.329519323734,-4.20081883445633));
#19670=CARTESIAN_POINT('Ctrl Pts',(-9.70137553959111,-103.154519323734,
1.74701439383464E-11));
#19671=CARTESIAN_POINT('Ctrl Pts',(-7.27603165468577,-102.979519323734,
4.20081883448254));
#19672=CARTESIAN_POINT('Ctrl Pts',(-4.85068776978043,-102.804519323734,
8.40163766894761));
#19673=CARTESIAN_POINT('Ctrl Pts',(1.51290740064448E-11,-102.629519323734,
8.40163766893887));
#19674=CARTESIAN_POINT('Ctrl Pts',(4.85068776981068,-102.454519323734,8.40163766893014));
#19675=CARTESIAN_POINT('Ctrl Pts',(7.2760316547009,-102.279519323734,4.20081883445634));
#19676=CARTESIAN_POINT('Ctrl Pts',(9.70137553959111,-102.104519323734,-1.74689558624962E-11));
#19677=CARTESIAN_POINT('Ctrl Pts',(7.27603165468577,-101.929519323734,-4.20081883448253));
#19678=CARTESIAN_POINT('Ctrl Pts',(4.85068776978043,-101.754519323734,-8.4016376689476));
#19679=CARTESIAN_POINT('Ctrl Pts',(-1.51301029103127E-11,-101.579519323734,
-8.40163766893887));
#19680=CARTESIAN_POINT('Ctrl Pts',(-4.85068776981069,-101.404519323734,
-8.40163766893014));
#19681=CARTESIAN_POINT('Ctrl Pts',(-7.2760316547009,-101.229519323734,-4.20081883445633));
#19682=CARTESIAN_POINT('Ctrl Pts',(-9.70137553959111,-101.054519323734,
1.74701439383464E-11));
#19683=CARTESIAN_POINT('Ctrl Pts',(-7.27603165468577,-100.879519323734,
4.20081883448254));
#19684=CARTESIAN_POINT('Ctrl Pts',(-4.85068776978043,-100.704519323734,
8.40163766894761));
#19685=CARTESIAN_POINT('Ctrl Pts',(1.51290740064448E-11,-100.529519323734,
8.40163766893887));
#19686=CARTESIAN_POINT('Ctrl Pts',(4.85068776981068,-100.354519323734,8.40163766893014));
#19687=CARTESIAN_POINT('Ctrl Pts',(7.2760316547009,-100.179519323734,4.20081883445634));
#19688=CARTESIAN_POINT('Ctrl Pts',(9.70137553959111,-100.004519323734,-1.74689558624962E-11));
#19689=CARTESIAN_POINT('Ctrl Pts',(7.27603165468577,-99.8295193237339,-4.20081883448253));
#19690=CARTESIAN_POINT('Ctrl Pts',(4.85068776978043,-99.6545193237339,-8.4016376689476));
#19691=CARTESIAN_POINT('Ctrl Pts',(-1.51301029103127E-11,-99.4795193237339,
-8.40163766893887));
#19692=CARTESIAN_POINT('Ctrl Pts',(-4.85068776981069,-99.3045193237339,
-8.40163766893014));
#19693=CARTESIAN_POINT('Ctrl Pts',(-7.2760316547009,-99.1295193237339,-4.20081883445633));
#19694=CARTESIAN_POINT('Ctrl Pts',(-9.70137553959111,-98.9545193237339,
1.74701439383464E-11));
#19695=CARTESIAN_POINT('Ctrl Pts',(-7.27603165468577,-98.7795193237339,
4.20081883448254));
#19696=CARTESIAN_POINT('Ctrl Pts',(-4.85068776978043,-98.6045193237339,
8.40163766894761));
#19697=CARTESIAN_POINT('Ctrl Pts',(1.51290740064448E-11,-98.4295193237339,
8.40163766893887));
#19698=CARTESIAN_POINT('Ctrl Pts',(4.85068776981068,-98.2545193237339,8.40163766893014));
#19699=CARTESIAN_POINT('Ctrl Pts',(7.2760316547009,-98.0795193237339,4.20081883445634));
#19700=CARTESIAN_POINT('Ctrl Pts',(9.70137553959111,-97.904519323734,-1.74689558624962E-11));
#19701=CARTESIAN_POINT('Ctrl Pts',(7.27603165468577,-97.7295193237339,-4.20081883448253));
#19702=CARTESIAN_POINT('Ctrl Pts',(4.85068776978043,-97.5545193237339,-8.4016376689476));
#19703=CARTESIAN_POINT('Ctrl Pts',(-1.51301029103127E-11,-97.3795193237339,
-8.40163766893887));
#19704=CARTESIAN_POINT('Ctrl Pts',(-4.85068776981069,-97.2045193237339,
-8.40163766893014));
#19705=CARTESIAN_POINT('Ctrl Pts',(-7.2760316547009,-97.0295193237339,-4.20081883445633));
#19706=CARTESIAN_POINT('Ctrl Pts',(-9.70137553959111,-96.8545193237339,
1.74701439383464E-11));
#19707=CARTESIAN_POINT('Ctrl Pts',(-7.27603165468577,-96.6795193237339,
4.20081883448254));
#19708=CARTESIAN_POINT('Ctrl Pts',(-4.85068776978043,-96.5045193237339,
8.40163766894761));
#19709=CARTESIAN_POINT('Ctrl Pts',(1.51290740064448E-11,-96.3295193237339,
8.40163766893887));
#19710=CARTESIAN_POINT('Ctrl Pts',(4.85068776981068,-96.1545193237339,8.40163766893014));
#19711=CARTESIAN_POINT('Ctrl Pts',(7.2760316547009,-95.9795193237339,4.20081883445634));
#19712=CARTESIAN_POINT('Ctrl Pts',(9.70137553959111,-95.804519323734,-1.74689558624962E-11));
#19713=CARTESIAN_POINT('Ctrl Pts',(7.27603165468577,-95.6295193237339,-4.20081883448253));
#19714=CARTESIAN_POINT('Ctrl Pts',(4.85068776978043,-95.4545193237339,-8.4016376689476));
#19715=CARTESIAN_POINT('Ctrl Pts',(-1.51301029103127E-11,-95.2795193237339,
-8.40163766893887));
#19716=CARTESIAN_POINT('Ctrl Pts',(-4.85068776981069,-95.1045193237339,
-8.40163766893014));
#19717=CARTESIAN_POINT('Ctrl Pts',(-7.2760316547009,-94.9295193237339,-4.20081883445633));
#19718=CARTESIAN_POINT('Ctrl Pts',(-9.70137553959111,-94.7545193237339,
1.74701439383464E-11));
#19719=CARTESIAN_POINT('Ctrl Pts',(-7.27603165468577,-94.5795193237339,
4.20081883448254));
#19720=CARTESIAN_POINT('Ctrl Pts',(-4.85068776978043,-94.4045193237339,
8.40163766894761));
#19721=CARTESIAN_POINT('Ctrl Pts',(1.51290740064448E-11,-94.2295193237339,
8.40163766893887));
#19722=CARTESIAN_POINT('Ctrl Pts',(4.85068776981068,-94.0545193237339,8.40163766893014));
#19723=CARTESIAN_POINT('Ctrl Pts',(7.2760316547009,-93.8795193237339,4.20081883445634));
#19724=CARTESIAN_POINT('Ctrl Pts',(9.70137553959111,-93.7045193237339,-1.74689558624962E-11));
#19725=CARTESIAN_POINT('Ctrl Pts',(7.27603165468577,-93.5295193237339,-4.20081883448253));
#19726=CARTESIAN_POINT('Ctrl Pts',(4.85068776978043,-93.3545193237339,-8.4016376689476));
#19727=CARTESIAN_POINT('Ctrl Pts',(-1.51301029103127E-11,-93.1795193237339,
-8.40163766893887));
#19728=CARTESIAN_POINT('Ctrl Pts',(-4.85068776981069,-93.0045193237339,
-8.40163766893014));
#19729=CARTESIAN_POINT('Ctrl Pts',(-7.2760316547009,-92.8295193237339,-4.20081883445633));
#19730=CARTESIAN_POINT('Ctrl Pts',(-9.70137553959111,-92.6545193237339,
1.74701439383464E-11));
#19731=CARTESIAN_POINT('Ctrl Pts',(-7.27603165468577,-92.4795193237339,
4.20081883448254));
#19732=CARTESIAN_POINT('Ctrl Pts',(-4.85068776978043,-92.3045193237339,
8.40163766894761));
#19733=CARTESIAN_POINT('Ctrl Pts',(1.51290740064448E-11,-92.1295193237339,
8.40163766893887));
#19734=CARTESIAN_POINT('Ctrl Pts',(4.85068776981068,-91.9545193237339,8.40163766893014));
#19735=CARTESIAN_POINT('Ctrl Pts',(7.2760316547009,-91.7795193237339,4.20081883445634));
#19736=CARTESIAN_POINT('Ctrl Pts',(9.70137553959111,-91.6045193237339,-1.74689558624962E-11));
#19737=CARTESIAN_POINT('Ctrl Pts',(7.27603165468577,-91.4295193237339,-4.20081883448253));
#19738=CARTESIAN_POINT('Ctrl Pts',(4.85068776978043,-91.2545193237339,-8.4016376689476));
#19739=CARTESIAN_POINT('Ctrl Pts',(-1.51301029103127E-11,-91.0795193237339,
-8.40163766893887));
#19740=CARTESIAN_POINT('Ctrl Pts',(-4.85068776981069,-90.9045193237339,
-8.40163766893014));
#19741=CARTESIAN_POINT('Ctrl Pts',(-7.2760316547009,-90.7295193237339,-4.20081883445633));
#19742=CARTESIAN_POINT('Ctrl Pts',(-9.70137553959111,-90.5545193237339,
1.74701439383464E-11));
#19743=CARTESIAN_POINT('Ctrl Pts',(-7.27603165468577,-90.3795193237339,
4.20081883448254));
#19744=CARTESIAN_POINT('Ctrl Pts',(-4.85068776978043,-90.2045193237339,
8.40163766894761));
#19745=CARTESIAN_POINT('Ctrl Pts',(1.51290740064448E-11,-90.0295193237339,
8.40163766893887));
#19746=CARTESIAN_POINT('Ctrl Pts',(4.85068776981068,-89.8545193237339,8.40163766893014));
#19747=CARTESIAN_POINT('Ctrl Pts',(7.2760316547009,-89.6795193237339,4.20081883445634));
#19748=CARTESIAN_POINT('Ctrl Pts',(9.70137553959111,-89.5045193237339,-1.74689558624962E-11));
#19749=CARTESIAN_POINT('Ctrl Pts',(7.27603165468577,-89.3295193237339,-4.20081883448253));
#19750=CARTESIAN_POINT('Ctrl Pts',(4.85068776978043,-89.154519323734,-8.4016376689476));
#19751=CARTESIAN_POINT('Ctrl Pts',(-1.51301029103127E-11,-88.9795193237339,
-8.40163766893887));
#19752=CARTESIAN_POINT('Ctrl Pts',(-4.85068776981069,-88.8045193237339,
-8.40163766893014));
#19753=CARTESIAN_POINT('Ctrl Pts',(-7.2760316547009,-88.6295193237339,-4.20081883445633));
#19754=CARTESIAN_POINT('Ctrl Pts',(-9.70137553959111,-88.4545193237339,
1.74701439383464E-11));
#19755=CARTESIAN_POINT('Ctrl Pts',(-7.27603165468577,-88.2795193237339,
4.20081883448254));
#19756=CARTESIAN_POINT('Ctrl Pts',(-4.85068776978043,-88.104519323734,8.40163766894761));
#19757=CARTESIAN_POINT('Ctrl Pts',(1.51290740064448E-11,-87.9295193237339,
8.40163766893887));
#19758=CARTESIAN_POINT('Ctrl Pts',(4.85068776981068,-87.7545193237339,8.40163766893014));
#19759=CARTESIAN_POINT('Ctrl Pts',(7.2760316547009,-87.5795193237339,4.20081883445634));
#19760=CARTESIAN_POINT('Ctrl Pts',(9.70137553959111,-87.404519323734,-1.74689558624962E-11));
#19761=CARTESIAN_POINT('Ctrl Pts',(7.27603165468577,-87.2295193237339,-4.20081883448253));
#19762=CARTESIAN_POINT('Ctrl Pts',(4.85068776978043,-87.054519323734,-8.4016376689476));
#19763=CARTESIAN_POINT('Ctrl Pts',(-1.51301029103127E-11,-86.8795193237339,
-8.40163766893887));
#19764=CARTESIAN_POINT('Ctrl Pts',(-4.85068776981069,-86.7045193237339,
-8.40163766893014));
#19765=CARTESIAN_POINT('Ctrl Pts',(-7.2760316547009,-86.529519323734,-4.20081883445633));
#19766=CARTESIAN_POINT('Ctrl Pts',(-9.70137553959111,-86.3545193237339,
1.74701439383464E-11));
#19767=CARTESIAN_POINT('Ctrl Pts',(-7.27603165468577,-86.1795193237339,
4.20081883448254));
#19768=CARTESIAN_POINT('Ctrl Pts',(-4.85068776978043,-86.0045193237339,
8.40163766894761));
#19769=CARTESIAN_POINT('Ctrl Pts',(1.51290740064448E-11,-85.8295193237339,
8.40163766893887));
#19770=CARTESIAN_POINT('Ctrl Pts',(4.85068776981068,-85.6545193237339,8.40163766893014));
#19771=CARTESIAN_POINT('Ctrl Pts',(7.2760316547009,-85.4795193237339,4.20081883445634));
#19772=CARTESIAN_POINT('Ctrl Pts',(9.70137553959111,-85.3045193237339,-1.74689558624962E-11));
#19773=CARTESIAN_POINT('Ctrl Pts',(7.27603165468577,-85.1295193237339,-4.20081883448253));
#19774=CARTESIAN_POINT('Ctrl Pts',(4.85068776978043,-84.9545193237339,-8.4016376689476));
#19775=CARTESIAN_POINT('Ctrl Pts',(-1.51301029103127E-11,-84.7795193237339,
-8.40163766893887));
#19776=CARTESIAN_POINT('Ctrl Pts',(-4.85068776981069,-84.604519323734,-8.40163766893014));
#19777=CARTESIAN_POINT('Ctrl Pts',(-7.2760316547009,-84.4295193237339,-4.20081883445633));
#19778=CARTESIAN_POINT('Ctrl Pts',(-9.70137553959111,-84.2545193237339,
1.74701439383464E-11));
#19779=CARTESIAN_POINT('Ctrl Pts',(-7.27603165468577,-84.0795193237339,
4.20081883448254));
#19780=CARTESIAN_POINT('Ctrl Pts',(-4.85068776978043,-83.9045193237339,
8.40163766894761));
#19781=CARTESIAN_POINT('Ctrl Pts',(1.51290740064448E-11,-83.7295193237339,
8.40163766893887));
#19782=CARTESIAN_POINT('Ctrl Pts',(4.85068776981068,-83.554519323734,8.40163766893014));
#19783=CARTESIAN_POINT('Ctrl Pts',(7.2760316547009,-83.3795193237339,4.20081883445634));
#19784=CARTESIAN_POINT('Ctrl Pts',(9.70137553959111,-83.2045193237339,-1.74689558624962E-11));
#19785=CARTESIAN_POINT('Ctrl Pts',(7.27603165468577,-83.029519323734,-4.20081883448253));
#19786=CARTESIAN_POINT('Ctrl Pts',(4.85068776978043,-82.8545193237339,-8.4016376689476));
#19787=CARTESIAN_POINT('Ctrl Pts',(-1.51301029103127E-11,-82.6795193237339,
-8.40163766893887));
#19788=CARTESIAN_POINT('Ctrl Pts',(-4.85068776981069,-82.504519323734,-8.40163766893014));
#19789=CARTESIAN_POINT('Ctrl Pts',(-7.2760316547009,-82.3295193237339,-4.20081883445633));
#19790=CARTESIAN_POINT('Ctrl Pts',(-9.70137553959111,-82.154519323734,1.74701439383464E-11));
#19791=CARTESIAN_POINT('Ctrl Pts',(-7.27603165468577,-81.9795193237339,
4.20081883448254));
#19792=CARTESIAN_POINT('Ctrl Pts',(-4.85068776978043,-81.8045193237339,
8.40163766894761));
#19793=CARTESIAN_POINT('Ctrl Pts',(1.51290740064448E-11,-81.6295193237339,
8.40163766893887));
#19794=CARTESIAN_POINT('Ctrl Pts',(4.85068776981068,-81.454519323734,8.40163766893014));
#19795=CARTESIAN_POINT('Ctrl Pts',(7.2760316547009,-81.2795193237339,4.20081883445634));
#19796=CARTESIAN_POINT('Ctrl Pts',(9.70137553959111,-81.1045193237339,-1.74689558624962E-11));
#19797=CARTESIAN_POINT('Ctrl Pts',(7.27603165468577,-80.929519323734,-4.20081883448253));
#19798=CARTESIAN_POINT('Ctrl Pts',(4.85068776978043,-80.754519323734,-8.4016376689476));
#19799=CARTESIAN_POINT('Ctrl Pts',(-1.51301029103127E-11,-80.5795193237339,
-8.40163766893887));
#19800=CARTESIAN_POINT('Ctrl Pts',(-4.85068776981069,-80.404519323734,-8.40163766893014));
#19801=CARTESIAN_POINT('Ctrl Pts',(-7.2760316547009,-80.2295193237339,-4.20081883445633));
#19802=CARTESIAN_POINT('Ctrl Pts',(-9.70137553959111,-80.054519323734,1.74701439383464E-11));
#19803=CARTESIAN_POINT('Ctrl Pts',(-7.27603165468577,-79.879519323734,4.20081883448254));
#19804=CARTESIAN_POINT('Ctrl Pts',(-4.85068776978043,-79.7045193237339,
8.40163766894761));
#19805=CARTESIAN_POINT('Ctrl Pts',(1.51290740064448E-11,-79.5295193237339,
8.40163766893887));
#19806=CARTESIAN_POINT('Ctrl Pts',(4.85068776981068,-79.354519323734,8.40163766893014));
#19807=CARTESIAN_POINT('Ctrl Pts',(7.2760316547009,-79.179519323734,4.20081883445634));
#19808=CARTESIAN_POINT('Ctrl Pts',(9.70137553959111,-79.0045193237339,-1.74689558624962E-11));
#19809=CARTESIAN_POINT('Ctrl Pts',(7.27603165468577,-78.829519323734,-4.20081883448253));
#19810=CARTESIAN_POINT('Ctrl Pts',(4.85068776978043,-78.654519323734,-8.4016376689476));
#19811=CARTESIAN_POINT('Ctrl Pts',(-1.51301029103127E-11,-78.4795193237339,
-8.40163766893887));
#19812=CARTESIAN_POINT('Ctrl Pts',(-4.85068776981069,-78.304519323734,-8.40163766893014));
#19813=CARTESIAN_POINT('Ctrl Pts',(-7.2760316547009,-78.129519323734,-4.20081883445633));
#19814=CARTESIAN_POINT('Ctrl Pts',(-9.70137553959111,-77.954519323734,1.74701439383464E-11));
#19815=CARTESIAN_POINT('Ctrl Pts',(-7.27603165468577,-77.779519323734,4.20081883448254));
#19816=CARTESIAN_POINT('Ctrl Pts',(-4.85068776978043,-77.604519323734,8.40163766894761));
#19817=CARTESIAN_POINT('Ctrl Pts',(1.51290740064448E-11,-77.4295193237339,
8.40163766893887));
#19818=CARTESIAN_POINT('Ctrl Pts',(4.85068776981068,-77.254519323734,8.40163766893014));
#19819=CARTESIAN_POINT('Ctrl Pts',(7.2760316547009,-77.0795193237339,4.20081883445634));
#19820=CARTESIAN_POINT('Ctrl Pts',(9.70137553959111,-76.904519323734,-1.74689558624962E-11));
#19821=CARTESIAN_POINT('Ctrl Pts',(7.27603165468577,-76.729519323734,-4.20081883448253));
#19822=CARTESIAN_POINT('Ctrl Pts',(4.85068776978043,-76.5545193237339,-8.4016376689476));
#19823=CARTESIAN_POINT('Ctrl Pts',(-1.51301029103127E-11,-76.379519323734,
-8.40163766893887));
#19824=CARTESIAN_POINT('Ctrl Pts',(-4.85068776981069,-76.204519323734,-8.40163766893014));
#19825=CARTESIAN_POINT('Ctrl Pts',(-7.2760316547009,-76.0295193237339,-4.20081883445633));
#19826=CARTESIAN_POINT('Ctrl Pts',(-9.70137553959111,-75.854519323734,1.74701439383464E-11));
#19827=CARTESIAN_POINT('Ctrl Pts',(-7.27603165468577,-75.679519323734,4.20081883448254));
#19828=CARTESIAN_POINT('Ctrl Pts',(-4.85068776978043,-75.5045193237339,
8.40163766894761));
#19829=CARTESIAN_POINT('Ctrl Pts',(1.51290740064448E-11,-75.329519323734,
8.40163766893887));
#19830=CARTESIAN_POINT('Ctrl Pts',(4.85068776981068,-75.1545193237339,8.40163766893014));
#19831=CARTESIAN_POINT('Ctrl Pts',(7.2760316547009,-74.9795193237339,4.20081883445634));
#19832=CARTESIAN_POINT('Ctrl Pts',(9.70137553959111,-74.804519323734,-1.74689558624962E-11));
#19833=CARTESIAN_POINT('Ctrl Pts',(7.27603165468577,-74.6295193237339,-4.20081883448253));
#19834=CARTESIAN_POINT('Ctrl Pts',(4.85068776978043,-74.454519323734,-8.4016376689476));
#19835=CARTESIAN_POINT('Ctrl Pts',(-1.51301029103127E-11,-74.279519323734,
-8.40163766893887));
#19836=CARTESIAN_POINT('Ctrl Pts',(-4.85068776981069,-74.104519323734,-8.40163766893014));
#19837=CARTESIAN_POINT('Ctrl Pts',(-7.2760316547009,-73.9295193237339,-4.20081883445633));
#19838=CARTESIAN_POINT('Ctrl Pts',(-9.70137553959111,-73.754519323734,1.74701439383464E-11));
#19839=CARTESIAN_POINT('Ctrl Pts',(-7.27603165468577,-73.579519323734,4.20081883448254));
#19840=CARTESIAN_POINT('Ctrl Pts',(-4.85068776978043,-73.404519323734,8.40163766894761));
#19841=CARTESIAN_POINT('Ctrl Pts',(1.51290740064448E-11,-73.229519323734,
8.40163766893887));
#19842=CARTESIAN_POINT('Ctrl Pts',(4.85068776981068,-73.054519323734,8.40163766893014));
#19843=CARTESIAN_POINT('Ctrl Pts',(7.2760316547009,-72.8795193237339,4.20081883445634));
#19844=CARTESIAN_POINT('Ctrl Pts',(9.70137553959111,-72.704519323734,-1.74689558624962E-11));
#19845=CARTESIAN_POINT('Ctrl Pts',(7.27603165468577,-72.529519323734,-4.20081883448253));
#19846=CARTESIAN_POINT('Ctrl Pts',(4.85068776978043,-72.354519323734,-8.4016376689476));
#19847=CARTESIAN_POINT('Ctrl Pts',(-1.51301029103127E-11,-72.179519323734,
-8.40163766893887));
#19848=CARTESIAN_POINT('Ctrl Pts',(-4.85068776981069,-72.004519323734,-8.40163766893014));
#19849=CARTESIAN_POINT('Ctrl Pts',(-7.2760316547009,-71.829519323734,-4.20081883445633));
#19850=CARTESIAN_POINT('Ctrl Pts',(-9.70137553959111,-71.654519323734,1.74701439383464E-11));
#19851=CARTESIAN_POINT('Ctrl Pts',(-7.27603165468577,-71.479519323734,4.20081883448254));
#19852=CARTESIAN_POINT('Ctrl Pts',(-4.85068776978043,-71.304519323734,8.40163766894761));
#19853=CARTESIAN_POINT('Ctrl Pts',(1.51290740064448E-11,-71.129519323734,
8.40163766893887));
#19854=CARTESIAN_POINT('Ctrl Pts',(4.85068776981068,-70.954519323734,8.40163766893014));
#19855=CARTESIAN_POINT('Ctrl Pts',(7.2760316547009,-70.779519323734,4.20081883445634));
#19856=CARTESIAN_POINT('Ctrl Pts',(9.70137553959111,-70.604519323734,-1.74689558624962E-11));
#19857=CARTESIAN_POINT('Ctrl Pts',(7.27603165468577,-70.429519323734,-4.20081883448253));
#19858=CARTESIAN_POINT('Ctrl Pts',(4.85068776978043,-70.254519323734,-8.4016376689476));
#19859=CARTESIAN_POINT('Ctrl Pts',(-1.51301029103127E-11,-70.079519323734,
-8.40163766893887));
#19860=CARTESIAN_POINT('Ctrl Pts',(-4.85068776981069,-69.904519323734,-8.40163766893014));
#19861=CARTESIAN_POINT('Ctrl Pts',(-7.2760316547009,-69.729519323734,-4.20081883445633));
#19862=CARTESIAN_POINT('Ctrl Pts',(-9.70137553959111,-69.554519323734,1.74701439383464E-11));
#19863=CARTESIAN_POINT('Ctrl Pts',(-7.27603165468577,-69.379519323734,4.20081883448254));
#19864=CARTESIAN_POINT('Ctrl Pts',(-4.85068776978043,-69.204519323734,8.40163766894761));
#19865=CARTESIAN_POINT('Ctrl Pts',(1.51290740064448E-11,-69.029519323734,
8.40163766893887));
#19866=CARTESIAN_POINT('Ctrl Pts',(4.85068776981068,-68.854519323734,8.40163766893014));
#19867=CARTESIAN_POINT('Ctrl Pts',(7.2760316547009,-68.679519323734,4.20081883445634));
#19868=CARTESIAN_POINT('Ctrl Pts',(9.70137553959111,-68.504519323734,-1.74689558624962E-11));
#19869=CARTESIAN_POINT('Ctrl Pts',(7.27603165468577,-68.3295193237339,-4.20081883448253));
#19870=CARTESIAN_POINT('Ctrl Pts',(4.85068776978043,-68.154519323734,-8.4016376689476));
#19871=CARTESIAN_POINT('Ctrl Pts',(-1.51301029103127E-11,-67.979519323734,
-8.40163766893887));
#19872=CARTESIAN_POINT('Ctrl Pts',(-4.85068776981069,-67.804519323734,-8.40163766893014));
#19873=CARTESIAN_POINT('Ctrl Pts',(-7.2760316547009,-67.629519323734,-4.20081883445633));
#19874=CARTESIAN_POINT('Ctrl Pts',(-9.70137553959111,-67.454519323734,1.74701439383464E-11));
#19875=CARTESIAN_POINT('Ctrl Pts',(-7.27603165468577,-67.279519323734,4.20081883448254));
#19876=CARTESIAN_POINT('Ctrl Pts',(-4.85068776978043,-67.104519323734,8.40163766894761));
#19877=CARTESIAN_POINT('Ctrl Pts',(1.51290740064448E-11,-66.929519323734,
8.40163766893887));
#19878=CARTESIAN_POINT('Ctrl Pts',(4.85068776981068,-66.754519323734,8.40163766893014));
#19879=CARTESIAN_POINT('Ctrl Pts',(7.2760316547009,-66.579519323734,4.20081883445634));
#19880=CARTESIAN_POINT('Ctrl Pts',(9.70137553959111,-66.404519323734,-1.74689558624962E-11));
#19881=CARTESIAN_POINT('Ctrl Pts',(7.27603165468577,-66.229519323734,-4.20081883448253));
#19882=CARTESIAN_POINT('Ctrl Pts',(4.85068776978043,-66.054519323734,-8.4016376689476));
#19883=CARTESIAN_POINT('Ctrl Pts',(-1.51301029103127E-11,-65.879519323734,
-8.40163766893887));
#19884=CARTESIAN_POINT('Ctrl Pts',(-4.85068776981069,-65.704519323734,-8.40163766893014));
#19885=CARTESIAN_POINT('Ctrl Pts',(-7.2760316547009,-65.529519323734,-4.20081883445633));
#19886=CARTESIAN_POINT('Ctrl Pts',(-9.70137553959111,-65.354519323734,1.74701439383464E-11));
#19887=CARTESIAN_POINT('Ctrl Pts',(-7.27603165468577,-65.179519323734,4.20081883448254));
#19888=CARTESIAN_POINT('Ctrl Pts',(-4.85068776978043,-65.004519323734,8.40163766894761));
#19889=CARTESIAN_POINT('Ctrl Pts',(1.51290740064448E-11,-64.829519323734,
8.40163766893887));
#19890=CARTESIAN_POINT('Ctrl Pts',(4.85068776981068,-64.654519323734,8.40163766893014));
#19891=CARTESIAN_POINT('Ctrl Pts',(7.2760316547009,-64.479519323734,4.20081883445634));
#19892=CARTESIAN_POINT('Ctrl Pts',(9.70137553959111,-64.304519323734,-1.74689558624962E-11));
#19893=CARTESIAN_POINT('Ctrl Pts',(7.27603165468577,-64.129519323734,-4.20081883448253));
#19894=CARTESIAN_POINT('Ctrl Pts',(4.85068776978043,-63.954519323734,-8.4016376689476));
#19895=CARTESIAN_POINT('Ctrl Pts',(-1.51301029103127E-11,-63.779519323734,
-8.40163766893887));
#19896=CARTESIAN_POINT('Ctrl Pts',(-4.85068776981069,-63.604519323734,-8.40163766893014));
#19897=CARTESIAN_POINT('Ctrl Pts',(-7.2760316547009,-63.429519323734,-4.20081883445633));
#19898=CARTESIAN_POINT('Ctrl Pts',(-9.70137553959111,-63.254519323734,1.74701439383464E-11));
#19899=CARTESIAN_POINT('Ctrl Pts',(-7.27603165468577,-63.079519323734,4.20081883448254));
#19900=CARTESIAN_POINT('Ctrl Pts',(-4.85068776978043,-62.904519323734,8.40163766894761));
#19901=CARTESIAN_POINT('Ctrl Pts',(1.51290740064448E-11,-62.729519323734,
8.40163766893887));
#19902=CARTESIAN_POINT('Ctrl Pts',(4.85068776981068,-62.554519323734,8.40163766893014));
#19903=CARTESIAN_POINT('Ctrl Pts',(7.2760316547009,-62.379519323734,4.20081883445634));
#19904=CARTESIAN_POINT('Ctrl Pts',(9.70137553959111,-62.204519323734,-1.74689558624962E-11));
#19905=CARTESIAN_POINT('Ctrl Pts',(7.27603165468577,-62.029519323734,-4.20081883448253));
#19906=CARTESIAN_POINT('Ctrl Pts',(4.85068776978043,-61.854519323734,-8.4016376689476));
#19907=CARTESIAN_POINT('Ctrl Pts',(-1.51301029103127E-11,-61.679519323734,
-8.40163766893887));
#19908=CARTESIAN_POINT('Ctrl Pts',(-4.85068776981069,-61.504519323734,-8.40163766893014));
#19909=CARTESIAN_POINT('Ctrl Pts',(-7.2760316547009,-61.329519323734,-4.20081883445633));
#19910=CARTESIAN_POINT('Ctrl Pts',(-9.70137553959111,-61.154519323734,1.74701439383464E-11));
#19911=CARTESIAN_POINT('Ctrl Pts',(-7.27603165468577,-60.979519323734,4.20081883448254));
#19912=CARTESIAN_POINT('Ctrl Pts',(-4.85068776978043,-60.804519323734,8.40163766894761));
#19913=CARTESIAN_POINT('Ctrl Pts',(1.51290740064448E-11,-60.629519323734,
8.40163766893887));
#19914=CARTESIAN_POINT('Ctrl Pts',(4.85068776981068,-60.454519323734,8.40163766893014));
#19915=CARTESIAN_POINT('Ctrl Pts',(7.2760316547009,-60.279519323734,4.20081883445634));
#19916=CARTESIAN_POINT('Ctrl Pts',(9.70137553959111,-60.104519323734,-1.74689558624962E-11));
#19917=CARTESIAN_POINT('Ctrl Pts',(7.27603165468577,-59.929519323734,-4.20081883448253));
#19918=CARTESIAN_POINT('Ctrl Pts',(4.85068776978043,-59.754519323734,-8.4016376689476));
#19919=CARTESIAN_POINT('Ctrl Pts',(-1.51301029103127E-11,-59.579519323734,
-8.40163766893887));
#19920=CARTESIAN_POINT('Ctrl Pts',(-4.85068776981069,-59.404519323734,-8.40163766893014));
#19921=CARTESIAN_POINT('Ctrl Pts',(-7.2760316547009,-59.229519323734,-4.20081883445633));
#19922=CARTESIAN_POINT('Ctrl Pts',(-9.70137553959111,-59.054519323734,1.74701439383464E-11));
#19923=CARTESIAN_POINT('Ctrl Pts',(-7.27603165468577,-58.879519323734,4.20081883448254));
#19924=CARTESIAN_POINT('Ctrl Pts',(-4.85068776978043,-58.704519323734,8.40163766894761));
#19925=CARTESIAN_POINT('Ctrl Pts',(1.51290740064448E-11,-58.529519323734,
8.40163766893887));
#19926=CARTESIAN_POINT('Ctrl Pts',(4.85068776981068,-58.354519323734,8.40163766893014));
#19927=CARTESIAN_POINT('Ctrl Pts',(7.2760316547009,-58.179519323734,4.20081883445634));
#19928=CARTESIAN_POINT('Ctrl Pts',(9.70137553959111,-58.004519323734,-1.74689558624962E-11));
#19929=CARTESIAN_POINT('Ctrl Pts',(7.27603165468577,-57.829519323734,-4.20081883448253));
#19930=CARTESIAN_POINT('Ctrl Pts',(4.85068776978043,-57.654519323734,-8.4016376689476));
#19931=CARTESIAN_POINT('Ctrl Pts',(-1.51301029103127E-11,-57.479519323734,
-8.40163766893887));
#19932=CARTESIAN_POINT('Ctrl Pts',(-4.85068776981069,-57.304519323734,-8.40163766893014));
#19933=CARTESIAN_POINT('Ctrl Pts',(-7.2760316547009,-57.129519323734,-4.20081883445633));
#19934=CARTESIAN_POINT('Ctrl Pts',(-9.70137553959111,-56.954519323734,1.74701439383464E-11));
#19935=CARTESIAN_POINT('Ctrl Pts',(-7.27603165468577,-56.779519323734,4.20081883448254));
#19936=CARTESIAN_POINT('Ctrl Pts',(-4.85068776978043,-56.604519323734,8.40163766894761));
#19937=CARTESIAN_POINT('Ctrl Pts',(1.51290740064448E-11,-56.429519323734,
8.40163766893887));
#19938=CARTESIAN_POINT('Ctrl Pts',(4.85068776981068,-56.254519323734,8.40163766893014));
#19939=CARTESIAN_POINT('Ctrl Pts',(7.2760316547009,-56.079519323734,4.20081883445634));
#19940=CARTESIAN_POINT('Ctrl Pts',(9.70137553959111,-55.904519323734,-1.74689558624962E-11));
#19941=CARTESIAN_POINT('Ctrl Pts',(7.27603165468577,-55.729519323734,-4.20081883448253));
#19942=CARTESIAN_POINT('Ctrl Pts',(4.85068776978043,-55.554519323734,-8.4016376689476));
#19943=CARTESIAN_POINT('Ctrl Pts',(-1.51301029103127E-11,-55.379519323734,
-8.40163766893887));
#19944=CARTESIAN_POINT('Ctrl Pts',(-4.85068776981069,-55.204519323734,-8.40163766893014));
#19945=CARTESIAN_POINT('Ctrl Pts',(-7.2760316547009,-55.029519323734,-4.20081883445633));
#19946=CARTESIAN_POINT('Ctrl Pts',(-9.70137553959111,-54.854519323734,1.74701439383464E-11));
#19947=CARTESIAN_POINT('Ctrl Pts',(-7.27603165468577,-54.679519323734,4.20081883448254));
#19948=CARTESIAN_POINT('Ctrl Pts',(-4.85068776978043,-54.504519323734,8.40163766894761));
#19949=CARTESIAN_POINT('Ctrl Pts',(1.51290740064448E-11,-54.329519323734,
8.40163766893887));
#19950=CARTESIAN_POINT('Ctrl Pts',(4.85068776981068,-54.154519323734,8.40163766893014));
#19951=CARTESIAN_POINT('Ctrl Pts',(7.2760316547009,-53.979519323734,4.20081883445634));
#19952=CARTESIAN_POINT('Ctrl Pts',(9.70137553959111,-53.804519323734,-1.74689558624962E-11));
#19953=CARTESIAN_POINT('Ctrl Pts',(7.27603165468577,-53.629519323734,-4.20081883448253));
#19954=CARTESIAN_POINT('Ctrl Pts',(4.85068776978043,-53.454519323734,-8.4016376689476));
#19955=CARTESIAN_POINT('Ctrl Pts',(-1.51301029103127E-11,-53.279519323734,
-8.40163766893887));
#19956=CARTESIAN_POINT('Ctrl Pts',(-4.85068776981069,-53.104519323734,-8.40163766893014));
#19957=CARTESIAN_POINT('Ctrl Pts',(-7.2760316547009,-52.929519323734,-4.20081883445633));
#19958=CARTESIAN_POINT('Ctrl Pts',(-9.70137553959111,-52.754519323734,1.74701439383464E-11));
#19959=CARTESIAN_POINT('Ctrl Pts',(-7.27603165468577,-52.579519323734,4.20081883448254));
#19960=CARTESIAN_POINT('Ctrl Pts',(-4.85068776978043,-52.404519323734,8.40163766894761));
#19961=CARTESIAN_POINT('Ctrl Pts',(1.51290740064448E-11,-52.229519323734,
8.40163766893887));
#19962=CARTESIAN_POINT('Ctrl Pts',(4.85068776981068,-52.054519323734,8.40163766893014));
#19963=CARTESIAN_POINT('Ctrl Pts',(7.2760316547009,-51.879519323734,4.20081883445634));
#19964=CARTESIAN_POINT('Ctrl Pts',(9.70137553959111,-51.704519323734,-1.74689558624962E-11));
#19965=CARTESIAN_POINT('Ctrl Pts',(7.27603165468577,-51.529519323734,-4.20081883448253));
#19966=CARTESIAN_POINT('Ctrl Pts',(4.85068776978043,-51.354519323734,-8.4016376689476));
#19967=CARTESIAN_POINT('Ctrl Pts',(-1.51301029103127E-11,-51.179519323734,
-8.40163766893887));
#19968=CARTESIAN_POINT('Ctrl Pts',(-4.85068776981069,-51.004519323734,-8.40163766893014));
#19969=CARTESIAN_POINT('Ctrl Pts',(-7.2760316547009,-50.829519323734,-4.20081883445633));
#19970=CARTESIAN_POINT('Ctrl Pts',(-9.70137553959111,-50.654519323734,1.74701439383464E-11));
#19971=CARTESIAN_POINT('Ctrl Pts',(-7.27603165468577,-50.479519323734,4.20081883448254));
#19972=CARTESIAN_POINT('Ctrl Pts',(-4.85068776978043,-50.304519323734,8.40163766894761));
#19973=CARTESIAN_POINT('Ctrl Pts',(1.51290740064448E-11,-50.129519323734,
8.40163766893887));
#19974=CARTESIAN_POINT('Ctrl Pts',(4.85068776981068,-49.954519323734,8.40163766893014));
#19975=CARTESIAN_POINT('Ctrl Pts',(7.2760316547009,-49.779519323734,4.20081883445634));
#19976=CARTESIAN_POINT('Ctrl Pts',(9.70137553959111,-49.604519323734,-1.74689558624962E-11));
#19977=CARTESIAN_POINT('Ctrl Pts',(7.27603165468577,-49.429519323734,-4.20081883448253));
#19978=CARTESIAN_POINT('Ctrl Pts',(4.85068776978043,-49.254519323734,-8.4016376689476));
#19979=CARTESIAN_POINT('Ctrl Pts',(-1.51301029103127E-11,-49.079519323734,
-8.40163766893887));
#19980=CARTESIAN_POINT('Ctrl Pts',(-4.85068776981069,-48.904519323734,-8.40163766893014));
#19981=CARTESIAN_POINT('Ctrl Pts',(-7.2760316547009,-48.729519323734,-4.20081883445633));
#19982=CARTESIAN_POINT('Ctrl Pts',(-9.70137553959111,-48.554519323734,1.74701439383464E-11));
#19983=CARTESIAN_POINT('Ctrl Pts',(-7.27603165468577,-48.379519323734,4.20081883448254));
#19984=CARTESIAN_POINT('Ctrl Pts',(-4.85068776978043,-48.204519323734,8.40163766894761));
#19985=CARTESIAN_POINT('Ctrl Pts',(1.51290740064448E-11,-48.029519323734,
8.40163766893887));
#19986=CARTESIAN_POINT('Ctrl Pts',(4.85068776981068,-47.854519323734,8.40163766893014));
#19987=CARTESIAN_POINT('Ctrl Pts',(7.2760316547009,-47.679519323734,4.20081883445634));
#19988=CARTESIAN_POINT('Ctrl Pts',(9.70137553959111,-47.5045193237341,-1.74689558624962E-11));
#19989=CARTESIAN_POINT('Ctrl Pts',(7.27603165468577,-47.329519323734,-4.20081883448253));
#19990=CARTESIAN_POINT('Ctrl Pts',(4.85068776978043,-47.154519323734,-8.4016376689476));
#19991=CARTESIAN_POINT('Ctrl Pts',(-1.51301029103127E-11,-46.979519323734,
-8.40163766893887));
#19992=CARTESIAN_POINT('Ctrl Pts',(-4.85068776981069,-46.804519323734,-8.40163766893014));
#19993=CARTESIAN_POINT('Ctrl Pts',(-7.2760316547009,-46.629519323734,-4.20081883445633));
#19994=CARTESIAN_POINT('Ctrl Pts',(-9.70137553959111,-46.454519323734,1.74701439383464E-11));
#19995=CARTESIAN_POINT('Ctrl Pts',(-7.27603165468577,-46.279519323734,4.20081883448254));
#19996=CARTESIAN_POINT('Ctrl Pts',(-4.85068776978043,-46.104519323734,8.40163766894761));
#19997=CARTESIAN_POINT('Ctrl Pts',(1.51290740064448E-11,-45.929519323734,
8.40163766893887));
#19998=CARTESIAN_POINT('Ctrl Pts',(4.85068776981068,-45.754519323734,8.40163766893014));
#19999=CARTESIAN_POINT('Ctrl Pts',(7.2760316547009,-45.579519323734,4.20081883445634));
#20000=CARTESIAN_POINT('Ctrl Pts',(9.70137553959111,-45.404519323734,-1.74689558624962E-11));
#20001=CARTESIAN_POINT('Ctrl Pts',(7.27603165468577,-45.229519323734,-4.20081883448253));
#20002=CARTESIAN_POINT('Ctrl Pts',(4.85068776978043,-45.054519323734,-8.4016376689476));
#20003=CARTESIAN_POINT('Ctrl Pts',(-1.51301029103127E-11,-44.879519323734,
-8.40163766893887));
#20004=CARTESIAN_POINT('Ctrl Pts',(-4.85068776981069,-44.704519323734,-8.40163766893014));
#20005=CARTESIAN_POINT('Ctrl Pts',(-7.2760316547009,-44.529519323734,-4.20081883445633));
#20006=CARTESIAN_POINT('Ctrl Pts',(-9.70137553959111,-44.354519323734,1.74701439383464E-11));
#20007=CARTESIAN_POINT('Ctrl Pts',(-7.27603165468577,-44.179519323734,4.20081883448254));
#20008=CARTESIAN_POINT('Ctrl Pts',(-4.85068776978043,-44.004519323734,8.40163766894761));
#20009=CARTESIAN_POINT('Ctrl Pts',(1.51290740064448E-11,-43.829519323734,
8.40163766893887));
#20010=CARTESIAN_POINT('Ctrl Pts',(4.85068776981068,-43.654519323734,8.40163766893014));
#20011=CARTESIAN_POINT('Ctrl Pts',(7.2760316547009,-43.479519323734,4.20081883445634));
#20012=CARTESIAN_POINT('Ctrl Pts',(9.70137553959111,-43.304519323734,-1.74689558624962E-11));
#20013=CARTESIAN_POINT('Ctrl Pts',(7.27603165468577,-43.129519323734,-4.20081883448253));
#20014=CARTESIAN_POINT('Ctrl Pts',(4.85068776978043,-42.954519323734,-8.4016376689476));
#20015=CARTESIAN_POINT('Ctrl Pts',(-1.51301029103127E-11,-42.779519323734,
-8.40163766893887));
#20016=CARTESIAN_POINT('Ctrl Pts',(-4.85068776981069,-42.6045193237341,
-8.40163766893014));
#20017=CARTESIAN_POINT('Ctrl Pts',(-7.2760316547009,-42.429519323734,-4.20081883445633));
#20018=CARTESIAN_POINT('Ctrl Pts',(-9.70137553959111,-42.254519323734,1.74701439383464E-11));
#20019=CARTESIAN_POINT('Ctrl Pts',(-7.27603165468577,-42.079519323734,4.20081883448254));
#20020=CARTESIAN_POINT('Ctrl Pts',(-4.85068776978043,-41.904519323734,8.40163766894761));
#20021=CARTESIAN_POINT('Ctrl Pts',(1.51290740064448E-11,-41.729519323734,
8.40163766893887));
#20022=CARTESIAN_POINT('Ctrl Pts',(4.85068776981068,-41.554519323734,8.40163766893014));
#20023=CARTESIAN_POINT('Ctrl Pts',(7.2760316547009,-41.379519323734,4.20081883445634));
#20024=CARTESIAN_POINT('Ctrl Pts',(9.70137553959111,-41.2045193237341,-1.74689558624962E-11));
#20025=CARTESIAN_POINT('Ctrl Pts',(7.27603165468577,-41.029519323734,-4.20081883448253));
#20026=CARTESIAN_POINT('Ctrl Pts',(4.85068776978043,-40.854519323734,-8.4016376689476));
#20027=CARTESIAN_POINT('Ctrl Pts',(-1.51301029103127E-11,-40.679519323734,
-8.40163766893887));
#20028=CARTESIAN_POINT('Ctrl Pts',(-4.85068776981069,-40.504519323734,-8.40163766893014));
#20029=CARTESIAN_POINT('Ctrl Pts',(-7.2760316547009,-40.329519323734,-4.20081883445633));
#20030=CARTESIAN_POINT('Ctrl Pts',(-9.70137553959111,-40.154519323734,1.74701439383464E-11));
#20031=CARTESIAN_POINT('Ctrl Pts',(-7.27603165468577,-39.979519323734,4.20081883448254));
#20032=CARTESIAN_POINT('Ctrl Pts',(-4.85068776978043,-39.804519323734,8.40163766894761));
#20033=CARTESIAN_POINT('Ctrl Pts',(1.51290740064448E-11,-39.629519323734,
8.40163766893887));
#20034=CARTESIAN_POINT('Ctrl Pts',(4.85068776981068,-39.454519323734,8.40163766893014));
#20035=CARTESIAN_POINT('Ctrl Pts',(7.2760316547009,-39.279519323734,4.20081883445634));
#20036=CARTESIAN_POINT('Ctrl Pts',(9.70137553959111,-39.104519323734,-1.74689558624962E-11));
#20037=CARTESIAN_POINT('Ctrl Pts',(7.27603165468577,-38.929519323734,-4.20081883448253));
#20038=CARTESIAN_POINT('Ctrl Pts',(4.85068776978043,-38.7545193237341,-8.4016376689476));
#20039=CARTESIAN_POINT('Ctrl Pts',(-1.51301029103127E-11,-38.579519323734,
-8.40163766893887));
#20040=CARTESIAN_POINT('Ctrl Pts',(-4.85068776981069,-38.404519323734,-8.40163766893014));
#20041=CARTESIAN_POINT('Ctrl Pts',(-7.2760316547009,-38.2295193237341,-4.20081883445633));
#20042=CARTESIAN_POINT('Ctrl Pts',(-9.70137553959111,-38.054519323734,1.74701439383464E-11));
#20043=CARTESIAN_POINT('Ctrl Pts',(-7.27603165468577,-37.879519323734,4.20081883448254));
#20044=CARTESIAN_POINT('Ctrl Pts',(-4.85068776978043,-37.704519323734,8.40163766894761));
#20045=CARTESIAN_POINT('Ctrl Pts',(1.51290740064448E-11,-37.529519323734,
8.40163766893887));
#20046=CARTESIAN_POINT('Ctrl Pts',(4.85068776981068,-37.354519323734,8.40163766893014));
#20047=CARTESIAN_POINT('Ctrl Pts',(7.2760316547009,-37.179519323734,4.20081883445634));
#20048=CARTESIAN_POINT('Ctrl Pts',(9.70137553959111,-37.0045193237341,-1.74689558624962E-11));
#20049=CARTESIAN_POINT('Ctrl Pts',(7.27603165468577,-36.829519323734,-4.20081883448253));
#20050=CARTESIAN_POINT('Ctrl Pts',(4.85068776978043,-36.654519323734,-8.4016376689476));
#20051=CARTESIAN_POINT('Ctrl Pts',(-1.51301029103127E-11,-36.479519323734,
-8.40163766893887));
#20052=CARTESIAN_POINT('Ctrl Pts',(-4.85068776981069,-36.3045193237341,
-8.40163766893014));
#20053=CARTESIAN_POINT('Ctrl Pts',(-7.2760316547009,-36.129519323734,-4.20081883445633));
#20054=CARTESIAN_POINT('Ctrl Pts',(-9.70137553959111,-35.9545193237341,
1.74701439383464E-11));
#20055=CARTESIAN_POINT('Ctrl Pts',(-7.27603165468577,-35.779519323734,4.20081883448254));
#20056=CARTESIAN_POINT('Ctrl Pts',(-4.85068776978043,-35.604519323734,8.40163766894761));
#20057=CARTESIAN_POINT('Ctrl Pts',(1.51290740064448E-11,-35.429519323734,
8.40163766893887));
#20058=CARTESIAN_POINT('Ctrl Pts',(4.85068776981068,-35.2545193237341,8.40163766893014));
#20059=CARTESIAN_POINT('Ctrl Pts',(7.2760316547009,-35.079519323734,4.20081883445634));
#20060=CARTESIAN_POINT('Ctrl Pts',(9.70137553959111,-34.9045193237341,-1.74689558624962E-11));
#20061=CARTESIAN_POINT('Ctrl Pts',(7.27603165468577,-34.729519323734,-4.20081883448253));
#20062=CARTESIAN_POINT('Ctrl Pts',(4.85068776978043,-34.5545193237341,-8.4016376689476));
#20063=CARTESIAN_POINT('Ctrl Pts',(-1.51301029103127E-11,-34.3795193237341,
-8.40163766893887));
#20064=CARTESIAN_POINT('Ctrl Pts',(-4.85068776981069,-34.204519323734,-8.40163766893014));
#20065=CARTESIAN_POINT('Ctrl Pts',(-7.2760316547009,-34.029519323734,-4.20081883445633));
#20066=CARTESIAN_POINT('Ctrl Pts',(-9.70137553959111,-33.8545193237341,
1.74701439383464E-11));
#20067=CARTESIAN_POINT('Ctrl Pts',(-7.27603165468577,-33.679519323734,4.20081883448254));
#20068=CARTESIAN_POINT('Ctrl Pts',(-4.85068776978043,-33.504519323734,8.40163766894761));
#20069=CARTESIAN_POINT('Ctrl Pts',(1.51290740064448E-11,-33.3295193237341,
8.40163766893887));
#20070=CARTESIAN_POINT('Ctrl Pts',(4.85068776981068,-33.154519323734,8.40163766893014));
#20071=CARTESIAN_POINT('Ctrl Pts',(7.2760316547009,-32.9795193237341,4.20081883445634));
#20072=CARTESIAN_POINT('Ctrl Pts',(9.70137553959111,-32.8045193237341,-1.74689558624962E-11));
#20073=CARTESIAN_POINT('Ctrl Pts',(7.27603165468577,-32.6295193237341,-4.20081883448253));
#20074=CARTESIAN_POINT('Ctrl Pts',(4.85068776978043,-32.4545193237341,-8.4016376689476));
#20075=CARTESIAN_POINT('Ctrl Pts',(-1.51301029103127E-11,-32.279519323734,
-8.40163766893887));
#20076=CARTESIAN_POINT('Ctrl Pts',(-4.85068776981069,-32.1045193237341,
-8.40163766893014));
#20077=CARTESIAN_POINT('Ctrl Pts',(-7.2760316547009,-31.9295193237341,-4.20081883445633));
#20078=CARTESIAN_POINT('Ctrl Pts',(-9.70137553959111,-31.7545193237341,
1.74701439383464E-11));
#20079=CARTESIAN_POINT('Ctrl Pts',(-7.27603165468577,-31.5795193237341,
4.20081883448254));
#20080=CARTESIAN_POINT('Ctrl Pts',(-4.85068776978043,-31.4045193237341,
8.40163766894761));
#20081=CARTESIAN_POINT('Ctrl Pts',(1.51290740064448E-11,-31.2295193237341,
8.40163766893887));
#20082=CARTESIAN_POINT('Ctrl Pts',(4.85068776981068,-31.0545193237341,8.40163766893014));
#20083=CARTESIAN_POINT('Ctrl Pts',(7.2760316547009,-30.8795193237341,4.20081883445634));
#20084=CARTESIAN_POINT('Ctrl Pts',(9.70137553959111,-30.7045193237341,-1.74689558624962E-11));
#20085=CARTESIAN_POINT('Ctrl Pts',(7.27603165468577,-30.5295193237341,-4.20081883448253));
#20086=CARTESIAN_POINT('Ctrl Pts',(4.85068776978043,-30.3545193237341,-8.4016376689476));
#20087=CARTESIAN_POINT('Ctrl Pts',(-1.51301029103127E-11,-30.1795193237341,
-8.40163766893887));
#20088=CARTESIAN_POINT('Ctrl Pts',(-4.85068776981069,-30.0045193237341,
-8.40163766893014));
#20089=CARTESIAN_POINT('Ctrl Pts',(-7.2760316547009,-29.8295193237341,-4.20081883445633));
#20090=CARTESIAN_POINT('Ctrl Pts',(-9.70137553959111,-29.6545193237341,
1.74701439383464E-11));
#20091=CARTESIAN_POINT('Ctrl Pts',(-7.27603165468577,-29.4795193237341,
4.20081883448254));
#20092=CARTESIAN_POINT('Ctrl Pts',(-4.85068776978043,-29.3045193237341,
8.40163766894761));
#20093=CARTESIAN_POINT('Ctrl Pts',(1.51290740064448E-11,-29.1295193237341,
8.40163766893887));
#20094=CARTESIAN_POINT('Ctrl Pts',(4.85068776981068,-28.9545193237341,8.40163766893014));
#20095=CARTESIAN_POINT('Ctrl Pts',(7.2760316547009,-28.7795193237341,4.20081883445634));
#20096=CARTESIAN_POINT('Ctrl Pts',(9.70137553959111,-28.6045193237341,-1.74689558624962E-11));
#20097=CARTESIAN_POINT('Ctrl Pts',(7.27603165468577,-28.4295193237341,-4.20081883448253));
#20098=CARTESIAN_POINT('Ctrl Pts',(4.85068776978043,-28.2545193237341,-8.4016376689476));
#20099=CARTESIAN_POINT('Ctrl Pts',(-1.51301029103127E-11,-28.0795193237341,
-8.40163766893887));
#20100=CARTESIAN_POINT('Ctrl Pts',(-4.85068776981069,-27.9045193237341,
-8.40163766893014));
#20101=CARTESIAN_POINT('Ctrl Pts',(-7.2760316547009,-27.7295193237341,-4.20081883445633));
#20102=CARTESIAN_POINT('Ctrl Pts',(-9.70137553959111,-27.5545193237341,
1.74701439383464E-11));
#20103=CARTESIAN_POINT('Ctrl Pts',(-7.27603165468577,-27.3795193237341,
4.20081883448254));
#20104=CARTESIAN_POINT('Ctrl Pts',(-4.85068776978043,-27.2045193237341,
8.40163766894761));
#20105=CARTESIAN_POINT('Ctrl Pts',(1.51290740064448E-11,-27.0295193237341,
8.40163766893887));
#20106=CARTESIAN_POINT('Ctrl Pts',(4.85068776981068,-26.8545193237341,8.40163766893014));
#20107=CARTESIAN_POINT('Ctrl Pts',(7.2760316547009,-26.6795193237341,4.20081883445634));
#20108=CARTESIAN_POINT('Ctrl Pts',(9.70137553959111,-26.5045193237341,-1.74689558624962E-11));
#20109=CARTESIAN_POINT('Ctrl Pts',(7.27603165468577,-26.3295193237341,-4.20081883448253));
#20110=CARTESIAN_POINT('Ctrl Pts',(4.85068776978043,-26.1545193237341,-8.4016376689476));
#20111=CARTESIAN_POINT('Ctrl Pts',(-1.51301029103127E-11,-25.9795193237341,
-8.40163766893887));
#20112=CARTESIAN_POINT('Ctrl Pts',(-4.85068776981069,-25.8045193237341,
-8.40163766893014));
#20113=CARTESIAN_POINT('Ctrl Pts',(-7.2760316547009,-25.6295193237341,-4.20081883445633));
#20114=CARTESIAN_POINT('Ctrl Pts',(-9.70137553959111,-25.4545193237341,
1.74701439383464E-11));
#20115=CARTESIAN_POINT('Ctrl Pts',(-7.27603165468577,-25.2795193237341,
4.20081883448254));
#20116=CARTESIAN_POINT('Ctrl Pts',(-4.85068776978043,-25.1045193237341,
8.40163766894761));
#20117=CARTESIAN_POINT('Ctrl Pts',(1.51290740064448E-11,-24.9295193237341,
8.40163766893887));
#20118=CARTESIAN_POINT('Ctrl Pts',(4.85068776981068,-24.7545193237341,8.40163766893014));
#20119=CARTESIAN_POINT('Ctrl Pts',(7.2760316547009,-24.5795193237341,4.20081883445634));
#20120=CARTESIAN_POINT('Ctrl Pts',(9.70137553959111,-24.4045193237341,-1.74689558624962E-11));
#20121=CARTESIAN_POINT('Ctrl Pts',(7.27603165468577,-24.2295193237341,-4.20081883448253));
#20122=CARTESIAN_POINT('Ctrl Pts',(4.85068776978043,-24.0545193237341,-8.4016376689476));
#20123=CARTESIAN_POINT('Ctrl Pts',(-1.51301029103127E-11,-23.8795193237341,
-8.40163766893887));
#20124=CARTESIAN_POINT('Ctrl Pts',(-4.85068776981069,-23.7045193237341,
-8.40163766893014));
#20125=CARTESIAN_POINT('Ctrl Pts',(-7.2760316547009,-23.5295193237341,-4.20081883445633));
#20126=CARTESIAN_POINT('Ctrl Pts',(-9.70137553959111,-23.3545193237341,
1.74701439383464E-11));
#20127=CARTESIAN_POINT('Ctrl Pts',(-7.27603165468577,-23.1795193237341,
4.20081883448254));
#20128=CARTESIAN_POINT('Ctrl Pts',(-4.85068776978043,-23.0045193237341,
8.40163766894761));
#20129=CARTESIAN_POINT('Ctrl Pts',(1.51290740064448E-11,-22.8295193237341,
8.40163766893887));
#20130=CARTESIAN_POINT('Ctrl Pts',(4.85068776981068,-22.6545193237341,8.40163766893014));
#20131=CARTESIAN_POINT('Ctrl Pts',(7.2760316547009,-22.4795193237341,4.20081883445634));
#20132=CARTESIAN_POINT('Ctrl Pts',(9.70137553959111,-22.3045193237341,-1.74689558624962E-11));
#20133=CARTESIAN_POINT('Ctrl Pts',(7.27603165468577,-22.1295193237341,-4.20081883448253));
#20134=CARTESIAN_POINT('Ctrl Pts',(4.85068776978043,-21.9545193237341,-8.4016376689476));
#20135=CARTESIAN_POINT('Ctrl Pts',(-1.51301029103127E-11,-21.7795193237341,
-8.40163766893887));
#20136=CARTESIAN_POINT('Ctrl Pts',(-4.85068776981069,-21.6045193237341,
-8.40163766893014));
#20137=CARTESIAN_POINT('Ctrl Pts',(-7.2760316547009,-21.4295193237341,-4.20081883445633));
#20138=CARTESIAN_POINT('Ctrl Pts',(-9.70137553959111,-21.2545193237341,
1.74701439383464E-11));
#20139=CARTESIAN_POINT('Ctrl Pts',(-7.27603165468577,-21.0795193237341,
4.20081883448254));
#20140=CARTESIAN_POINT('Ctrl Pts',(-4.85068776978043,-20.9045193237341,
8.40163766894761));
#20141=CARTESIAN_POINT('Ctrl Pts',(1.51290740064448E-11,-20.7295193237341,
8.40163766893887));
#20142=CARTESIAN_POINT('Ctrl Pts',(4.85068776981068,-20.5545193237341,8.40163766893014));
#20143=CARTESIAN_POINT('Ctrl Pts',(7.2760316547009,-20.3795193237341,4.20081883445634));
#20144=CARTESIAN_POINT('Ctrl Pts',(9.70137553959111,-20.2045193237341,-1.74689558624962E-11));
#20145=CARTESIAN_POINT('Ctrl Pts',(7.27603165468577,-20.0295193237341,-4.20081883448253));
#20146=CARTESIAN_POINT('Ctrl Pts',(4.85068776978043,-19.8545193237341,-8.4016376689476));
#20147=CARTESIAN_POINT('Ctrl Pts',(-1.51301029103127E-11,-19.6795193237341,
-8.40163766893887));
#20148=CARTESIAN_POINT('Ctrl Pts',(-4.85068776981069,-19.5045193237341,
-8.40163766893014));
#20149=CARTESIAN_POINT('Ctrl Pts',(-7.2760316547009,-19.3295193237341,-4.20081883445633));
#20150=CARTESIAN_POINT('Ctrl Pts',(-9.70137553959111,-19.1545193237341,
1.74701439383464E-11));
#20151=CARTESIAN_POINT('Ctrl Pts',(-7.27603165468577,-18.9795193237341,
4.20081883448254));
#20152=CARTESIAN_POINT('Ctrl Pts',(-4.85068776978043,-18.8045193237341,
8.40163766894761));
#20153=CARTESIAN_POINT('Ctrl Pts',(1.51290740064448E-11,-18.6295193237341,
8.40163766893887));
#20154=CARTESIAN_POINT('Ctrl Pts',(4.85068776981068,-18.4545193237341,8.40163766893014));
#20155=CARTESIAN_POINT('Ctrl Pts',(7.2760316547009,-18.2795193237341,4.20081883445634));
#20156=CARTESIAN_POINT('Ctrl Pts',(9.70137553959111,-18.1045193237341,-1.74689558624962E-11));
#20157=CARTESIAN_POINT('Ctrl Pts',(7.27603165468577,-17.9295193237341,-4.20081883448253));
#20158=CARTESIAN_POINT('Ctrl Pts',(4.85068776978043,-17.7545193237341,-8.4016376689476));
#20159=CARTESIAN_POINT('Ctrl Pts',(-1.51301029103127E-11,-17.5795193237341,
-8.40163766893887));
#20160=CARTESIAN_POINT('Ctrl Pts',(-4.85068776981069,-17.4045193237341,
-8.40163766893014));
#20161=CARTESIAN_POINT('Ctrl Pts',(-7.2760316547009,-17.2295193237341,-4.20081883445633));
#20162=CARTESIAN_POINT('Ctrl Pts',(-9.70137553959111,-17.0545193237341,
1.74701439383464E-11));
#20163=CARTESIAN_POINT('Ctrl Pts',(-7.27603165468577,-16.8795193237341,
4.20081883448254));
#20164=CARTESIAN_POINT('Ctrl Pts',(-4.85068776978043,-16.7045193237341,
8.40163766894761));
#20165=CARTESIAN_POINT('Ctrl Pts',(1.51290740064448E-11,-16.5295193237341,
8.40163766893887));
#20166=CARTESIAN_POINT('Ctrl Pts',(4.85068776981068,-16.3545193237341,8.40163766893014));
#20167=CARTESIAN_POINT('Ctrl Pts',(7.2760316547009,-16.1795193237341,4.20081883445634));
#20168=CARTESIAN_POINT('Ctrl Pts',(9.70137553959111,-16.0045193237341,-1.74689558624962E-11));
#20169=CARTESIAN_POINT('Ctrl Pts',(7.27603165468577,-15.8295193237341,-4.20081883448253));
#20170=CARTESIAN_POINT('Ctrl Pts',(4.85068776978043,-15.6545193237341,-8.4016376689476));
#20171=CARTESIAN_POINT('Ctrl Pts',(-1.51301029103127E-11,-15.4795193237341,
-8.40163766893887));
#20172=CARTESIAN_POINT('Ctrl Pts',(-4.85068776981069,-15.3045193237341,
-8.40163766893014));
#20173=CARTESIAN_POINT('Ctrl Pts',(-7.2760316547009,-15.1295193237341,-4.20081883445633));
#20174=CARTESIAN_POINT('Ctrl Pts',(-9.70137553959111,-14.9545193237341,
1.74701439383464E-11));
#20175=CARTESIAN_POINT('Ctrl Pts',(-7.27603165468577,-14.7795193237341,
4.20081883448254));
#20176=CARTESIAN_POINT('Ctrl Pts',(-4.85068776978043,-14.6045193237341,
8.40163766894761));
#20177=CARTESIAN_POINT('Ctrl Pts',(1.51290740064448E-11,-14.4295193237341,
8.40163766893887));
#20178=CARTESIAN_POINT('Ctrl Pts',(4.85068776981068,-14.2545193237341,8.40163766893014));
#20179=CARTESIAN_POINT('Ctrl Pts',(7.2760316547009,-14.0795193237341,4.20081883445634));
#20180=CARTESIAN_POINT('Ctrl Pts',(9.70137553959111,-13.9045193237341,-1.74689558624962E-11));
#20181=CARTESIAN_POINT('Ctrl Pts',(7.27603165468577,-13.7295193237341,-4.20081883448253));
#20182=CARTESIAN_POINT('Ctrl Pts',(4.85068776978043,-13.5545193237341,-8.4016376689476));
#20183=CARTESIAN_POINT('Ctrl Pts',(-1.51301029103127E-11,-13.3795193237341,
-8.40163766893887));
#20184=CARTESIAN_POINT('Ctrl Pts',(-4.85068776981069,-13.2045193237341,
-8.40163766893014));
#20185=CARTESIAN_POINT('Ctrl Pts',(-7.2760316547009,-13.0295193237341,-4.20081883445633));
#20186=CARTESIAN_POINT('Ctrl Pts',(-9.70137553959111,-12.8545193237341,
1.74701439383464E-11));
#20187=CARTESIAN_POINT('Ctrl Pts',(-7.27603165468577,-12.6795193237341,
4.20081883448254));
#20188=CARTESIAN_POINT('Ctrl Pts',(-4.85068776978043,-12.5045193237341,
8.40163766894761));
#20189=CARTESIAN_POINT('Ctrl Pts',(1.51290740064448E-11,-12.3295193237341,
8.40163766893887));
#20190=CARTESIAN_POINT('Ctrl Pts',(4.85068776981068,-12.1545193237341,8.40163766893014));
#20191=CARTESIAN_POINT('Ctrl Pts',(7.2760316547009,-11.9795193237341,4.20081883445634));
#20192=CARTESIAN_POINT('Ctrl Pts',(9.70137553959111,-11.8045193237341,-1.74689558624962E-11));
#20193=CARTESIAN_POINT('Ctrl Pts',(7.27603165468577,-11.6295193237341,-4.20081883448253));
#20194=CARTESIAN_POINT('Ctrl Pts',(4.85068776978043,-11.4545193237341,-8.4016376689476));
#20195=CARTESIAN_POINT('Ctrl Pts',(-1.51301029103127E-11,-11.2795193237341,
-8.40163766893887));
#20196=CARTESIAN_POINT('Ctrl Pts',(-4.85068776981069,-11.1045193237341,
-8.40163766893014));
#20197=CARTESIAN_POINT('Ctrl Pts',(-7.2760316547009,-10.9295193237341,-4.20081883445633));
#20198=CARTESIAN_POINT('Ctrl Pts',(-9.70137553959111,-10.7545193237341,
1.74701439383464E-11));
#20199=CARTESIAN_POINT('Ctrl Pts',(-7.27603165468577,-10.5795193237341,
4.20081883448254));
#20200=CARTESIAN_POINT('Ctrl Pts',(-4.85068776978043,-10.4045193237341,
8.40163766894761));
#20201=CARTESIAN_POINT('Ctrl Pts',(1.51290740064448E-11,-10.2295193237341,
8.40163766893887));
#20202=CARTESIAN_POINT('Ctrl Pts',(4.85068776981068,-10.0545193237341,8.40163766893014));
#20203=CARTESIAN_POINT('Ctrl Pts',(7.2760316547009,-9.87951932373411,4.20081883445634));
#20204=CARTESIAN_POINT('Ctrl Pts',(9.70137553959111,-9.70451932373411,-1.74689558624962E-11));
#20205=CARTESIAN_POINT('Ctrl Pts',(7.27603165468577,-9.5295193237341,-4.20081883448253));
#20206=CARTESIAN_POINT('Ctrl Pts',(4.85068776978043,-9.35451932373412,-8.4016376689476));
#20207=CARTESIAN_POINT('Ctrl Pts',(-1.51301029103127E-11,-9.17951932373411,
-8.40163766893887));
#20208=CARTESIAN_POINT('Ctrl Pts',(-4.85068776981069,-9.00451932373411,
-8.40163766893014));
#20209=CARTESIAN_POINT('Ctrl Pts',(-7.2760316547009,-8.82951932373412,-4.20081883445633));
#20210=CARTESIAN_POINT('Ctrl Pts',(-9.70137553959111,-8.65451932373411,
1.74701439383464E-11));
#20211=CARTESIAN_POINT('Ctrl Pts',(-7.27603165468577,-8.4795193237341,4.20081883448254));
#20212=CARTESIAN_POINT('Ctrl Pts',(-4.85068776978043,-8.30451932373413,
8.40163766894761));
#20213=CARTESIAN_POINT('Ctrl Pts',(1.51290740064448E-11,-8.12951932373411,
8.40163766893887));
#20214=CARTESIAN_POINT('Ctrl Pts',(4.85068776981068,-7.95451932373411,8.40163766893014));
#20215=CARTESIAN_POINT('Ctrl Pts',(7.2760316547009,-7.77951932373412,4.20081883445634));
#20216=CARTESIAN_POINT('Ctrl Pts',(9.70137553959111,-7.60451932373411,-1.74689558624962E-11));
#20217=CARTESIAN_POINT('Ctrl Pts',(7.27603165468577,-7.42951932373411,-4.20081883448253));
#20218=CARTESIAN_POINT('Ctrl Pts',(4.85068776978043,-7.25451932373413,-8.4016376689476));
#20219=CARTESIAN_POINT('Ctrl Pts',(-1.51301029103127E-11,-7.07951932373412,
-8.40163766893887));
#20220=CARTESIAN_POINT('Ctrl Pts',(-4.85068776981069,-6.90451932373412,
-8.40163766893014));
#20221=CARTESIAN_POINT('Ctrl Pts',(-7.2760316547009,-6.7295193237341,-4.20081883445633));
#20222=CARTESIAN_POINT('Ctrl Pts',(-9.70137553959111,-6.55451932373412,
1.74701439383464E-11));
#20223=CARTESIAN_POINT('Ctrl Pts',(-7.27603165468577,-6.37951932373411,
4.20081883448254));
#20224=CARTESIAN_POINT('Ctrl Pts',(-4.85068776978043,-6.2045193237341,8.40163766894761));
#20225=CARTESIAN_POINT('Ctrl Pts',(1.51290740064448E-11,-6.02951932373412,
8.40163766893887));
#20226=CARTESIAN_POINT('Ctrl Pts',(4.85068776981068,-5.85451932373412,8.40163766893014));
#20227=CARTESIAN_POINT('Ctrl Pts',(7.2760316547009,-5.6795193237341,4.20081883445634));
#20228=CARTESIAN_POINT('Ctrl Pts',(9.70137553959111,-5.50451932373412,-1.74689558624962E-11));
#20229=CARTESIAN_POINT('Ctrl Pts',(7.27603165468577,-5.32951932373411,-4.20081883448253));
#20230=CARTESIAN_POINT('Ctrl Pts',(4.85068776978043,-5.15451932373411,-8.4016376689476));
#20231=CARTESIAN_POINT('Ctrl Pts',(-1.51301029103127E-11,-4.97951932373413,
-8.40163766893887));
#20232=CARTESIAN_POINT('Ctrl Pts',(-4.85068776981069,-4.80451932373413,
-8.40163766893014));
#20233=CARTESIAN_POINT('Ctrl Pts',(-7.2760316547009,-4.62951932373411,-4.20081883445633));
#20234=CARTESIAN_POINT('Ctrl Pts',(-9.70137553959111,-4.45451932373413,
1.74701439383464E-11));
#20235=CARTESIAN_POINT('Ctrl Pts',(-7.27603165468577,-4.27951932373412,
4.20081883448254));
#20236=CARTESIAN_POINT('Ctrl Pts',(-4.85068776978043,-4.10451932373411,
8.40163766894761));
#20237=CARTESIAN_POINT('Ctrl Pts',(1.51290740064448E-11,-3.92951932373413,
8.40163766893887));
#20238=CARTESIAN_POINT('Ctrl Pts',(4.85068776981068,-3.75451932373413,8.40163766893014));
#20239=CARTESIAN_POINT('Ctrl Pts',(7.2760316547009,-3.57951932373411,4.20081883445634));
#20240=CARTESIAN_POINT('Ctrl Pts',(9.70137553959111,-3.40451932373413,-1.74689558624962E-11));
#20241=CARTESIAN_POINT('Ctrl Pts',(7.27603165468577,-3.22951932373412,-4.20081883448253));
#20242=CARTESIAN_POINT('Ctrl Pts',(4.85068776978043,-3.05451932373412,-8.4016376689476));
#20243=CARTESIAN_POINT('Ctrl Pts',(-1.51301029103127E-11,-2.87951932373413,
-8.40163766893887));
#20244=CARTESIAN_POINT('Ctrl Pts',(-4.85068776981069,-2.70451932373414,
-8.40163766893014));
#20245=CARTESIAN_POINT('Ctrl Pts',(-7.2760316547009,-2.52951932373412,-4.20081883445633));
#20246=CARTESIAN_POINT('Ctrl Pts',(-9.70137553959111,-2.35451932373412,
1.74701439383464E-11));
#20247=CARTESIAN_POINT('Ctrl Pts',(-7.27603165468577,-2.17951932373413,
4.20081883448254));
#20248=CARTESIAN_POINT('Ctrl Pts',(-4.85068776978043,-2.00451932373412,
8.40163766894761));
#20249=CARTESIAN_POINT('Ctrl Pts',(1.51290740064448E-11,-1.82951932373411,
8.40163766893887));
#20250=CARTESIAN_POINT('Ctrl Pts',(4.85068776981068,-1.65451932373413,8.40163766893014));
#20251=CARTESIAN_POINT('Ctrl Pts',(7.2760316547009,-1.47951932373412,4.20081883445634));
#20252=CARTESIAN_POINT('Ctrl Pts',(9.70137553959111,-1.30451932373412,-1.74689558624962E-11));
#20253=CARTESIAN_POINT('Ctrl Pts',(7.27603165468577,-1.12951932373413,-4.20081883448253));
#20254=CARTESIAN_POINT('Ctrl Pts',(4.85068776978043,-0.954519323734127,
-8.4016376689476));
#20255=CARTESIAN_POINT('Ctrl Pts',(-1.51301029103127E-11,-0.779519323734116,
-8.40163766893887));
#20256=CARTESIAN_POINT('Ctrl Pts',(-4.85068776981069,-0.604519323734136,
-8.40163766893014));
#20257=CARTESIAN_POINT('Ctrl Pts',(-7.2760316547009,-0.429519323734127,
-4.20081883445633));
#20258=CARTESIAN_POINT('Ctrl Pts',(-9.70137553959111,-0.254519323734122,
1.74701439383464E-11));
#20259=CARTESIAN_POINT('Ctrl Pts',(-7.27603165468577,-0.0795193237341377,
4.20081883448254));
#20260=CARTESIAN_POINT('Ctrl Pts',(-4.85068776978043,0.0954806762658689,
8.40163766894761));
#20261=CARTESIAN_POINT('Ctrl Pts',(1.51290740064448E-11,0.270480676265879,
8.40163766893887));
#20262=CARTESIAN_POINT('Ctrl Pts',(4.85068776981068,0.445480676265859,8.40163766893014));
#20263=CARTESIAN_POINT('Ctrl Pts',(7.2760316547009,0.620480676265869,4.20081883445634));
#20264=CARTESIAN_POINT('Ctrl Pts',(9.70137553959111,0.795480676265874,-1.74689558624962E-11));
#20265=CARTESIAN_POINT('Ctrl Pts',(7.27603165468577,0.970480676265858,-4.20081883448253));
#20266=CARTESIAN_POINT('Ctrl Pts',(4.85068776978043,1.14548067626586,-8.4016376689476));
#20267=CARTESIAN_POINT('Ctrl Pts',(-1.51301029103127E-11,1.32048067626587,
-8.40163766893887));
#20268=CARTESIAN_POINT('Ctrl Pts',(-4.85068776981069,1.49548067626586,-8.40163766893014));
#20269=CARTESIAN_POINT('Ctrl Pts',(-7.2760316547009,1.67048067626586,-4.20081883445633));
#20270=CARTESIAN_POINT('Ctrl Pts',(-9.70137553959111,1.84548067626587,1.74701439383464E-11));
#20271=CARTESIAN_POINT('Ctrl Pts',(-7.27603165468577,2.02048067626588,4.20081883448254));
#20272=CARTESIAN_POINT('Ctrl Pts',(-4.85068776978043,2.19548067626586,8.40163766894761));
#20273=CARTESIAN_POINT('Ctrl Pts',(1.51290740064448E-11,2.37048067626587,
8.40163766893887));
#20274=CARTESIAN_POINT('Ctrl Pts',(4.85068776981068,2.54548067626587,8.40163766893014));
#20275=CARTESIAN_POINT('Ctrl Pts',(7.2760316547009,2.72048067626586,4.20081883445634));
#20276=CARTESIAN_POINT('Ctrl Pts',(9.70137553959111,2.89548067626586,-1.74689558624962E-11));
#20277=CARTESIAN_POINT('Ctrl Pts',(7.27603165468577,3.07048067626588,-4.20081883448253));
#20278=CARTESIAN_POINT('Ctrl Pts',(4.85068776978043,3.24548067626586,-8.4016376689476));
#20279=CARTESIAN_POINT('Ctrl Pts',(-1.51301029103127E-11,3.42048067626587,
-8.40163766893887));
#20280=CARTESIAN_POINT('Ctrl Pts',(-4.85068776981069,3.59548067626587,-8.40163766893014));
#20281=CARTESIAN_POINT('Ctrl Pts',(-7.2760316547009,3.77048067626585,-4.20081883445633));
#20282=CARTESIAN_POINT('Ctrl Pts',(-9.70137553959111,3.94548067626586,1.74701439383464E-11));
#20283=CARTESIAN_POINT('Ctrl Pts',(-7.27603165468577,4.12048067626587,4.20081883448254));
#20284=CARTESIAN_POINT('Ctrl Pts',(-4.85068776978043,4.29548067626585,8.40163766894761));
#20285=CARTESIAN_POINT('Ctrl Pts',(1.51290740064448E-11,4.47048067626586,
8.40163766893887));
#20286=CARTESIAN_POINT('Ctrl Pts',(4.85068776981068,4.64548067626587,8.40163766893014));
#20287=CARTESIAN_POINT('Ctrl Pts',(7.2760316547009,4.82048067626585,4.20081883445634));
#20288=CARTESIAN_POINT('Ctrl Pts',(9.70137553959111,4.99548067626586,-1.74689558624962E-11));
#20289=CARTESIAN_POINT('Ctrl Pts',(7.27603165468577,5.17048067626587,-4.20081883448253));
#20290=CARTESIAN_POINT('Ctrl Pts',(4.85068776978043,5.34548067626585,-8.4016376689476));
#20291=CARTESIAN_POINT('Ctrl Pts',(-1.51301029103127E-11,5.52048067626585,
-8.40163766893887));
#20292=CARTESIAN_POINT('Ctrl Pts',(-4.85068776981069,5.69548067626586,-8.40163766893014));
#20293=CARTESIAN_POINT('Ctrl Pts',(-7.2760316547009,5.87048067626585,-4.20081883445633));
#20294=CARTESIAN_POINT('Ctrl Pts',(-9.70137553959111,6.04548067626585,1.74701439383464E-11));
#20295=CARTESIAN_POINT('Ctrl Pts',(-7.27603165468577,6.22048067626586,4.20081883448254));
#20296=CARTESIAN_POINT('Ctrl Pts',(-4.85068776978043,6.39548067626584,8.40163766894761));
#20297=CARTESIAN_POINT('Ctrl Pts',(1.51290740064448E-11,6.57048067626585,
8.40163766893887));
#20298=CARTESIAN_POINT('Ctrl Pts',(4.85068776981068,6.74548067626586,8.40163766893014));
#20299=CARTESIAN_POINT('Ctrl Pts',(7.2760316547009,6.92048067626587,4.20081883445634));
#20300=CARTESIAN_POINT('Ctrl Pts',(9.70137553959111,7.09548067626585,-1.74689558624962E-11));
#20301=CARTESIAN_POINT('Ctrl Pts',(7.27603165468577,7.27048067626586,-4.20081883448253));
#20302=CARTESIAN_POINT('Ctrl Pts',(4.85068776978043,7.44548067626586,-8.4016376689476));
#20303=CARTESIAN_POINT('Ctrl Pts',(-1.51301029103127E-11,7.62048067626585,
-8.40163766893887));
#20304=CARTESIAN_POINT('Ctrl Pts',(-4.85068776981069,7.79548067626585,-8.40163766893014));
#20305=CARTESIAN_POINT('Ctrl Pts',(-7.2760316547009,7.97048067626586,-4.20081883445633));
#20306=CARTESIAN_POINT('Ctrl Pts',(-9.70137553959111,8.14548067626584,1.74701439383464E-11));
#20307=CARTESIAN_POINT('Ctrl Pts',(-7.27603165468577,8.32048067626585,4.20081883448254));
#20308=CARTESIAN_POINT('Ctrl Pts',(-4.85068776978043,8.49548067626586,8.40163766894761));
#20309=CARTESIAN_POINT('Ctrl Pts',(1.51290740064448E-11,8.67048067626584,
8.40163766893887));
#20310=CARTESIAN_POINT('Ctrl Pts',(4.85068776981068,8.84548067626585,8.40163766893014));
#20311=CARTESIAN_POINT('Ctrl Pts',(7.2760316547009,9.02048067626586,4.20081883445634));
#20312=CARTESIAN_POINT('Ctrl Pts',(9.70137553959111,9.19548067626584,-1.74689558624962E-11));
#20313=CARTESIAN_POINT('Ctrl Pts',(7.27603165468577,9.37048067626585,-4.20081883448253));
#20314=CARTESIAN_POINT('Ctrl Pts',(4.85068776978043,9.54548067626585,-8.4016376689476));
#20315=CARTESIAN_POINT('Ctrl Pts',(-1.51301029103127E-11,9.72048067626584,
-8.40163766893887));
#20316=CARTESIAN_POINT('Ctrl Pts',(-4.85068776981069,9.89548067626584,-8.40163766893014));
#20317=CARTESIAN_POINT('Ctrl Pts',(-7.2760316547009,10.0704806762659,-4.20081883445633));
#20318=CARTESIAN_POINT('Ctrl Pts',(-9.70137553959111,10.2454806762658,1.74701439383464E-11));
#20319=CARTESIAN_POINT('Ctrl Pts',(-7.27603165468577,10.4204806762658,4.20081883448254));
#20320=CARTESIAN_POINT('Ctrl Pts',(-4.85068776978043,10.5954806762658,8.40163766894761));
#20321=CARTESIAN_POINT('Ctrl Pts',(1.51290740064448E-11,10.7704806762658,
8.40163766893887));
#20322=CARTESIAN_POINT('Ctrl Pts',(4.85068776981068,10.9454806762658,8.40163766893014));
#20323=CARTESIAN_POINT('Ctrl Pts',(7.2760316547009,11.1204806762658,4.20081883445634));
#20324=CARTESIAN_POINT('Ctrl Pts',(9.70137553959111,11.2954806762659,-1.74689558624962E-11));
#20325=CARTESIAN_POINT('Ctrl Pts',(7.27603165468577,11.4704806762658,-4.20081883448253));
#20326=CARTESIAN_POINT('Ctrl Pts',(4.85068776978043,11.6454806762658,-8.4016376689476));
#20327=CARTESIAN_POINT('Ctrl Pts',(-1.51301029103127E-11,11.8204806762659,
-8.40163766893887));
#20328=CARTESIAN_POINT('Ctrl Pts',(-4.85068776981069,11.9954806762658,-8.40163766893014));
#20329=CARTESIAN_POINT('Ctrl Pts',(-7.2760316547009,12.1704806762658,-4.20081883445633));
#20330=CARTESIAN_POINT('Ctrl Pts',(-9.70137553959111,12.3454806762658,1.74701439383464E-11));
#20331=CARTESIAN_POINT('Ctrl Pts',(-7.27603165468577,12.5204806762658,4.20081883448254));
#20332=CARTESIAN_POINT('Ctrl Pts',(-4.85068776978043,12.6954806762658,8.40163766894761));
#20333=CARTESIAN_POINT('Ctrl Pts',(1.51290740064448E-11,12.8704806762659,
8.40163766893887));
#20334=CARTESIAN_POINT('Ctrl Pts',(4.85068776981068,13.0454806762658,8.40163766893014));
#20335=CARTESIAN_POINT('Ctrl Pts',(7.2760316547009,13.2204806762658,4.20081883445634));
#20336=CARTESIAN_POINT('Ctrl Pts',(9.70137553959111,13.3954806762658,-1.74689558624962E-11));
#20337=CARTESIAN_POINT('Ctrl Pts',(7.27603165468577,13.5704806762658,-4.20081883448253));
#20338=CARTESIAN_POINT('Ctrl Pts',(4.85068776978043,13.7454806762658,-8.4016376689476));
#20339=CARTESIAN_POINT('Ctrl Pts',(-1.51301029103127E-11,13.9204806762658,
-8.40163766893887));
#20340=CARTESIAN_POINT('Ctrl Pts',(-4.85068776981069,14.0954806762658,-8.40163766893014));
#20341=CARTESIAN_POINT('Ctrl Pts',(-7.2760316547009,14.2704806762658,-4.20081883445633));
#20342=CARTESIAN_POINT('Ctrl Pts',(-9.70137553959111,14.4454806762658,1.74701439383464E-11));
#20343=CARTESIAN_POINT('Ctrl Pts',(-7.27603165468577,14.6204806762658,4.20081883448254));
#20344=CARTESIAN_POINT('Ctrl Pts',(-4.85068776978043,14.7954806762658,8.40163766894761));
#20345=CARTESIAN_POINT('Ctrl Pts',(1.51290740064448E-11,14.9704806762658,
8.40163766893887));
#20346=CARTESIAN_POINT('Ctrl Pts',(4.85068776981068,15.1454806762658,8.40163766893014));
#20347=CARTESIAN_POINT('Ctrl Pts',(7.2760316547009,15.3204806762658,4.20081883445634));
#20348=CARTESIAN_POINT('Ctrl Pts',(9.70137553959111,15.4954806762658,-1.74689558624962E-11));
#20349=CARTESIAN_POINT('Ctrl Pts',(7.27603165468577,15.6704806762658,-4.20081883448253));
#20350=CARTESIAN_POINT('Ctrl Pts',(4.85068776978043,15.8454806762658,-8.4016376689476));
#20351=CARTESIAN_POINT('Ctrl Pts',(-1.51301029103127E-11,16.0204806762658,
-8.40163766893887));
#20352=CARTESIAN_POINT('Ctrl Pts',(-4.85068776981069,16.1954806762658,-8.40163766893014));
#20353=CARTESIAN_POINT('Ctrl Pts',(-7.2760316547009,16.3704806762658,-4.20081883445633));
#20354=CARTESIAN_POINT('Ctrl Pts',(-9.70137553959111,16.5454806762658,1.74701439383464E-11));
#20355=CARTESIAN_POINT('Ctrl Pts',(-7.27603165468577,16.7204806762658,4.20081883448254));
#20356=CARTESIAN_POINT('Ctrl Pts',(-4.85068776978043,16.8954806762658,8.40163766894761));
#20357=CARTESIAN_POINT('Ctrl Pts',(1.51290740064448E-11,17.0704806762658,
8.40163766893887));
#20358=CARTESIAN_POINT('Ctrl Pts',(4.85068776981068,17.2454806762658,8.40163766893014));
#20359=CARTESIAN_POINT('Ctrl Pts',(7.2760316547009,17.4204806762658,4.20081883445634));
#20360=CARTESIAN_POINT('Ctrl Pts',(9.70137553959111,17.5954806762658,-1.74689558624962E-11));
#20361=CARTESIAN_POINT('Ctrl Pts',(7.27603165468577,17.7704806762658,-4.20081883448253));
#20362=CARTESIAN_POINT('Ctrl Pts',(4.85068776978043,17.9454806762658,-8.4016376689476));
#20363=CARTESIAN_POINT('Ctrl Pts',(-1.51301029103127E-11,18.1204806762658,
-8.40163766893887));
#20364=CARTESIAN_POINT('Ctrl Pts',(-4.85068776981069,18.2954806762658,-8.40163766893014));
#20365=CARTESIAN_POINT('Ctrl Pts',(-7.2760316547009,18.4704806762658,-4.20081883445633));
#20366=CARTESIAN_POINT('Ctrl Pts',(-9.70137553959111,18.6454806762658,1.74701439383464E-11));
#20367=CARTESIAN_POINT('Ctrl Pts',(-7.27603165468577,18.8204806762658,4.20081883448254));
#20368=CARTESIAN_POINT('Ctrl Pts',(-4.85068776978043,18.9954806762658,8.40163766894761));
#20369=CARTESIAN_POINT('Ctrl Pts',(1.51290740064448E-11,19.1704806762658,
8.40163766893887));
#20370=CARTESIAN_POINT('Ctrl Pts',(4.85068776981068,19.3454806762658,8.40163766893014));
#20371=CARTESIAN_POINT('Ctrl Pts',(7.2760316547009,19.5204806762658,4.20081883445634));
#20372=CARTESIAN_POINT('Ctrl Pts',(9.70137553959111,19.6954806762658,-1.74689558624962E-11));
#20373=CARTESIAN_POINT('Ctrl Pts',(7.27603165468577,19.8704806762658,-4.20081883448253));
#20374=CARTESIAN_POINT('Ctrl Pts',(4.85068776978043,20.0454806762658,-8.4016376689476));
#20375=CARTESIAN_POINT('Ctrl Pts',(-1.51301029103127E-11,20.2204806762658,
-8.40163766893887));
#20376=CARTESIAN_POINT('Ctrl Pts',(-4.85068776981069,20.3954806762658,-8.40163766893014));
#20377=CARTESIAN_POINT('Ctrl Pts',(-7.2760316547009,20.5704806762658,-4.20081883445633));
#20378=CARTESIAN_POINT('Ctrl Pts',(-9.70137553959111,20.7454806762658,1.74701439383464E-11));
#20379=CARTESIAN_POINT('Ctrl Pts',(-7.27603165468577,20.9204806762658,4.20081883448254));
#20380=CARTESIAN_POINT('Ctrl Pts',(-4.85068776978043,21.0954806762658,8.40163766894761));
#20381=CARTESIAN_POINT('Ctrl Pts',(1.51290740064448E-11,21.2704806762658,
8.40163766893887));
#20382=CARTESIAN_POINT('Ctrl Pts',(4.85068776981068,21.4454806762658,8.40163766893014));
#20383=CARTESIAN_POINT('Ctrl Pts',(7.2760316547009,21.6204806762658,4.20081883445634));
#20384=CARTESIAN_POINT('Ctrl Pts',(9.70137553959111,21.7954806762658,-1.74689558624962E-11));
#20385=CARTESIAN_POINT('Ctrl Pts',(7.27603165468577,21.9704806762658,-4.20081883448253));
#20386=CARTESIAN_POINT('Ctrl Pts',(4.85068776978043,22.1454806762658,-8.4016376689476));
#20387=CARTESIAN_POINT('Ctrl Pts',(-1.51301029103127E-11,22.3204806762658,
-8.40163766893887));
#20388=CARTESIAN_POINT('Ctrl Pts',(-4.85068776981069,22.4954806762658,-8.40163766893014));
#20389=CARTESIAN_POINT('Ctrl Pts',(-7.2760316547009,22.6704806762658,-4.20081883445633));
#20390=CARTESIAN_POINT('Ctrl Pts',(-9.70137553959111,22.8454806762658,1.74701439383464E-11));
#20391=CARTESIAN_POINT('Ctrl Pts',(-7.27603165468577,23.0204806762658,4.20081883448254));
#20392=CARTESIAN_POINT('Ctrl Pts',(-4.85068776978043,23.1954806762658,8.40163766894761));
#20393=CARTESIAN_POINT('Ctrl Pts',(1.51290740064448E-11,23.3704806762658,
8.40163766893887));
#20394=CARTESIAN_POINT('Ctrl Pts',(4.85068776981068,23.5454806762658,8.40163766893014));
#20395=CARTESIAN_POINT('Ctrl Pts',(7.2760316547009,23.7204806762658,4.20081883445634));
#20396=CARTESIAN_POINT('Ctrl Pts',(9.70137553959111,23.8954806762658,-1.74689558624962E-11));
#20397=CARTESIAN_POINT('Ctrl Pts',(7.27603165468577,24.0704806762658,-4.20081883448253));
#20398=CARTESIAN_POINT('Ctrl Pts',(4.85068776978043,24.2454806762658,-8.4016376689476));
#20399=CARTESIAN_POINT('Ctrl Pts',(-1.51301029103127E-11,24.4204806762658,
-8.40163766893887));
#20400=CARTESIAN_POINT('Ctrl Pts',(-4.85068776981069,24.5954806762658,-8.40163766893014));
#20401=CARTESIAN_POINT('Ctrl Pts',(-7.2760316547009,24.7704806762658,-4.20081883445633));
#20402=CARTESIAN_POINT('Ctrl Pts',(-9.70137553959111,24.9454806762658,1.74701439383464E-11));
#20403=CARTESIAN_POINT('Ctrl Pts',(-7.27603165468577,25.1204806762658,4.20081883448254));
#20404=CARTESIAN_POINT('Ctrl Pts',(-4.85068776978043,25.2954806762658,8.40163766894761));
#20405=CARTESIAN_POINT('Ctrl Pts',(1.51290740064448E-11,25.4704806762658,
8.40163766893887));
#20406=CARTESIAN_POINT('Ctrl Pts',(4.85068776981068,25.6454806762658,8.40163766893014));
#20407=CARTESIAN_POINT('Ctrl Pts',(7.2760316547009,25.8204806762658,4.20081883445634));
#20408=CARTESIAN_POINT('Ctrl Pts',(9.70137553959111,25.9954806762658,-1.74689558624962E-11));
#20409=CARTESIAN_POINT('Ctrl Pts',(7.27603165468577,26.1704806762658,-4.20081883448253));
#20410=CARTESIAN_POINT('Ctrl Pts',(4.85068776978043,26.3454806762658,-8.4016376689476));
#20411=CARTESIAN_POINT('Ctrl Pts',(-1.51301029103127E-11,26.5204806762658,
-8.40163766893887));
#20412=CARTESIAN_POINT('Ctrl Pts',(-1.78726082715848E-11,-142.78675111262,
-9.92453123331945));
#20413=CARTESIAN_POINT('Ctrl Pts',(-5.7299307791557,-142.61175111262,-9.92453123330913));
#20414=CARTESIAN_POINT('Ctrl Pts',(-8.59489616871569,-142.43675111262,-4.96226561664425));
#20415=CARTESIAN_POINT('Ctrl Pts',(-11.4598615582757,-142.26175111262,2.06368086793017E-11));
#20416=CARTESIAN_POINT('Ctrl Pts',(-8.59489616869782,-142.08675111262,4.9622656166752));
#20417=CARTESIAN_POINT('Ctrl Pts',(-5.72993077911996,-141.91175111262,9.92453123332977));
#20418=CARTESIAN_POINT('Ctrl Pts',(1.7871392867044E-11,-141.73675111262,
9.92453123331945));
#20419=CARTESIAN_POINT('Ctrl Pts',(5.7299307791557,-141.56175111262,9.92453123330913));
#20420=CARTESIAN_POINT('Ctrl Pts',(8.59489616871569,-141.38675111262,4.96226561664425));
#20421=CARTESIAN_POINT('Ctrl Pts',(11.4598615582757,-141.21175111262,-2.06354052510241E-11));
#20422=CARTESIAN_POINT('Ctrl Pts',(8.59489616869782,-141.03675111262,-4.9622656166752));
#20423=CARTESIAN_POINT('Ctrl Pts',(5.72993077911996,-140.86175111262,-9.92453123332976));
#20424=CARTESIAN_POINT('Ctrl Pts',(-1.78726082715848E-11,-140.68675111262,
-9.92453123331945));
#20425=CARTESIAN_POINT('Ctrl Pts',(-5.7299307791557,-140.51175111262,-9.92453123330913));
#20426=CARTESIAN_POINT('Ctrl Pts',(-8.59489616871569,-140.33675111262,-4.96226561664425));
#20427=CARTESIAN_POINT('Ctrl Pts',(-11.4598615582757,-140.16175111262,2.06368086793017E-11));
#20428=CARTESIAN_POINT('Ctrl Pts',(-8.59489616869782,-139.98675111262,4.9622656166752));
#20429=CARTESIAN_POINT('Ctrl Pts',(-5.72993077911996,-139.81175111262,9.92453123332977));
#20430=CARTESIAN_POINT('Ctrl Pts',(1.7871392867044E-11,-139.63675111262,
9.92453123331945));
#20431=CARTESIAN_POINT('Ctrl Pts',(5.7299307791557,-139.46175111262,9.92453123330913));
#20432=CARTESIAN_POINT('Ctrl Pts',(8.59489616871569,-139.28675111262,4.96226561664425));
#20433=CARTESIAN_POINT('Ctrl Pts',(11.4598615582757,-139.11175111262,-2.06354052510241E-11));
#20434=CARTESIAN_POINT('Ctrl Pts',(8.59489616869782,-138.93675111262,-4.9622656166752));
#20435=CARTESIAN_POINT('Ctrl Pts',(5.72993077911996,-138.76175111262,-9.92453123332976));
#20436=CARTESIAN_POINT('Ctrl Pts',(-1.78726082715848E-11,-138.58675111262,
-9.92453123331945));
#20437=CARTESIAN_POINT('Ctrl Pts',(-5.7299307791557,-138.41175111262,-9.92453123330913));
#20438=CARTESIAN_POINT('Ctrl Pts',(-8.59489616871569,-138.23675111262,-4.96226561664425));
#20439=CARTESIAN_POINT('Ctrl Pts',(-11.4598615582757,-138.06175111262,2.06368086793017E-11));
#20440=CARTESIAN_POINT('Ctrl Pts',(-8.59489616869782,-137.88675111262,4.9622656166752));
#20441=CARTESIAN_POINT('Ctrl Pts',(-5.72993077911996,-137.71175111262,9.92453123332977));
#20442=CARTESIAN_POINT('Ctrl Pts',(1.7871392867044E-11,-137.53675111262,
9.92453123331945));
#20443=CARTESIAN_POINT('Ctrl Pts',(5.7299307791557,-137.36175111262,9.92453123330913));
#20444=CARTESIAN_POINT('Ctrl Pts',(8.59489616871569,-137.18675111262,4.96226561664425));
#20445=CARTESIAN_POINT('Ctrl Pts',(11.4598615582757,-137.01175111262,-2.06354052510241E-11));
#20446=CARTESIAN_POINT('Ctrl Pts',(8.59489616869782,-136.83675111262,-4.9622656166752));
#20447=CARTESIAN_POINT('Ctrl Pts',(5.72993077911996,-136.66175111262,-9.92453123332976));
#20448=CARTESIAN_POINT('Ctrl Pts',(-1.78726082715848E-11,-136.48675111262,
-9.92453123331945));
#20449=CARTESIAN_POINT('Ctrl Pts',(-5.7299307791557,-136.31175111262,-9.92453123330913));
#20450=CARTESIAN_POINT('Ctrl Pts',(-8.59489616871569,-136.13675111262,-4.96226561664425));
#20451=CARTESIAN_POINT('Ctrl Pts',(-11.4598615582757,-135.96175111262,2.06368086793017E-11));
#20452=CARTESIAN_POINT('Ctrl Pts',(-8.59489616869782,-135.78675111262,4.9622656166752));
#20453=CARTESIAN_POINT('Ctrl Pts',(-5.72993077911996,-135.61175111262,9.92453123332977));
#20454=CARTESIAN_POINT('Ctrl Pts',(1.7871392867044E-11,-135.43675111262,
9.92453123331945));
#20455=CARTESIAN_POINT('Ctrl Pts',(5.7299307791557,-135.26175111262,9.92453123330913));
#20456=CARTESIAN_POINT('Ctrl Pts',(8.59489616871569,-135.08675111262,4.96226561664425));
#20457=CARTESIAN_POINT('Ctrl Pts',(11.4598615582757,-134.91175111262,-2.06354052510241E-11));
#20458=CARTESIAN_POINT('Ctrl Pts',(8.59489616869782,-134.73675111262,-4.9622656166752));
#20459=CARTESIAN_POINT('Ctrl Pts',(5.72993077911996,-134.56175111262,-9.92453123332976));
#20460=CARTESIAN_POINT('Ctrl Pts',(-1.78726082715848E-11,-134.38675111262,
-9.92453123331945));
#20461=CARTESIAN_POINT('Ctrl Pts',(-5.7299307791557,-134.21175111262,-9.92453123330913));
#20462=CARTESIAN_POINT('Ctrl Pts',(-8.59489616871569,-134.03675111262,-4.96226561664425));
#20463=CARTESIAN_POINT('Ctrl Pts',(-11.4598615582757,-133.86175111262,2.06368086793017E-11));
#20464=CARTESIAN_POINT('Ctrl Pts',(-8.59489616869782,-133.68675111262,4.9622656166752));
#20465=CARTESIAN_POINT('Ctrl Pts',(-5.72993077911996,-133.51175111262,9.92453123332977));
#20466=CARTESIAN_POINT('Ctrl Pts',(1.7871392867044E-11,-133.33675111262,
9.92453123331945));
#20467=CARTESIAN_POINT('Ctrl Pts',(5.7299307791557,-133.16175111262,9.92453123330913));
#20468=CARTESIAN_POINT('Ctrl Pts',(8.59489616871569,-132.98675111262,4.96226561664425));
#20469=CARTESIAN_POINT('Ctrl Pts',(11.4598615582757,-132.81175111262,-2.06354052510241E-11));
#20470=CARTESIAN_POINT('Ctrl Pts',(8.59489616869782,-132.63675111262,-4.9622656166752));
#20471=CARTESIAN_POINT('Ctrl Pts',(5.72993077911996,-132.46175111262,-9.92453123332976));
#20472=CARTESIAN_POINT('Ctrl Pts',(-1.78726082715848E-11,-132.28675111262,
-9.92453123331945));
#20473=CARTESIAN_POINT('Ctrl Pts',(-5.7299307791557,-132.11175111262,-9.92453123330913));
#20474=CARTESIAN_POINT('Ctrl Pts',(-8.59489616871569,-131.93675111262,-4.96226561664425));
#20475=CARTESIAN_POINT('Ctrl Pts',(-11.4598615582757,-131.76175111262,2.06368086793017E-11));
#20476=CARTESIAN_POINT('Ctrl Pts',(-8.59489616869782,-131.58675111262,4.9622656166752));
#20477=CARTESIAN_POINT('Ctrl Pts',(-5.72993077911996,-131.41175111262,9.92453123332977));
#20478=CARTESIAN_POINT('Ctrl Pts',(1.7871392867044E-11,-131.23675111262,
9.92453123331945));
#20479=CARTESIAN_POINT('Ctrl Pts',(5.7299307791557,-131.06175111262,9.92453123330913));
#20480=CARTESIAN_POINT('Ctrl Pts',(8.59489616871569,-130.88675111262,4.96226561664425));
#20481=CARTESIAN_POINT('Ctrl Pts',(11.4598615582757,-130.71175111262,-2.06354052510241E-11));
#20482=CARTESIAN_POINT('Ctrl Pts',(8.59489616869782,-130.53675111262,-4.9622656166752));
#20483=CARTESIAN_POINT('Ctrl Pts',(5.72993077911996,-130.36175111262,-9.92453123332976));
#20484=CARTESIAN_POINT('Ctrl Pts',(-1.78726082715848E-11,-130.18675111262,
-9.92453123331945));
#20485=CARTESIAN_POINT('Ctrl Pts',(-5.7299307791557,-130.01175111262,-9.92453123330913));
#20486=CARTESIAN_POINT('Ctrl Pts',(-8.59489616871569,-129.83675111262,-4.96226561664425));
#20487=CARTESIAN_POINT('Ctrl Pts',(-11.4598615582757,-129.66175111262,2.06368086793017E-11));
#20488=CARTESIAN_POINT('Ctrl Pts',(-8.59489616869782,-129.48675111262,4.9622656166752));
#20489=CARTESIAN_POINT('Ctrl Pts',(-5.72993077911996,-129.31175111262,9.92453123332977));
#20490=CARTESIAN_POINT('Ctrl Pts',(1.7871392867044E-11,-129.13675111262,
9.92453123331945));
#20491=CARTESIAN_POINT('Ctrl Pts',(5.7299307791557,-128.96175111262,9.92453123330913));
#20492=CARTESIAN_POINT('Ctrl Pts',(8.59489616871569,-128.78675111262,4.96226561664425));
#20493=CARTESIAN_POINT('Ctrl Pts',(11.4598615582757,-128.61175111262,-2.06354052510241E-11));
#20494=CARTESIAN_POINT('Ctrl Pts',(8.59489616869782,-128.43675111262,-4.9622656166752));
#20495=CARTESIAN_POINT('Ctrl Pts',(5.72993077911996,-128.26175111262,-9.92453123332976));
#20496=CARTESIAN_POINT('Ctrl Pts',(-1.78726082715848E-11,-128.08675111262,
-9.92453123331945));
#20497=CARTESIAN_POINT('Ctrl Pts',(-5.7299307791557,-127.91175111262,-9.92453123330913));
#20498=CARTESIAN_POINT('Ctrl Pts',(-8.59489616871569,-127.73675111262,-4.96226561664425));
#20499=CARTESIAN_POINT('Ctrl Pts',(-11.4598615582757,-127.56175111262,2.06368086793017E-11));
#20500=CARTESIAN_POINT('Ctrl Pts',(-8.59489616869782,-127.38675111262,4.9622656166752));
#20501=CARTESIAN_POINT('Ctrl Pts',(-5.72993077911996,-127.21175111262,9.92453123332977));
#20502=CARTESIAN_POINT('Ctrl Pts',(1.7871392867044E-11,-127.03675111262,
9.92453123331945));
#20503=CARTESIAN_POINT('Ctrl Pts',(5.7299307791557,-126.86175111262,9.92453123330913));
#20504=CARTESIAN_POINT('Ctrl Pts',(8.59489616871569,-126.68675111262,4.96226561664425));
#20505=CARTESIAN_POINT('Ctrl Pts',(11.4598615582757,-126.51175111262,-2.06354052510241E-11));
#20506=CARTESIAN_POINT('Ctrl Pts',(8.59489616869782,-126.33675111262,-4.9622656166752));
#20507=CARTESIAN_POINT('Ctrl Pts',(5.72993077911996,-126.16175111262,-9.92453123332976));
#20508=CARTESIAN_POINT('Ctrl Pts',(-1.78726082715848E-11,-125.98675111262,
-9.92453123331945));
#20509=CARTESIAN_POINT('Ctrl Pts',(-5.7299307791557,-125.81175111262,-9.92453123330913));
#20510=CARTESIAN_POINT('Ctrl Pts',(-8.59489616871569,-125.63675111262,-4.96226561664425));
#20511=CARTESIAN_POINT('Ctrl Pts',(-11.4598615582757,-125.46175111262,2.06368086793017E-11));
#20512=CARTESIAN_POINT('Ctrl Pts',(-8.59489616869782,-125.28675111262,4.9622656166752));
#20513=CARTESIAN_POINT('Ctrl Pts',(-5.72993077911996,-125.11175111262,9.92453123332977));
#20514=CARTESIAN_POINT('Ctrl Pts',(1.7871392867044E-11,-124.93675111262,
9.92453123331945));
#20515=CARTESIAN_POINT('Ctrl Pts',(5.7299307791557,-124.76175111262,9.92453123330913));
#20516=CARTESIAN_POINT('Ctrl Pts',(8.59489616871569,-124.58675111262,4.96226561664425));
#20517=CARTESIAN_POINT('Ctrl Pts',(11.4598615582757,-124.41175111262,-2.06354052510241E-11));
#20518=CARTESIAN_POINT('Ctrl Pts',(8.59489616869782,-124.23675111262,-4.9622656166752));
#20519=CARTESIAN_POINT('Ctrl Pts',(5.72993077911996,-124.06175111262,-9.92453123332976));
#20520=CARTESIAN_POINT('Ctrl Pts',(-1.78726082715848E-11,-123.88675111262,
-9.92453123331945));
#20521=CARTESIAN_POINT('Ctrl Pts',(-5.7299307791557,-123.71175111262,-9.92453123330913));
#20522=CARTESIAN_POINT('Ctrl Pts',(-8.59489616871569,-123.53675111262,-4.96226561664425));
#20523=CARTESIAN_POINT('Ctrl Pts',(-11.4598615582757,-123.36175111262,2.06368086793017E-11));
#20524=CARTESIAN_POINT('Ctrl Pts',(-8.59489616869782,-123.18675111262,4.9622656166752));
#20525=CARTESIAN_POINT('Ctrl Pts',(-5.72993077911996,-123.01175111262,9.92453123332977));
#20526=CARTESIAN_POINT('Ctrl Pts',(1.7871392867044E-11,-122.83675111262,
9.92453123331945));
#20527=CARTESIAN_POINT('Ctrl Pts',(5.7299307791557,-122.66175111262,9.92453123330913));
#20528=CARTESIAN_POINT('Ctrl Pts',(8.59489616871569,-122.48675111262,4.96226561664425));
#20529=CARTESIAN_POINT('Ctrl Pts',(11.4598615582757,-122.31175111262,-2.06354052510241E-11));
#20530=CARTESIAN_POINT('Ctrl Pts',(8.59489616869782,-122.13675111262,-4.9622656166752));
#20531=CARTESIAN_POINT('Ctrl Pts',(5.72993077911996,-121.96175111262,-9.92453123332976));
#20532=CARTESIAN_POINT('Ctrl Pts',(-1.78726082715848E-11,-121.78675111262,
-9.92453123331945));
#20533=CARTESIAN_POINT('Ctrl Pts',(-5.7299307791557,-121.61175111262,-9.92453123330913));
#20534=CARTESIAN_POINT('Ctrl Pts',(-8.59489616871569,-121.43675111262,-4.96226561664425));
#20535=CARTESIAN_POINT('Ctrl Pts',(-11.4598615582757,-121.26175111262,2.06368086793017E-11));
#20536=CARTESIAN_POINT('Ctrl Pts',(-8.59489616869782,-121.08675111262,4.9622656166752));
#20537=CARTESIAN_POINT('Ctrl Pts',(-5.72993077911996,-120.91175111262,9.92453123332977));
#20538=CARTESIAN_POINT('Ctrl Pts',(1.7871392867044E-11,-120.73675111262,
9.92453123331945));
#20539=CARTESIAN_POINT('Ctrl Pts',(5.7299307791557,-120.56175111262,9.92453123330913));
#20540=CARTESIAN_POINT('Ctrl Pts',(8.59489616871569,-120.38675111262,4.96226561664425));
#20541=CARTESIAN_POINT('Ctrl Pts',(11.4598615582757,-120.21175111262,-2.06354052510241E-11));
#20542=CARTESIAN_POINT('Ctrl Pts',(8.59489616869782,-120.03675111262,-4.9622656166752));
#20543=CARTESIAN_POINT('Ctrl Pts',(5.72993077911996,-119.86175111262,-9.92453123332976));
#20544=CARTESIAN_POINT('Ctrl Pts',(-1.78726082715848E-11,-119.68675111262,
-9.92453123331945));
#20545=CARTESIAN_POINT('Ctrl Pts',(-5.7299307791557,-119.51175111262,-9.92453123330913));
#20546=CARTESIAN_POINT('Ctrl Pts',(-8.59489616871569,-119.33675111262,-4.96226561664425));
#20547=CARTESIAN_POINT('Ctrl Pts',(-11.4598615582757,-119.16175111262,2.06368086793017E-11));
#20548=CARTESIAN_POINT('Ctrl Pts',(-8.59489616869782,-118.98675111262,4.9622656166752));
#20549=CARTESIAN_POINT('Ctrl Pts',(-5.72993077911996,-118.81175111262,9.92453123332977));
#20550=CARTESIAN_POINT('Ctrl Pts',(1.7871392867044E-11,-118.63675111262,
9.92453123331945));
#20551=CARTESIAN_POINT('Ctrl Pts',(5.7299307791557,-118.46175111262,9.92453123330913));
#20552=CARTESIAN_POINT('Ctrl Pts',(8.59489616871569,-118.28675111262,4.96226561664425));
#20553=CARTESIAN_POINT('Ctrl Pts',(11.4598615582757,-118.11175111262,-2.06354052510241E-11));
#20554=CARTESIAN_POINT('Ctrl Pts',(8.59489616869782,-117.93675111262,-4.9622656166752));
#20555=CARTESIAN_POINT('Ctrl Pts',(5.72993077911996,-117.76175111262,-9.92453123332976));
#20556=CARTESIAN_POINT('Ctrl Pts',(-1.78726082715848E-11,-117.58675111262,
-9.92453123331945));
#20557=CARTESIAN_POINT('Ctrl Pts',(-5.7299307791557,-117.41175111262,-9.92453123330913));
#20558=CARTESIAN_POINT('Ctrl Pts',(-8.59489616871569,-117.23675111262,-4.96226561664425));
#20559=CARTESIAN_POINT('Ctrl Pts',(-11.4598615582757,-117.06175111262,2.06368086793017E-11));
#20560=CARTESIAN_POINT('Ctrl Pts',(-8.59489616869782,-116.88675111262,4.9622656166752));
#20561=CARTESIAN_POINT('Ctrl Pts',(-5.72993077911996,-116.71175111262,9.92453123332977));
#20562=CARTESIAN_POINT('Ctrl Pts',(1.7871392867044E-11,-116.53675111262,
9.92453123331945));
#20563=CARTESIAN_POINT('Ctrl Pts',(5.7299307791557,-116.36175111262,9.92453123330913));
#20564=CARTESIAN_POINT('Ctrl Pts',(8.59489616871569,-116.18675111262,4.96226561664425));
#20565=CARTESIAN_POINT('Ctrl Pts',(11.4598615582757,-116.01175111262,-2.06354052510241E-11));
#20566=CARTESIAN_POINT('Ctrl Pts',(8.59489616869782,-115.83675111262,-4.9622656166752));
#20567=CARTESIAN_POINT('Ctrl Pts',(5.72993077911996,-115.66175111262,-9.92453123332976));
#20568=CARTESIAN_POINT('Ctrl Pts',(-1.78726082715848E-11,-115.48675111262,
-9.92453123331945));
#20569=CARTESIAN_POINT('Ctrl Pts',(-5.7299307791557,-115.31175111262,-9.92453123330913));
#20570=CARTESIAN_POINT('Ctrl Pts',(-8.59489616871569,-115.13675111262,-4.96226561664425));
#20571=CARTESIAN_POINT('Ctrl Pts',(-11.4598615582757,-114.96175111262,2.06368086793017E-11));
#20572=CARTESIAN_POINT('Ctrl Pts',(-8.59489616869782,-114.78675111262,4.9622656166752));
#20573=CARTESIAN_POINT('Ctrl Pts',(-5.72993077911996,-114.61175111262,9.92453123332977));
#20574=CARTESIAN_POINT('Ctrl Pts',(1.7871392867044E-11,-114.43675111262,
9.92453123331945));
#20575=CARTESIAN_POINT('Ctrl Pts',(5.7299307791557,-114.26175111262,9.92453123330913));
#20576=CARTESIAN_POINT('Ctrl Pts',(8.59489616871569,-114.08675111262,4.96226561664425));
#20577=CARTESIAN_POINT('Ctrl Pts',(11.4598615582757,-113.91175111262,-2.06354052510241E-11));
#20578=CARTESIAN_POINT('Ctrl Pts',(8.59489616869782,-113.73675111262,-4.9622656166752));
#20579=CARTESIAN_POINT('Ctrl Pts',(5.72993077911996,-113.56175111262,-9.92453123332976));
#20580=CARTESIAN_POINT('Ctrl Pts',(-1.78726082715848E-11,-113.38675111262,
-9.92453123331945));
#20581=CARTESIAN_POINT('Ctrl Pts',(-5.7299307791557,-113.21175111262,-9.92453123330913));
#20582=CARTESIAN_POINT('Ctrl Pts',(-8.59489616871569,-113.03675111262,-4.96226561664425));
#20583=CARTESIAN_POINT('Ctrl Pts',(-11.4598615582757,-112.86175111262,2.06368086793017E-11));
#20584=CARTESIAN_POINT('Ctrl Pts',(-8.59489616869782,-112.68675111262,4.9622656166752));
#20585=CARTESIAN_POINT('Ctrl Pts',(-5.72993077911996,-112.51175111262,9.92453123332977));
#20586=CARTESIAN_POINT('Ctrl Pts',(1.7871392867044E-11,-112.33675111262,
9.92453123331945));
#20587=CARTESIAN_POINT('Ctrl Pts',(5.7299307791557,-112.16175111262,9.92453123330913));
#20588=CARTESIAN_POINT('Ctrl Pts',(8.59489616871569,-111.98675111262,4.96226561664425));
#20589=CARTESIAN_POINT('Ctrl Pts',(11.4598615582757,-111.81175111262,-2.06354052510241E-11));
#20590=CARTESIAN_POINT('Ctrl Pts',(8.59489616869782,-111.63675111262,-4.9622656166752));
#20591=CARTESIAN_POINT('Ctrl Pts',(5.72993077911996,-111.46175111262,-9.92453123332976));
#20592=CARTESIAN_POINT('Ctrl Pts',(-1.78726082715848E-11,-111.28675111262,
-9.92453123331945));
#20593=CARTESIAN_POINT('Ctrl Pts',(-5.7299307791557,-111.11175111262,-9.92453123330913));
#20594=CARTESIAN_POINT('Ctrl Pts',(-8.59489616871569,-110.93675111262,-4.96226561664425));
#20595=CARTESIAN_POINT('Ctrl Pts',(-11.4598615582757,-110.76175111262,2.06368086793017E-11));
#20596=CARTESIAN_POINT('Ctrl Pts',(-8.59489616869782,-110.58675111262,4.9622656166752));
#20597=CARTESIAN_POINT('Ctrl Pts',(-5.72993077911996,-110.41175111262,9.92453123332977));
#20598=CARTESIAN_POINT('Ctrl Pts',(1.7871392867044E-11,-110.23675111262,
9.92453123331945));
#20599=CARTESIAN_POINT('Ctrl Pts',(5.7299307791557,-110.06175111262,9.92453123330913));
#20600=CARTESIAN_POINT('Ctrl Pts',(8.59489616871569,-109.88675111262,4.96226561664425));
#20601=CARTESIAN_POINT('Ctrl Pts',(11.4598615582757,-109.71175111262,-2.06354052510241E-11));
#20602=CARTESIAN_POINT('Ctrl Pts',(8.59489616869782,-109.53675111262,-4.9622656166752));
#20603=CARTESIAN_POINT('Ctrl Pts',(5.72993077911996,-109.36175111262,-9.92453123332976));
#20604=CARTESIAN_POINT('Ctrl Pts',(-1.78726082715848E-11,-109.18675111262,
-9.92453123331945));
#20605=CARTESIAN_POINT('Ctrl Pts',(-5.7299307791557,-109.01175111262,-9.92453123330913));
#20606=CARTESIAN_POINT('Ctrl Pts',(-8.59489616871569,-108.83675111262,-4.96226561664425));
#20607=CARTESIAN_POINT('Ctrl Pts',(-11.4598615582757,-108.66175111262,2.06368086793017E-11));
#20608=CARTESIAN_POINT('Ctrl Pts',(-8.59489616869782,-108.48675111262,4.9622656166752));
#20609=CARTESIAN_POINT('Ctrl Pts',(-5.72993077911996,-108.31175111262,9.92453123332977));
#20610=CARTESIAN_POINT('Ctrl Pts',(1.7871392867044E-11,-108.13675111262,
9.92453123331945));
#20611=CARTESIAN_POINT('Ctrl Pts',(5.7299307791557,-107.96175111262,9.92453123330913));
#20612=CARTESIAN_POINT('Ctrl Pts',(8.59489616871569,-107.78675111262,4.96226561664425));
#20613=CARTESIAN_POINT('Ctrl Pts',(11.4598615582757,-107.61175111262,-2.06354052510241E-11));
#20614=CARTESIAN_POINT('Ctrl Pts',(8.59489616869782,-107.43675111262,-4.9622656166752));
#20615=CARTESIAN_POINT('Ctrl Pts',(5.72993077911996,-107.26175111262,-9.92453123332976));
#20616=CARTESIAN_POINT('Ctrl Pts',(-1.78726082715848E-11,-107.08675111262,
-9.92453123331945));
#20617=CARTESIAN_POINT('Ctrl Pts',(-5.7299307791557,-106.91175111262,-9.92453123330913));
#20618=CARTESIAN_POINT('Ctrl Pts',(-8.59489616871569,-106.73675111262,-4.96226561664425));
#20619=CARTESIAN_POINT('Ctrl Pts',(-11.4598615582757,-106.56175111262,2.06368086793017E-11));
#20620=CARTESIAN_POINT('Ctrl Pts',(-8.59489616869782,-106.38675111262,4.9622656166752));
#20621=CARTESIAN_POINT('Ctrl Pts',(-5.72993077911996,-106.21175111262,9.92453123332977));
#20622=CARTESIAN_POINT('Ctrl Pts',(1.7871392867044E-11,-106.03675111262,
9.92453123331945));
#20623=CARTESIAN_POINT('Ctrl Pts',(5.7299307791557,-105.86175111262,9.92453123330913));
#20624=CARTESIAN_POINT('Ctrl Pts',(8.59489616871569,-105.68675111262,4.96226561664425));
#20625=CARTESIAN_POINT('Ctrl Pts',(11.4598615582757,-105.51175111262,-2.06354052510241E-11));
#20626=CARTESIAN_POINT('Ctrl Pts',(8.59489616869782,-105.33675111262,-4.9622656166752));
#20627=CARTESIAN_POINT('Ctrl Pts',(5.72993077911996,-105.16175111262,-9.92453123332976));
#20628=CARTESIAN_POINT('Ctrl Pts',(-1.78726082715848E-11,-104.98675111262,
-9.92453123331945));
#20629=CARTESIAN_POINT('Ctrl Pts',(-5.7299307791557,-104.81175111262,-9.92453123330913));
#20630=CARTESIAN_POINT('Ctrl Pts',(-8.59489616871569,-104.63675111262,-4.96226561664425));
#20631=CARTESIAN_POINT('Ctrl Pts',(-11.4598615582757,-104.46175111262,2.06368086793017E-11));
#20632=CARTESIAN_POINT('Ctrl Pts',(-8.59489616869782,-104.28675111262,4.9622656166752));
#20633=CARTESIAN_POINT('Ctrl Pts',(-5.72993077911996,-104.11175111262,9.92453123332977));
#20634=CARTESIAN_POINT('Ctrl Pts',(1.7871392867044E-11,-103.93675111262,
9.92453123331945));
#20635=CARTESIAN_POINT('Ctrl Pts',(5.7299307791557,-103.76175111262,9.92453123330913));
#20636=CARTESIAN_POINT('Ctrl Pts',(8.59489616871569,-103.58675111262,4.96226561664425));
#20637=CARTESIAN_POINT('Ctrl Pts',(11.4598615582757,-103.41175111262,-2.06354052510241E-11));
#20638=CARTESIAN_POINT('Ctrl Pts',(8.59489616869782,-103.23675111262,-4.9622656166752));
#20639=CARTESIAN_POINT('Ctrl Pts',(5.72993077911996,-103.06175111262,-9.92453123332976));
#20640=CARTESIAN_POINT('Ctrl Pts',(-1.78726082715848E-11,-102.88675111262,
-9.92453123331945));
#20641=CARTESIAN_POINT('Ctrl Pts',(-5.7299307791557,-102.71175111262,-9.92453123330913));
#20642=CARTESIAN_POINT('Ctrl Pts',(-8.59489616871569,-102.53675111262,-4.96226561664425));
#20643=CARTESIAN_POINT('Ctrl Pts',(-11.4598615582757,-102.36175111262,2.06368086793017E-11));
#20644=CARTESIAN_POINT('Ctrl Pts',(-8.59489616869782,-102.18675111262,4.9622656166752));
#20645=CARTESIAN_POINT('Ctrl Pts',(-5.72993077911996,-102.01175111262,9.92453123332977));
#20646=CARTESIAN_POINT('Ctrl Pts',(1.7871392867044E-11,-101.83675111262,
9.92453123331945));
#20647=CARTESIAN_POINT('Ctrl Pts',(5.7299307791557,-101.66175111262,9.92453123330913));
#20648=CARTESIAN_POINT('Ctrl Pts',(8.59489616871569,-101.48675111262,4.96226561664425));
#20649=CARTESIAN_POINT('Ctrl Pts',(11.4598615582757,-101.31175111262,-2.06354052510241E-11));
#20650=CARTESIAN_POINT('Ctrl Pts',(8.59489616869782,-101.13675111262,-4.9622656166752));
#20651=CARTESIAN_POINT('Ctrl Pts',(5.72993077911996,-100.96175111262,-9.92453123332976));
#20652=CARTESIAN_POINT('Ctrl Pts',(-1.78726082715848E-11,-100.78675111262,
-9.92453123331945));
#20653=CARTESIAN_POINT('Ctrl Pts',(-5.7299307791557,-100.61175111262,-9.92453123330913));
#20654=CARTESIAN_POINT('Ctrl Pts',(-8.59489616871569,-100.43675111262,-4.96226561664425));
#20655=CARTESIAN_POINT('Ctrl Pts',(-11.4598615582757,-100.26175111262,2.06368086793017E-11));
#20656=CARTESIAN_POINT('Ctrl Pts',(-8.59489616869782,-100.08675111262,4.9622656166752));
#20657=CARTESIAN_POINT('Ctrl Pts',(-5.72993077911996,-99.91175111262,9.92453123332977));
#20658=CARTESIAN_POINT('Ctrl Pts',(1.7871392867044E-11,-99.7367511126201,
9.92453123331945));
#20659=CARTESIAN_POINT('Ctrl Pts',(5.7299307791557,-99.5617511126201,9.92453123330913));
#20660=CARTESIAN_POINT('Ctrl Pts',(8.59489616871569,-99.3867511126201,4.96226561664425));
#20661=CARTESIAN_POINT('Ctrl Pts',(11.4598615582757,-99.2117511126201,-2.06354052510241E-11));
#20662=CARTESIAN_POINT('Ctrl Pts',(8.59489616869782,-99.0367511126201,-4.9622656166752));
#20663=CARTESIAN_POINT('Ctrl Pts',(5.72993077911996,-98.8617511126201,-9.92453123332976));
#20664=CARTESIAN_POINT('Ctrl Pts',(-1.78726082715848E-11,-98.6867511126201,
-9.92453123331945));
#20665=CARTESIAN_POINT('Ctrl Pts',(-5.7299307791557,-98.5117511126201,-9.92453123330913));
#20666=CARTESIAN_POINT('Ctrl Pts',(-8.59489616871569,-98.33675111262,-4.96226561664425));
#20667=CARTESIAN_POINT('Ctrl Pts',(-11.4598615582757,-98.16175111262,2.06368086793017E-11));
#20668=CARTESIAN_POINT('Ctrl Pts',(-8.59489616869782,-97.9867511126201,
4.9622656166752));
#20669=CARTESIAN_POINT('Ctrl Pts',(-5.72993077911996,-97.81175111262,9.92453123332977));
#20670=CARTESIAN_POINT('Ctrl Pts',(1.7871392867044E-11,-97.6367511126201,
9.92453123331945));
#20671=CARTESIAN_POINT('Ctrl Pts',(5.7299307791557,-97.46175111262,9.92453123330913));
#20672=CARTESIAN_POINT('Ctrl Pts',(8.59489616871569,-97.2867511126201,4.96226561664425));
#20673=CARTESIAN_POINT('Ctrl Pts',(11.4598615582757,-97.1117511126201,-2.06354052510241E-11));
#20674=CARTESIAN_POINT('Ctrl Pts',(8.59489616869782,-96.9367511126201,-4.9622656166752));
#20675=CARTESIAN_POINT('Ctrl Pts',(5.72993077911996,-96.7617511126201,-9.92453123332976));
#20676=CARTESIAN_POINT('Ctrl Pts',(-1.78726082715848E-11,-96.5867511126201,
-9.92453123331945));
#20677=CARTESIAN_POINT('Ctrl Pts',(-5.7299307791557,-96.4117511126201,-9.92453123330913));
#20678=CARTESIAN_POINT('Ctrl Pts',(-8.59489616871569,-96.2367511126201,
-4.96226561664425));
#20679=CARTESIAN_POINT('Ctrl Pts',(-11.4598615582757,-96.0617511126201,
2.06368086793017E-11));
#20680=CARTESIAN_POINT('Ctrl Pts',(-8.59489616869782,-95.8867511126201,
4.9622656166752));
#20681=CARTESIAN_POINT('Ctrl Pts',(-5.72993077911996,-95.7117511126201,
9.92453123332977));
#20682=CARTESIAN_POINT('Ctrl Pts',(1.7871392867044E-11,-95.5367511126201,
9.92453123331945));
#20683=CARTESIAN_POINT('Ctrl Pts',(5.7299307791557,-95.3617511126201,9.92453123330913));
#20684=CARTESIAN_POINT('Ctrl Pts',(8.59489616871569,-95.1867511126201,4.96226561664425));
#20685=CARTESIAN_POINT('Ctrl Pts',(11.4598615582757,-95.0117511126201,-2.06354052510241E-11));
#20686=CARTESIAN_POINT('Ctrl Pts',(8.59489616869782,-94.8367511126201,-4.9622656166752));
#20687=CARTESIAN_POINT('Ctrl Pts',(5.72993077911996,-94.6617511126201,-9.92453123332976));
#20688=CARTESIAN_POINT('Ctrl Pts',(-1.78726082715848E-11,-94.4867511126201,
-9.92453123331945));
#20689=CARTESIAN_POINT('Ctrl Pts',(-5.7299307791557,-94.3117511126201,-9.92453123330913));
#20690=CARTESIAN_POINT('Ctrl Pts',(-8.59489616871569,-94.1367511126201,
-4.96226561664425));
#20691=CARTESIAN_POINT('Ctrl Pts',(-11.4598615582757,-93.9617511126201,
2.06368086793017E-11));
#20692=CARTESIAN_POINT('Ctrl Pts',(-8.59489616869782,-93.7867511126201,
4.9622656166752));
#20693=CARTESIAN_POINT('Ctrl Pts',(-5.72993077911996,-93.6117511126201,
9.92453123332977));
#20694=CARTESIAN_POINT('Ctrl Pts',(1.7871392867044E-11,-93.4367511126201,
9.92453123331945));
#20695=CARTESIAN_POINT('Ctrl Pts',(5.7299307791557,-93.2617511126201,9.92453123330913));
#20696=CARTESIAN_POINT('Ctrl Pts',(8.59489616871569,-93.0867511126201,4.96226561664425));
#20697=CARTESIAN_POINT('Ctrl Pts',(11.4598615582757,-92.9117511126201,-2.06354052510241E-11));
#20698=CARTESIAN_POINT('Ctrl Pts',(8.59489616869782,-92.7367511126201,-4.9622656166752));
#20699=CARTESIAN_POINT('Ctrl Pts',(5.72993077911996,-92.5617511126201,-9.92453123332976));
#20700=CARTESIAN_POINT('Ctrl Pts',(-1.78726082715848E-11,-92.3867511126201,
-9.92453123331945));
#20701=CARTESIAN_POINT('Ctrl Pts',(-5.7299307791557,-92.2117511126201,-9.92453123330913));
#20702=CARTESIAN_POINT('Ctrl Pts',(-8.59489616871569,-92.0367511126201,
-4.96226561664425));
#20703=CARTESIAN_POINT('Ctrl Pts',(-11.4598615582757,-91.8617511126201,
2.06368086793017E-11));
#20704=CARTESIAN_POINT('Ctrl Pts',(-8.59489616869782,-91.6867511126201,
4.9622656166752));
#20705=CARTESIAN_POINT('Ctrl Pts',(-5.72993077911996,-91.5117511126201,
9.92453123332977));
#20706=CARTESIAN_POINT('Ctrl Pts',(1.7871392867044E-11,-91.3367511126201,
9.92453123331945));
#20707=CARTESIAN_POINT('Ctrl Pts',(5.7299307791557,-91.1617511126201,9.92453123330913));
#20708=CARTESIAN_POINT('Ctrl Pts',(8.59489616871569,-90.9867511126201,4.96226561664425));
#20709=CARTESIAN_POINT('Ctrl Pts',(11.4598615582757,-90.8117511126201,-2.06354052510241E-11));
#20710=CARTESIAN_POINT('Ctrl Pts',(8.59489616869782,-90.6367511126201,-4.9622656166752));
#20711=CARTESIAN_POINT('Ctrl Pts',(5.72993077911996,-90.4617511126201,-9.92453123332976));
#20712=CARTESIAN_POINT('Ctrl Pts',(-1.78726082715848E-11,-90.2867511126201,
-9.92453123331945));
#20713=CARTESIAN_POINT('Ctrl Pts',(-5.7299307791557,-90.1117511126201,-9.92453123330913));
#20714=CARTESIAN_POINT('Ctrl Pts',(-8.59489616871569,-89.9367511126201,
-4.96226561664425));
#20715=CARTESIAN_POINT('Ctrl Pts',(-11.4598615582757,-89.7617511126201,
2.06368086793017E-11));
#20716=CARTESIAN_POINT('Ctrl Pts',(-8.59489616869782,-89.5867511126201,
4.9622656166752));
#20717=CARTESIAN_POINT('Ctrl Pts',(-5.72993077911996,-89.4117511126201,
9.92453123332977));
#20718=CARTESIAN_POINT('Ctrl Pts',(1.7871392867044E-11,-89.2367511126201,
9.92453123331945));
#20719=CARTESIAN_POINT('Ctrl Pts',(5.7299307791557,-89.0617511126201,9.92453123330913));
#20720=CARTESIAN_POINT('Ctrl Pts',(8.59489616871569,-88.8867511126201,4.96226561664425));
#20721=CARTESIAN_POINT('Ctrl Pts',(11.4598615582757,-88.7117511126201,-2.06354052510241E-11));
#20722=CARTESIAN_POINT('Ctrl Pts',(8.59489616869782,-88.5367511126201,-4.9622656166752));
#20723=CARTESIAN_POINT('Ctrl Pts',(5.72993077911996,-88.3617511126201,-9.92453123332976));
#20724=CARTESIAN_POINT('Ctrl Pts',(-1.78726082715848E-11,-88.1867511126201,
-9.92453123331945));
#20725=CARTESIAN_POINT('Ctrl Pts',(-5.7299307791557,-88.0117511126201,-9.92453123330913));
#20726=CARTESIAN_POINT('Ctrl Pts',(-8.59489616871569,-87.8367511126201,
-4.96226561664425));
#20727=CARTESIAN_POINT('Ctrl Pts',(-11.4598615582757,-87.6617511126201,
2.06368086793017E-11));
#20728=CARTESIAN_POINT('Ctrl Pts',(-8.59489616869782,-87.4867511126201,
4.9622656166752));
#20729=CARTESIAN_POINT('Ctrl Pts',(-5.72993077911996,-87.3117511126201,
9.92453123332977));
#20730=CARTESIAN_POINT('Ctrl Pts',(1.7871392867044E-11,-87.1367511126201,
9.92453123331945));
#20731=CARTESIAN_POINT('Ctrl Pts',(5.7299307791557,-86.9617511126201,9.92453123330913));
#20732=CARTESIAN_POINT('Ctrl Pts',(8.59489616871569,-86.7867511126201,4.96226561664425));
#20733=CARTESIAN_POINT('Ctrl Pts',(11.4598615582757,-86.6117511126201,-2.06354052510241E-11));
#20734=CARTESIAN_POINT('Ctrl Pts',(8.59489616869782,-86.4367511126201,-4.9622656166752));
#20735=CARTESIAN_POINT('Ctrl Pts',(5.72993077911996,-86.2617511126201,-9.92453123332976));
#20736=CARTESIAN_POINT('Ctrl Pts',(-1.78726082715848E-11,-86.0867511126201,
-9.92453123331945));
#20737=CARTESIAN_POINT('Ctrl Pts',(-5.7299307791557,-85.9117511126201,-9.92453123330913));
#20738=CARTESIAN_POINT('Ctrl Pts',(-8.59489616871569,-85.7367511126201,
-4.96226561664425));
#20739=CARTESIAN_POINT('Ctrl Pts',(-11.4598615582757,-85.5617511126201,
2.06368086793017E-11));
#20740=CARTESIAN_POINT('Ctrl Pts',(-8.59489616869782,-85.3867511126201,
4.9622656166752));
#20741=CARTESIAN_POINT('Ctrl Pts',(-5.72993077911996,-85.2117511126201,
9.92453123332977));
#20742=CARTESIAN_POINT('Ctrl Pts',(1.7871392867044E-11,-85.0367511126201,
9.92453123331945));
#20743=CARTESIAN_POINT('Ctrl Pts',(5.7299307791557,-84.8617511126201,9.92453123330913));
#20744=CARTESIAN_POINT('Ctrl Pts',(8.59489616871569,-84.6867511126201,4.96226561664425));
#20745=CARTESIAN_POINT('Ctrl Pts',(11.4598615582757,-84.5117511126201,-2.06354052510241E-11));
#20746=CARTESIAN_POINT('Ctrl Pts',(8.59489616869782,-84.3367511126201,-4.9622656166752));
#20747=CARTESIAN_POINT('Ctrl Pts',(5.72993077911996,-84.1617511126201,-9.92453123332976));
#20748=CARTESIAN_POINT('Ctrl Pts',(-1.78726082715848E-11,-83.9867511126201,
-9.92453123331945));
#20749=CARTESIAN_POINT('Ctrl Pts',(-5.7299307791557,-83.8117511126201,-9.92453123330913));
#20750=CARTESIAN_POINT('Ctrl Pts',(-8.59489616871569,-83.6367511126201,
-4.96226561664425));
#20751=CARTESIAN_POINT('Ctrl Pts',(-11.4598615582757,-83.4617511126201,
2.06368086793017E-11));
#20752=CARTESIAN_POINT('Ctrl Pts',(-8.59489616869782,-83.2867511126201,
4.9622656166752));
#20753=CARTESIAN_POINT('Ctrl Pts',(-5.72993077911996,-83.1117511126201,
9.92453123332977));
#20754=CARTESIAN_POINT('Ctrl Pts',(1.7871392867044E-11,-82.9367511126201,
9.92453123331945));
#20755=CARTESIAN_POINT('Ctrl Pts',(5.7299307791557,-82.7617511126201,9.92453123330913));
#20756=CARTESIAN_POINT('Ctrl Pts',(8.59489616871569,-82.5867511126201,4.96226561664425));
#20757=CARTESIAN_POINT('Ctrl Pts',(11.4598615582757,-82.4117511126201,-2.06354052510241E-11));
#20758=CARTESIAN_POINT('Ctrl Pts',(8.59489616869782,-82.2367511126201,-4.9622656166752));
#20759=CARTESIAN_POINT('Ctrl Pts',(5.72993077911996,-82.0617511126201,-9.92453123332976));
#20760=CARTESIAN_POINT('Ctrl Pts',(-1.78726082715848E-11,-81.8867511126201,
-9.92453123331945));
#20761=CARTESIAN_POINT('Ctrl Pts',(-5.7299307791557,-81.7117511126201,-9.92453123330913));
#20762=CARTESIAN_POINT('Ctrl Pts',(-8.59489616871569,-81.5367511126201,
-4.96226561664425));
#20763=CARTESIAN_POINT('Ctrl Pts',(-11.4598615582757,-81.3617511126201,
2.06368086793017E-11));
#20764=CARTESIAN_POINT('Ctrl Pts',(-8.59489616869782,-81.1867511126201,
4.9622656166752));
#20765=CARTESIAN_POINT('Ctrl Pts',(-5.72993077911996,-81.0117511126201,
9.92453123332977));
#20766=CARTESIAN_POINT('Ctrl Pts',(1.7871392867044E-11,-80.8367511126201,
9.92453123331945));
#20767=CARTESIAN_POINT('Ctrl Pts',(5.7299307791557,-80.6617511126201,9.92453123330913));
#20768=CARTESIAN_POINT('Ctrl Pts',(8.59489616871569,-80.4867511126201,4.96226561664425));
#20769=CARTESIAN_POINT('Ctrl Pts',(11.4598615582757,-80.3117511126201,-2.06354052510241E-11));
#20770=CARTESIAN_POINT('Ctrl Pts',(8.59489616869782,-80.1367511126201,-4.9622656166752));
#20771=CARTESIAN_POINT('Ctrl Pts',(5.72993077911996,-79.9617511126201,-9.92453123332976));
#20772=CARTESIAN_POINT('Ctrl Pts',(-1.78726082715848E-11,-79.7867511126201,
-9.92453123331945));
#20773=CARTESIAN_POINT('Ctrl Pts',(-5.7299307791557,-79.6117511126201,-9.92453123330913));
#20774=CARTESIAN_POINT('Ctrl Pts',(-8.59489616871569,-79.4367511126201,
-4.96226561664425));
#20775=CARTESIAN_POINT('Ctrl Pts',(-11.4598615582757,-79.2617511126201,
2.06368086793017E-11));
#20776=CARTESIAN_POINT('Ctrl Pts',(-8.59489616869782,-79.0867511126201,
4.9622656166752));
#20777=CARTESIAN_POINT('Ctrl Pts',(-5.72993077911996,-78.9117511126201,
9.92453123332977));
#20778=CARTESIAN_POINT('Ctrl Pts',(1.7871392867044E-11,-78.7367511126201,
9.92453123331945));
#20779=CARTESIAN_POINT('Ctrl Pts',(5.7299307791557,-78.5617511126201,9.92453123330913));
#20780=CARTESIAN_POINT('Ctrl Pts',(8.59489616871569,-78.3867511126201,4.96226561664425));
#20781=CARTESIAN_POINT('Ctrl Pts',(11.4598615582757,-78.2117511126201,-2.06354052510241E-11));
#20782=CARTESIAN_POINT('Ctrl Pts',(8.59489616869782,-78.0367511126201,-4.9622656166752));
#20783=CARTESIAN_POINT('Ctrl Pts',(5.72993077911996,-77.8617511126201,-9.92453123332976));
#20784=CARTESIAN_POINT('Ctrl Pts',(-1.78726082715848E-11,-77.6867511126201,
-9.92453123331945));
#20785=CARTESIAN_POINT('Ctrl Pts',(-5.7299307791557,-77.5117511126201,-9.92453123330913));
#20786=CARTESIAN_POINT('Ctrl Pts',(-8.59489616871569,-77.3367511126201,
-4.96226561664425));
#20787=CARTESIAN_POINT('Ctrl Pts',(-11.4598615582757,-77.1617511126201,
2.06368086793017E-11));
#20788=CARTESIAN_POINT('Ctrl Pts',(-8.59489616869782,-76.9867511126201,
4.9622656166752));
#20789=CARTESIAN_POINT('Ctrl Pts',(-5.72993077911996,-76.8117511126201,
9.92453123332977));
#20790=CARTESIAN_POINT('Ctrl Pts',(1.7871392867044E-11,-76.6367511126201,
9.92453123331945));
#20791=CARTESIAN_POINT('Ctrl Pts',(5.7299307791557,-76.4617511126201,9.92453123330913));
#20792=CARTESIAN_POINT('Ctrl Pts',(8.59489616871569,-76.2867511126201,4.96226561664425));
#20793=CARTESIAN_POINT('Ctrl Pts',(11.4598615582757,-76.1117511126201,-2.06354052510241E-11));
#20794=CARTESIAN_POINT('Ctrl Pts',(8.59489616869782,-75.9367511126201,-4.9622656166752));
#20795=CARTESIAN_POINT('Ctrl Pts',(5.72993077911996,-75.7617511126201,-9.92453123332976));
#20796=CARTESIAN_POINT('Ctrl Pts',(-1.78726082715848E-11,-75.5867511126201,
-9.92453123331945));
#20797=CARTESIAN_POINT('Ctrl Pts',(-5.7299307791557,-75.4117511126202,-9.92453123330913));
#20798=CARTESIAN_POINT('Ctrl Pts',(-8.59489616871569,-75.2367511126201,
-4.96226561664425));
#20799=CARTESIAN_POINT('Ctrl Pts',(-11.4598615582757,-75.0617511126201,
2.06368086793017E-11));
#20800=CARTESIAN_POINT('Ctrl Pts',(-8.59489616869782,-74.8867511126201,
4.9622656166752));
#20801=CARTESIAN_POINT('Ctrl Pts',(-5.72993077911996,-74.7117511126201,
9.92453123332977));
#20802=CARTESIAN_POINT('Ctrl Pts',(1.7871392867044E-11,-74.5367511126201,
9.92453123331945));
#20803=CARTESIAN_POINT('Ctrl Pts',(5.7299307791557,-74.3617511126201,9.92453123330913));
#20804=CARTESIAN_POINT('Ctrl Pts',(8.59489616871569,-74.1867511126201,4.96226561664425));
#20805=CARTESIAN_POINT('Ctrl Pts',(11.4598615582757,-74.0117511126201,-2.06354052510241E-11));
#20806=CARTESIAN_POINT('Ctrl Pts',(8.59489616869782,-73.8367511126201,-4.9622656166752));
#20807=CARTESIAN_POINT('Ctrl Pts',(5.72993077911996,-73.6617511126201,-9.92453123332976));
#20808=CARTESIAN_POINT('Ctrl Pts',(-1.78726082715848E-11,-73.4867511126201,
-9.92453123331945));
#20809=CARTESIAN_POINT('Ctrl Pts',(-5.7299307791557,-73.3117511126201,-9.92453123330913));
#20810=CARTESIAN_POINT('Ctrl Pts',(-8.59489616871569,-73.1367511126201,
-4.96226561664425));
#20811=CARTESIAN_POINT('Ctrl Pts',(-11.4598615582757,-72.9617511126201,
2.06368086793017E-11));
#20812=CARTESIAN_POINT('Ctrl Pts',(-8.59489616869782,-72.7867511126201,
4.9622656166752));
#20813=CARTESIAN_POINT('Ctrl Pts',(-5.72993077911996,-72.6117511126201,
9.92453123332977));
#20814=CARTESIAN_POINT('Ctrl Pts',(1.7871392867044E-11,-72.4367511126201,
9.92453123331945));
#20815=CARTESIAN_POINT('Ctrl Pts',(5.7299307791557,-72.2617511126201,9.92453123330913));
#20816=CARTESIAN_POINT('Ctrl Pts',(8.59489616871569,-72.0867511126201,4.96226561664425));
#20817=CARTESIAN_POINT('Ctrl Pts',(11.4598615582757,-71.9117511126201,-2.06354052510241E-11));
#20818=CARTESIAN_POINT('Ctrl Pts',(8.59489616869782,-71.7367511126201,-4.9622656166752));
#20819=CARTESIAN_POINT('Ctrl Pts',(5.72993077911996,-71.5617511126201,-9.92453123332976));
#20820=CARTESIAN_POINT('Ctrl Pts',(-1.78726082715848E-11,-71.3867511126201,
-9.92453123331945));
#20821=CARTESIAN_POINT('Ctrl Pts',(-5.7299307791557,-71.2117511126201,-9.92453123330913));
#20822=CARTESIAN_POINT('Ctrl Pts',(-8.59489616871569,-71.0367511126201,
-4.96226561664425));
#20823=CARTESIAN_POINT('Ctrl Pts',(-11.4598615582757,-70.8617511126201,
2.06368086793017E-11));
#20824=CARTESIAN_POINT('Ctrl Pts',(-8.59489616869782,-70.6867511126201,
4.9622656166752));
#20825=CARTESIAN_POINT('Ctrl Pts',(-5.72993077911996,-70.5117511126201,
9.92453123332977));
#20826=CARTESIAN_POINT('Ctrl Pts',(1.7871392867044E-11,-70.3367511126201,
9.92453123331945));
#20827=CARTESIAN_POINT('Ctrl Pts',(5.7299307791557,-70.1617511126201,9.92453123330913));
#20828=CARTESIAN_POINT('Ctrl Pts',(8.59489616871569,-69.9867511126201,4.96226561664425));
#20829=CARTESIAN_POINT('Ctrl Pts',(11.4598615582757,-69.8117511126202,-2.06354052510241E-11));
#20830=CARTESIAN_POINT('Ctrl Pts',(8.59489616869782,-69.6367511126201,-4.9622656166752));
#20831=CARTESIAN_POINT('Ctrl Pts',(5.72993077911996,-69.4617511126201,-9.92453123332976));
#20832=CARTESIAN_POINT('Ctrl Pts',(-1.78726082715848E-11,-69.2867511126201,
-9.92453123331945));
#20833=CARTESIAN_POINT('Ctrl Pts',(-5.7299307791557,-69.1117511126201,-9.92453123330913));
#20834=CARTESIAN_POINT('Ctrl Pts',(-8.59489616871569,-68.9367511126201,
-4.96226561664425));
#20835=CARTESIAN_POINT('Ctrl Pts',(-11.4598615582757,-68.7617511126201,
2.06368086793017E-11));
#20836=CARTESIAN_POINT('Ctrl Pts',(-8.59489616869782,-68.5867511126201,
4.9622656166752));
#20837=CARTESIAN_POINT('Ctrl Pts',(-5.72993077911996,-68.4117511126201,
9.92453123332977));
#20838=CARTESIAN_POINT('Ctrl Pts',(1.7871392867044E-11,-68.2367511126201,
9.92453123331945));
#20839=CARTESIAN_POINT('Ctrl Pts',(5.7299307791557,-68.0617511126201,9.92453123330913));
#20840=CARTESIAN_POINT('Ctrl Pts',(8.59489616871569,-67.8867511126201,4.96226561664425));
#20841=CARTESIAN_POINT('Ctrl Pts',(11.4598615582757,-67.7117511126201,-2.06354052510241E-11));
#20842=CARTESIAN_POINT('Ctrl Pts',(8.59489616869782,-67.5367511126201,-4.9622656166752));
#20843=CARTESIAN_POINT('Ctrl Pts',(5.72993077911996,-67.3617511126201,-9.92453123332976));
#20844=CARTESIAN_POINT('Ctrl Pts',(-1.78726082715848E-11,-67.1867511126202,
-9.92453123331945));
#20845=CARTESIAN_POINT('Ctrl Pts',(-5.7299307791557,-67.0117511126201,-9.92453123330913));
#20846=CARTESIAN_POINT('Ctrl Pts',(-8.59489616871569,-66.8367511126201,
-4.96226561664425));
#20847=CARTESIAN_POINT('Ctrl Pts',(-11.4598615582757,-66.6617511126202,
2.06368086793017E-11));
#20848=CARTESIAN_POINT('Ctrl Pts',(-8.59489616869782,-66.4867511126201,
4.9622656166752));
#20849=CARTESIAN_POINT('Ctrl Pts',(-5.72993077911996,-66.3117511126201,
9.92453123332977));
#20850=CARTESIAN_POINT('Ctrl Pts',(1.7871392867044E-11,-66.1367511126202,
9.92453123331945));
#20851=CARTESIAN_POINT('Ctrl Pts',(5.7299307791557,-65.9617511126201,9.92453123330913));
#20852=CARTESIAN_POINT('Ctrl Pts',(8.59489616871569,-65.7867511126201,4.96226561664425));
#20853=CARTESIAN_POINT('Ctrl Pts',(11.4598615582757,-65.6117511126202,-2.06354052510241E-11));
#20854=CARTESIAN_POINT('Ctrl Pts',(8.59489616869782,-65.4367511126201,-4.9622656166752));
#20855=CARTESIAN_POINT('Ctrl Pts',(5.72993077911996,-65.2617511126201,-9.92453123332976));
#20856=CARTESIAN_POINT('Ctrl Pts',(-1.78726082715848E-11,-65.0867511126201,
-9.92453123331945));
#20857=CARTESIAN_POINT('Ctrl Pts',(-5.7299307791557,-64.9117511126201,-9.92453123330913));
#20858=CARTESIAN_POINT('Ctrl Pts',(-8.59489616871569,-64.7367511126201,
-4.96226561664425));
#20859=CARTESIAN_POINT('Ctrl Pts',(-11.4598615582757,-64.5617511126202,
2.06368086793017E-11));
#20860=CARTESIAN_POINT('Ctrl Pts',(-8.59489616869782,-64.3867511126201,
4.9622656166752));
#20861=CARTESIAN_POINT('Ctrl Pts',(-5.72993077911996,-64.2117511126201,
9.92453123332977));
#20862=CARTESIAN_POINT('Ctrl Pts',(1.7871392867044E-11,-64.0367511126202,
9.92453123331945));
#20863=CARTESIAN_POINT('Ctrl Pts',(5.7299307791557,-63.8617511126201,9.92453123330913));
#20864=CARTESIAN_POINT('Ctrl Pts',(8.59489616871569,-63.6867511126202,4.96226561664425));
#20865=CARTESIAN_POINT('Ctrl Pts',(11.4598615582757,-63.5117511126202,-2.06354052510241E-11));
#20866=CARTESIAN_POINT('Ctrl Pts',(8.59489616869782,-63.3367511126201,-4.9622656166752));
#20867=CARTESIAN_POINT('Ctrl Pts',(5.72993077911996,-63.1617511126202,-9.92453123332976));
#20868=CARTESIAN_POINT('Ctrl Pts',(-1.78726082715848E-11,-62.9867511126201,
-9.92453123331945));
#20869=CARTESIAN_POINT('Ctrl Pts',(-5.7299307791557,-62.8117511126201,-9.92453123330913));
#20870=CARTESIAN_POINT('Ctrl Pts',(-8.59489616871569,-62.6367511126202,
-4.96226561664425));
#20871=CARTESIAN_POINT('Ctrl Pts',(-11.4598615582757,-62.4617511126202,
2.06368086793017E-11));
#20872=CARTESIAN_POINT('Ctrl Pts',(-8.59489616869782,-62.2867511126201,
4.9622656166752));
#20873=CARTESIAN_POINT('Ctrl Pts',(-5.72993077911996,-62.1117511126202,
9.92453123332977));
#20874=CARTESIAN_POINT('Ctrl Pts',(1.7871392867044E-11,-61.9367511126202,
9.92453123331945));
#20875=CARTESIAN_POINT('Ctrl Pts',(5.7299307791557,-61.7617511126201,9.92453123330913));
#20876=CARTESIAN_POINT('Ctrl Pts',(8.59489616871569,-61.5867511126202,4.96226561664425));
#20877=CARTESIAN_POINT('Ctrl Pts',(11.4598615582757,-61.4117511126202,-2.06354052510241E-11));
#20878=CARTESIAN_POINT('Ctrl Pts',(8.59489616869782,-61.2367511126201,-4.9622656166752));
#20879=CARTESIAN_POINT('Ctrl Pts',(5.72993077911996,-61.0617511126202,-9.92453123332976));
#20880=CARTESIAN_POINT('Ctrl Pts',(-1.78726082715848E-11,-60.8867511126202,
-9.92453123331945));
#20881=CARTESIAN_POINT('Ctrl Pts',(-5.7299307791557,-60.7117511126201,-9.92453123330913));
#20882=CARTESIAN_POINT('Ctrl Pts',(-8.59489616871569,-60.5367511126202,
-4.96226561664425));
#20883=CARTESIAN_POINT('Ctrl Pts',(-11.4598615582757,-60.3617511126202,
2.06368086793017E-11));
#20884=CARTESIAN_POINT('Ctrl Pts',(-8.59489616869782,-60.1867511126201,
4.9622656166752));
#20885=CARTESIAN_POINT('Ctrl Pts',(-5.72993077911996,-60.0117511126202,
9.92453123332977));
#20886=CARTESIAN_POINT('Ctrl Pts',(1.7871392867044E-11,-59.8367511126202,
9.92453123331945));
#20887=CARTESIAN_POINT('Ctrl Pts',(5.7299307791557,-59.6617511126202,9.92453123330913));
#20888=CARTESIAN_POINT('Ctrl Pts',(8.59489616871569,-59.4867511126202,4.96226561664425));
#20889=CARTESIAN_POINT('Ctrl Pts',(11.4598615582757,-59.3117511126202,-2.06354052510241E-11));
#20890=CARTESIAN_POINT('Ctrl Pts',(8.59489616869782,-59.1367511126202,-4.9622656166752));
#20891=CARTESIAN_POINT('Ctrl Pts',(5.72993077911996,-58.9617511126202,-9.92453123332976));
#20892=CARTESIAN_POINT('Ctrl Pts',(-1.78726082715848E-11,-58.7867511126202,
-9.92453123331945));
#20893=CARTESIAN_POINT('Ctrl Pts',(-5.7299307791557,-58.6117511126201,-9.92453123330913));
#20894=CARTESIAN_POINT('Ctrl Pts',(-8.59489616871569,-58.4367511126202,
-4.96226561664425));
#20895=CARTESIAN_POINT('Ctrl Pts',(-11.4598615582757,-58.2617511126201,
2.06368086793017E-11));
#20896=CARTESIAN_POINT('Ctrl Pts',(-8.59489616869782,-58.0867511126202,
4.9622656166752));
#20897=CARTESIAN_POINT('Ctrl Pts',(-5.72993077911996,-57.9117511126202,
9.92453123332977));
#20898=CARTESIAN_POINT('Ctrl Pts',(1.7871392867044E-11,-57.7367511126201,
9.92453123331945));
#20899=CARTESIAN_POINT('Ctrl Pts',(5.7299307791557,-57.5617511126202,9.92453123330913));
#20900=CARTESIAN_POINT('Ctrl Pts',(8.59489616871569,-57.3867511126202,4.96226561664425));
#20901=CARTESIAN_POINT('Ctrl Pts',(11.4598615582757,-57.2117511126201,-2.06354052510241E-11));
#20902=CARTESIAN_POINT('Ctrl Pts',(8.59489616869782,-57.0367511126202,-4.9622656166752));
#20903=CARTESIAN_POINT('Ctrl Pts',(5.72993077911996,-56.8617511126202,-9.92453123332976));
#20904=CARTESIAN_POINT('Ctrl Pts',(-1.78726082715848E-11,-56.6867511126202,
-9.92453123331945));
#20905=CARTESIAN_POINT('Ctrl Pts',(-5.7299307791557,-56.5117511126202,-9.92453123330913));
#20906=CARTESIAN_POINT('Ctrl Pts',(-8.59489616871569,-56.3367511126202,
-4.96226561664425));
#20907=CARTESIAN_POINT('Ctrl Pts',(-11.4598615582757,-56.1617511126202,
2.06368086793017E-11));
#20908=CARTESIAN_POINT('Ctrl Pts',(-8.59489616869782,-55.9867511126202,
4.9622656166752));
#20909=CARTESIAN_POINT('Ctrl Pts',(-5.72993077911996,-55.8117511126202,
9.92453123332977));
#20910=CARTESIAN_POINT('Ctrl Pts',(1.7871392867044E-11,-55.6367511126201,
9.92453123331945));
#20911=CARTESIAN_POINT('Ctrl Pts',(5.7299307791557,-55.4617511126202,9.92453123330913));
#20912=CARTESIAN_POINT('Ctrl Pts',(8.59489616871569,-55.2867511126202,4.96226561664425));
#20913=CARTESIAN_POINT('Ctrl Pts',(11.4598615582757,-55.1117511126202,-2.06354052510241E-11));
#20914=CARTESIAN_POINT('Ctrl Pts',(8.59489616869782,-54.9367511126202,-4.9622656166752));
#20915=CARTESIAN_POINT('Ctrl Pts',(5.72993077911996,-54.7617511126202,-9.92453123332976));
#20916=CARTESIAN_POINT('Ctrl Pts',(-1.78726082715848E-11,-54.5867511126202,
-9.92453123331945));
#20917=CARTESIAN_POINT('Ctrl Pts',(-5.7299307791557,-54.4117511126202,-9.92453123330913));
#20918=CARTESIAN_POINT('Ctrl Pts',(-8.59489616871569,-54.2367511126202,
-4.96226561664425));
#20919=CARTESIAN_POINT('Ctrl Pts',(-11.4598615582757,-54.0617511126202,
2.06368086793017E-11));
#20920=CARTESIAN_POINT('Ctrl Pts',(-8.59489616869782,-53.8867511126202,
4.9622656166752));
#20921=CARTESIAN_POINT('Ctrl Pts',(-5.72993077911996,-53.7117511126202,
9.92453123332977));
#20922=CARTESIAN_POINT('Ctrl Pts',(1.7871392867044E-11,-53.5367511126202,
9.92453123331945));
#20923=CARTESIAN_POINT('Ctrl Pts',(5.7299307791557,-53.3617511126202,9.92453123330913));
#20924=CARTESIAN_POINT('Ctrl Pts',(8.59489616871569,-53.1867511126202,4.96226561664425));
#20925=CARTESIAN_POINT('Ctrl Pts',(11.4598615582757,-53.0117511126202,-2.06354052510241E-11));
#20926=CARTESIAN_POINT('Ctrl Pts',(8.59489616869782,-52.8367511126202,-4.9622656166752));
#20927=CARTESIAN_POINT('Ctrl Pts',(5.72993077911996,-52.6617511126202,-9.92453123332976));
#20928=CARTESIAN_POINT('Ctrl Pts',(-1.78726082715848E-11,-52.4867511126202,
-9.92453123331945));
#20929=CARTESIAN_POINT('Ctrl Pts',(-5.7299307791557,-52.3117511126202,-9.92453123330913));
#20930=CARTESIAN_POINT('Ctrl Pts',(-8.59489616871569,-52.1367511126202,
-4.96226561664425));
#20931=CARTESIAN_POINT('Ctrl Pts',(-11.4598615582757,-51.9617511126202,
2.06368086793017E-11));
#20932=CARTESIAN_POINT('Ctrl Pts',(-8.59489616869782,-51.7867511126202,
4.9622656166752));
#20933=CARTESIAN_POINT('Ctrl Pts',(-5.72993077911996,-51.6117511126202,
9.92453123332977));
#20934=CARTESIAN_POINT('Ctrl Pts',(1.7871392867044E-11,-51.4367511126202,
9.92453123331945));
#20935=CARTESIAN_POINT('Ctrl Pts',(5.7299307791557,-51.2617511126202,9.92453123330913));
#20936=CARTESIAN_POINT('Ctrl Pts',(8.59489616871569,-51.0867511126202,4.96226561664425));
#20937=CARTESIAN_POINT('Ctrl Pts',(11.4598615582757,-50.9117511126202,-2.06354052510241E-11));
#20938=CARTESIAN_POINT('Ctrl Pts',(8.59489616869782,-50.7367511126202,-4.9622656166752));
#20939=CARTESIAN_POINT('Ctrl Pts',(5.72993077911996,-50.5617511126202,-9.92453123332976));
#20940=CARTESIAN_POINT('Ctrl Pts',(-1.78726082715848E-11,-50.3867511126202,
-9.92453123331945));
#20941=CARTESIAN_POINT('Ctrl Pts',(-5.7299307791557,-50.2117511126202,-9.92453123330913));
#20942=CARTESIAN_POINT('Ctrl Pts',(-8.59489616871569,-50.0367511126202,
-4.96226561664425));
#20943=CARTESIAN_POINT('Ctrl Pts',(-11.4598615582757,-49.8617511126202,
2.06368086793017E-11));
#20944=CARTESIAN_POINT('Ctrl Pts',(-8.59489616869782,-49.6867511126202,
4.9622656166752));
#20945=CARTESIAN_POINT('Ctrl Pts',(-5.72993077911996,-49.5117511126202,
9.92453123332977));
#20946=CARTESIAN_POINT('Ctrl Pts',(1.7871392867044E-11,-49.3367511126202,
9.92453123331945));
#20947=CARTESIAN_POINT('Ctrl Pts',(5.7299307791557,-49.1617511126202,9.92453123330913));
#20948=CARTESIAN_POINT('Ctrl Pts',(8.59489616871569,-48.9867511126202,4.96226561664425));
#20949=CARTESIAN_POINT('Ctrl Pts',(11.4598615582757,-48.8117511126202,-2.06354052510241E-11));
#20950=CARTESIAN_POINT('Ctrl Pts',(8.59489616869782,-48.6367511126202,-4.9622656166752));
#20951=CARTESIAN_POINT('Ctrl Pts',(5.72993077911996,-48.4617511126202,-9.92453123332976));
#20952=CARTESIAN_POINT('Ctrl Pts',(-1.78726082715848E-11,-48.2867511126202,
-9.92453123331945));
#20953=CARTESIAN_POINT('Ctrl Pts',(-5.7299307791557,-48.1117511126202,-9.92453123330913));
#20954=CARTESIAN_POINT('Ctrl Pts',(-8.59489616871569,-47.9367511126202,
-4.96226561664425));
#20955=CARTESIAN_POINT('Ctrl Pts',(-11.4598615582757,-47.7617511126202,
2.06368086793017E-11));
#20956=CARTESIAN_POINT('Ctrl Pts',(-8.59489616869782,-47.5867511126202,
4.9622656166752));
#20957=CARTESIAN_POINT('Ctrl Pts',(-5.72993077911996,-47.4117511126202,
9.92453123332977));
#20958=CARTESIAN_POINT('Ctrl Pts',(1.7871392867044E-11,-47.2367511126202,
9.92453123331945));
#20959=CARTESIAN_POINT('Ctrl Pts',(5.7299307791557,-47.0617511126202,9.92453123330913));
#20960=CARTESIAN_POINT('Ctrl Pts',(8.59489616871569,-46.8867511126202,4.96226561664425));
#20961=CARTESIAN_POINT('Ctrl Pts',(11.4598615582757,-46.7117511126202,-2.06354052510241E-11));
#20962=CARTESIAN_POINT('Ctrl Pts',(8.59489616869782,-46.5367511126202,-4.9622656166752));
#20963=CARTESIAN_POINT('Ctrl Pts',(5.72993077911996,-46.3617511126202,-9.92453123332976));
#20964=CARTESIAN_POINT('Ctrl Pts',(-1.78726082715848E-11,-46.1867511126202,
-9.92453123331945));
#20965=CARTESIAN_POINT('Ctrl Pts',(-5.7299307791557,-46.0117511126202,-9.92453123330913));
#20966=CARTESIAN_POINT('Ctrl Pts',(-8.59489616871569,-45.8367511126202,
-4.96226561664425));
#20967=CARTESIAN_POINT('Ctrl Pts',(-11.4598615582757,-45.6617511126202,
2.06368086793017E-11));
#20968=CARTESIAN_POINT('Ctrl Pts',(-8.59489616869782,-45.4867511126202,
4.9622656166752));
#20969=CARTESIAN_POINT('Ctrl Pts',(-5.72993077911996,-45.3117511126202,
9.92453123332977));
#20970=CARTESIAN_POINT('Ctrl Pts',(1.7871392867044E-11,-45.1367511126202,
9.92453123331945));
#20971=CARTESIAN_POINT('Ctrl Pts',(5.7299307791557,-44.9617511126202,9.92453123330913));
#20972=CARTESIAN_POINT('Ctrl Pts',(8.59489616871569,-44.7867511126202,4.96226561664425));
#20973=CARTESIAN_POINT('Ctrl Pts',(11.4598615582757,-44.6117511126202,-2.06354052510241E-11));
#20974=CARTESIAN_POINT('Ctrl Pts',(8.59489616869782,-44.4367511126202,-4.9622656166752));
#20975=CARTESIAN_POINT('Ctrl Pts',(5.72993077911996,-44.2617511126202,-9.92453123332976));
#20976=CARTESIAN_POINT('Ctrl Pts',(-1.78726082715848E-11,-44.0867511126202,
-9.92453123331945));
#20977=CARTESIAN_POINT('Ctrl Pts',(-5.7299307791557,-43.9117511126202,-9.92453123330913));
#20978=CARTESIAN_POINT('Ctrl Pts',(-8.59489616871569,-43.7367511126202,
-4.96226561664425));
#20979=CARTESIAN_POINT('Ctrl Pts',(-11.4598615582757,-43.5617511126202,
2.06368086793017E-11));
#20980=CARTESIAN_POINT('Ctrl Pts',(-8.59489616869782,-43.3867511126202,
4.9622656166752));
#20981=CARTESIAN_POINT('Ctrl Pts',(-5.72993077911996,-43.2117511126202,
9.92453123332977));
#20982=CARTESIAN_POINT('Ctrl Pts',(1.7871392867044E-11,-43.0367511126202,
9.92453123331945));
#20983=CARTESIAN_POINT('Ctrl Pts',(5.7299307791557,-42.8617511126202,9.92453123330913));
#20984=CARTESIAN_POINT('Ctrl Pts',(8.59489616871569,-42.6867511126202,4.96226561664425));
#20985=CARTESIAN_POINT('Ctrl Pts',(11.4598615582757,-42.5117511126202,-2.06354052510241E-11));
#20986=CARTESIAN_POINT('Ctrl Pts',(8.59489616869782,-42.3367511126202,-4.9622656166752));
#20987=CARTESIAN_POINT('Ctrl Pts',(5.72993077911996,-42.1617511126202,-9.92453123332976));
#20988=CARTESIAN_POINT('Ctrl Pts',(-1.78726082715848E-11,-41.9867511126202,
-9.92453123331945));
#20989=CARTESIAN_POINT('Ctrl Pts',(-5.7299307791557,-41.8117511126202,-9.92453123330913));
#20990=CARTESIAN_POINT('Ctrl Pts',(-8.59489616871569,-41.6367511126202,
-4.96226561664425));
#20991=CARTESIAN_POINT('Ctrl Pts',(-11.4598615582757,-41.4617511126202,
2.06368086793017E-11));
#20992=CARTESIAN_POINT('Ctrl Pts',(-8.59489616869782,-41.2867511126202,
4.9622656166752));
#20993=CARTESIAN_POINT('Ctrl Pts',(-5.72993077911996,-41.1117511126202,
9.92453123332977));
#20994=CARTESIAN_POINT('Ctrl Pts',(1.7871392867044E-11,-40.9367511126202,
9.92453123331945));
#20995=CARTESIAN_POINT('Ctrl Pts',(5.7299307791557,-40.7617511126202,9.92453123330913));
#20996=CARTESIAN_POINT('Ctrl Pts',(8.59489616871569,-40.5867511126202,4.96226561664425));
#20997=CARTESIAN_POINT('Ctrl Pts',(11.4598615582757,-40.4117511126202,-2.06354052510241E-11));
#20998=CARTESIAN_POINT('Ctrl Pts',(8.59489616869782,-40.2367511126202,-4.9622656166752));
#20999=CARTESIAN_POINT('Ctrl Pts',(5.72993077911996,-40.0617511126202,-9.92453123332976));
#21000=CARTESIAN_POINT('Ctrl Pts',(-1.78726082715848E-11,-39.8867511126202,
-9.92453123331945));
#21001=CARTESIAN_POINT('Ctrl Pts',(-5.7299307791557,-39.7117511126202,-9.92453123330913));
#21002=CARTESIAN_POINT('Ctrl Pts',(-8.59489616871569,-39.5367511126202,
-4.96226561664425));
#21003=CARTESIAN_POINT('Ctrl Pts',(-11.4598615582757,-39.3617511126202,
2.06368086793017E-11));
#21004=CARTESIAN_POINT('Ctrl Pts',(-8.59489616869782,-39.1867511126202,
4.9622656166752));
#21005=CARTESIAN_POINT('Ctrl Pts',(-5.72993077911996,-39.0117511126202,
9.92453123332977));
#21006=CARTESIAN_POINT('Ctrl Pts',(1.7871392867044E-11,-38.8367511126202,
9.92453123331945));
#21007=CARTESIAN_POINT('Ctrl Pts',(5.7299307791557,-38.6617511126202,9.92453123330913));
#21008=CARTESIAN_POINT('Ctrl Pts',(8.59489616871569,-38.4867511126202,4.96226561664425));
#21009=CARTESIAN_POINT('Ctrl Pts',(11.4598615582757,-38.3117511126202,-2.06354052510241E-11));
#21010=CARTESIAN_POINT('Ctrl Pts',(8.59489616869782,-38.1367511126202,-4.9622656166752));
#21011=CARTESIAN_POINT('Ctrl Pts',(5.72993077911996,-37.9617511126202,-9.92453123332976));
#21012=CARTESIAN_POINT('Ctrl Pts',(-1.78726082715848E-11,-37.7867511126202,
-9.92453123331945));
#21013=CARTESIAN_POINT('Ctrl Pts',(-5.7299307791557,-37.6117511126202,-9.92453123330913));
#21014=CARTESIAN_POINT('Ctrl Pts',(-8.59489616871569,-37.4367511126202,
-4.96226561664425));
#21015=CARTESIAN_POINT('Ctrl Pts',(-11.4598615582757,-37.2617511126202,
2.06368086793017E-11));
#21016=CARTESIAN_POINT('Ctrl Pts',(-8.59489616869782,-37.0867511126202,
4.9622656166752));
#21017=CARTESIAN_POINT('Ctrl Pts',(-5.72993077911996,-36.9117511126202,
9.92453123332977));
#21018=CARTESIAN_POINT('Ctrl Pts',(1.7871392867044E-11,-36.7367511126202,
9.92453123331945));
#21019=CARTESIAN_POINT('Ctrl Pts',(5.7299307791557,-36.5617511126202,9.92453123330913));
#21020=CARTESIAN_POINT('Ctrl Pts',(8.59489616871569,-36.3867511126202,4.96226561664425));
#21021=CARTESIAN_POINT('Ctrl Pts',(11.4598615582757,-36.2117511126202,-2.06354052510241E-11));
#21022=CARTESIAN_POINT('Ctrl Pts',(8.59489616869782,-36.0367511126202,-4.9622656166752));
#21023=CARTESIAN_POINT('Ctrl Pts',(5.72993077911996,-35.8617511126202,-9.92453123332976));
#21024=CARTESIAN_POINT('Ctrl Pts',(-1.78726082715848E-11,-35.6867511126202,
-9.92453123331945));
#21025=CARTESIAN_POINT('Ctrl Pts',(-5.7299307791557,-35.5117511126202,-9.92453123330913));
#21026=CARTESIAN_POINT('Ctrl Pts',(-8.59489616871569,-35.3367511126202,
-4.96226561664425));
#21027=CARTESIAN_POINT('Ctrl Pts',(-11.4598615582757,-35.1617511126202,
2.06368086793017E-11));
#21028=CARTESIAN_POINT('Ctrl Pts',(-8.59489616869782,-34.9867511126202,
4.9622656166752));
#21029=CARTESIAN_POINT('Ctrl Pts',(-5.72993077911996,-34.8117511126202,
9.92453123332977));
#21030=CARTESIAN_POINT('Ctrl Pts',(1.7871392867044E-11,-34.6367511126202,
9.92453123331945));
#21031=CARTESIAN_POINT('Ctrl Pts',(5.7299307791557,-34.4617511126202,9.92453123330913));
#21032=CARTESIAN_POINT('Ctrl Pts',(8.59489616871569,-34.2867511126202,4.96226561664425));
#21033=CARTESIAN_POINT('Ctrl Pts',(11.4598615582757,-34.1117511126202,-2.06354052510241E-11));
#21034=CARTESIAN_POINT('Ctrl Pts',(8.59489616869782,-33.9367511126202,-4.9622656166752));
#21035=CARTESIAN_POINT('Ctrl Pts',(5.72993077911996,-33.7617511126202,-9.92453123332976));
#21036=CARTESIAN_POINT('Ctrl Pts',(-1.78726082715848E-11,-33.5867511126202,
-9.92453123331945));
#21037=CARTESIAN_POINT('Ctrl Pts',(-5.7299307791557,-33.4117511126202,-9.92453123330913));
#21038=CARTESIAN_POINT('Ctrl Pts',(-8.59489616871569,-33.2367511126202,
-4.96226561664425));
#21039=CARTESIAN_POINT('Ctrl Pts',(-11.4598615582757,-33.0617511126202,
2.06368086793017E-11));
#21040=CARTESIAN_POINT('Ctrl Pts',(-8.59489616869782,-32.8867511126202,
4.9622656166752));
#21041=CARTESIAN_POINT('Ctrl Pts',(-5.72993077911996,-32.7117511126202,
9.92453123332977));
#21042=CARTESIAN_POINT('Ctrl Pts',(1.7871392867044E-11,-32.5367511126202,
9.92453123331945));
#21043=CARTESIAN_POINT('Ctrl Pts',(5.7299307791557,-32.3617511126202,9.92453123330913));
#21044=CARTESIAN_POINT('Ctrl Pts',(8.59489616871569,-32.1867511126202,4.96226561664425));
#21045=CARTESIAN_POINT('Ctrl Pts',(11.4598615582757,-32.0117511126202,-2.06354052510241E-11));
#21046=CARTESIAN_POINT('Ctrl Pts',(8.59489616869782,-31.8367511126202,-4.9622656166752));
#21047=CARTESIAN_POINT('Ctrl Pts',(5.72993077911996,-31.6617511126202,-9.92453123332976));
#21048=CARTESIAN_POINT('Ctrl Pts',(-1.78726082715848E-11,-31.4867511126202,
-9.92453123331945));
#21049=CARTESIAN_POINT('Ctrl Pts',(-5.7299307791557,-31.3117511126202,-9.92453123330913));
#21050=CARTESIAN_POINT('Ctrl Pts',(-8.59489616871569,-31.1367511126202,
-4.96226561664425));
#21051=CARTESIAN_POINT('Ctrl Pts',(-11.4598615582757,-30.9617511126202,
2.06368086793017E-11));
#21052=CARTESIAN_POINT('Ctrl Pts',(-8.59489616869782,-30.7867511126202,
4.9622656166752));
#21053=CARTESIAN_POINT('Ctrl Pts',(-5.72993077911996,-30.6117511126202,
9.92453123332977));
#21054=CARTESIAN_POINT('Ctrl Pts',(1.7871392867044E-11,-30.4367511126202,
9.92453123331945));
#21055=CARTESIAN_POINT('Ctrl Pts',(5.7299307791557,-30.2617511126202,9.92453123330913));
#21056=CARTESIAN_POINT('Ctrl Pts',(8.59489616871569,-30.0867511126202,4.96226561664425));
#21057=CARTESIAN_POINT('Ctrl Pts',(11.4598615582757,-29.9117511126202,-2.06354052510241E-11));
#21058=CARTESIAN_POINT('Ctrl Pts',(8.59489616869782,-29.7367511126202,-4.9622656166752));
#21059=CARTESIAN_POINT('Ctrl Pts',(5.72993077911996,-29.5617511126202,-9.92453123332976));
#21060=CARTESIAN_POINT('Ctrl Pts',(-1.78726082715848E-11,-29.3867511126202,
-9.92453123331945));
#21061=CARTESIAN_POINT('Ctrl Pts',(-5.7299307791557,-29.2117511126202,-9.92453123330913));
#21062=CARTESIAN_POINT('Ctrl Pts',(-8.59489616871569,-29.0367511126202,
-4.96226561664425));
#21063=CARTESIAN_POINT('Ctrl Pts',(-11.4598615582757,-28.8617511126202,
2.06368086793017E-11));
#21064=CARTESIAN_POINT('Ctrl Pts',(-8.59489616869782,-28.6867511126202,
4.9622656166752));
#21065=CARTESIAN_POINT('Ctrl Pts',(-5.72993077911996,-28.5117511126202,
9.92453123332977));
#21066=CARTESIAN_POINT('Ctrl Pts',(1.7871392867044E-11,-28.3367511126202,
9.92453123331945));
#21067=CARTESIAN_POINT('Ctrl Pts',(5.7299307791557,-28.1617511126202,9.92453123330913));
#21068=CARTESIAN_POINT('Ctrl Pts',(8.59489616871569,-27.9867511126202,4.96226561664425));
#21069=CARTESIAN_POINT('Ctrl Pts',(11.4598615582757,-27.8117511126202,-2.06354052510241E-11));
#21070=CARTESIAN_POINT('Ctrl Pts',(8.59489616869782,-27.6367511126202,-4.9622656166752));
#21071=CARTESIAN_POINT('Ctrl Pts',(5.72993077911996,-27.4617511126202,-9.92453123332976));
#21072=CARTESIAN_POINT('Ctrl Pts',(-1.78726082715848E-11,-27.2867511126202,
-9.92453123331945));
#21073=CARTESIAN_POINT('Ctrl Pts',(-5.7299307791557,-27.1117511126202,-9.92453123330913));
#21074=CARTESIAN_POINT('Ctrl Pts',(-8.59489616871569,-26.9367511126202,
-4.96226561664425));
#21075=CARTESIAN_POINT('Ctrl Pts',(-11.4598615582757,-26.7617511126202,
2.06368086793017E-11));
#21076=CARTESIAN_POINT('Ctrl Pts',(-8.59489616869782,-26.5867511126202,
4.9622656166752));
#21077=CARTESIAN_POINT('Ctrl Pts',(-5.72993077911996,-26.4117511126202,
9.92453123332977));
#21078=CARTESIAN_POINT('Ctrl Pts',(1.7871392867044E-11,-26.2367511126202,
9.92453123331945));
#21079=CARTESIAN_POINT('Ctrl Pts',(5.7299307791557,-26.0617511126202,9.92453123330913));
#21080=CARTESIAN_POINT('Ctrl Pts',(8.59489616871569,-25.8867511126202,4.96226561664425));
#21081=CARTESIAN_POINT('Ctrl Pts',(11.4598615582757,-25.7117511126202,-2.06354052510241E-11));
#21082=CARTESIAN_POINT('Ctrl Pts',(8.59489616869782,-25.5367511126202,-4.9622656166752));
#21083=CARTESIAN_POINT('Ctrl Pts',(5.72993077911996,-25.3617511126202,-9.92453123332976));
#21084=CARTESIAN_POINT('Ctrl Pts',(-1.78726082715848E-11,-25.1867511126202,
-9.92453123331945));
#21085=CARTESIAN_POINT('Ctrl Pts',(-5.7299307791557,-25.0117511126202,-9.92453123330913));
#21086=CARTESIAN_POINT('Ctrl Pts',(-8.59489616871569,-24.8367511126202,
-4.96226561664425));
#21087=CARTESIAN_POINT('Ctrl Pts',(-11.4598615582757,-24.6617511126202,
2.06368086793017E-11));
#21088=CARTESIAN_POINT('Ctrl Pts',(-8.59489616869782,-24.4867511126202,
4.9622656166752));
#21089=CARTESIAN_POINT('Ctrl Pts',(-5.72993077911996,-24.3117511126202,
9.92453123332977));
#21090=CARTESIAN_POINT('Ctrl Pts',(1.7871392867044E-11,-24.1367511126202,
9.92453123331945));
#21091=CARTESIAN_POINT('Ctrl Pts',(5.7299307791557,-23.9617511126202,9.92453123330913));
#21092=CARTESIAN_POINT('Ctrl Pts',(8.59489616871569,-23.7867511126202,4.96226561664425));
#21093=CARTESIAN_POINT('Ctrl Pts',(11.4598615582757,-23.6117511126202,-2.06354052510241E-11));
#21094=CARTESIAN_POINT('Ctrl Pts',(8.59489616869782,-23.4367511126202,-4.9622656166752));
#21095=CARTESIAN_POINT('Ctrl Pts',(5.72993077911996,-23.2617511126202,-9.92453123332976));
#21096=CARTESIAN_POINT('Ctrl Pts',(-1.78726082715848E-11,-23.0867511126202,
-9.92453123331945));
#21097=CARTESIAN_POINT('Ctrl Pts',(-5.7299307791557,-22.9117511126202,-9.92453123330913));
#21098=CARTESIAN_POINT('Ctrl Pts',(-8.59489616871569,-22.7367511126202,
-4.96226561664425));
#21099=CARTESIAN_POINT('Ctrl Pts',(-11.4598615582757,-22.5617511126203,
2.06368086793017E-11));
#21100=CARTESIAN_POINT('Ctrl Pts',(-8.59489616869782,-22.3867511126202,
4.9622656166752));
#21101=CARTESIAN_POINT('Ctrl Pts',(-5.72993077911996,-22.2117511126202,
9.92453123332977));
#21102=CARTESIAN_POINT('Ctrl Pts',(1.7871392867044E-11,-22.0367511126202,
9.92453123331945));
#21103=CARTESIAN_POINT('Ctrl Pts',(5.7299307791557,-21.8617511126203,9.92453123330913));
#21104=CARTESIAN_POINT('Ctrl Pts',(8.59489616871569,-21.6867511126202,4.96226561664425));
#21105=CARTESIAN_POINT('Ctrl Pts',(11.4598615582757,-21.5117511126203,-2.06354052510241E-11));
#21106=CARTESIAN_POINT('Ctrl Pts',(8.59489616869782,-21.3367511126203,-4.9622656166752));
#21107=CARTESIAN_POINT('Ctrl Pts',(5.72993077911996,-21.1617511126202,-9.92453123332976));
#21108=CARTESIAN_POINT('Ctrl Pts',(-1.78726082715848E-11,-20.9867511126202,
-9.92453123331945));
#21109=CARTESIAN_POINT('Ctrl Pts',(-5.7299307791557,-20.8117511126203,-9.92453123330913));
#21110=CARTESIAN_POINT('Ctrl Pts',(-8.59489616871569,-20.6367511126202,
-4.96226561664425));
#21111=CARTESIAN_POINT('Ctrl Pts',(-11.4598615582757,-20.4617511126203,
2.06368086793017E-11));
#21112=CARTESIAN_POINT('Ctrl Pts',(-8.59489616869782,-20.2867511126202,
4.9622656166752));
#21113=CARTESIAN_POINT('Ctrl Pts',(-5.72993077911996,-20.1117511126202,
9.92453123332977));
#21114=CARTESIAN_POINT('Ctrl Pts',(1.7871392867044E-11,-19.9367511126203,
9.92453123331945));
#21115=CARTESIAN_POINT('Ctrl Pts',(5.7299307791557,-19.7617511126202,9.92453123330913));
#21116=CARTESIAN_POINT('Ctrl Pts',(8.59489616871569,-19.5867511126202,4.96226561664425));
#21117=CARTESIAN_POINT('Ctrl Pts',(11.4598615582757,-19.4117511126203,-2.06354052510241E-11));
#21118=CARTESIAN_POINT('Ctrl Pts',(8.59489616869782,-19.2367511126202,-4.9622656166752));
#21119=CARTESIAN_POINT('Ctrl Pts',(5.72993077911996,-19.0617511126203,-9.92453123332976));
#21120=CARTESIAN_POINT('Ctrl Pts',(-1.78726082715848E-11,-18.8867511126203,
-9.92453123331945));
#21121=CARTESIAN_POINT('Ctrl Pts',(-5.7299307791557,-18.7117511126203,-9.92453123330913));
#21122=CARTESIAN_POINT('Ctrl Pts',(-8.59489616871569,-18.5367511126203,
-4.96226561664425));
#21123=CARTESIAN_POINT('Ctrl Pts',(-11.4598615582757,-18.3617511126203,
2.06368086793017E-11));
#21124=CARTESIAN_POINT('Ctrl Pts',(-8.59489616869782,-18.1867511126202,
4.9622656166752));
#21125=CARTESIAN_POINT('Ctrl Pts',(-5.72993077911996,-18.0117511126203,
9.92453123332977));
#21126=CARTESIAN_POINT('Ctrl Pts',(1.7871392867044E-11,-17.8367511126202,
9.92453123331945));
#21127=CARTESIAN_POINT('Ctrl Pts',(5.7299307791557,-17.6617511126203,9.92453123330913));
#21128=CARTESIAN_POINT('Ctrl Pts',(8.59489616871569,-17.4867511126202,4.96226561664425));
#21129=CARTESIAN_POINT('Ctrl Pts',(11.4598615582757,-17.3117511126203,-2.06354052510241E-11));
#21130=CARTESIAN_POINT('Ctrl Pts',(8.59489616869782,-17.1367511126203,-4.9622656166752));
#21131=CARTESIAN_POINT('Ctrl Pts',(5.72993077911996,-16.9617511126202,-9.92453123332976));
#21132=CARTESIAN_POINT('Ctrl Pts',(-1.78726082715848E-11,-16.7867511126203,
-9.92453123331945));
#21133=CARTESIAN_POINT('Ctrl Pts',(-5.7299307791557,-16.6117511126203,-9.92453123330913));
#21134=CARTESIAN_POINT('Ctrl Pts',(-8.59489616871569,-16.4367511126202,
-4.96226561664425));
#21135=CARTESIAN_POINT('Ctrl Pts',(-11.4598615582757,-16.2617511126203,
2.06368086793017E-11));
#21136=CARTESIAN_POINT('Ctrl Pts',(-8.59489616869782,-16.0867511126203,
4.9622656166752));
#21137=CARTESIAN_POINT('Ctrl Pts',(-5.72993077911996,-15.9117511126202,
9.92453123332977));
#21138=CARTESIAN_POINT('Ctrl Pts',(1.7871392867044E-11,-15.7367511126203,
9.92453123331945));
#21139=CARTESIAN_POINT('Ctrl Pts',(5.7299307791557,-15.5617511126203,9.92453123330913));
#21140=CARTESIAN_POINT('Ctrl Pts',(8.59489616871569,-15.3867511126203,4.96226561664425));
#21141=CARTESIAN_POINT('Ctrl Pts',(11.4598615582757,-15.2117511126203,-2.06354052510241E-11));
#21142=CARTESIAN_POINT('Ctrl Pts',(8.59489616869782,-15.0367511126203,-4.9622656166752));
#21143=CARTESIAN_POINT('Ctrl Pts',(5.72993077911996,-14.8617511126203,-9.92453123332976));
#21144=CARTESIAN_POINT('Ctrl Pts',(-1.78726082715848E-11,-14.6867511126202,
-9.92453123331945));
#21145=CARTESIAN_POINT('Ctrl Pts',(-5.7299307791557,-14.5117511126203,-9.92453123330913));
#21146=CARTESIAN_POINT('Ctrl Pts',(-8.59489616871569,-14.3367511126203,
-4.96226561664425));
#21147=CARTESIAN_POINT('Ctrl Pts',(-11.4598615582757,-14.1617511126203,
2.06368086793017E-11));
#21148=CARTESIAN_POINT('Ctrl Pts',(-8.59489616869782,-13.9867511126203,
4.9622656166752));
#21149=CARTESIAN_POINT('Ctrl Pts',(-5.72993077911996,-13.8117511126203,
9.92453123332977));
#21150=CARTESIAN_POINT('Ctrl Pts',(1.7871392867044E-11,-13.6367511126203,
9.92453123331945));
#21151=CARTESIAN_POINT('Ctrl Pts',(5.7299307791557,-13.4617511126203,9.92453123330913));
#21152=CARTESIAN_POINT('Ctrl Pts',(8.59489616871569,-13.2867511126203,4.96226561664425));
#21153=CARTESIAN_POINT('Ctrl Pts',(11.4598615582757,-13.1117511126203,-2.06354052510241E-11));
#21154=CARTESIAN_POINT('Ctrl Pts',(8.59489616869782,-12.9367511126203,-4.9622656166752));
#21155=CARTESIAN_POINT('Ctrl Pts',(5.72993077911996,-12.7617511126203,-9.92453123332976));
#21156=CARTESIAN_POINT('Ctrl Pts',(-1.78726082715848E-11,-12.5867511126203,
-9.92453123331945));
#21157=CARTESIAN_POINT('Ctrl Pts',(-5.7299307791557,-12.4117511126203,-9.92453123330913));
#21158=CARTESIAN_POINT('Ctrl Pts',(-8.59489616871569,-12.2367511126203,
-4.96226561664425));
#21159=CARTESIAN_POINT('Ctrl Pts',(-11.4598615582757,-12.0617511126203,
2.06368086793017E-11));
#21160=CARTESIAN_POINT('Ctrl Pts',(-8.59489616869782,-11.8867511126203,
4.9622656166752));
#21161=CARTESIAN_POINT('Ctrl Pts',(-5.72993077911996,-11.7117511126203,
9.92453123332977));
#21162=CARTESIAN_POINT('Ctrl Pts',(1.7871392867044E-11,-11.5367511126203,
9.92453123331945));
#21163=CARTESIAN_POINT('Ctrl Pts',(5.7299307791557,-11.3617511126203,9.92453123330913));
#21164=CARTESIAN_POINT('Ctrl Pts',(8.59489616871569,-11.1867511126203,4.96226561664425));
#21165=CARTESIAN_POINT('Ctrl Pts',(11.4598615582757,-11.0117511126203,-2.06354052510241E-11));
#21166=CARTESIAN_POINT('Ctrl Pts',(8.59489616869782,-10.8367511126203,-4.9622656166752));
#21167=CARTESIAN_POINT('Ctrl Pts',(5.72993077911996,-10.6617511126203,-9.92453123332976));
#21168=CARTESIAN_POINT('Ctrl Pts',(-1.78726082715848E-11,-10.4867511126203,
-9.92453123331945));
#21169=CARTESIAN_POINT('Ctrl Pts',(-5.7299307791557,-10.3117511126203,-9.92453123330913));
#21170=CARTESIAN_POINT('Ctrl Pts',(-8.59489616871569,-10.1367511126203,
-4.96226561664425));
#21171=CARTESIAN_POINT('Ctrl Pts',(-11.4598615582757,-9.96175111262027,
2.06368086793017E-11));
#21172=CARTESIAN_POINT('Ctrl Pts',(-8.59489616869782,-9.78675111262026,
4.9622656166752));
#21173=CARTESIAN_POINT('Ctrl Pts',(-5.72993077911996,-9.61175111262028,
9.92453123332977));
#21174=CARTESIAN_POINT('Ctrl Pts',(1.7871392867044E-11,-9.43675111262027,
9.92453123331945));
#21175=CARTESIAN_POINT('Ctrl Pts',(5.7299307791557,-9.26175111262026,9.92453123330913));
#21176=CARTESIAN_POINT('Ctrl Pts',(8.59489616871569,-9.08675111262028,4.96226561664425));
#21177=CARTESIAN_POINT('Ctrl Pts',(11.4598615582757,-8.91175111262028,-2.06354052510241E-11));
#21178=CARTESIAN_POINT('Ctrl Pts',(8.59489616869782,-8.73675111262026,-4.9622656166752));
#21179=CARTESIAN_POINT('Ctrl Pts',(5.72993077911996,-8.56175111262028,-9.92453123332976));
#21180=CARTESIAN_POINT('Ctrl Pts',(-1.78726082715848E-11,-8.38675111262027,
-9.92453123331945));
#21181=CARTESIAN_POINT('Ctrl Pts',(-5.7299307791557,-8.21175111262026,-9.92453123330913));
#21182=CARTESIAN_POINT('Ctrl Pts',(-8.59489616871569,-8.03675111262028,
-4.96226561664425));
#21183=CARTESIAN_POINT('Ctrl Pts',(-11.4598615582757,-7.86175111262028,
2.06368086793017E-11));
#21184=CARTESIAN_POINT('Ctrl Pts',(-8.59489616869782,-7.68675111262027,
4.9622656166752));
#21185=CARTESIAN_POINT('Ctrl Pts',(-5.72993077911996,-7.51175111262028,
9.92453123332977));
#21186=CARTESIAN_POINT('Ctrl Pts',(1.7871392867044E-11,-7.33675111262028,
9.92453123331945));
#21187=CARTESIAN_POINT('Ctrl Pts',(5.7299307791557,-7.16175111262027,9.92453123330913));
#21188=CARTESIAN_POINT('Ctrl Pts',(8.59489616871569,-6.98675111262029,4.96226561664425));
#21189=CARTESIAN_POINT('Ctrl Pts',(11.4598615582757,-6.81175111262029,-2.06354052510241E-11));
#21190=CARTESIAN_POINT('Ctrl Pts',(8.59489616869782,-6.63675111262027,-4.9622656166752));
#21191=CARTESIAN_POINT('Ctrl Pts',(5.72993077911996,-6.46175111262029,-9.92453123332976));
#21192=CARTESIAN_POINT('Ctrl Pts',(-1.78726082715848E-11,-6.28675111262028,
-9.92453123331945));
#21193=CARTESIAN_POINT('Ctrl Pts',(-5.7299307791557,-6.11175111262027,-9.92453123330913));
#21194=CARTESIAN_POINT('Ctrl Pts',(-8.59489616871569,-5.93675111262026,
-4.96226561664425));
#21195=CARTESIAN_POINT('Ctrl Pts',(-11.4598615582757,-5.76175111262029,
2.06368086793017E-11));
#21196=CARTESIAN_POINT('Ctrl Pts',(-8.59489616869782,-5.58675111262028,
4.9622656166752));
#21197=CARTESIAN_POINT('Ctrl Pts',(-5.72993077911996,-5.41175111262028,
9.92453123332977));
#21198=CARTESIAN_POINT('Ctrl Pts',(1.7871392867044E-11,-5.23675111262029,
9.92453123331945));
#21199=CARTESIAN_POINT('Ctrl Pts',(5.7299307791557,-5.06175111262028,9.92453123330913));
#21200=CARTESIAN_POINT('Ctrl Pts',(8.59489616871569,-4.88675111262027,4.96226561664425));
#21201=CARTESIAN_POINT('Ctrl Pts',(11.4598615582757,-4.7117511126203,-2.06354052510241E-11));
#21202=CARTESIAN_POINT('Ctrl Pts',(8.59489616869782,-4.53675111262028,-4.9622656166752));
#21203=CARTESIAN_POINT('Ctrl Pts',(5.72993077911996,-4.36175111262028,-9.92453123332976));
#21204=CARTESIAN_POINT('Ctrl Pts',(-1.78726082715848E-11,-4.18675111262029,
-9.92453123331945));
#21205=CARTESIAN_POINT('Ctrl Pts',(-5.7299307791557,-4.01175111262028,-9.92453123330913));
#21206=CARTESIAN_POINT('Ctrl Pts',(-8.59489616871569,-3.83675111262027,
-4.96226561664425));
#21207=CARTESIAN_POINT('Ctrl Pts',(-11.4598615582757,-3.6617511126203,2.06368086793017E-11));
#21208=CARTESIAN_POINT('Ctrl Pts',(-8.59489616869782,-3.48675111262029,
4.9622656166752));
#21209=CARTESIAN_POINT('Ctrl Pts',(-5.72993077911996,-3.31175111262029,
9.92453123332977));
#21210=CARTESIAN_POINT('Ctrl Pts',(1.7871392867044E-11,-3.1367511126203,
9.92453123331945));
#21211=CARTESIAN_POINT('Ctrl Pts',(5.7299307791557,-2.96175111262029,9.92453123330913));
#21212=CARTESIAN_POINT('Ctrl Pts',(8.59489616871569,-2.78675111262028,4.96226561664425));
#21213=CARTESIAN_POINT('Ctrl Pts',(11.4598615582757,-2.61175111262031,-2.06354052510241E-11));
#21214=CARTESIAN_POINT('Ctrl Pts',(8.59489616869782,-2.43675111262029,-4.9622656166752));
#21215=CARTESIAN_POINT('Ctrl Pts',(5.72993077911996,-2.26175111262028,-9.92453123332976));
#21216=CARTESIAN_POINT('Ctrl Pts',(-1.78726082715848E-11,-2.0867511126203,
-9.92453123331945));
#21217=CARTESIAN_POINT('Ctrl Pts',(-5.7299307791557,-1.91175111262029,-9.92453123330913));
#21218=CARTESIAN_POINT('Ctrl Pts',(-8.59489616871569,-1.73675111262028,
-4.96226561664425));
#21219=CARTESIAN_POINT('Ctrl Pts',(-11.4598615582757,-1.56175111262028,
2.06368086793017E-11));
#21220=CARTESIAN_POINT('Ctrl Pts',(-8.59489616869782,-1.38675111262029,
4.9622656166752));
#21221=CARTESIAN_POINT('Ctrl Pts',(-5.72993077911996,-1.21175111262029,
9.92453123332977));
#21222=CARTESIAN_POINT('Ctrl Pts',(1.7871392867044E-11,-1.03675111262028,
9.92453123331945));
#21223=CARTESIAN_POINT('Ctrl Pts',(5.7299307791557,-0.861751112620297,9.92453123330913));
#21224=CARTESIAN_POINT('Ctrl Pts',(8.59489616871569,-0.686751112620287,
4.96226561664425));
#21225=CARTESIAN_POINT('Ctrl Pts',(11.4598615582757,-0.511751112620282,
-2.06354052510241E-11));
#21226=CARTESIAN_POINT('Ctrl Pts',(8.59489616869782,-0.336751112620298,
-4.9622656166752));
#21227=CARTESIAN_POINT('Ctrl Pts',(5.72993077911996,-0.161751112620292,
-9.92453123332976));
#21228=CARTESIAN_POINT('Ctrl Pts',(-1.78726082715848E-11,0.0132488873797187,
-9.92453123331945));
#21229=CARTESIAN_POINT('Ctrl Pts',(-5.7299307791557,0.188248887379698,-9.92453123330913));
#21230=CARTESIAN_POINT('Ctrl Pts',(-8.59489616871569,0.363248887379708,
-4.96226561664425));
#21231=CARTESIAN_POINT('Ctrl Pts',(-11.4598615582757,0.538248887379713,
2.06368086793017E-11));
#21232=CARTESIAN_POINT('Ctrl Pts',(-8.59489616869782,0.713248887379697,
4.9622656166752));
#21233=CARTESIAN_POINT('Ctrl Pts',(-5.72993077911996,0.888248887379703,
9.92453123332977));
#21234=CARTESIAN_POINT('Ctrl Pts',(1.7871392867044E-11,1.06324888737971,
9.92453123331945));
#21235=CARTESIAN_POINT('Ctrl Pts',(5.7299307791557,1.23824888737969,9.92453123330913));
#21236=CARTESIAN_POINT('Ctrl Pts',(8.59489616871569,1.4132488873797,4.96226561664425));
#21237=CARTESIAN_POINT('Ctrl Pts',(11.4598615582757,1.58824888737971,-2.06354052510241E-11));
#21238=CARTESIAN_POINT('Ctrl Pts',(8.59489616869782,1.76324888737969,-4.9622656166752));
#21239=CARTESIAN_POINT('Ctrl Pts',(5.72993077911996,1.9382488873797,-9.92453123332976));
#21240=CARTESIAN_POINT('Ctrl Pts',(-1.78726082715848E-11,2.11324888737971,
-9.92453123331945));
#21241=CARTESIAN_POINT('Ctrl Pts',(-5.7299307791557,2.28824888737969,-9.92453123330913));
#21242=CARTESIAN_POINT('Ctrl Pts',(-8.59489616871569,2.4632488873797,-4.96226561664425));
#21243=CARTESIAN_POINT('Ctrl Pts',(-11.4598615582757,2.6382488873797,2.06368086793017E-11));
#21244=CARTESIAN_POINT('Ctrl Pts',(-8.59489616869782,2.81324888737972,4.9622656166752));
#21245=CARTESIAN_POINT('Ctrl Pts',(-5.72993077911996,2.98824888737969,9.92453123332977));
#21246=CARTESIAN_POINT('Ctrl Pts',(1.7871392867044E-11,3.16324888737971,
9.92453123331945));
#21247=CARTESIAN_POINT('Ctrl Pts',(5.7299307791557,3.33824888737971,9.92453123330913));
#21248=CARTESIAN_POINT('Ctrl Pts',(8.59489616871569,3.51324888737969,4.96226561664425));
#21249=CARTESIAN_POINT('Ctrl Pts',(11.4598615582757,3.6882488873797,-2.06354052510241E-11));
#21250=CARTESIAN_POINT('Ctrl Pts',(8.59489616869782,3.86324888737971,-4.9622656166752));
#21251=CARTESIAN_POINT('Ctrl Pts',(5.72993077911996,4.03824888737969,-9.92453123332976));
#21252=CARTESIAN_POINT('Ctrl Pts',(-1.78726082715848E-11,4.2132488873797,
-9.92453123331945));
#21253=CARTESIAN_POINT('Ctrl Pts',(-5.7299307791557,4.3882488873797,-9.92453123330913));
#21254=CARTESIAN_POINT('Ctrl Pts',(-8.59489616871569,4.56324888737969,-4.96226561664425));
#21255=CARTESIAN_POINT('Ctrl Pts',(-11.4598615582757,4.73824888737969,2.06368086793017E-11));
#21256=CARTESIAN_POINT('Ctrl Pts',(-8.59489616869782,4.91324888737971,4.9622656166752));
#21257=CARTESIAN_POINT('Ctrl Pts',(-5.72993077911996,5.08824888737969,9.92453123332977));
#21258=CARTESIAN_POINT('Ctrl Pts',(1.7871392867044E-11,5.2632488873797,
9.92453123331945));
#21259=CARTESIAN_POINT('Ctrl Pts',(5.7299307791557,5.4382488873797,9.92453123330913));
#21260=CARTESIAN_POINT('Ctrl Pts',(8.59489616871569,5.61324888737968,4.96226561664425));
#21261=CARTESIAN_POINT('Ctrl Pts',(11.4598615582757,5.78824888737969,-2.06354052510241E-11));
#21262=CARTESIAN_POINT('Ctrl Pts',(8.59489616869782,5.9632488873797,-4.9622656166752));
#21263=CARTESIAN_POINT('Ctrl Pts',(5.72993077911996,6.13824888737968,-9.92453123332976));
#21264=CARTESIAN_POINT('Ctrl Pts',(-1.78726082715848E-11,6.31324888737969,
-9.92453123331945));
#21265=CARTESIAN_POINT('Ctrl Pts',(-5.7299307791557,6.4882488873797,-9.92453123330913));
#21266=CARTESIAN_POINT('Ctrl Pts',(-8.59489616871569,6.66324888737968,-4.96226561664425));
#21267=CARTESIAN_POINT('Ctrl Pts',(-11.4598615582757,6.83824888737969,2.06368086793017E-11));
#21268=CARTESIAN_POINT('Ctrl Pts',(-8.59489616869782,7.0132488873797,4.9622656166752));
#21269=CARTESIAN_POINT('Ctrl Pts',(-5.72993077911996,7.18824888737968,9.92453123332977));
#21270=CARTESIAN_POINT('Ctrl Pts',(1.7871392867044E-11,7.36324888737969,
9.92453123331945));
#21271=CARTESIAN_POINT('Ctrl Pts',(5.7299307791557,7.53824888737969,9.92453123330913));
#21272=CARTESIAN_POINT('Ctrl Pts',(8.59489616871569,7.7132488873797,4.96226561664425));
#21273=CARTESIAN_POINT('Ctrl Pts',(11.4598615582757,7.88824888737968,-2.06354052510241E-11));
#21274=CARTESIAN_POINT('Ctrl Pts',(8.59489616869782,8.06324888737969,-4.9622656166752));
#21275=CARTESIAN_POINT('Ctrl Pts',(5.72993077911996,8.2382488873797,-9.92453123332976));
#21276=CARTESIAN_POINT('Ctrl Pts',(-1.78726082715848E-11,8.41324888737968,
-9.92453123331945));
#21277=CARTESIAN_POINT('Ctrl Pts',(-5.7299307791557,8.58824888737968,-9.92453123330913));
#21278=CARTESIAN_POINT('Ctrl Pts',(-8.59489616871569,8.7632488873797,-4.96226561664425));
#21279=CARTESIAN_POINT('Ctrl Pts',(-11.4598615582757,8.93824888737968,2.06368086793017E-11));
#21280=CARTESIAN_POINT('Ctrl Pts',(-8.59489616869782,9.11324888737969,4.9622656166752));
#21281=CARTESIAN_POINT('Ctrl Pts',(-5.72993077911996,9.28824888737969,9.92453123332977));
#21282=CARTESIAN_POINT('Ctrl Pts',(1.7871392867044E-11,9.46324888737968,
9.92453123331945));
#21283=CARTESIAN_POINT('Ctrl Pts',(5.7299307791557,9.63824888737968,9.92453123330913));
#21284=CARTESIAN_POINT('Ctrl Pts',(8.59489616871569,9.81324888737969,4.96226561664425));
#21285=CARTESIAN_POINT('Ctrl Pts',(11.4598615582757,9.98824888737967,-2.06354052510241E-11));
#21286=CARTESIAN_POINT('Ctrl Pts',(8.59489616869782,10.1632488873797,-4.9622656166752));
#21287=CARTESIAN_POINT('Ctrl Pts',(5.72993077911996,10.3382488873797,-9.92453123332976));
#21288=CARTESIAN_POINT('Ctrl Pts',(-1.78726082715848E-11,10.5132488873797,
-9.92453123331945));
#21289=CARTESIAN_POINT('Ctrl Pts',(-5.7299307791557,10.6882488873797,-9.92453123330913));
#21290=CARTESIAN_POINT('Ctrl Pts',(-8.59489616871569,10.8632488873797,-4.96226561664425));
#21291=CARTESIAN_POINT('Ctrl Pts',(-11.4598615582757,11.0382488873797,2.06368086793017E-11));
#21292=CARTESIAN_POINT('Ctrl Pts',(-8.59489616869782,11.2132488873797,4.9622656166752));
#21293=CARTESIAN_POINT('Ctrl Pts',(-5.72993077911996,11.3882488873797,9.92453123332977));
#21294=CARTESIAN_POINT('Ctrl Pts',(1.7871392867044E-11,11.5632488873797,
9.92453123331945));
#21295=CARTESIAN_POINT('Ctrl Pts',(5.7299307791557,11.7382488873797,9.92453123330913));
#21296=CARTESIAN_POINT('Ctrl Pts',(8.59489616871569,11.9132488873797,4.96226561664425));
#21297=CARTESIAN_POINT('Ctrl Pts',(11.4598615582757,12.0882488873797,-2.06354052510241E-11));
#21298=CARTESIAN_POINT('Ctrl Pts',(8.59489616869782,12.2632488873797,-4.9622656166752));
#21299=CARTESIAN_POINT('Ctrl Pts',(5.72993077911996,12.4382488873797,-9.92453123332976));
#21300=CARTESIAN_POINT('Ctrl Pts',(-1.78726082715848E-11,12.6132488873797,
-9.92453123331945));
#21301=CARTESIAN_POINT('Ctrl Pts',(-5.7299307791557,12.7882488873797,-9.92453123330913));
#21302=CARTESIAN_POINT('Ctrl Pts',(-8.59489616871569,12.9632488873797,-4.96226561664425));
#21303=CARTESIAN_POINT('Ctrl Pts',(-11.4598615582757,13.1382488873797,2.06368086793017E-11));
#21304=CARTESIAN_POINT('Ctrl Pts',(-8.59489616869782,13.3132488873797,4.9622656166752));
#21305=CARTESIAN_POINT('Ctrl Pts',(-5.72993077911996,13.4882488873797,9.92453123332977));
#21306=CARTESIAN_POINT('Ctrl Pts',(1.7871392867044E-11,13.6632488873797,
9.92453123331945));
#21307=CARTESIAN_POINT('Ctrl Pts',(5.7299307791557,13.8382488873797,9.92453123330913));
#21308=CARTESIAN_POINT('Ctrl Pts',(8.59489616871569,14.0132488873797,4.96226561664425));
#21309=CARTESIAN_POINT('Ctrl Pts',(11.4598615582757,14.1882488873797,-2.06354052510241E-11));
#21310=CARTESIAN_POINT('Ctrl Pts',(8.59489616869782,14.3632488873797,-4.9622656166752));
#21311=CARTESIAN_POINT('Ctrl Pts',(5.72993077911996,14.5382488873797,-9.92453123332976));
#21312=CARTESIAN_POINT('Ctrl Pts',(-1.78726082715848E-11,14.7132488873797,
-9.92453123331945));
#21313=CARTESIAN_POINT('Ctrl Pts',(-5.7299307791557,14.8882488873797,-9.92453123330913));
#21314=CARTESIAN_POINT('Ctrl Pts',(-8.59489616871569,15.0632488873797,-4.96226561664425));
#21315=CARTESIAN_POINT('Ctrl Pts',(-11.4598615582757,15.2382488873797,2.06368086793017E-11));
#21316=CARTESIAN_POINT('Ctrl Pts',(-8.59489616869782,15.4132488873797,4.9622656166752));
#21317=CARTESIAN_POINT('Ctrl Pts',(-5.72993077911996,15.5882488873797,9.92453123332977));
#21318=CARTESIAN_POINT('Ctrl Pts',(1.7871392867044E-11,15.7632488873797,
9.92453123331945));
#21319=CARTESIAN_POINT('Ctrl Pts',(5.7299307791557,15.9382488873797,9.92453123330913));
#21320=CARTESIAN_POINT('Ctrl Pts',(8.59489616871569,16.1132488873797,4.96226561664425));
#21321=CARTESIAN_POINT('Ctrl Pts',(11.4598615582757,16.2882488873797,-2.06354052510241E-11));
#21322=CARTESIAN_POINT('Ctrl Pts',(8.59489616869782,16.4632488873797,-4.9622656166752));
#21323=CARTESIAN_POINT('Ctrl Pts',(5.72993077911996,16.6382488873797,-9.92453123332976));
#21324=CARTESIAN_POINT('Ctrl Pts',(-1.78726082715848E-11,16.8132488873797,
-9.92453123331945));
#21325=CARTESIAN_POINT('Ctrl Pts',(-5.7299307791557,16.9882488873797,-9.92453123330913));
#21326=CARTESIAN_POINT('Ctrl Pts',(-8.59489616871569,17.1632488873797,-4.96226561664425));
#21327=CARTESIAN_POINT('Ctrl Pts',(-11.4598615582757,17.3382488873797,2.06368086793017E-11));
#21328=CARTESIAN_POINT('Ctrl Pts',(-8.59489616869782,17.5132488873797,4.9622656166752));
#21329=CARTESIAN_POINT('Ctrl Pts',(-5.72993077911996,17.6882488873797,9.92453123332977));
#21330=CARTESIAN_POINT('Ctrl Pts',(1.7871392867044E-11,17.8632488873797,
9.92453123331945));
#21331=CARTESIAN_POINT('Ctrl Pts',(5.7299307791557,18.0382488873797,9.92453123330913));
#21332=CARTESIAN_POINT('Ctrl Pts',(8.59489616871569,18.2132488873797,4.96226561664425));
#21333=CARTESIAN_POINT('Ctrl Pts',(11.4598615582757,18.3882488873797,-2.06354052510241E-11));
#21334=CARTESIAN_POINT('Ctrl Pts',(8.59489616869782,18.5632488873797,-4.9622656166752));
#21335=CARTESIAN_POINT('Ctrl Pts',(5.72993077911996,18.7382488873796,-9.92453123332976));
#21336=CARTESIAN_POINT('Ctrl Pts',(-1.78726082715848E-11,18.9132488873797,
-9.92453123331945));
#21337=CARTESIAN_POINT('Ctrl Pts',(-5.7299307791557,19.0882488873797,-9.92453123330913));
#21338=CARTESIAN_POINT('Ctrl Pts',(-8.59489616871569,19.2632488873797,-4.96226561664425));
#21339=CARTESIAN_POINT('Ctrl Pts',(-11.4598615582757,19.4382488873797,2.06368086793017E-11));
#21340=CARTESIAN_POINT('Ctrl Pts',(-8.59489616869782,19.6132488873797,4.9622656166752));
#21341=CARTESIAN_POINT('Ctrl Pts',(-5.72993077911996,19.7882488873796,9.92453123332977));
#21342=CARTESIAN_POINT('Ctrl Pts',(1.7871392867044E-11,19.9632488873797,
9.92453123331945));
#21343=CARTESIAN_POINT('Ctrl Pts',(5.7299307791557,20.1382488873797,9.92453123330913));
#21344=CARTESIAN_POINT('Ctrl Pts',(8.59489616871569,20.3132488873796,4.96226561664425));
#21345=CARTESIAN_POINT('Ctrl Pts',(11.4598615582757,20.4882488873796,-2.06354052510241E-11));
#21346=CARTESIAN_POINT('Ctrl Pts',(8.59489616869782,20.6632488873797,-4.9622656166752));
#21347=CARTESIAN_POINT('Ctrl Pts',(5.72993077911996,20.8382488873797,-9.92453123332976));
#21348=CARTESIAN_POINT('Ctrl Pts',(-1.78726082715848E-11,21.0132488873797,
-9.92453123331945));
#21349=CARTESIAN_POINT('Ctrl Pts',(-5.7299307791557,21.1882488873797,-9.92453123330913));
#21350=CARTESIAN_POINT('Ctrl Pts',(-8.59489616871569,21.3632488873797,-4.96226561664425));
#21351=CARTESIAN_POINT('Ctrl Pts',(-11.4598615582757,21.5382488873796,2.06368086793017E-11));
#21352=CARTESIAN_POINT('Ctrl Pts',(-8.59489616869782,21.7132488873797,4.9622656166752));
#21353=CARTESIAN_POINT('Ctrl Pts',(-5.72993077911996,21.8882488873797,9.92453123332977));
#21354=CARTESIAN_POINT('Ctrl Pts',(1.7871392867044E-11,22.0632488873797,
9.92453123331945));
#21355=CARTESIAN_POINT('Ctrl Pts',(5.7299307791557,22.2382488873797,9.92453123330913));
#21356=CARTESIAN_POINT('Ctrl Pts',(8.59489616871569,22.4132488873797,4.96226561664425));
#21357=CARTESIAN_POINT('Ctrl Pts',(11.4598615582757,22.5882488873796,-2.06354052510241E-11));
#21358=CARTESIAN_POINT('Ctrl Pts',(8.59489616869782,22.7632488873797,-4.9622656166752));
#21359=CARTESIAN_POINT('Ctrl Pts',(5.72993077911996,22.9382488873797,-9.92453123332976));
#21360=CARTESIAN_POINT('Ctrl Pts',(-1.78726082715848E-11,23.1132488873796,
-9.92453123331945));
#21361=CARTESIAN_POINT('Ctrl Pts',(-5.7299307791557,23.2882488873797,-9.92453123330913));
#21362=CARTESIAN_POINT('Ctrl Pts',(-8.59489616871569,23.4632488873797,-4.96226561664425));
#21363=CARTESIAN_POINT('Ctrl Pts',(-11.4598615582757,23.6382488873796,2.06368086793017E-11));
#21364=CARTESIAN_POINT('Ctrl Pts',(-8.59489616869782,23.8132488873797,4.9622656166752));
#21365=CARTESIAN_POINT('Ctrl Pts',(-5.72993077911996,23.9882488873797,9.92453123332977));
#21366=CARTESIAN_POINT('Ctrl Pts',(1.7871392867044E-11,24.1632488873796,
9.92453123331945));
#21367=CARTESIAN_POINT('Ctrl Pts',(5.7299307791557,24.3382488873796,9.92453123330913));
#21368=CARTESIAN_POINT('Ctrl Pts',(8.59489616871569,24.5132488873797,4.96226561664425));
#21369=CARTESIAN_POINT('Ctrl Pts',(11.4598615582757,24.6882488873796,-2.06354052510241E-11));
#21370=CARTESIAN_POINT('Ctrl Pts',(8.59489616869782,24.8632488873796,-4.9622656166752));
#21371=CARTESIAN_POINT('Ctrl Pts',(5.72993077911996,25.0382488873797,-9.92453123332976));
#21372=CARTESIAN_POINT('Ctrl Pts',(-1.78726082715848E-11,25.2132488873796,
-9.92453123331945));
#21373=CARTESIAN_POINT('Ctrl Pts',(-5.7299307791557,25.3882488873796,-9.92453123330913));
#21374=CARTESIAN_POINT('Ctrl Pts',(-8.59489616871569,25.5632488873797,-4.96226561664425));
#21375=CARTESIAN_POINT('Ctrl Pts',(-11.4598615582757,25.7382488873797,2.06368086793017E-11));
#21376=CARTESIAN_POINT('Ctrl Pts',(-8.59489616869782,25.9132488873796,4.9622656166752));
#21377=CARTESIAN_POINT('Ctrl Pts',(-5.72993077911996,26.0882488873797,9.92453123332977));
#21378=CARTESIAN_POINT('Ctrl Pts',(1.7871392867044E-11,26.2632488873797,
9.92453123331945));
#21379=CARTESIAN_POINT('Ctrl Pts',(5.7299307791557,26.4382488873796,9.92453123330913));
#21380=CARTESIAN_POINT('Ctrl Pts',(8.59489616871569,26.6132488873797,4.96226561664425));
#21381=CARTESIAN_POINT('Ctrl Pts',(11.4598615582757,26.7882488873797,-2.06354052510241E-11));
#21382=CARTESIAN_POINT('Ctrl Pts',(8.59489616869782,26.9632488873796,-4.9622656166752));
#21383=CARTESIAN_POINT('Ctrl Pts',(5.72993077911996,27.1382488873796,-9.92453123332976));
#21384=CARTESIAN_POINT('Ctrl Pts',(-1.78726082715848E-11,27.3132488873797,
-9.92453123331945));
#21385=CARTESIAN_POINT('Ctrl Pts',(-1.22646583495775,-24.9756402675196,
8.31163887211714));
#21386=CARTESIAN_POINT('Ctrl Pts',(-0.616535190940158,-24.9517609250221,
8.40164026752071));
#21387=CARTESIAN_POINT('Ctrl Pts',(1.49242955500311E-11,-24.9295179709985,
8.40164026751963));
#21388=CARTESIAN_POINT('Ctrl Pts',(4.85068927010145,-24.7545179709985,8.40164026751121));
#21389=CARTESIAN_POINT('Ctrl Pts',(7.27603390513766,-24.5795179709986,4.20082013374705));
#21390=CARTESIAN_POINT('Ctrl Pts',(9.70137854017372,-24.4045179709986,-1.71807987380788E-11));
#21391=CARTESIAN_POINT('Ctrl Pts',(7.27603390512277,-24.2295179709986,-4.20082013377283));
#21392=CARTESIAN_POINT('Ctrl Pts',(4.85068927007217,-24.0545179709986,-8.40164026752811));
#21393=CARTESIAN_POINT('Ctrl Pts',(-1.48337207789367E-11,-23.8795179709986,
-8.40164026751963));
#21394=CARTESIAN_POINT('Ctrl Pts',(-4.85068927010184,-23.7045179709986,
-8.40164026751098));
#21395=CARTESIAN_POINT('Ctrl Pts',(-7.27603390513761,-23.5295179709985,
-4.20082013374713));
#21396=CARTESIAN_POINT('Ctrl Pts',(-9.70137854017372,-23.3545179709986,
1.70762120011325E-11));
#21397=CARTESIAN_POINT('Ctrl Pts',(-7.27603390512282,-23.1795179709986,
4.20082013377275));
#21398=CARTESIAN_POINT('Ctrl Pts',(-4.85068927007226,-23.0045179709986,
8.40164026752806));
#21399=CARTESIAN_POINT('Ctrl Pts',(1.47431460078422E-11,-22.8295179709986,
8.40164026751963));
#21400=CARTESIAN_POINT('Ctrl Pts',(4.85068927010175,-22.6545179709986,8.40164026751103));
#21401=CARTESIAN_POINT('Ctrl Pts',(7.2760339051378,-22.4795179709986,4.2008201337468));
#21402=CARTESIAN_POINT('Ctrl Pts',(9.70137854017372,-22.3045179709986,-1.69716252641861E-11));
#21403=CARTESIAN_POINT('Ctrl Pts',(7.27603390512287,-22.1295179709986,-4.20082013377267));
#21404=CARTESIAN_POINT('Ctrl Pts',(4.85068927007187,-21.9545179709986,-8.40164026752828));
#21405=CARTESIAN_POINT('Ctrl Pts',(-1.46525712367478E-11,-21.7795179709986,
-8.40164026751963));
#21406=CARTESIAN_POINT('Ctrl Pts',(-4.85068927010165,-21.6045179709986,
-8.40164026751109));
#21407=CARTESIAN_POINT('Ctrl Pts',(-7.27603390513776,-21.4295179709986,
-4.20082013374688));
#21408=CARTESIAN_POINT('Ctrl Pts',(-9.70137854017372,-21.2545179709986,
1.68670385272398E-11));
#21409=CARTESIAN_POINT('Ctrl Pts',(-7.27603390512291,-21.0795179709986,
4.20082013377259));
#21410=CARTESIAN_POINT('Ctrl Pts',(-4.85068927007196,-20.9045179709986,
8.40164026752823));
#21411=CARTESIAN_POINT('Ctrl Pts',(1.45619964656533E-11,-20.7295179709986,
8.40164026751963));
#21412=CARTESIAN_POINT('Ctrl Pts',(4.85068927010157,-20.5545179709986,8.40164026751114));
#21413=CARTESIAN_POINT('Ctrl Pts',(7.27603390513771,-20.3795179709986,4.20082013374695));
#21414=CARTESIAN_POINT('Ctrl Pts',(9.70137854017372,-20.2045179709986,-1.73139113141798E-11));
#21415=CARTESIAN_POINT('Ctrl Pts',(7.27603390512296,-20.0295179709986,-4.20082013377251));
#21416=CARTESIAN_POINT('Ctrl Pts',(4.85068927007205,-19.8545179709986,-8.40164026752818));
#21417=CARTESIAN_POINT('Ctrl Pts',(-1.49489996514033E-11,-19.6795179709986,
-8.40164026751963));
#21418=CARTESIAN_POINT('Ctrl Pts',(-4.85068927010147,-19.5045179709986,
-8.40164026751119));
#21419=CARTESIAN_POINT('Ctrl Pts',(-7.27603390513767,-19.3295179709986,
-4.20082013374703));
#21420=CARTESIAN_POINT('Ctrl Pts',(-9.70137854017372,-19.1545179709986,
1.72093245772335E-11));
#21421=CARTESIAN_POINT('Ctrl Pts',(-7.276033905123,-18.9795179709986,4.20082013377243));
#21422=CARTESIAN_POINT('Ctrl Pts',(-4.85068927007214,-18.8045179709986,
8.40164026752813));
#21423=CARTESIAN_POINT('Ctrl Pts',(1.48584248803088E-11,-18.6295179709986,
8.40164026751963));
#21424=CARTESIAN_POINT('Ctrl Pts',(4.85068927010186,-18.4545179709986,8.40164026751097));
#21425=CARTESIAN_POINT('Ctrl Pts',(7.27603390513762,-18.2795179709986,4.20082013374711));
#21426=CARTESIAN_POINT('Ctrl Pts',(9.70137854017372,-18.1045179709986,-1.71047378402871E-11));
#21427=CARTESIAN_POINT('Ctrl Pts',(7.27603390512281,-17.9295179709986,-4.20082013377277));
#21428=CARTESIAN_POINT('Ctrl Pts',(4.85068927007223,-17.7545179709986,-8.40164026752807));
#21429=CARTESIAN_POINT('Ctrl Pts',(-1.47678501092144E-11,-17.5795179709986,
-8.40164026751963));
#21430=CARTESIAN_POINT('Ctrl Pts',(-4.85068927010177,-17.4045179709986,
-8.40164026751102));
#21431=CARTESIAN_POINT('Ctrl Pts',(-7.27603390513758,-17.2295179709986,
-4.20082013374719));
#21432=CARTESIAN_POINT('Ctrl Pts',(-9.70137854017372,-17.0545179709986,
1.70001511033408E-11));
#21433=CARTESIAN_POINT('Ctrl Pts',(-7.27603390512285,-16.8795179709986,
4.20082013377269));
#21434=CARTESIAN_POINT('Ctrl Pts',(-4.85068927007185,-16.7045179709986,
8.4016402675283));
#21435=CARTESIAN_POINT('Ctrl Pts',(1.46772753381199E-11,-16.5295179709986,
8.40164026751963));
#21436=CARTESIAN_POINT('Ctrl Pts',(4.85068927010168,-16.3545179709986,8.40164026751107));
#21437=CARTESIAN_POINT('Ctrl Pts',(7.27603390513777,-16.1795179709986,4.20082013374685));
#21438=CARTESIAN_POINT('Ctrl Pts',(9.70137854017372,-16.0045179709986,-1.68955643663944E-11));
#21439=CARTESIAN_POINT('Ctrl Pts',(7.2760339051229,-15.8295179709986,-4.20082013377261));
#21440=CARTESIAN_POINT('Ctrl Pts',(4.85068927007194,-15.6545179709986,-8.40164026752825));
#21441=CARTESIAN_POINT('Ctrl Pts',(-1.45867005670255E-11,-15.4795179709986,
-8.40164026751963));
#21442=CARTESIAN_POINT('Ctrl Pts',(-4.85068927010159,-15.3045179709986,
-8.40164026751112));
#21443=CARTESIAN_POINT('Ctrl Pts',(-7.27603390513773,-15.1295179709986,
-4.20082013374693));
#21444=CARTESIAN_POINT('Ctrl Pts',(-9.70137854017372,-14.9545179709986,
1.67909776294481E-11));
#21445=CARTESIAN_POINT('Ctrl Pts',(-7.27603390512294,-14.7795179709986,
4.20082013377253));
#21446=CARTESIAN_POINT('Ctrl Pts',(-4.85068927007203,-14.6045179709986,
8.40164026752819));
#21447=CARTESIAN_POINT('Ctrl Pts',(1.49737037527755E-11,-14.4295179709986,
8.40164026751963));
#21448=CARTESIAN_POINT('Ctrl Pts',(4.8506892701015,-14.2545179709986,8.40164026751117));
#21449=CARTESIAN_POINT('Ctrl Pts',(7.27603390513768,-14.0795179709986,4.20082013374701));
#21450=CARTESIAN_POINT('Ctrl Pts',(9.70137854017372,-13.9045179709986,-1.72378504163881E-11));
#21451=CARTESIAN_POINT('Ctrl Pts',(7.27603390512299,-13.7295179709986,-4.20082013377245));
#21452=CARTESIAN_POINT('Ctrl Pts',(4.85068927007212,-13.5545179709986,-8.40164026752814));
#21453=CARTESIAN_POINT('Ctrl Pts',(-1.4883128981681E-11,-13.3795179709986,
-8.40164026751963));
#21454=CARTESIAN_POINT('Ctrl Pts',(-4.85068927010141,-13.2045179709986,
-8.40164026751123));
#21455=CARTESIAN_POINT('Ctrl Pts',(-7.27603390513763,-13.0295179709986,
-4.20082013374709));
#21456=CARTESIAN_POINT('Ctrl Pts',(-9.70137854017372,-12.8545179709986,
1.71332636794417E-11));
#21457=CARTESIAN_POINT('Ctrl Pts',(-7.2760339051228,-12.6795179709986,4.20082013377279));
#21458=CARTESIAN_POINT('Ctrl Pts',(-4.85068927007221,-12.5045179709986,
8.40164026752809));
#21459=CARTESIAN_POINT('Ctrl Pts',(1.47925542105866E-11,-12.3295179709986,
8.40164026751963));
#21460=CARTESIAN_POINT('Ctrl Pts',(4.85068927010179,-12.1545179709986,8.401640267511));
#21461=CARTESIAN_POINT('Ctrl Pts',(7.27603390513759,-11.9795179709986,4.20082013374717));
#21462=CARTESIAN_POINT('Ctrl Pts',(9.70137854017372,-11.8045179709986,-1.70286769424954E-11));
#21463=CARTESIAN_POINT('Ctrl Pts',(7.27603390512284,-11.6295179709986,-4.20082013377271));
#21464=CARTESIAN_POINT('Ctrl Pts',(4.8506892700723,-11.4545179709986,-8.40164026752804));
#21465=CARTESIAN_POINT('Ctrl Pts',(-1.47019794394921E-11,-11.2795179709986,
-8.40164026751963));
#21466=CARTESIAN_POINT('Ctrl Pts',(-4.8506892701017,-11.1045179709986,-8.40164026751106));
#21467=CARTESIAN_POINT('Ctrl Pts',(-7.27603390513778,-10.9295179709986,
-4.20082013374683));
#21468=CARTESIAN_POINT('Ctrl Pts',(-9.70137854017372,-10.7545179709986,
1.69240902055491E-11));
#21469=CARTESIAN_POINT('Ctrl Pts',(-7.27603390512289,-10.5795179709986,
4.20082013377263));
#21470=CARTESIAN_POINT('Ctrl Pts',(-4.85068927007191,-10.4045179709986,
8.40164026752826));
#21471=CARTESIAN_POINT('Ctrl Pts',(1.46114046683977E-11,-10.2295179709986,
8.40164026751963));
#21472=CARTESIAN_POINT('Ctrl Pts',(4.85068927010161,-10.0545179709986,8.40164026751111));
#21473=CARTESIAN_POINT('Ctrl Pts',(7.27603390513774,-9.87951797099859,4.20082013374691));
#21474=CARTESIAN_POINT('Ctrl Pts',(9.70137854017372,-9.70451797099858,-1.68195034686027E-11));
#21475=CARTESIAN_POINT('Ctrl Pts',(7.27603390512293,-9.52951797099857,-4.20082013377256));
#21476=CARTESIAN_POINT('Ctrl Pts',(4.850689270072,-9.3545179709986,-8.40164026752821));
#21477=CARTESIAN_POINT('Ctrl Pts',(-1.49984078541476E-11,-9.17951797099859,
-8.40164026751963));
#21478=CARTESIAN_POINT('Ctrl Pts',(-4.85068927010152,-9.00451797099859,
-8.40164026751116));
#21479=CARTESIAN_POINT('Ctrl Pts',(-7.27603390513769,-8.8295179709986,-4.20082013374699));
#21480=CARTESIAN_POINT('Ctrl Pts',(-9.70137854017372,-8.65451797099859,
1.72663762555427E-11));
#21481=CARTESIAN_POINT('Ctrl Pts',(-7.27603390512298,-8.47951797099858,
4.20082013377248));
#21482=CARTESIAN_POINT('Ctrl Pts',(-4.85068927007209,-8.3045179709986,8.40164026752815));
#21483=CARTESIAN_POINT('Ctrl Pts',(1.49078330830532E-11,-8.12951797099859,
8.40164026751963));
#21484=CARTESIAN_POINT('Ctrl Pts',(4.85068927010143,-7.95451797099859,8.40164026751122));
#21485=CARTESIAN_POINT('Ctrl Pts',(7.27603390513765,-7.7795179709986,4.20082013374707));
#21486=CARTESIAN_POINT('Ctrl Pts',(9.70137854017372,-7.60451797099859,-1.71617895185964E-11));
#21487=CARTESIAN_POINT('Ctrl Pts',(7.27603390512302,-7.42951797099858,-4.2008201337724));
#21488=CARTESIAN_POINT('Ctrl Pts',(4.85068927007219,-7.25451797099861,-8.4016402675281));
#21489=CARTESIAN_POINT('Ctrl Pts',(-1.48172583119587E-11,-7.07951797099859,
-8.40164026751963));
#21490=CARTESIAN_POINT('Ctrl Pts',(-4.85068927010182,-6.90451797099859,
-8.40164026751099));
#21491=CARTESIAN_POINT('Ctrl Pts',(-7.2760339051376,-6.72951797099858,-4.20082013374715));
#21492=CARTESIAN_POINT('Ctrl Pts',(-9.70137854017372,-6.5545179709986,1.705720278165E-11));
#21493=CARTESIAN_POINT('Ctrl Pts',(-7.27603390512283,-6.37951797099859,
4.20082013377273));
#21494=CARTESIAN_POINT('Ctrl Pts',(-4.85068927007227,-6.20451797099858,
8.40164026752805));
#21495=CARTESIAN_POINT('Ctrl Pts',(1.47266835408643E-11,-6.0295179709986,
8.40164026751963));
#21496=CARTESIAN_POINT('Ctrl Pts',(4.85068927010173,-5.8545179709986,8.40164026751104));
#21497=CARTESIAN_POINT('Ctrl Pts',(7.27603390513756,-5.67951797099858,4.20082013374722));
#21498=CARTESIAN_POINT('Ctrl Pts',(9.70137854017372,-5.5045179709986,-1.69526160447037E-11));
#21499=CARTESIAN_POINT('Ctrl Pts',(7.27603390512287,-5.32951797099859,-4.20082013377265));
#21500=CARTESIAN_POINT('Ctrl Pts',(4.85068927007189,-5.15451797099859,-8.40164026752827));
#21501=CARTESIAN_POINT('Ctrl Pts',(-1.46361087697698E-11,-4.9795179709986,
-8.40164026751963));
#21502=CARTESIAN_POINT('Ctrl Pts',(-4.85068927010164,-4.8045179709986,-8.40164026751109));
#21503=CARTESIAN_POINT('Ctrl Pts',(-7.27603390513775,-4.62951797099859,
-4.20082013374689));
#21504=CARTESIAN_POINT('Ctrl Pts',(-9.70137854017372,-4.45451797099861,
1.68480293077573E-11));
#21505=CARTESIAN_POINT('Ctrl Pts',(-7.27603390512292,-4.2795179709986,4.20082013377258));
#21506=CARTESIAN_POINT('Ctrl Pts',(-4.85068927007198,-4.10451797099859,
8.40164026752822));
#21507=CARTESIAN_POINT('Ctrl Pts',(1.45455339986754E-11,-3.92951797099861,
8.40164026751963));
#21508=CARTESIAN_POINT('Ctrl Pts',(4.85068927010155,-3.75451797099861,8.40164026751115));
#21509=CARTESIAN_POINT('Ctrl Pts',(7.2760339051377,-3.57951797099859,4.20082013374697));
#21510=CARTESIAN_POINT('Ctrl Pts',(9.70137854017372,-3.40451797099861,-1.72949020946973E-11));
#21511=CARTESIAN_POINT('Ctrl Pts',(7.27603390512296,-3.2295179709986,-4.2008201337725));
#21512=CARTESIAN_POINT('Ctrl Pts',(4.85068927007207,-3.0545179709986,-8.40164026752817));
#21513=CARTESIAN_POINT('Ctrl Pts',(-1.49325371844254E-11,-2.87951797099861,
-8.40164026751963));
#21514=CARTESIAN_POINT('Ctrl Pts',(-4.85068927010146,-2.70451797099861,
-8.4016402675112));
#21515=CARTESIAN_POINT('Ctrl Pts',(-7.27603390513766,-2.5295179709986,-4.20082013374705));
#21516=CARTESIAN_POINT('Ctrl Pts',(-9.70137854017372,-2.3545179709986,1.7190315357751E-11));
#21517=CARTESIAN_POINT('Ctrl Pts',(-7.27603390512301,-2.17951797099861,
4.20082013377242));
#21518=CARTESIAN_POINT('Ctrl Pts',(-4.85068927007216,-2.0045179709986,8.40164026752812));
#21519=CARTESIAN_POINT('Ctrl Pts',(1.48419624133309E-11,-1.82951797099859,
8.40164026751963));
#21520=CARTESIAN_POINT('Ctrl Pts',(4.85068927010137,-1.65451797099861,8.40164026751125));
#21521=CARTESIAN_POINT('Ctrl Pts',(7.27603390513761,-1.4795179709986,4.20082013374713));
#21522=CARTESIAN_POINT('Ctrl Pts',(9.70137854017372,-1.3045179709986,-1.70857286208046E-11));
#21523=CARTESIAN_POINT('Ctrl Pts',(7.27603390512282,-1.12951797099861,-4.20082013377275));
#21524=CARTESIAN_POINT('Ctrl Pts',(4.85068927007225,-0.954517970998605,
-8.40164026752806));
#21525=CARTESIAN_POINT('Ctrl Pts',(-1.47513876422365E-11,-0.779517970998594,
-8.40164026751963));
#21526=CARTESIAN_POINT('Ctrl Pts',(-4.85068927010175,-0.604517970998614,
-8.40164026751103));
#21527=CARTESIAN_POINT('Ctrl Pts',(-7.27603390513757,-0.429517970998605,
-4.2008201337472));
#21528=CARTESIAN_POINT('Ctrl Pts',(-9.70137854017372,-0.2545179709986,1.69811418838583E-11));
#21529=CARTESIAN_POINT('Ctrl Pts',(-7.27603390512286,-0.079517970998616,
4.20082013377267));
#21530=CARTESIAN_POINT('Ctrl Pts',(-4.85068927007234,0.0954820290013905,
8.40164026752801));
#21531=CARTESIAN_POINT('Ctrl Pts',(1.4660812871142E-11,0.270482029001401,
8.40164026751963));
#21532=CARTESIAN_POINT('Ctrl Pts',(4.85068927010166,0.445482029001381,8.40164026751108));
#21533=CARTESIAN_POINT('Ctrl Pts',(7.27603390513776,0.62048202900139,4.20082013374687));
#21534=CARTESIAN_POINT('Ctrl Pts',(9.70137854017372,0.795482029001396,-1.6876555146912E-11));
#21535=CARTESIAN_POINT('Ctrl Pts',(7.27603390512291,0.970482029001379,-4.2008201337726));
#21536=CARTESIAN_POINT('Ctrl Pts',(4.85068927007195,1.14548202900139,-8.40164026752823));
#21537=CARTESIAN_POINT('Ctrl Pts',(-1.45702381000475E-11,1.3204820290014,
-8.40164026751963));
#21538=CARTESIAN_POINT('Ctrl Pts',(-4.85068927010157,1.49548202900138,-8.40164026751113));
#21539=CARTESIAN_POINT('Ctrl Pts',(-7.27603390513772,1.67048202900139,-4.20082013374695));
#21540=CARTESIAN_POINT('Ctrl Pts',(-9.70137854017372,1.84548202900139,1.67719684099656E-11));
#21541=CARTESIAN_POINT('Ctrl Pts',(-7.27603390512295,2.0204820290014,4.20082013377252));
#21542=CARTESIAN_POINT('Ctrl Pts',(-4.85068927007204,2.19548202900138,8.40164026752818));
#21543=CARTESIAN_POINT('Ctrl Pts',(1.49572412857975E-11,2.37048202900139,
8.40164026751963));
#21544=CARTESIAN_POINT('Ctrl Pts',(4.85068927010148,2.5454820290014,8.40164026751119));
#21545=CARTESIAN_POINT('Ctrl Pts',(7.27603390513767,2.72048202900138,4.20082013374703));
#21546=CARTESIAN_POINT('Ctrl Pts',(9.70137854017372,2.89548202900139,-1.72188411969056E-11));
#21547=CARTESIAN_POINT('Ctrl Pts',(7.276033905123,3.0704820290014,-4.20082013377244));
#21548=CARTESIAN_POINT('Ctrl Pts',(4.85068927007213,3.24548202900138,-8.40164026752813));
#21549=CARTESIAN_POINT('Ctrl Pts',(-1.48666665147031E-11,3.42048202900139,
-8.40164026751963));
#21550=CARTESIAN_POINT('Ctrl Pts',(-4.85068927010139,3.59548202900139,-8.40164026751124));
#21551=CARTESIAN_POINT('Ctrl Pts',(-7.27603390513763,3.77048202900138,-4.2008201337471));
#21552=CARTESIAN_POINT('Ctrl Pts',(-9.70137854017372,3.94548202900138,1.71142544599593E-11));
#21553=CARTESIAN_POINT('Ctrl Pts',(-7.27603390512304,4.12048202900139,4.20082013377236));
#21554=CARTESIAN_POINT('Ctrl Pts',(-4.85068927007222,4.29548202900137,8.40164026752808));
#21555=CARTESIAN_POINT('Ctrl Pts',(1.47760917436086E-11,4.47048202900138,
8.40164026751963));
#21556=CARTESIAN_POINT('Ctrl Pts',(4.85068927010178,4.64548202900139,8.40164026751101));
#21557=CARTESIAN_POINT('Ctrl Pts',(7.27603390513758,4.82048202900137,4.20082013374718));
#21558=CARTESIAN_POINT('Ctrl Pts',(9.70137854017372,4.99548202900138,-1.70096677230129E-11));
#21559=CARTESIAN_POINT('Ctrl Pts',(7.27603390512285,5.17048202900139,-4.2008201337727));
#21560=CARTESIAN_POINT('Ctrl Pts',(4.85068927007232,5.34548202900137,-8.40164026752803));
#21561=CARTESIAN_POINT('Ctrl Pts',(-1.46855169725142E-11,5.52048202900138,
-8.40164026751963));
#21562=CARTESIAN_POINT('Ctrl Pts',(-4.85068927010169,5.69548202900138,-8.40164026751107));
#21563=CARTESIAN_POINT('Ctrl Pts',(-7.27603390513754,5.87048202900137,-4.20082013374726));
#21564=CARTESIAN_POINT('Ctrl Pts',(-9.70137854017372,6.04548202900137,1.69050809860666E-11));
#21565=CARTESIAN_POINT('Ctrl Pts',(-7.27603390512289,6.22048202900138,4.20082013377262));
#21566=CARTESIAN_POINT('Ctrl Pts',(-4.85068927007193,6.39548202900136,8.40164026752825));
#21567=CARTESIAN_POINT('Ctrl Pts',(1.45949422014197E-11,6.57048202900137,
8.40164026751963));
#21568=CARTESIAN_POINT('Ctrl Pts',(4.8506892701016,6.74548202900138,8.40164026751112));
#21569=CARTESIAN_POINT('Ctrl Pts',(7.27603390513773,6.92048202900139,4.20082013374692));
#21570=CARTESIAN_POINT('Ctrl Pts',(9.70137854017372,7.09548202900137,-1.68004942491202E-11));
#21571=CARTESIAN_POINT('Ctrl Pts',(7.27603390512294,7.27048202900138,-4.20082013377254));
#21572=CARTESIAN_POINT('Ctrl Pts',(4.85068927007202,7.44548202900138,-8.4016402675282));
#21573=CARTESIAN_POINT('Ctrl Pts',(-1.45043674303253E-11,7.62048202900137,
-8.40164026751963));
#21574=CARTESIAN_POINT('Ctrl Pts',(-4.85068927010151,7.79548202900137,-8.40164026751117));
#21575=CARTESIAN_POINT('Ctrl Pts',(-7.27603390513768,7.97048202900139,-4.200820133747));
#21576=CARTESIAN_POINT('Ctrl Pts',(-9.70137854017372,8.14548202900136,1.72473670360602E-11));
#21577=CARTESIAN_POINT('Ctrl Pts',(-7.27603390512298,8.32048202900138,4.20082013377246));
#21578=CARTESIAN_POINT('Ctrl Pts',(-4.85068927007211,8.49548202900138,8.40164026752814));
#21579=CARTESIAN_POINT('Ctrl Pts',(1.48913706160753E-11,8.67048202900136,
8.40164026751963));
#21580=CARTESIAN_POINT('Ctrl Pts',(4.85068927010141,8.84548202900137,8.40164026751122));
#21581=CARTESIAN_POINT('Ctrl Pts',(7.27603390513764,9.02048202900138,4.20082013374708));
#21582=CARTESIAN_POINT('Ctrl Pts',(9.70137854017372,9.19548202900136,-1.71427802991139E-11));
#21583=CARTESIAN_POINT('Ctrl Pts',(7.27603390512303,9.37048202900137,-4.20082013377238));
#21584=CARTESIAN_POINT('Ctrl Pts',(4.8506892700722,9.54548202900137,-8.40164026752809));
#21585=CARTESIAN_POINT('Ctrl Pts',(-1.48007958449808E-11,9.72048202900136,
-8.40164026751963));
#21586=CARTESIAN_POINT('Ctrl Pts',(-4.8506892701018,9.89548202900136,-8.401640267511));
#21587=CARTESIAN_POINT('Ctrl Pts',(-7.27603390513759,10.0704820290014,-4.20082013374716));
#21588=CARTESIAN_POINT('Ctrl Pts',(-9.70137854017372,10.2454820290014,1.70381935621676E-11));
#21589=CARTESIAN_POINT('Ctrl Pts',(-7.27603390512284,10.4204820290014,4.20082013377272));
#21590=CARTESIAN_POINT('Ctrl Pts',(-4.85068927007229,10.5954820290014,8.40164026752804));
#21591=CARTESIAN_POINT('Ctrl Pts',(1.47102210738864E-11,10.7704820290014,
8.40164026751963));
#21592=CARTESIAN_POINT('Ctrl Pts',(4.85068927010171,10.9454820290014,8.40164026751105));
#21593=CARTESIAN_POINT('Ctrl Pts',(7.27603390513755,11.1204820290014,4.20082013374724));
#21594=CARTESIAN_POINT('Ctrl Pts',(9.70137854017372,11.2954820290014,-1.69336068252212E-11));
#21595=CARTESIAN_POINT('Ctrl Pts',(7.27603390512288,11.4704820290014,-4.20082013377264));
#21596=CARTESIAN_POINT('Ctrl Pts',(4.85068927007238,11.6454820290014,-8.40164026752799));
#21597=CARTESIAN_POINT('Ctrl Pts',(-1.46196463027919E-11,11.8204820290014,
-8.40164026751963));
#21598=CARTESIAN_POINT('Ctrl Pts',(-4.85068927010162,11.9954820290014,-8.40164026751111));
#21599=CARTESIAN_POINT('Ctrl Pts',(-7.27603390513774,12.1704820290014,-4.2008201337469));
#21600=CARTESIAN_POINT('Ctrl Pts',(-9.70137854017372,12.3454820290014,1.68290200882749E-11));
#21601=CARTESIAN_POINT('Ctrl Pts',(-7.27603390512293,12.5204820290014,4.20082013377256));
#21602=CARTESIAN_POINT('Ctrl Pts',(-4.85068927007199,12.6954820290014,8.40164026752821));
#21603=CARTESIAN_POINT('Ctrl Pts',(1.45290715316974E-11,12.8704820290014,
8.40164026751963));
#21604=CARTESIAN_POINT('Ctrl Pts',(4.85068927010153,13.0454820290013,8.40164026751116));
#21605=CARTESIAN_POINT('Ctrl Pts',(7.2760339051377,13.2204820290014,4.20082013374698));
#21606=CARTESIAN_POINT('Ctrl Pts',(9.70137854017372,13.3954820290014,-1.67244333513285E-11));
#21607=CARTESIAN_POINT('Ctrl Pts',(7.27603390512297,13.5704820290014,-4.20082013377248));
#21608=CARTESIAN_POINT('Ctrl Pts',(4.85068927007208,13.7454820290014,-8.40164026752816));
#21609=CARTESIAN_POINT('Ctrl Pts',(-1.49160747174474E-11,13.9204820290014,
-8.40164026751963));
#21610=CARTESIAN_POINT('Ctrl Pts',(-4.85068927010144,14.0954820290013,-8.40164026751121));
#21611=CARTESIAN_POINT('Ctrl Pts',(-7.27603390513765,14.2704820290014,-4.20082013374706));
#21612=CARTESIAN_POINT('Ctrl Pts',(-9.70137854017372,14.4454820290014,1.71713061382685E-11));
#21613=CARTESIAN_POINT('Ctrl Pts',(-7.27603390512302,14.6204820290013,4.2008201337724));
#21614=CARTESIAN_POINT('Ctrl Pts',(-4.85068927007218,14.7954820290014,8.40164026752811));
#21615=CARTESIAN_POINT('Ctrl Pts',(1.4825499946353E-11,14.9704820290014,
8.40164026751963));
#21616=CARTESIAN_POINT('Ctrl Pts',(4.85068927010135,15.1454820290013,8.40164026751126));
#21617=CARTESIAN_POINT('Ctrl Pts',(7.27603390513761,15.3204820290014,4.20082013374714));
#21618=CARTESIAN_POINT('Ctrl Pts',(9.70137854017372,15.4954820290014,-1.70667194013222E-11));
#21619=CARTESIAN_POINT('Ctrl Pts',(7.27603390512282,15.6704820290014,-4.20082013377274));
#21620=CARTESIAN_POINT('Ctrl Pts',(4.85068927007227,15.8454820290013,-8.40164026752806));
#21621=CARTESIAN_POINT('Ctrl Pts',(-1.47349251752585E-11,16.0204820290014,
-8.40164026751963));
#21622=CARTESIAN_POINT('Ctrl Pts',(-4.85068927010174,16.1954820290014,-8.40164026751104));
#21623=CARTESIAN_POINT('Ctrl Pts',(-7.27603390513756,16.3704820290014,-4.20082013374722));
#21624=CARTESIAN_POINT('Ctrl Pts',(-9.70137854017372,16.5454820290013,1.69621326643758E-11));
#21625=CARTESIAN_POINT('Ctrl Pts',(-7.27603390512287,16.7204820290014,4.20082013377266));
#21626=CARTESIAN_POINT('Ctrl Pts',(-4.85068927007236,16.8954820290013,8.401640267528));
#21627=CARTESIAN_POINT('Ctrl Pts',(1.46443504041641E-11,17.0704820290014,
8.40164026751963));
#21628=CARTESIAN_POINT('Ctrl Pts',(4.85068927010165,17.2454820290014,8.40164026751109));
#21629=CARTESIAN_POINT('Ctrl Pts',(7.27603390513752,17.4204820290013,4.2008201337473));
#21630=CARTESIAN_POINT('Ctrl Pts',(9.70137854017372,17.5954820290013,-1.68575459274295E-11));
#21631=CARTESIAN_POINT('Ctrl Pts',(7.27603390512292,17.7704820290014,-4.20082013377258));
#21632=CARTESIAN_POINT('Ctrl Pts',(4.85068927007197,17.9454820290013,-8.40164026752823));
#21633=CARTESIAN_POINT('Ctrl Pts',(-1.45537756330696E-11,18.1204820290014,
-8.40164026751963));
#21634=CARTESIAN_POINT('Ctrl Pts',(-4.85068927010155,18.2954820290014,-8.40164026751114));
#21635=CARTESIAN_POINT('Ctrl Pts',(-7.27603390513771,18.4704820290013,-4.20082013374696));
#21636=CARTESIAN_POINT('Ctrl Pts',(-9.70137854017372,18.6454820290013,1.67529591904832E-11));
#21637=CARTESIAN_POINT('Ctrl Pts',(-7.27603390512296,18.8204820290014,4.2008201337725));
#21638=CARTESIAN_POINT('Ctrl Pts',(-4.85068927007206,18.9954820290013,8.40164026752817));
#21639=CARTESIAN_POINT('Ctrl Pts',(1.44632008619752E-11,19.1704820290013,
8.40164026751963));
#21640=CARTESIAN_POINT('Ctrl Pts',(4.85068927010146,19.3454820290013,8.4016402675112));
#21641=CARTESIAN_POINT('Ctrl Pts',(7.27603390513766,19.5204820290013,4.20082013374704));
#21642=CARTESIAN_POINT('Ctrl Pts',(9.70137854017372,19.6954820290013,-1.71998319774232E-11));
#21643=CARTESIAN_POINT('Ctrl Pts',(7.27603390512301,19.8704820290014,-4.20082013377243));
#21644=CARTESIAN_POINT('Ctrl Pts',(4.85068927007215,20.0454820290014,-8.40164026752812));
#21645=CARTESIAN_POINT('Ctrl Pts',(-1.48502040477252E-11,20.2204820290013,
-8.40164026751963));
#21646=CARTESIAN_POINT('Ctrl Pts',(-4.85068927010137,20.3954820290014,-8.40164026751125));
#21647=CARTESIAN_POINT('Ctrl Pts',(-7.27603390513762,20.5704820290014,-4.20082013374712));
#21648=CARTESIAN_POINT('Ctrl Pts',(-9.70137854017372,20.7454820290013,1.70952452404768E-11));
#21649=CARTESIAN_POINT('Ctrl Pts',(-7.27603390512305,20.9204820290013,4.20082013377235));
#21650=CARTESIAN_POINT('Ctrl Pts',(-4.85068927007224,21.0954820290014,8.40164026752807));
#21651=CARTESIAN_POINT('Ctrl Pts',(1.47596292766307E-11,21.2704820290013,
8.40164026751963));
#21652=CARTESIAN_POINT('Ctrl Pts',(4.85068927010176,21.4454820290013,8.40164026751102));
#21653=CARTESIAN_POINT('Ctrl Pts',(7.27603390513757,21.6204820290014,4.2008201337472));
#21654=CARTESIAN_POINT('Ctrl Pts',(9.70137854017372,21.7954820290013,-1.69906585035305E-11));
#21655=CARTESIAN_POINT('Ctrl Pts',(7.27603390512286,21.9704820290013,-4.20082013377268));
#21656=CARTESIAN_POINT('Ctrl Pts',(5.65116042235429,22.0877242779482,-7.015183561788));
#21657=CARTESIAN_POINT('Ctrl Pts',(2.55537495509676,22.22,-8.00360031633711));
#21658=CARTESIAN_POINT('Ctrl Pts',(-1.51301075899711E-11,-144.093984254242,
-8.40164026751963));
#21659=CARTESIAN_POINT('Ctrl Pts',(-4.85068927010199,-143.918984254242,
-8.4016402675109));
#21660=CARTESIAN_POINT('Ctrl Pts',(-7.27603390513785,-143.743984254242,
-4.20082013374671));
#21661=CARTESIAN_POINT('Ctrl Pts',(-9.70137854017372,-143.568984254242,
1.74701493417668E-11));
#21662=CARTESIAN_POINT('Ctrl Pts',(-7.27603390512272,-143.393984254242,
4.20082013377292));
#21663=CARTESIAN_POINT('Ctrl Pts',(-4.85068927007173,-143.218984254242,
8.40164026752836));
#21664=CARTESIAN_POINT('Ctrl Pts',(1.5129078685785E-11,-143.043984254242,
8.40164026751963));
#21665=CARTESIAN_POINT('Ctrl Pts',(4.85068927010198,-142.868984254242,8.4016402675109));
#21666=CARTESIAN_POINT('Ctrl Pts',(7.27603390513785,-142.693984254242,4.20082013374672));
#21667=CARTESIAN_POINT('Ctrl Pts',(9.70137854017372,-142.518984254242,-1.74689612655491E-11));
#21668=CARTESIAN_POINT('Ctrl Pts',(7.27603390512273,-142.343984254242,-4.20082013377291));
#21669=CARTESIAN_POINT('Ctrl Pts',(4.85068927007173,-142.168984254242,-8.40164026752836));
#21670=CARTESIAN_POINT('Ctrl Pts',(-1.51301075899711E-11,-141.993984254242,
-8.40164026751963));
#21671=CARTESIAN_POINT('Ctrl Pts',(-4.85068927010199,-141.818984254242,
-8.4016402675109));
#21672=CARTESIAN_POINT('Ctrl Pts',(-7.27603390513785,-141.643984254242,
-4.20082013374671));
#21673=CARTESIAN_POINT('Ctrl Pts',(-9.70137854017372,-141.468984254242,
1.74701493417668E-11));
#21674=CARTESIAN_POINT('Ctrl Pts',(-7.27603390512272,-141.293984254242,
4.20082013377292));
#21675=CARTESIAN_POINT('Ctrl Pts',(-4.85068927007173,-141.118984254242,
8.40164026752836));
#21676=CARTESIAN_POINT('Ctrl Pts',(1.5129078685785E-11,-140.943984254242,
8.40164026751963));
#21677=CARTESIAN_POINT('Ctrl Pts',(4.85068927010198,-140.768984254242,8.4016402675109));
#21678=CARTESIAN_POINT('Ctrl Pts',(7.27603390513785,-140.593984254242,4.20082013374672));
#21679=CARTESIAN_POINT('Ctrl Pts',(9.70137854017372,-140.418984254242,-1.74689612655491E-11));
#21680=CARTESIAN_POINT('Ctrl Pts',(7.27603390512273,-140.243984254242,-4.20082013377291));
#21681=CARTESIAN_POINT('Ctrl Pts',(4.85068927007173,-140.068984254242,-8.40164026752836));
#21682=CARTESIAN_POINT('Ctrl Pts',(-1.51301075899711E-11,-139.893984254242,
-8.40164026751963));
#21683=CARTESIAN_POINT('Ctrl Pts',(-4.85068927010199,-139.718984254242,
-8.4016402675109));
#21684=CARTESIAN_POINT('Ctrl Pts',(-7.27603390513785,-139.543984254242,
-4.20082013374671));
#21685=CARTESIAN_POINT('Ctrl Pts',(-9.70137854017372,-139.368984254242,
1.74701493417668E-11));
#21686=CARTESIAN_POINT('Ctrl Pts',(-7.27603390512272,-139.193984254242,
4.20082013377292));
#21687=CARTESIAN_POINT('Ctrl Pts',(-4.85068927007173,-139.018984254242,
8.40164026752836));
#21688=CARTESIAN_POINT('Ctrl Pts',(1.5129078685785E-11,-138.843984254242,
8.40164026751963));
#21689=CARTESIAN_POINT('Ctrl Pts',(4.85068927010198,-138.668984254242,8.4016402675109));
#21690=CARTESIAN_POINT('Ctrl Pts',(7.27603390513785,-138.493984254242,4.20082013374672));
#21691=CARTESIAN_POINT('Ctrl Pts',(9.70137854017372,-138.318984254242,-1.74689612655491E-11));
#21692=CARTESIAN_POINT('Ctrl Pts',(7.27603390512273,-138.143984254242,-4.20082013377291));
#21693=CARTESIAN_POINT('Ctrl Pts',(4.85068927007173,-137.968984254242,-8.40164026752836));
#21694=CARTESIAN_POINT('Ctrl Pts',(-1.51301075899711E-11,-137.793984254242,
-8.40164026751963));
#21695=CARTESIAN_POINT('Ctrl Pts',(-4.85068927010199,-137.618984254242,
-8.4016402675109));
#21696=CARTESIAN_POINT('Ctrl Pts',(-7.27603390513785,-137.443984254242,
-4.20082013374671));
#21697=CARTESIAN_POINT('Ctrl Pts',(-9.70137854017372,-137.268984254242,
1.74701493417668E-11));
#21698=CARTESIAN_POINT('Ctrl Pts',(-7.27603390512272,-137.093984254242,
4.20082013377292));
#21699=CARTESIAN_POINT('Ctrl Pts',(-4.85068927007173,-136.918984254242,
8.40164026752836));
#21700=CARTESIAN_POINT('Ctrl Pts',(1.5129078685785E-11,-136.743984254242,
8.40164026751963));
#21701=CARTESIAN_POINT('Ctrl Pts',(4.85068927010198,-136.568984254242,8.4016402675109));
#21702=CARTESIAN_POINT('Ctrl Pts',(7.27603390513785,-136.393984254242,4.20082013374672));
#21703=CARTESIAN_POINT('Ctrl Pts',(9.70137854017372,-136.218984254242,-1.74689612655491E-11));
#21704=CARTESIAN_POINT('Ctrl Pts',(7.27603390512273,-136.043984254242,-4.20082013377291));
#21705=CARTESIAN_POINT('Ctrl Pts',(4.85068927007173,-135.868984254242,-8.40164026752836));
#21706=CARTESIAN_POINT('Ctrl Pts',(-1.51301075899711E-11,-135.693984254242,
-8.40164026751963));
#21707=CARTESIAN_POINT('Ctrl Pts',(-4.85068927010199,-135.518984254242,
-8.4016402675109));
#21708=CARTESIAN_POINT('Ctrl Pts',(-7.27603390513785,-135.343984254242,
-4.20082013374671));
#21709=CARTESIAN_POINT('Ctrl Pts',(-9.70137854017372,-135.168984254242,
1.74701493417668E-11));
#21710=CARTESIAN_POINT('Ctrl Pts',(-7.27603390512272,-134.993984254242,
4.20082013377292));
#21711=CARTESIAN_POINT('Ctrl Pts',(-4.85068927007173,-134.818984254242,
8.40164026752836));
#21712=CARTESIAN_POINT('Ctrl Pts',(1.5129078685785E-11,-134.643984254242,
8.40164026751963));
#21713=CARTESIAN_POINT('Ctrl Pts',(4.85068927010198,-134.468984254242,8.4016402675109));
#21714=CARTESIAN_POINT('Ctrl Pts',(7.27603390513785,-134.293984254242,4.20082013374672));
#21715=CARTESIAN_POINT('Ctrl Pts',(9.70137854017372,-134.118984254242,-1.74689612655491E-11));
#21716=CARTESIAN_POINT('Ctrl Pts',(7.27603390512273,-133.943984254242,-4.20082013377291));
#21717=CARTESIAN_POINT('Ctrl Pts',(4.85068927007173,-133.768984254242,-8.40164026752836));
#21718=CARTESIAN_POINT('Ctrl Pts',(-1.51301075899711E-11,-133.593984254242,
-8.40164026751963));
#21719=CARTESIAN_POINT('Ctrl Pts',(-4.85068927010199,-133.418984254242,
-8.4016402675109));
#21720=CARTESIAN_POINT('Ctrl Pts',(-7.27603390513785,-133.243984254242,
-4.20082013374671));
#21721=CARTESIAN_POINT('Ctrl Pts',(-9.70137854017372,-133.068984254242,
1.74701493417668E-11));
#21722=CARTESIAN_POINT('Ctrl Pts',(-7.27603390512272,-132.893984254242,
4.20082013377292));
#21723=CARTESIAN_POINT('Ctrl Pts',(-4.85068927007173,-132.718984254242,
8.40164026752836));
#21724=CARTESIAN_POINT('Ctrl Pts',(1.5129078685785E-11,-132.543984254242,
8.40164026751963));
#21725=CARTESIAN_POINT('Ctrl Pts',(4.85068927010198,-132.368984254242,8.4016402675109));
#21726=CARTESIAN_POINT('Ctrl Pts',(7.27603390513785,-132.193984254242,4.20082013374672));
#21727=CARTESIAN_POINT('Ctrl Pts',(9.70137854017372,-132.018984254242,-1.74689612655491E-11));
#21728=CARTESIAN_POINT('Ctrl Pts',(7.27603390512273,-131.843984254242,-4.20082013377291));
#21729=CARTESIAN_POINT('Ctrl Pts',(4.85068927007173,-131.668984254242,-8.40164026752836));
#21730=CARTESIAN_POINT('Ctrl Pts',(-1.51301075899711E-11,-131.493984254242,
-8.40164026751963));
#21731=CARTESIAN_POINT('Ctrl Pts',(-4.85068927010199,-131.318984254242,
-8.4016402675109));
#21732=CARTESIAN_POINT('Ctrl Pts',(-7.27603390513785,-131.143984254242,
-4.20082013374671));
#21733=CARTESIAN_POINT('Ctrl Pts',(-9.70137854017372,-130.968984254242,
1.74701493417668E-11));
#21734=CARTESIAN_POINT('Ctrl Pts',(-7.27603390512272,-130.793984254242,
4.20082013377292));
#21735=CARTESIAN_POINT('Ctrl Pts',(-4.85068927007173,-130.618984254242,
8.40164026752836));
#21736=CARTESIAN_POINT('Ctrl Pts',(1.5129078685785E-11,-130.443984254242,
8.40164026751963));
#21737=CARTESIAN_POINT('Ctrl Pts',(4.85068927010198,-130.268984254242,8.4016402675109));
#21738=CARTESIAN_POINT('Ctrl Pts',(7.27603390513785,-130.093984254242,4.20082013374672));
#21739=CARTESIAN_POINT('Ctrl Pts',(9.70137854017372,-129.918984254242,-1.74689612655491E-11));
#21740=CARTESIAN_POINT('Ctrl Pts',(7.27603390512273,-129.743984254242,-4.20082013377291));
#21741=CARTESIAN_POINT('Ctrl Pts',(4.85068927007173,-129.568984254242,-8.40164026752836));
#21742=CARTESIAN_POINT('Ctrl Pts',(-1.51301075899711E-11,-129.393984254242,
-8.40164026751963));
#21743=CARTESIAN_POINT('Ctrl Pts',(-4.85068927010199,-129.218984254242,
-8.4016402675109));
#21744=CARTESIAN_POINT('Ctrl Pts',(-7.27603390513785,-129.043984254242,
-4.20082013374671));
#21745=CARTESIAN_POINT('Ctrl Pts',(-9.70137854017372,-128.868984254242,
1.74701493417668E-11));
#21746=CARTESIAN_POINT('Ctrl Pts',(-7.27603390512272,-128.693984254242,
4.20082013377292));
#21747=CARTESIAN_POINT('Ctrl Pts',(-4.85068927007173,-128.518984254242,
8.40164026752836));
#21748=CARTESIAN_POINT('Ctrl Pts',(1.5129078685785E-11,-128.343984254242,
8.40164026751963));
#21749=CARTESIAN_POINT('Ctrl Pts',(4.85068927010198,-128.168984254242,8.4016402675109));
#21750=CARTESIAN_POINT('Ctrl Pts',(7.27603390513785,-127.993984254242,4.20082013374672));
#21751=CARTESIAN_POINT('Ctrl Pts',(9.70137854017372,-127.818984254242,-1.74689612655491E-11));
#21752=CARTESIAN_POINT('Ctrl Pts',(7.27603390512273,-127.643984254242,-4.20082013377291));
#21753=CARTESIAN_POINT('Ctrl Pts',(4.85068927007173,-127.468984254242,-8.40164026752836));
#21754=CARTESIAN_POINT('Ctrl Pts',(-1.51301075899711E-11,-127.293984254242,
-8.40164026751963));
#21755=CARTESIAN_POINT('Ctrl Pts',(-4.85068927010199,-127.118984254242,
-8.4016402675109));
#21756=CARTESIAN_POINT('Ctrl Pts',(-7.27603390513785,-126.943984254242,
-4.20082013374671));
#21757=CARTESIAN_POINT('Ctrl Pts',(-9.70137854017372,-126.768984254242,
1.74701493417668E-11));
#21758=CARTESIAN_POINT('Ctrl Pts',(-7.27603390512272,-126.593984254242,
4.20082013377292));
#21759=CARTESIAN_POINT('Ctrl Pts',(-4.85068927007173,-126.418984254242,
8.40164026752836));
#21760=CARTESIAN_POINT('Ctrl Pts',(1.5129078685785E-11,-126.243984254242,
8.40164026751963));
#21761=CARTESIAN_POINT('Ctrl Pts',(4.85068927010198,-126.068984254242,8.4016402675109));
#21762=CARTESIAN_POINT('Ctrl Pts',(7.27603390513785,-125.893984254242,4.20082013374672));
#21763=CARTESIAN_POINT('Ctrl Pts',(9.70137854017372,-125.718984254242,-1.74689612655491E-11));
#21764=CARTESIAN_POINT('Ctrl Pts',(7.27603390512273,-125.543984254242,-4.20082013377291));
#21765=CARTESIAN_POINT('Ctrl Pts',(4.85068927007173,-125.368984254242,-8.40164026752836));
#21766=CARTESIAN_POINT('Ctrl Pts',(-1.51301075899711E-11,-125.193984254242,
-8.40164026751963));
#21767=CARTESIAN_POINT('Ctrl Pts',(-4.85068927010199,-125.018984254242,
-8.4016402675109));
#21768=CARTESIAN_POINT('Ctrl Pts',(-7.27603390513785,-124.843984254242,
-4.20082013374671));
#21769=CARTESIAN_POINT('Ctrl Pts',(-9.70137854017372,-124.668984254242,
1.74701493417668E-11));
#21770=CARTESIAN_POINT('Ctrl Pts',(-7.27603390512272,-124.493984254242,
4.20082013377292));
#21771=CARTESIAN_POINT('Ctrl Pts',(-4.85068927007173,-124.318984254242,
8.40164026752836));
#21772=CARTESIAN_POINT('Ctrl Pts',(1.5129078685785E-11,-124.143984254242,
8.40164026751963));
#21773=CARTESIAN_POINT('Ctrl Pts',(4.85068927010198,-123.968984254242,8.4016402675109));
#21774=CARTESIAN_POINT('Ctrl Pts',(7.27603390513785,-123.793984254242,4.20082013374672));
#21775=CARTESIAN_POINT('Ctrl Pts',(9.70137854017372,-123.618984254242,-1.74689612655491E-11));
#21776=CARTESIAN_POINT('Ctrl Pts',(7.27603390512273,-123.443984254242,-4.20082013377291));
#21777=CARTESIAN_POINT('Ctrl Pts',(4.85068927007173,-123.268984254242,-8.40164026752836));
#21778=CARTESIAN_POINT('Ctrl Pts',(-1.51301075899711E-11,-123.093984254242,
-8.40164026751963));
#21779=CARTESIAN_POINT('Ctrl Pts',(-4.85068927010199,-122.918984254242,
-8.4016402675109));
#21780=CARTESIAN_POINT('Ctrl Pts',(-7.27603390513785,-122.743984254242,
-4.20082013374671));
#21781=CARTESIAN_POINT('Ctrl Pts',(-9.70137854017372,-122.568984254242,
1.74701493417668E-11));
#21782=CARTESIAN_POINT('Ctrl Pts',(-7.27603390512272,-122.393984254242,
4.20082013377292));
#21783=CARTESIAN_POINT('Ctrl Pts',(-4.85068927007173,-122.218984254242,
8.40164026752836));
#21784=CARTESIAN_POINT('Ctrl Pts',(1.5129078685785E-11,-122.043984254242,
8.40164026751963));
#21785=CARTESIAN_POINT('Ctrl Pts',(4.85068927010198,-121.868984254242,8.4016402675109));
#21786=CARTESIAN_POINT('Ctrl Pts',(7.27603390513785,-121.693984254242,4.20082013374672));
#21787=CARTESIAN_POINT('Ctrl Pts',(9.70137854017372,-121.518984254242,-1.74689612655491E-11));
#21788=CARTESIAN_POINT('Ctrl Pts',(7.27603390512273,-121.343984254242,-4.20082013377291));
#21789=CARTESIAN_POINT('Ctrl Pts',(4.85068927007173,-121.168984254242,-8.40164026752836));
#21790=CARTESIAN_POINT('Ctrl Pts',(-1.51301075899711E-11,-120.993984254242,
-8.40164026751963));
#21791=CARTESIAN_POINT('Ctrl Pts',(-4.85068927010199,-120.818984254242,
-8.4016402675109));
#21792=CARTESIAN_POINT('Ctrl Pts',(-7.27603390513785,-120.643984254242,
-4.20082013374671));
#21793=CARTESIAN_POINT('Ctrl Pts',(-9.70137854017372,-120.468984254242,
1.74701493417668E-11));
#21794=CARTESIAN_POINT('Ctrl Pts',(-7.27603390512272,-120.293984254242,
4.20082013377292));
#21795=CARTESIAN_POINT('Ctrl Pts',(-4.85068927007173,-120.118984254242,
8.40164026752836));
#21796=CARTESIAN_POINT('Ctrl Pts',(1.5129078685785E-11,-119.943984254242,
8.40164026751963));
#21797=CARTESIAN_POINT('Ctrl Pts',(4.85068927010198,-119.768984254242,8.4016402675109));
#21798=CARTESIAN_POINT('Ctrl Pts',(7.27603390513785,-119.593984254242,4.20082013374672));
#21799=CARTESIAN_POINT('Ctrl Pts',(9.70137854017372,-119.418984254242,-1.74689612655491E-11));
#21800=CARTESIAN_POINT('Ctrl Pts',(7.27603390512273,-119.243984254242,-4.20082013377291));
#21801=CARTESIAN_POINT('Ctrl Pts',(4.85068927007173,-119.068984254242,-8.40164026752836));
#21802=CARTESIAN_POINT('Ctrl Pts',(-1.51301075899711E-11,-118.893984254242,
-8.40164026751963));
#21803=CARTESIAN_POINT('Ctrl Pts',(-4.85068927010199,-118.718984254242,
-8.4016402675109));
#21804=CARTESIAN_POINT('Ctrl Pts',(-7.27603390513785,-118.543984254242,
-4.20082013374671));
#21805=CARTESIAN_POINT('Ctrl Pts',(-9.70137854017372,-118.368984254242,
1.74701493417668E-11));
#21806=CARTESIAN_POINT('Ctrl Pts',(-7.27603390512272,-118.193984254242,
4.20082013377292));
#21807=CARTESIAN_POINT('Ctrl Pts',(-4.85068927007173,-118.018984254242,
8.40164026752836));
#21808=CARTESIAN_POINT('Ctrl Pts',(1.5129078685785E-11,-117.843984254242,
8.40164026751963));
#21809=CARTESIAN_POINT('Ctrl Pts',(4.85068927010198,-117.668984254242,8.4016402675109));
#21810=CARTESIAN_POINT('Ctrl Pts',(7.27603390513785,-117.493984254242,4.20082013374672));
#21811=CARTESIAN_POINT('Ctrl Pts',(9.70137854017372,-117.318984254242,-1.74689612655491E-11));
#21812=CARTESIAN_POINT('Ctrl Pts',(7.27603390512273,-117.143984254242,-4.20082013377291));
#21813=CARTESIAN_POINT('Ctrl Pts',(4.85068927007173,-116.968984254242,-8.40164026752836));
#21814=CARTESIAN_POINT('Ctrl Pts',(-1.51301075899711E-11,-116.793984254242,
-8.40164026751963));
#21815=CARTESIAN_POINT('Ctrl Pts',(-4.85068927010199,-116.618984254242,
-8.4016402675109));
#21816=CARTESIAN_POINT('Ctrl Pts',(-7.27603390513785,-116.443984254242,
-4.20082013374671));
#21817=CARTESIAN_POINT('Ctrl Pts',(-9.70137854017372,-116.268984254242,
1.74701493417668E-11));
#21818=CARTESIAN_POINT('Ctrl Pts',(-7.27603390512272,-116.093984254242,
4.20082013377292));
#21819=CARTESIAN_POINT('Ctrl Pts',(-4.85068927007173,-115.918984254242,
8.40164026752836));
#21820=CARTESIAN_POINT('Ctrl Pts',(1.5129078685785E-11,-115.743984254242,
8.40164026751963));
#21821=CARTESIAN_POINT('Ctrl Pts',(4.85068927010198,-115.568984254242,8.4016402675109));
#21822=CARTESIAN_POINT('Ctrl Pts',(7.27603390513785,-115.393984254242,4.20082013374672));
#21823=CARTESIAN_POINT('Ctrl Pts',(9.70137854017372,-115.218984254242,-1.74689612655491E-11));
#21824=CARTESIAN_POINT('Ctrl Pts',(7.27603390512273,-115.043984254242,-4.20082013377291));
#21825=CARTESIAN_POINT('Ctrl Pts',(4.85068927007173,-114.868984254242,-8.40164026752836));
#21826=CARTESIAN_POINT('Ctrl Pts',(-1.51301075899711E-11,-114.693984254242,
-8.40164026751963));
#21827=CARTESIAN_POINT('Ctrl Pts',(-4.85068927010199,-114.518984254242,
-8.4016402675109));
#21828=CARTESIAN_POINT('Ctrl Pts',(-7.27603390513785,-114.343984254242,
-4.20082013374671));
#21829=CARTESIAN_POINT('Ctrl Pts',(-9.70137854017372,-114.168984254242,
1.74701493417668E-11));
#21830=CARTESIAN_POINT('Ctrl Pts',(-7.27603390512272,-113.993984254242,
4.20082013377292));
#21831=CARTESIAN_POINT('Ctrl Pts',(-4.85068927007173,-113.818984254242,
8.40164026752836));
#21832=CARTESIAN_POINT('Ctrl Pts',(1.5129078685785E-11,-113.643984254242,
8.40164026751963));
#21833=CARTESIAN_POINT('Ctrl Pts',(4.85068927010198,-113.468984254242,8.4016402675109));
#21834=CARTESIAN_POINT('Ctrl Pts',(7.27603390513785,-113.293984254242,4.20082013374672));
#21835=CARTESIAN_POINT('Ctrl Pts',(9.70137854017372,-113.118984254242,-1.74689612655491E-11));
#21836=CARTESIAN_POINT('Ctrl Pts',(7.27603390512273,-112.943984254242,-4.20082013377291));
#21837=CARTESIAN_POINT('Ctrl Pts',(4.85068927007173,-112.768984254242,-8.40164026752836));
#21838=CARTESIAN_POINT('Ctrl Pts',(-1.51301075899711E-11,-112.593984254242,
-8.40164026751963));
#21839=CARTESIAN_POINT('Ctrl Pts',(-4.85068927010199,-112.418984254242,
-8.4016402675109));
#21840=CARTESIAN_POINT('Ctrl Pts',(-7.27603390513785,-112.243984254242,
-4.20082013374671));
#21841=CARTESIAN_POINT('Ctrl Pts',(-9.70137854017372,-112.068984254242,
1.74701493417668E-11));
#21842=CARTESIAN_POINT('Ctrl Pts',(-7.27603390512272,-111.893984254242,
4.20082013377292));
#21843=CARTESIAN_POINT('Ctrl Pts',(-4.85068927007173,-111.718984254242,
8.40164026752836));
#21844=CARTESIAN_POINT('Ctrl Pts',(1.5129078685785E-11,-111.543984254242,
8.40164026751963));
#21845=CARTESIAN_POINT('Ctrl Pts',(4.85068927010198,-111.368984254242,8.4016402675109));
#21846=CARTESIAN_POINT('Ctrl Pts',(7.27603390513785,-111.193984254242,4.20082013374672));
#21847=CARTESIAN_POINT('Ctrl Pts',(9.70137854017372,-111.018984254242,-1.74689612655491E-11));
#21848=CARTESIAN_POINT('Ctrl Pts',(7.27603390512273,-110.843984254242,-4.20082013377291));
#21849=CARTESIAN_POINT('Ctrl Pts',(4.85068927007173,-110.668984254242,-8.40164026752836));
#21850=CARTESIAN_POINT('Ctrl Pts',(-1.51301075899711E-11,-110.493984254242,
-8.40164026751963));
#21851=CARTESIAN_POINT('Ctrl Pts',(-4.85068927010199,-110.318984254242,
-8.4016402675109));
#21852=CARTESIAN_POINT('Ctrl Pts',(-7.27603390513785,-110.143984254242,
-4.20082013374671));
#21853=CARTESIAN_POINT('Ctrl Pts',(-9.70137854017372,-109.968984254242,
1.74701493417668E-11));
#21854=CARTESIAN_POINT('Ctrl Pts',(-7.27603390512272,-109.793984254242,
4.20082013377292));
#21855=CARTESIAN_POINT('Ctrl Pts',(-4.85068927007173,-109.618984254242,
8.40164026752836));
#21856=CARTESIAN_POINT('Ctrl Pts',(1.5129078685785E-11,-109.443984254242,
8.40164026751963));
#21857=CARTESIAN_POINT('Ctrl Pts',(4.85068927010198,-109.268984254242,8.4016402675109));
#21858=CARTESIAN_POINT('Ctrl Pts',(7.27603390513785,-109.093984254242,4.20082013374672));
#21859=CARTESIAN_POINT('Ctrl Pts',(9.70137854017372,-108.918984254242,-1.74689612655491E-11));
#21860=CARTESIAN_POINT('Ctrl Pts',(7.27603390512273,-108.743984254242,-4.20082013377291));
#21861=CARTESIAN_POINT('Ctrl Pts',(4.85068927007173,-108.568984254242,-8.40164026752836));
#21862=CARTESIAN_POINT('Ctrl Pts',(-1.51301075899711E-11,-108.393984254242,
-8.40164026751963));
#21863=CARTESIAN_POINT('Ctrl Pts',(-4.85068927010199,-108.218984254242,
-8.4016402675109));
#21864=CARTESIAN_POINT('Ctrl Pts',(-7.27603390513785,-108.043984254242,
-4.20082013374671));
#21865=CARTESIAN_POINT('Ctrl Pts',(-9.70137854017372,-107.868984254242,
1.74701493417668E-11));
#21866=CARTESIAN_POINT('Ctrl Pts',(-7.27603390512272,-107.693984254242,
4.20082013377292));
#21867=CARTESIAN_POINT('Ctrl Pts',(-4.85068927007173,-107.518984254242,
8.40164026752836));
#21868=CARTESIAN_POINT('Ctrl Pts',(1.5129078685785E-11,-107.343984254242,
8.40164026751963));
#21869=CARTESIAN_POINT('Ctrl Pts',(4.85068927010198,-107.168984254242,8.4016402675109));
#21870=CARTESIAN_POINT('Ctrl Pts',(7.27603390513785,-106.993984254242,4.20082013374672));
#21871=CARTESIAN_POINT('Ctrl Pts',(9.70137854017372,-106.818984254242,-1.74689612655491E-11));
#21872=CARTESIAN_POINT('Ctrl Pts',(7.27603390512273,-106.643984254242,-4.20082013377291));
#21873=CARTESIAN_POINT('Ctrl Pts',(4.85068927007173,-106.468984254242,-8.40164026752836));
#21874=CARTESIAN_POINT('Ctrl Pts',(-1.51301075899711E-11,-106.293984254242,
-8.40164026751963));
#21875=CARTESIAN_POINT('Ctrl Pts',(-4.85068927010199,-106.118984254242,
-8.4016402675109));
#21876=CARTESIAN_POINT('Ctrl Pts',(-7.27603390513785,-105.943984254242,
-4.20082013374671));
#21877=CARTESIAN_POINT('Ctrl Pts',(-9.70137854017372,-105.768984254242,
1.74701493417668E-11));
#21878=CARTESIAN_POINT('Ctrl Pts',(-7.27603390512272,-105.593984254242,
4.20082013377292));
#21879=CARTESIAN_POINT('Ctrl Pts',(-4.85068927007173,-105.418984254242,
8.40164026752836));
#21880=CARTESIAN_POINT('Ctrl Pts',(1.5129078685785E-11,-105.243984254242,
8.40164026751963));
#21881=CARTESIAN_POINT('Ctrl Pts',(4.85068927010198,-105.068984254242,8.4016402675109));
#21882=CARTESIAN_POINT('Ctrl Pts',(7.27603390513785,-104.893984254242,4.20082013374672));
#21883=CARTESIAN_POINT('Ctrl Pts',(9.70137854017372,-104.718984254242,-1.74689612655491E-11));
#21884=CARTESIAN_POINT('Ctrl Pts',(7.27603390512273,-104.543984254242,-4.20082013377291));
#21885=CARTESIAN_POINT('Ctrl Pts',(4.85068927007173,-104.368984254242,-8.40164026752836));
#21886=CARTESIAN_POINT('Ctrl Pts',(-1.51301075899711E-11,-104.193984254242,
-8.40164026751963));
#21887=CARTESIAN_POINT('Ctrl Pts',(-4.85068927010199,-104.018984254242,
-8.4016402675109));
#21888=CARTESIAN_POINT('Ctrl Pts',(-7.27603390513785,-103.843984254242,
-4.20082013374671));
#21889=CARTESIAN_POINT('Ctrl Pts',(-9.70137854017372,-103.668984254242,
1.74701493417668E-11));
#21890=CARTESIAN_POINT('Ctrl Pts',(-7.27603390512272,-103.493984254242,
4.20082013377292));
#21891=CARTESIAN_POINT('Ctrl Pts',(-4.85068927007173,-103.318984254242,
8.40164026752836));
#21892=CARTESIAN_POINT('Ctrl Pts',(1.5129078685785E-11,-103.143984254242,
8.40164026751963));
#21893=CARTESIAN_POINT('Ctrl Pts',(4.85068927010198,-102.968984254242,8.4016402675109));
#21894=CARTESIAN_POINT('Ctrl Pts',(7.27603390513785,-102.793984254242,4.20082013374672));
#21895=CARTESIAN_POINT('Ctrl Pts',(9.70137854017372,-102.618984254242,-1.74689612655491E-11));
#21896=CARTESIAN_POINT('Ctrl Pts',(7.27603390512273,-102.443984254242,-4.20082013377291));
#21897=CARTESIAN_POINT('Ctrl Pts',(4.85068927007173,-102.268984254242,-8.40164026752836));
#21898=CARTESIAN_POINT('Ctrl Pts',(-1.51301075899711E-11,-102.093984254242,
-8.40164026751963));
#21899=CARTESIAN_POINT('Ctrl Pts',(-4.85068927010199,-101.918984254242,
-8.4016402675109));
#21900=CARTESIAN_POINT('Ctrl Pts',(-7.27603390513785,-101.743984254242,
-4.20082013374671));
#21901=CARTESIAN_POINT('Ctrl Pts',(-9.70137854017372,-101.568984254242,
1.74701493417668E-11));
#21902=CARTESIAN_POINT('Ctrl Pts',(-7.27603390512272,-101.393984254242,
4.20082013377292));
#21903=CARTESIAN_POINT('Ctrl Pts',(-4.85068927007173,-101.218984254242,
8.40164026752836));
#21904=CARTESIAN_POINT('Ctrl Pts',(1.5129078685785E-11,-101.043984254242,
8.40164026751963));
#21905=CARTESIAN_POINT('Ctrl Pts',(4.85068927010198,-100.868984254242,8.4016402675109));
#21906=CARTESIAN_POINT('Ctrl Pts',(7.27603390513785,-100.693984254242,4.20082013374672));
#21907=CARTESIAN_POINT('Ctrl Pts',(9.70137854017372,-100.518984254242,-1.74689612655491E-11));
#21908=CARTESIAN_POINT('Ctrl Pts',(7.27603390512273,-100.343984254242,-4.20082013377291));
#21909=CARTESIAN_POINT('Ctrl Pts',(4.85068927007173,-100.168984254242,-8.40164026752836));
#21910=CARTESIAN_POINT('Ctrl Pts',(-1.51301075899711E-11,-99.9939842542418,
-8.40164026751963));
#21911=CARTESIAN_POINT('Ctrl Pts',(-4.85068927010199,-99.8189842542418,
-8.4016402675109));
#21912=CARTESIAN_POINT('Ctrl Pts',(-7.27603390513785,-99.6439842542417,
-4.20082013374671));
#21913=CARTESIAN_POINT('Ctrl Pts',(-9.70137854017372,-99.4689842542418,
1.74701493417668E-11));
#21914=CARTESIAN_POINT('Ctrl Pts',(-7.27603390512272,-99.2939842542417,
4.20082013377292));
#21915=CARTESIAN_POINT('Ctrl Pts',(-4.85068927007173,-99.1189842542418,
8.40164026752836));
#21916=CARTESIAN_POINT('Ctrl Pts',(1.5129078685785E-11,-98.9439842542418,
8.40164026751963));
#21917=CARTESIAN_POINT('Ctrl Pts',(4.85068927010198,-98.7689842542417,8.4016402675109));
#21918=CARTESIAN_POINT('Ctrl Pts',(7.27603390513785,-98.5939842542417,4.20082013374672));
#21919=CARTESIAN_POINT('Ctrl Pts',(9.70137854017372,-98.4189842542418,-1.74689612655491E-11));
#21920=CARTESIAN_POINT('Ctrl Pts',(7.27603390512273,-98.2439842542418,-4.20082013377291));
#21921=CARTESIAN_POINT('Ctrl Pts',(4.85068927007173,-98.0689842542417,-8.40164026752836));
#21922=CARTESIAN_POINT('Ctrl Pts',(-1.51301075899711E-11,-97.8939842542418,
-8.40164026751963));
#21923=CARTESIAN_POINT('Ctrl Pts',(-4.85068927010199,-97.7189842542418,
-8.4016402675109));
#21924=CARTESIAN_POINT('Ctrl Pts',(-7.27603390513785,-97.5439842542417,
-4.20082013374671));
#21925=CARTESIAN_POINT('Ctrl Pts',(-9.70137854017372,-97.3689842542418,
1.74701493417668E-11));
#21926=CARTESIAN_POINT('Ctrl Pts',(-7.27603390512272,-97.1939842542418,
4.20082013377292));
#21927=CARTESIAN_POINT('Ctrl Pts',(-4.85068927007173,-97.0189842542418,
8.40164026752836));
#21928=CARTESIAN_POINT('Ctrl Pts',(1.5129078685785E-11,-96.8439842542418,
8.40164026751963));
#21929=CARTESIAN_POINT('Ctrl Pts',(4.85068927010198,-96.6689842542418,8.4016402675109));
#21930=CARTESIAN_POINT('Ctrl Pts',(7.27603390513785,-96.4939842542417,4.20082013374672));
#21931=CARTESIAN_POINT('Ctrl Pts',(9.70137854017372,-96.3189842542418,-1.74689612655491E-11));
#21932=CARTESIAN_POINT('Ctrl Pts',(7.27603390512273,-96.1439842542418,-4.20082013377291));
#21933=CARTESIAN_POINT('Ctrl Pts',(4.85068927007173,-95.9689842542417,-8.40164026752836));
#21934=CARTESIAN_POINT('Ctrl Pts',(-1.51301075899711E-11,-95.7939842542418,
-8.40164026751963));
#21935=CARTESIAN_POINT('Ctrl Pts',(-4.85068927010199,-95.6189842542418,
-8.4016402675109));
#21936=CARTESIAN_POINT('Ctrl Pts',(-7.27603390513785,-95.4439842542418,
-4.20082013374671));
#21937=CARTESIAN_POINT('Ctrl Pts',(-9.70137854017372,-95.2689842542418,
1.74701493417668E-11));
#21938=CARTESIAN_POINT('Ctrl Pts',(-7.27603390512272,-95.0939842542418,
4.20082013377292));
#21939=CARTESIAN_POINT('Ctrl Pts',(-4.85068927007173,-94.9189842542418,
8.40164026752836));
#21940=CARTESIAN_POINT('Ctrl Pts',(1.5129078685785E-11,-94.7439842542418,
8.40164026751963));
#21941=CARTESIAN_POINT('Ctrl Pts',(4.85068927010198,-94.5689842542417,8.4016402675109));
#21942=CARTESIAN_POINT('Ctrl Pts',(7.27603390513785,-94.3939842542418,4.20082013374672));
#21943=CARTESIAN_POINT('Ctrl Pts',(9.70137854017372,-94.2189842542417,-1.74689612655491E-11));
#21944=CARTESIAN_POINT('Ctrl Pts',(7.27603390512273,-94.0439842542417,-4.20082013377291));
#21945=CARTESIAN_POINT('Ctrl Pts',(4.85068927007173,-93.8689842542418,-8.40164026752836));
#21946=CARTESIAN_POINT('Ctrl Pts',(-1.51301075899711E-11,-93.6939842542417,
-8.40164026751963));
#21947=CARTESIAN_POINT('Ctrl Pts',(-4.85068927010199,-93.5189842542417,
-8.4016402675109));
#21948=CARTESIAN_POINT('Ctrl Pts',(-7.27603390513785,-93.3439842542418,
-4.20082013374671));
#21949=CARTESIAN_POINT('Ctrl Pts',(-9.70137854017372,-93.1689842542418,
1.74701493417668E-11));
#21950=CARTESIAN_POINT('Ctrl Pts',(-7.27603390512272,-92.9939842542417,
4.20082013377292));
#21951=CARTESIAN_POINT('Ctrl Pts',(-4.85068927007173,-92.8189842542418,
8.40164026752836));
#21952=CARTESIAN_POINT('Ctrl Pts',(1.5129078685785E-11,-92.6439842542418,
8.40164026751963));
#21953=CARTESIAN_POINT('Ctrl Pts',(4.85068927010198,-92.4689842542418,8.4016402675109));
#21954=CARTESIAN_POINT('Ctrl Pts',(7.27603390513785,-92.2939842542418,4.20082013374672));
#21955=CARTESIAN_POINT('Ctrl Pts',(9.70137854017372,-92.1189842542418,-1.74689612655491E-11));
#21956=CARTESIAN_POINT('Ctrl Pts',(7.27603390512273,-91.9439842542417,-4.20082013377291));
#21957=CARTESIAN_POINT('Ctrl Pts',(4.85068927007173,-91.7689842542418,-8.40164026752836));
#21958=CARTESIAN_POINT('Ctrl Pts',(-1.51301075899711E-11,-91.5939842542418,
-8.40164026751963));
#21959=CARTESIAN_POINT('Ctrl Pts',(-4.85068927010199,-91.4189842542417,
-8.4016402675109));
#21960=CARTESIAN_POINT('Ctrl Pts',(-7.27603390513785,-91.2439842542418,
-4.20082013374671));
#21961=CARTESIAN_POINT('Ctrl Pts',(-9.70137854017372,-91.0689842542418,
1.74701493417668E-11));
#21962=CARTESIAN_POINT('Ctrl Pts',(-7.27603390512272,-90.8939842542418,
4.20082013377292));
#21963=CARTESIAN_POINT('Ctrl Pts',(-4.85068927007173,-90.7189842542418,
8.40164026752836));
#21964=CARTESIAN_POINT('Ctrl Pts',(1.5129078685785E-11,-90.5439842542418,
8.40164026751963));
#21965=CARTESIAN_POINT('Ctrl Pts',(4.85068927010198,-90.3689842542418,8.4016402675109));
#21966=CARTESIAN_POINT('Ctrl Pts',(7.27603390513785,-90.1939842542418,4.20082013374672));
#21967=CARTESIAN_POINT('Ctrl Pts',(9.70137854017372,-90.0189842542418,-1.74689612655491E-11));
#21968=CARTESIAN_POINT('Ctrl Pts',(7.27603390512273,-89.8439842542418,-4.20082013377291));
#21969=CARTESIAN_POINT('Ctrl Pts',(4.85068927007173,-89.6689842542418,-8.40164026752836));
#21970=CARTESIAN_POINT('Ctrl Pts',(-1.51301075899711E-11,-89.4939842542418,
-8.40164026751963));
#21971=CARTESIAN_POINT('Ctrl Pts',(-4.85068927010199,-89.3189842542418,
-8.4016402675109));
#21972=CARTESIAN_POINT('Ctrl Pts',(-7.27603390513785,-89.1439842542418,
-4.20082013374671));
#21973=CARTESIAN_POINT('Ctrl Pts',(-9.70137854017372,-88.9689842542418,
1.74701493417668E-11));
#21974=CARTESIAN_POINT('Ctrl Pts',(-7.27603390512272,-88.7939842542418,
4.20082013377292));
#21975=CARTESIAN_POINT('Ctrl Pts',(-4.85068927007173,-88.6189842542418,
8.40164026752836));
#21976=CARTESIAN_POINT('Ctrl Pts',(1.5129078685785E-11,-88.4439842542418,
8.40164026751963));
#21977=CARTESIAN_POINT('Ctrl Pts',(4.85068927010198,-88.2689842542418,8.4016402675109));
#21978=CARTESIAN_POINT('Ctrl Pts',(7.27603390513785,-88.0939842542418,4.20082013374672));
#21979=CARTESIAN_POINT('Ctrl Pts',(9.70137854017372,-87.9189842542418,-1.74689612655491E-11));
#21980=CARTESIAN_POINT('Ctrl Pts',(7.27603390512273,-87.7439842542418,-4.20082013377291));
#21981=CARTESIAN_POINT('Ctrl Pts',(4.85068927007173,-87.5689842542418,-8.40164026752836));
#21982=CARTESIAN_POINT('Ctrl Pts',(-1.51301075899711E-11,-87.3939842542418,
-8.40164026751963));
#21983=CARTESIAN_POINT('Ctrl Pts',(-4.85068927010199,-87.2189842542418,
-8.4016402675109));
#21984=CARTESIAN_POINT('Ctrl Pts',(-7.27603390513785,-87.0439842542418,
-4.20082013374671));
#21985=CARTESIAN_POINT('Ctrl Pts',(-9.70137854017372,-86.8689842542418,
1.74701493417668E-11));
#21986=CARTESIAN_POINT('Ctrl Pts',(-7.27603390512272,-86.6939842542418,
4.20082013377292));
#21987=CARTESIAN_POINT('Ctrl Pts',(-4.85068927007173,-86.5189842542418,
8.40164026752836));
#21988=CARTESIAN_POINT('Ctrl Pts',(1.5129078685785E-11,-86.3439842542418,
8.40164026751963));
#21989=CARTESIAN_POINT('Ctrl Pts',(4.85068927010198,-86.1689842542418,8.4016402675109));
#21990=CARTESIAN_POINT('Ctrl Pts',(7.27603390513785,-85.9939842542418,4.20082013374672));
#21991=CARTESIAN_POINT('Ctrl Pts',(9.70137854017372,-85.8189842542418,-1.74689612655491E-11));
#21992=CARTESIAN_POINT('Ctrl Pts',(7.27603390512273,-85.6439842542418,-4.20082013377291));
#21993=CARTESIAN_POINT('Ctrl Pts',(4.85068927007173,-85.4689842542418,-8.40164026752836));
#21994=CARTESIAN_POINT('Ctrl Pts',(-1.51301075899711E-11,-85.2939842542417,
-8.40164026751963));
#21995=CARTESIAN_POINT('Ctrl Pts',(-4.85068927010199,-85.1189842542418,
-8.4016402675109));
#21996=CARTESIAN_POINT('Ctrl Pts',(-7.27603390513785,-84.9439842542418,
-4.20082013374671));
#21997=CARTESIAN_POINT('Ctrl Pts',(-9.70137854017372,-84.7689842542418,
1.74701493417668E-11));
#21998=CARTESIAN_POINT('Ctrl Pts',(-7.27603390512272,-84.5939842542418,
4.20082013377292));
#21999=CARTESIAN_POINT('Ctrl Pts',(-4.85068927007173,-84.4189842542418,
8.40164026752836));
#22000=CARTESIAN_POINT('Ctrl Pts',(1.5129078685785E-11,-84.2439842542418,
8.40164026751963));
#22001=CARTESIAN_POINT('Ctrl Pts',(4.85068927010198,-84.0689842542418,8.4016402675109));
#22002=CARTESIAN_POINT('Ctrl Pts',(7.27603390513785,-83.8939842542418,4.20082013374672));
#22003=CARTESIAN_POINT('Ctrl Pts',(9.70137854017372,-83.7189842542418,-1.74689612655491E-11));
#22004=CARTESIAN_POINT('Ctrl Pts',(7.27603390512273,-83.5439842542418,-4.20082013377291));
#22005=CARTESIAN_POINT('Ctrl Pts',(4.85068927007173,-83.3689842542418,-8.40164026752836));
#22006=CARTESIAN_POINT('Ctrl Pts',(-1.51301075899711E-11,-83.1939842542418,
-8.40164026751963));
#22007=CARTESIAN_POINT('Ctrl Pts',(-4.85068927010199,-83.0189842542418,
-8.4016402675109));
#22008=CARTESIAN_POINT('Ctrl Pts',(-7.27603390513785,-82.8439842542418,
-4.20082013374671));
#22009=CARTESIAN_POINT('Ctrl Pts',(-9.70137854017372,-82.6689842542418,
1.74701493417668E-11));
#22010=CARTESIAN_POINT('Ctrl Pts',(-7.27603390512272,-82.4939842542418,
4.20082013377292));
#22011=CARTESIAN_POINT('Ctrl Pts',(-4.85068927007173,-82.3189842542418,
8.40164026752836));
#22012=CARTESIAN_POINT('Ctrl Pts',(1.5129078685785E-11,-82.1439842542418,
8.40164026751963));
#22013=CARTESIAN_POINT('Ctrl Pts',(4.85068927010198,-81.9689842542418,8.4016402675109));
#22014=CARTESIAN_POINT('Ctrl Pts',(7.27603390513785,-81.7939842542418,4.20082013374672));
#22015=CARTESIAN_POINT('Ctrl Pts',(9.70137854017372,-81.6189842542418,-1.74689612655491E-11));
#22016=CARTESIAN_POINT('Ctrl Pts',(7.27603390512273,-81.4439842542418,-4.20082013377291));
#22017=CARTESIAN_POINT('Ctrl Pts',(4.85068927007173,-81.2689842542418,-8.40164026752836));
#22018=CARTESIAN_POINT('Ctrl Pts',(-1.51301075899711E-11,-81.0939842542418,
-8.40164026751963));
#22019=CARTESIAN_POINT('Ctrl Pts',(-4.85068927010199,-80.9189842542418,
-8.4016402675109));
#22020=CARTESIAN_POINT('Ctrl Pts',(-7.27603390513785,-80.7439842542418,
-4.20082013374671));
#22021=CARTESIAN_POINT('Ctrl Pts',(-9.70137854017372,-80.5689842542418,
1.74701493417668E-11));
#22022=CARTESIAN_POINT('Ctrl Pts',(-7.27603390512272,-80.3939842542418,
4.20082013377292));
#22023=CARTESIAN_POINT('Ctrl Pts',(-4.85068927007173,-80.2189842542418,
8.40164026752836));
#22024=CARTESIAN_POINT('Ctrl Pts',(1.5129078685785E-11,-80.0439842542418,
8.40164026751963));
#22025=CARTESIAN_POINT('Ctrl Pts',(4.85068927010198,-79.8689842542418,8.4016402675109));
#22026=CARTESIAN_POINT('Ctrl Pts',(7.27603390513785,-79.6939842542418,4.20082013374672));
#22027=CARTESIAN_POINT('Ctrl Pts',(9.70137854017372,-79.5189842542418,-1.74689612655491E-11));
#22028=CARTESIAN_POINT('Ctrl Pts',(7.27603390512273,-79.3439842542418,-4.20082013377291));
#22029=CARTESIAN_POINT('Ctrl Pts',(4.85068927007173,-79.1689842542418,-8.40164026752836));
#22030=CARTESIAN_POINT('Ctrl Pts',(-1.51301075899711E-11,-78.9939842542418,
-8.40164026751963));
#22031=CARTESIAN_POINT('Ctrl Pts',(-4.85068927010199,-78.8189842542418,
-8.4016402675109));
#22032=CARTESIAN_POINT('Ctrl Pts',(-7.27603390513785,-78.6439842542418,
-4.20082013374671));
#22033=CARTESIAN_POINT('Ctrl Pts',(-9.70137854017372,-78.4689842542418,
1.74701493417668E-11));
#22034=CARTESIAN_POINT('Ctrl Pts',(-7.27603390512272,-78.2939842542418,
4.20082013377292));
#22035=CARTESIAN_POINT('Ctrl Pts',(-4.85068927007173,-78.1189842542418,
8.40164026752836));
#22036=CARTESIAN_POINT('Ctrl Pts',(1.5129078685785E-11,-77.9439842542418,
8.40164026751963));
#22037=CARTESIAN_POINT('Ctrl Pts',(4.85068927010198,-77.7689842542418,8.4016402675109));
#22038=CARTESIAN_POINT('Ctrl Pts',(7.27603390513785,-77.5939842542418,4.20082013374672));
#22039=CARTESIAN_POINT('Ctrl Pts',(9.70137854017372,-77.4189842542418,-1.74689612655491E-11));
#22040=CARTESIAN_POINT('Ctrl Pts',(7.27603390512273,-77.2439842542418,-4.20082013377291));
#22041=CARTESIAN_POINT('Ctrl Pts',(4.85068927007173,-77.0689842542418,-8.40164026752836));
#22042=CARTESIAN_POINT('Ctrl Pts',(-1.51301075899711E-11,-76.8939842542418,
-8.40164026751963));
#22043=CARTESIAN_POINT('Ctrl Pts',(-4.85068927010199,-76.7189842542418,
-8.4016402675109));
#22044=CARTESIAN_POINT('Ctrl Pts',(-7.27603390513785,-76.5439842542418,
-4.20082013374671));
#22045=CARTESIAN_POINT('Ctrl Pts',(-9.70137854017372,-76.3689842542418,
1.74701493417668E-11));
#22046=CARTESIAN_POINT('Ctrl Pts',(-7.27603390512272,-76.1939842542418,
4.20082013377292));
#22047=CARTESIAN_POINT('Ctrl Pts',(-4.85068927007173,-76.0189842542418,
8.40164026752836));
#22048=CARTESIAN_POINT('Ctrl Pts',(1.5129078685785E-11,-75.8439842542418,
8.40164026751963));
#22049=CARTESIAN_POINT('Ctrl Pts',(4.85068927010198,-75.6689842542418,8.4016402675109));
#22050=CARTESIAN_POINT('Ctrl Pts',(7.27603390513785,-75.4939842542418,4.20082013374672));
#22051=CARTESIAN_POINT('Ctrl Pts',(9.70137854017372,-75.3189842542418,-1.74689612655491E-11));
#22052=CARTESIAN_POINT('Ctrl Pts',(7.27603390512273,-75.1439842542418,-4.20082013377291));
#22053=CARTESIAN_POINT('Ctrl Pts',(4.85068927007173,-74.9689842542418,-8.40164026752836));
#22054=CARTESIAN_POINT('Ctrl Pts',(-1.51301075899711E-11,-74.7939842542418,
-8.40164026751963));
#22055=CARTESIAN_POINT('Ctrl Pts',(-4.85068927010199,-74.6189842542418,
-8.4016402675109));
#22056=CARTESIAN_POINT('Ctrl Pts',(-7.27603390513785,-74.4439842542418,
-4.20082013374671));
#22057=CARTESIAN_POINT('Ctrl Pts',(-9.70137854017372,-74.2689842542418,
1.74701493417668E-11));
#22058=CARTESIAN_POINT('Ctrl Pts',(-7.27603390512272,-74.0939842542418,
4.20082013377292));
#22059=CARTESIAN_POINT('Ctrl Pts',(-4.85068927007173,-73.9189842542418,
8.40164026752836));
#22060=CARTESIAN_POINT('Ctrl Pts',(1.5129078685785E-11,-73.7439842542418,
8.40164026751963));
#22061=CARTESIAN_POINT('Ctrl Pts',(4.85068927010198,-73.5689842542418,8.4016402675109));
#22062=CARTESIAN_POINT('Ctrl Pts',(7.27603390513785,-73.3939842542418,4.20082013374672));
#22063=CARTESIAN_POINT('Ctrl Pts',(9.70137854017372,-73.2189842542418,-1.74689612655491E-11));
#22064=CARTESIAN_POINT('Ctrl Pts',(7.27603390512273,-73.0439842542418,-4.20082013377291));
#22065=CARTESIAN_POINT('Ctrl Pts',(4.85068927007173,-72.8689842542418,-8.40164026752836));
#22066=CARTESIAN_POINT('Ctrl Pts',(-1.51301075899711E-11,-72.6939842542418,
-8.40164026751963));
#22067=CARTESIAN_POINT('Ctrl Pts',(-4.85068927010199,-72.5189842542418,
-8.4016402675109));
#22068=CARTESIAN_POINT('Ctrl Pts',(-7.27603390513785,-72.3439842542418,
-4.20082013374671));
#22069=CARTESIAN_POINT('Ctrl Pts',(-9.70137854017372,-72.1689842542418,
1.74701493417668E-11));
#22070=CARTESIAN_POINT('Ctrl Pts',(-7.27603390512272,-71.9939842542418,
4.20082013377292));
#22071=CARTESIAN_POINT('Ctrl Pts',(-4.85068927007173,-71.8189842542418,
8.40164026752836));
#22072=CARTESIAN_POINT('Ctrl Pts',(1.5129078685785E-11,-71.6439842542418,
8.40164026751963));
#22073=CARTESIAN_POINT('Ctrl Pts',(4.85068927010198,-71.4689842542418,8.4016402675109));
#22074=CARTESIAN_POINT('Ctrl Pts',(7.27603390513785,-71.2939842542418,4.20082013374672));
#22075=CARTESIAN_POINT('Ctrl Pts',(9.70137854017372,-71.1189842542418,-1.74689612655491E-11));
#22076=CARTESIAN_POINT('Ctrl Pts',(7.27603390512273,-70.9439842542418,-4.20082013377291));
#22077=CARTESIAN_POINT('Ctrl Pts',(4.85068927007173,-70.7689842542418,-8.40164026752836));
#22078=CARTESIAN_POINT('Ctrl Pts',(-1.51301075899711E-11,-70.5939842542418,
-8.40164026751963));
#22079=CARTESIAN_POINT('Ctrl Pts',(-4.85068927010199,-70.4189842542418,
-8.4016402675109));
#22080=CARTESIAN_POINT('Ctrl Pts',(-7.27603390513785,-70.2439842542418,
-4.20082013374671));
#22081=CARTESIAN_POINT('Ctrl Pts',(-9.70137854017372,-70.0689842542418,
1.74701493417668E-11));
#22082=CARTESIAN_POINT('Ctrl Pts',(-7.27603390512272,-69.8939842542418,
4.20082013377292));
#22083=CARTESIAN_POINT('Ctrl Pts',(-4.85068927007173,-69.7189842542418,
8.40164026752836));
#22084=CARTESIAN_POINT('Ctrl Pts',(1.5129078685785E-11,-69.5439842542418,
8.40164026751963));
#22085=CARTESIAN_POINT('Ctrl Pts',(4.85068927010198,-69.3689842542418,8.4016402675109));
#22086=CARTESIAN_POINT('Ctrl Pts',(7.27603390513785,-69.1939842542418,4.20082013374672));
#22087=CARTESIAN_POINT('Ctrl Pts',(9.70137854017372,-69.0189842542418,-1.74689612655491E-11));
#22088=CARTESIAN_POINT('Ctrl Pts',(7.27603390512273,-68.8439842542418,-4.20082013377291));
#22089=CARTESIAN_POINT('Ctrl Pts',(4.85068927007173,-68.6689842542418,-8.40164026752836));
#22090=CARTESIAN_POINT('Ctrl Pts',(-1.51301075899711E-11,-68.4939842542418,
-8.40164026751963));
#22091=CARTESIAN_POINT('Ctrl Pts',(-4.85068927010199,-68.3189842542418,
-8.4016402675109));
#22092=CARTESIAN_POINT('Ctrl Pts',(-7.27603390513785,-68.1439842542418,
-4.20082013374671));
#22093=CARTESIAN_POINT('Ctrl Pts',(-9.70137854017372,-67.9689842542418,
1.74701493417668E-11));
#22094=CARTESIAN_POINT('Ctrl Pts',(-7.27603390512272,-67.7939842542418,
4.20082013377292));
#22095=CARTESIAN_POINT('Ctrl Pts',(-4.85068927007173,-67.6189842542418,
8.40164026752836));
#22096=CARTESIAN_POINT('Ctrl Pts',(1.5129078685785E-11,-67.4439842542418,
8.40164026751963));
#22097=CARTESIAN_POINT('Ctrl Pts',(4.85068927010198,-67.2689842542418,8.4016402675109));
#22098=CARTESIAN_POINT('Ctrl Pts',(7.27603390513785,-67.0939842542418,4.20082013374672));
#22099=CARTESIAN_POINT('Ctrl Pts',(9.70137854017372,-66.9189842542418,-1.74689612655491E-11));
#22100=CARTESIAN_POINT('Ctrl Pts',(7.27603390512273,-66.7439842542418,-4.20082013377291));
#22101=CARTESIAN_POINT('Ctrl Pts',(4.85068927007173,-66.5689842542419,-8.40164026752836));
#22102=CARTESIAN_POINT('Ctrl Pts',(-1.51301075899711E-11,-66.3939842542418,
-8.40164026751963));
#22103=CARTESIAN_POINT('Ctrl Pts',(-4.85068927010199,-66.2189842542418,
-8.4016402675109));
#22104=CARTESIAN_POINT('Ctrl Pts',(-7.27603390513785,-66.0439842542418,
-4.20082013374671));
#22105=CARTESIAN_POINT('Ctrl Pts',(-9.70137854017372,-65.8689842542418,
1.74701493417668E-11));
#22106=CARTESIAN_POINT('Ctrl Pts',(-7.27603390512272,-65.6939842542418,
4.20082013377292));
#22107=CARTESIAN_POINT('Ctrl Pts',(-4.85068927007173,-65.5189842542418,
8.40164026752836));
#22108=CARTESIAN_POINT('Ctrl Pts',(1.5129078685785E-11,-65.3439842542418,
8.40164026751963));
#22109=CARTESIAN_POINT('Ctrl Pts',(4.85068927010198,-65.1689842542418,8.4016402675109));
#22110=CARTESIAN_POINT('Ctrl Pts',(7.27603390513785,-64.9939842542418,4.20082013374672));
#22111=CARTESIAN_POINT('Ctrl Pts',(9.70137854017372,-64.8189842542418,-1.74689612655491E-11));
#22112=CARTESIAN_POINT('Ctrl Pts',(7.27603390512273,-64.6439842542418,-4.20082013377291));
#22113=CARTESIAN_POINT('Ctrl Pts',(4.85068927007173,-64.4689842542418,-8.40164026752836));
#22114=CARTESIAN_POINT('Ctrl Pts',(-1.51301075899711E-11,-64.2939842542418,
-8.40164026751963));
#22115=CARTESIAN_POINT('Ctrl Pts',(-4.85068927010199,-64.1189842542418,
-8.4016402675109));
#22116=CARTESIAN_POINT('Ctrl Pts',(-7.27603390513785,-63.9439842542418,
-4.20082013374671));
#22117=CARTESIAN_POINT('Ctrl Pts',(-9.70137854017372,-63.7689842542418,
1.74701493417668E-11));
#22118=CARTESIAN_POINT('Ctrl Pts',(-7.27603390512272,-63.5939842542418,
4.20082013377292));
#22119=CARTESIAN_POINT('Ctrl Pts',(-4.85068927007173,-63.4189842542418,
8.40164026752836));
#22120=CARTESIAN_POINT('Ctrl Pts',(1.5129078685785E-11,-63.2439842542418,
8.40164026751963));
#22121=CARTESIAN_POINT('Ctrl Pts',(4.85068927010198,-63.0689842542418,8.4016402675109));
#22122=CARTESIAN_POINT('Ctrl Pts',(7.27603390513785,-62.8939842542418,4.20082013374672));
#22123=CARTESIAN_POINT('Ctrl Pts',(9.70137854017372,-62.7189842542418,-1.74689612655491E-11));
#22124=CARTESIAN_POINT('Ctrl Pts',(7.27603390512273,-62.5439842542418,-4.20082013377291));
#22125=CARTESIAN_POINT('Ctrl Pts',(4.85068927007173,-62.3689842542419,-8.40164026752836));
#22126=CARTESIAN_POINT('Ctrl Pts',(-1.51301075899711E-11,-62.1939842542418,
-8.40164026751963));
#22127=CARTESIAN_POINT('Ctrl Pts',(-4.85068927010199,-62.0189842542418,
-8.4016402675109));
#22128=CARTESIAN_POINT('Ctrl Pts',(-7.27603390513785,-61.8439842542418,
-4.20082013374671));
#22129=CARTESIAN_POINT('Ctrl Pts',(-9.70137854017372,-61.6689842542418,
1.74701493417668E-11));
#22130=CARTESIAN_POINT('Ctrl Pts',(-7.27603390512272,-61.4939842542418,
4.20082013377292));
#22131=CARTESIAN_POINT('Ctrl Pts',(-4.85068927007173,-61.3189842542419,
8.40164026752836));
#22132=CARTESIAN_POINT('Ctrl Pts',(1.5129078685785E-11,-61.1439842542418,
8.40164026751963));
#22133=CARTESIAN_POINT('Ctrl Pts',(4.85068927010198,-60.9689842542418,8.4016402675109));
#22134=CARTESIAN_POINT('Ctrl Pts',(7.27603390513785,-60.7939842542418,4.20082013374672));
#22135=CARTESIAN_POINT('Ctrl Pts',(9.70137854017372,-60.6189842542418,-1.74689612655491E-11));
#22136=CARTESIAN_POINT('Ctrl Pts',(7.27603390512273,-60.4439842542418,-4.20082013377291));
#22137=CARTESIAN_POINT('Ctrl Pts',(4.85068927007173,-60.2689842542419,-8.40164026752836));
#22138=CARTESIAN_POINT('Ctrl Pts',(-1.51301075899711E-11,-60.0939842542418,
-8.40164026751963));
#22139=CARTESIAN_POINT('Ctrl Pts',(-4.85068927010199,-59.9189842542418,
-8.4016402675109));
#22140=CARTESIAN_POINT('Ctrl Pts',(-7.27603390513785,-59.7439842542419,
-4.20082013374671));
#22141=CARTESIAN_POINT('Ctrl Pts',(-9.70137854017372,-59.5689842542418,
1.74701493417668E-11));
#22142=CARTESIAN_POINT('Ctrl Pts',(-7.27603390512272,-59.3939842542418,
4.20082013377292));
#22143=CARTESIAN_POINT('Ctrl Pts',(-4.85068927007173,-59.2189842542419,
8.40164026752836));
#22144=CARTESIAN_POINT('Ctrl Pts',(1.5129078685785E-11,-59.0439842542418,
8.40164026751963));
#22145=CARTESIAN_POINT('Ctrl Pts',(4.85068927010198,-58.8689842542419,8.4016402675109));
#22146=CARTESIAN_POINT('Ctrl Pts',(7.27603390513785,-58.6939842542419,4.20082013374672));
#22147=CARTESIAN_POINT('Ctrl Pts',(9.70137854017372,-58.5189842542418,-1.74689612655491E-11));
#22148=CARTESIAN_POINT('Ctrl Pts',(7.27603390512273,-58.3439842542418,-4.20082013377291));
#22149=CARTESIAN_POINT('Ctrl Pts',(4.85068927007173,-58.1689842542419,-8.40164026752836));
#22150=CARTESIAN_POINT('Ctrl Pts',(-1.51301075899711E-11,-57.9939842542418,
-8.40164026751963));
#22151=CARTESIAN_POINT('Ctrl Pts',(-4.85068927010199,-57.8189842542418,
-8.4016402675109));
#22152=CARTESIAN_POINT('Ctrl Pts',(-7.27603390513785,-57.6439842542418,
-4.20082013374671));
#22153=CARTESIAN_POINT('Ctrl Pts',(-9.70137854017372,-57.4689842542418,
1.74701493417668E-11));
#22154=CARTESIAN_POINT('Ctrl Pts',(-7.27603390512272,-57.2939842542418,
4.20082013377292));
#22155=CARTESIAN_POINT('Ctrl Pts',(-4.85068927007173,-57.1189842542418,
8.40164026752836));
#22156=CARTESIAN_POINT('Ctrl Pts',(1.5129078685785E-11,-56.9439842542418,
8.40164026751963));
#22157=CARTESIAN_POINT('Ctrl Pts',(4.85068927010198,-56.7689842542419,8.4016402675109));
#22158=CARTESIAN_POINT('Ctrl Pts',(7.27603390513785,-56.5939842542418,4.20082013374672));
#22159=CARTESIAN_POINT('Ctrl Pts',(9.70137854017372,-56.4189842542418,-1.74689612655491E-11));
#22160=CARTESIAN_POINT('Ctrl Pts',(7.27603390512273,-56.2439842542419,-4.20082013377291));
#22161=CARTESIAN_POINT('Ctrl Pts',(4.85068927007173,-56.0689842542418,-8.40164026752836));
#22162=CARTESIAN_POINT('Ctrl Pts',(-1.51301075899711E-11,-55.8939842542418,
-8.40164026751963));
#22163=CARTESIAN_POINT('Ctrl Pts',(-4.85068927010199,-55.7189842542419,
-8.4016402675109));
#22164=CARTESIAN_POINT('Ctrl Pts',(-7.27603390513785,-55.5439842542418,
-4.20082013374671));
#22165=CARTESIAN_POINT('Ctrl Pts',(-9.70137854017372,-55.3689842542418,
1.74701493417668E-11));
#22166=CARTESIAN_POINT('Ctrl Pts',(-7.27603390512272,-55.1939842542419,
4.20082013377292));
#22167=CARTESIAN_POINT('Ctrl Pts',(-4.85068927007173,-55.0189842542419,
8.40164026752836));
#22168=CARTESIAN_POINT('Ctrl Pts',(1.5129078685785E-11,-54.8439842542419,
8.40164026751963));
#22169=CARTESIAN_POINT('Ctrl Pts',(4.85068927010198,-54.6689842542418,8.4016402675109));
#22170=CARTESIAN_POINT('Ctrl Pts',(7.27603390513785,-54.4939842542419,4.20082013374672));
#22171=CARTESIAN_POINT('Ctrl Pts',(9.70137854017372,-54.3189842542419,-1.74689612655491E-11));
#22172=CARTESIAN_POINT('Ctrl Pts',(7.27603390512273,-54.1439842542419,-4.20082013377291));
#22173=CARTESIAN_POINT('Ctrl Pts',(4.85068927007173,-53.9689842542419,-8.40164026752836));
#22174=CARTESIAN_POINT('Ctrl Pts',(-1.51301075899711E-11,-53.7939842542419,
-8.40164026751963));
#22175=CARTESIAN_POINT('Ctrl Pts',(-4.85068927010199,-53.6189842542419,
-8.4016402675109));
#22176=CARTESIAN_POINT('Ctrl Pts',(-7.27603390513785,-53.4439842542418,
-4.20082013374671));
#22177=CARTESIAN_POINT('Ctrl Pts',(-9.70137854017372,-53.2689842542418,
1.74701493417668E-11));
#22178=CARTESIAN_POINT('Ctrl Pts',(-7.27603390512272,-53.0939842542418,
4.20082013377292));
#22179=CARTESIAN_POINT('Ctrl Pts',(-4.85068927007173,-52.9189842542419,
8.40164026752836));
#22180=CARTESIAN_POINT('Ctrl Pts',(1.5129078685785E-11,-52.7439842542418,
8.40164026751963));
#22181=CARTESIAN_POINT('Ctrl Pts',(4.85068927010198,-52.5689842542419,8.4016402675109));
#22182=CARTESIAN_POINT('Ctrl Pts',(7.27603390513785,-52.3939842542419,4.20082013374672));
#22183=CARTESIAN_POINT('Ctrl Pts',(9.70137854017372,-52.2189842542419,-1.74689612655491E-11));
#22184=CARTESIAN_POINT('Ctrl Pts',(7.27603390512273,-52.0439842542418,-4.20082013377291));
#22185=CARTESIAN_POINT('Ctrl Pts',(4.85068927007173,-51.8689842542419,-8.40164026752836));
#22186=CARTESIAN_POINT('Ctrl Pts',(-1.51301075899711E-11,-51.6939842542418,
-8.40164026751963));
#22187=CARTESIAN_POINT('Ctrl Pts',(-4.85068927010199,-51.5189842542419,
-8.4016402675109));
#22188=CARTESIAN_POINT('Ctrl Pts',(-7.27603390513785,-51.3439842542419,
-4.20082013374671));
#22189=CARTESIAN_POINT('Ctrl Pts',(-9.70137854017372,-51.1689842542419,
1.74701493417668E-11));
#22190=CARTESIAN_POINT('Ctrl Pts',(-7.27603390512272,-50.9939842542419,
4.20082013377292));
#22191=CARTESIAN_POINT('Ctrl Pts',(-4.85068927007173,-50.8189842542419,
8.40164026752836));
#22192=CARTESIAN_POINT('Ctrl Pts',(1.5129078685785E-11,-50.6439842542419,
8.40164026751963));
#22193=CARTESIAN_POINT('Ctrl Pts',(4.85068927010198,-50.4689842542419,8.4016402675109));
#22194=CARTESIAN_POINT('Ctrl Pts',(7.27603390513785,-50.2939842542418,4.20082013374672));
#22195=CARTESIAN_POINT('Ctrl Pts',(9.70137854017372,-50.1189842542419,-1.74689612655491E-11));
#22196=CARTESIAN_POINT('Ctrl Pts',(7.27603390512273,-49.9439842542419,-4.20082013377291));
#22197=CARTESIAN_POINT('Ctrl Pts',(4.85068927007173,-49.7689842542419,-8.40164026752836));
#22198=CARTESIAN_POINT('Ctrl Pts',(-1.51301075899711E-11,-49.5939842542419,
-8.40164026751963));
#22199=CARTESIAN_POINT('Ctrl Pts',(-4.85068927010199,-49.4189842542419,
-8.4016402675109));
#22200=CARTESIAN_POINT('Ctrl Pts',(-7.27603390513785,-49.2439842542419,
-4.20082013374671));
#22201=CARTESIAN_POINT('Ctrl Pts',(-9.70137854017372,-49.0689842542419,
1.74701493417668E-11));
#22202=CARTESIAN_POINT('Ctrl Pts',(-7.27603390512272,-48.8939842542419,
4.20082013377292));
#22203=CARTESIAN_POINT('Ctrl Pts',(-4.85068927007173,-48.7189842542419,
8.40164026752836));
#22204=CARTESIAN_POINT('Ctrl Pts',(1.5129078685785E-11,-48.5439842542419,
8.40164026751963));
#22205=CARTESIAN_POINT('Ctrl Pts',(4.85068927010198,-48.3689842542419,8.4016402675109));
#22206=CARTESIAN_POINT('Ctrl Pts',(7.27603390513785,-48.1939842542419,4.20082013374672));
#22207=CARTESIAN_POINT('Ctrl Pts',(9.70137854017372,-48.0189842542419,-1.74689612655491E-11));
#22208=CARTESIAN_POINT('Ctrl Pts',(7.27603390512273,-47.8439842542419,-4.20082013377291));
#22209=CARTESIAN_POINT('Ctrl Pts',(4.85068927007173,-47.6689842542419,-8.40164026752836));
#22210=CARTESIAN_POINT('Ctrl Pts',(-1.51301075899711E-11,-47.4939842542419,
-8.40164026751963));
#22211=CARTESIAN_POINT('Ctrl Pts',(-4.85068927010199,-47.3189842542419,
-8.4016402675109));
#22212=CARTESIAN_POINT('Ctrl Pts',(-7.27603390513785,-47.1439842542419,
-4.20082013374671));
#22213=CARTESIAN_POINT('Ctrl Pts',(-9.70137854017372,-46.9689842542419,
1.74701493417668E-11));
#22214=CARTESIAN_POINT('Ctrl Pts',(-7.27603390512272,-46.7939842542419,
4.20082013377292));
#22215=CARTESIAN_POINT('Ctrl Pts',(-4.85068927007173,-46.6189842542419,
8.40164026752836));
#22216=CARTESIAN_POINT('Ctrl Pts',(1.5129078685785E-11,-46.4439842542419,
8.40164026751963));
#22217=CARTESIAN_POINT('Ctrl Pts',(4.85068927010198,-46.2689842542419,8.4016402675109));
#22218=CARTESIAN_POINT('Ctrl Pts',(7.27603390513785,-46.0939842542419,4.20082013374672));
#22219=CARTESIAN_POINT('Ctrl Pts',(9.70137854017372,-45.9189842542419,-1.74689612655491E-11));
#22220=CARTESIAN_POINT('Ctrl Pts',(7.27603390512273,-45.7439842542419,-4.20082013377291));
#22221=CARTESIAN_POINT('Ctrl Pts',(4.85068927007173,-45.5689842542419,-8.40164026752836));
#22222=CARTESIAN_POINT('Ctrl Pts',(-1.51301075899711E-11,-45.3939842542419,
-8.40164026751963));
#22223=CARTESIAN_POINT('Ctrl Pts',(-4.85068927010199,-45.2189842542419,
-8.4016402675109));
#22224=CARTESIAN_POINT('Ctrl Pts',(-7.27603390513785,-45.0439842542419,
-4.20082013374671));
#22225=CARTESIAN_POINT('Ctrl Pts',(-9.70137854017372,-44.8689842542419,
1.74701493417668E-11));
#22226=CARTESIAN_POINT('Ctrl Pts',(-7.27603390512272,-44.6939842542419,
4.20082013377292));
#22227=CARTESIAN_POINT('Ctrl Pts',(-4.85068927007173,-44.5189842542419,
8.40164026752836));
#22228=CARTESIAN_POINT('Ctrl Pts',(1.5129078685785E-11,-44.3439842542419,
8.40164026751963));
#22229=CARTESIAN_POINT('Ctrl Pts',(4.85068927010198,-44.1689842542419,8.4016402675109));
#22230=CARTESIAN_POINT('Ctrl Pts',(7.27603390513785,-43.9939842542419,4.20082013374672));
#22231=CARTESIAN_POINT('Ctrl Pts',(9.70137854017372,-43.8189842542419,-1.74689612655491E-11));
#22232=CARTESIAN_POINT('Ctrl Pts',(7.27603390512273,-43.6439842542419,-4.20082013377291));
#22233=CARTESIAN_POINT('Ctrl Pts',(4.85068927007173,-43.4689842542419,-8.40164026752836));
#22234=CARTESIAN_POINT('Ctrl Pts',(-1.51301075899711E-11,-43.2939842542419,
-8.40164026751963));
#22235=CARTESIAN_POINT('Ctrl Pts',(-4.85068927010199,-43.1189842542419,
-8.4016402675109));
#22236=CARTESIAN_POINT('Ctrl Pts',(-7.27603390513785,-42.9439842542419,
-4.20082013374671));
#22237=CARTESIAN_POINT('Ctrl Pts',(-9.70137854017372,-42.7689842542419,
1.74701493417668E-11));
#22238=CARTESIAN_POINT('Ctrl Pts',(-7.27603390512272,-42.5939842542419,
4.20082013377292));
#22239=CARTESIAN_POINT('Ctrl Pts',(-4.85068927007173,-42.4189842542419,
8.40164026752836));
#22240=CARTESIAN_POINT('Ctrl Pts',(1.5129078685785E-11,-42.2439842542419,
8.40164026751963));
#22241=CARTESIAN_POINT('Ctrl Pts',(4.85068927010198,-42.0689842542419,8.4016402675109));
#22242=CARTESIAN_POINT('Ctrl Pts',(7.27603390513785,-41.8939842542419,4.20082013374672));
#22243=CARTESIAN_POINT('Ctrl Pts',(9.70137854017372,-41.7189842542419,-1.74689612655491E-11));
#22244=CARTESIAN_POINT('Ctrl Pts',(7.27603390512273,-41.5439842542419,-4.20082013377291));
#22245=CARTESIAN_POINT('Ctrl Pts',(4.85068927007173,-41.3689842542419,-8.40164026752836));
#22246=CARTESIAN_POINT('Ctrl Pts',(-1.51301075899711E-11,-41.1939842542419,
-8.40164026751963));
#22247=CARTESIAN_POINT('Ctrl Pts',(-4.85068927010199,-41.0189842542419,
-8.4016402675109));
#22248=CARTESIAN_POINT('Ctrl Pts',(-7.27603390513785,-40.8439842542419,
-4.20082013374671));
#22249=CARTESIAN_POINT('Ctrl Pts',(-9.70137854017372,-40.6689842542419,
1.74701493417668E-11));
#22250=CARTESIAN_POINT('Ctrl Pts',(-7.27603390512272,-40.4939842542419,
4.20082013377292));
#22251=CARTESIAN_POINT('Ctrl Pts',(-4.85068927007173,-40.3189842542419,
8.40164026752836));
#22252=CARTESIAN_POINT('Ctrl Pts',(1.5129078685785E-11,-40.1439842542419,
8.40164026751963));
#22253=CARTESIAN_POINT('Ctrl Pts',(4.85068927010198,-39.9689842542419,8.4016402675109));
#22254=CARTESIAN_POINT('Ctrl Pts',(7.27603390513785,-39.7939842542419,4.20082013374672));
#22255=CARTESIAN_POINT('Ctrl Pts',(9.70137854017372,-39.6189842542419,-1.74689612655491E-11));
#22256=CARTESIAN_POINT('Ctrl Pts',(7.27603390512273,-39.4439842542419,-4.20082013377291));
#22257=CARTESIAN_POINT('Ctrl Pts',(4.85068927007173,-39.2689842542419,-8.40164026752836));
#22258=CARTESIAN_POINT('Ctrl Pts',(-1.51301075899711E-11,-39.0939842542419,
-8.40164026751963));
#22259=CARTESIAN_POINT('Ctrl Pts',(-4.85068927010199,-38.9189842542419,
-8.4016402675109));
#22260=CARTESIAN_POINT('Ctrl Pts',(-7.27603390513785,-38.7439842542419,
-4.20082013374671));
#22261=CARTESIAN_POINT('Ctrl Pts',(-9.70137854017372,-38.5689842542419,
1.74701493417668E-11));
#22262=CARTESIAN_POINT('Ctrl Pts',(-7.27603390512272,-38.3939842542419,
4.20082013377292));
#22263=CARTESIAN_POINT('Ctrl Pts',(-4.85068927007173,-38.2189842542419,
8.40164026752836));
#22264=CARTESIAN_POINT('Ctrl Pts',(1.5129078685785E-11,-38.0439842542419,
8.40164026751963));
#22265=CARTESIAN_POINT('Ctrl Pts',(4.85068927010198,-37.8689842542419,8.4016402675109));
#22266=CARTESIAN_POINT('Ctrl Pts',(7.27603390513785,-37.6939842542419,4.20082013374672));
#22267=CARTESIAN_POINT('Ctrl Pts',(9.70137854017372,-37.5189842542419,-1.74689612655491E-11));
#22268=CARTESIAN_POINT('Ctrl Pts',(7.27603390512273,-37.3439842542419,-4.20082013377291));
#22269=CARTESIAN_POINT('Ctrl Pts',(4.85068927007173,-37.1689842542419,-8.40164026752836));
#22270=CARTESIAN_POINT('Ctrl Pts',(-1.51301075899711E-11,-36.9939842542419,
-8.40164026751963));
#22271=CARTESIAN_POINT('Ctrl Pts',(-4.85068927010199,-36.8189842542419,
-8.4016402675109));
#22272=CARTESIAN_POINT('Ctrl Pts',(-7.27603390513785,-36.6439842542419,
-4.20082013374671));
#22273=CARTESIAN_POINT('Ctrl Pts',(-9.70137854017372,-36.4689842542419,
1.74701493417668E-11));
#22274=CARTESIAN_POINT('Ctrl Pts',(-7.27603390512272,-36.2939842542419,
4.20082013377292));
#22275=CARTESIAN_POINT('Ctrl Pts',(-4.85068927007173,-36.1189842542419,
8.40164026752836));
#22276=CARTESIAN_POINT('Ctrl Pts',(1.5129078685785E-11,-35.9439842542419,
8.40164026751963));
#22277=CARTESIAN_POINT('Ctrl Pts',(4.85068927010198,-35.7689842542419,8.4016402675109));
#22278=CARTESIAN_POINT('Ctrl Pts',(7.27603390513785,-35.5939842542419,4.20082013374672));
#22279=CARTESIAN_POINT('Ctrl Pts',(9.70137854017372,-35.4189842542419,-1.74689612655491E-11));
#22280=CARTESIAN_POINT('Ctrl Pts',(7.27603390512273,-35.2439842542419,-4.20082013377291));
#22281=CARTESIAN_POINT('Ctrl Pts',(4.85068927007173,-35.0689842542419,-8.40164026752836));
#22282=CARTESIAN_POINT('Ctrl Pts',(-1.51301075899711E-11,-34.8939842542419,
-8.40164026751963));
#22283=CARTESIAN_POINT('Ctrl Pts',(-4.85068927010199,-34.7189842542419,
-8.4016402675109));
#22284=CARTESIAN_POINT('Ctrl Pts',(-7.27603390513785,-34.5439842542419,
-4.20082013374671));
#22285=CARTESIAN_POINT('Ctrl Pts',(-9.70137854017372,-34.3689842542419,
1.74701493417668E-11));
#22286=CARTESIAN_POINT('Ctrl Pts',(-7.27603390512272,-34.1939842542419,
4.20082013377292));
#22287=CARTESIAN_POINT('Ctrl Pts',(-4.85068927007173,-34.0189842542419,
8.40164026752836));
#22288=CARTESIAN_POINT('Ctrl Pts',(1.5129078685785E-11,-33.8439842542419,
8.40164026751963));
#22289=CARTESIAN_POINT('Ctrl Pts',(4.85068927010198,-33.6689842542419,8.4016402675109));
#22290=CARTESIAN_POINT('Ctrl Pts',(7.27603390513785,-33.4939842542419,4.20082013374672));
#22291=CARTESIAN_POINT('Ctrl Pts',(9.70137854017372,-33.3189842542419,-1.74689612655491E-11));
#22292=CARTESIAN_POINT('Ctrl Pts',(7.27603390512273,-33.1439842542419,-4.20082013377291));
#22293=CARTESIAN_POINT('Ctrl Pts',(4.85068927007173,-32.9689842542419,-8.40164026752836));
#22294=CARTESIAN_POINT('Ctrl Pts',(-1.51301075899711E-11,-32.7939842542419,
-8.40164026751963));
#22295=CARTESIAN_POINT('Ctrl Pts',(-4.85068927010199,-32.6189842542419,
-8.4016402675109));
#22296=CARTESIAN_POINT('Ctrl Pts',(-7.27603390513785,-32.4439842542419,
-4.20082013374671));
#22297=CARTESIAN_POINT('Ctrl Pts',(-9.70137854017372,-32.2689842542419,
1.74701493417668E-11));
#22298=CARTESIAN_POINT('Ctrl Pts',(-7.27603390512272,-32.0939842542419,
4.20082013377292));
#22299=CARTESIAN_POINT('Ctrl Pts',(-4.85068927007173,-31.9189842542419,
8.40164026752836));
#22300=CARTESIAN_POINT('Ctrl Pts',(1.5129078685785E-11,-31.7439842542419,
8.40164026751963));
#22301=CARTESIAN_POINT('Ctrl Pts',(4.85068927010198,-31.5689842542419,8.4016402675109));
#22302=CARTESIAN_POINT('Ctrl Pts',(7.27603390513785,-31.3939842542419,4.20082013374672));
#22303=CARTESIAN_POINT('Ctrl Pts',(9.70137854017372,-31.2189842542419,-1.74689612655491E-11));
#22304=CARTESIAN_POINT('Ctrl Pts',(7.27603390512273,-31.0439842542419,-4.20082013377291));
#22305=CARTESIAN_POINT('Ctrl Pts',(4.85068927007173,-30.8689842542419,-8.40164026752836));
#22306=CARTESIAN_POINT('Ctrl Pts',(-1.51301075899711E-11,-30.6939842542419,
-8.40164026751963));
#22307=CARTESIAN_POINT('Ctrl Pts',(-4.85068927010199,-30.5189842542419,
-8.4016402675109));
#22308=CARTESIAN_POINT('Ctrl Pts',(-7.27603390513785,-30.3439842542419,
-4.20082013374671));
#22309=CARTESIAN_POINT('Ctrl Pts',(-9.70137854017372,-30.1689842542419,
1.74701493417668E-11));
#22310=CARTESIAN_POINT('Ctrl Pts',(-7.27603390512272,-29.9939842542419,
4.20082013377292));
#22311=CARTESIAN_POINT('Ctrl Pts',(-4.85068927007173,-29.8189842542419,
8.40164026752836));
#22312=CARTESIAN_POINT('Ctrl Pts',(1.5129078685785E-11,-29.6439842542419,
8.40164026751963));
#22313=CARTESIAN_POINT('Ctrl Pts',(4.85068927010198,-29.4689842542419,8.4016402675109));
#22314=CARTESIAN_POINT('Ctrl Pts',(7.27603390513785,-29.2939842542419,4.20082013374672));
#22315=CARTESIAN_POINT('Ctrl Pts',(9.70137854017372,-29.1189842542419,-1.74689612655491E-11));
#22316=CARTESIAN_POINT('Ctrl Pts',(7.27603390512273,-28.9439842542419,-4.20082013377291));
#22317=CARTESIAN_POINT('Ctrl Pts',(4.85068927007173,-28.7689842542419,-8.40164026752836));
#22318=CARTESIAN_POINT('Ctrl Pts',(-1.51301075899711E-11,-28.5939842542419,
-8.40164026751963));
#22319=CARTESIAN_POINT('Ctrl Pts',(-4.85068927010199,-28.4189842542419,
-8.4016402675109));
#22320=CARTESIAN_POINT('Ctrl Pts',(-7.27603390513785,-28.2439842542419,
-4.20082013374671));
#22321=CARTESIAN_POINT('Ctrl Pts',(-9.70137854017372,-28.0689842542419,
1.74701493417668E-11));
#22322=CARTESIAN_POINT('Ctrl Pts',(-7.27603390512272,-27.8939842542419,
4.20082013377292));
#22323=CARTESIAN_POINT('Ctrl Pts',(-4.85068927007173,-27.7189842542419,
8.40164026752836));
#22324=CARTESIAN_POINT('Ctrl Pts',(1.5129078685785E-11,-27.5439842542419,
8.40164026751963));
#22325=CARTESIAN_POINT('Ctrl Pts',(4.85068927010198,-27.3689842542419,8.4016402675109));
#22326=CARTESIAN_POINT('Ctrl Pts',(7.27603390513785,-27.1939842542419,4.20082013374672));
#22327=CARTESIAN_POINT('Ctrl Pts',(9.70137854017372,-27.0189842542419,-1.74689612655491E-11));
#22328=CARTESIAN_POINT('Ctrl Pts',(7.27603390512273,-26.8439842542419,-4.20082013377291));
#22329=CARTESIAN_POINT('Ctrl Pts',(4.85068927007173,-26.6689842542419,-8.40164026752836));
#22330=CARTESIAN_POINT('Ctrl Pts',(-1.51301075899711E-11,-26.4939842542419,
-8.40164026751963));
#22331=CARTESIAN_POINT('Ctrl Pts',(-4.85068927010199,-26.3189842542419,
-8.4016402675109));
#22332=CARTESIAN_POINT('Ctrl Pts',(-7.27603390513785,-26.1439842542419,
-4.20082013374671));
#22333=CARTESIAN_POINT('Ctrl Pts',(-9.70137854017372,-25.9689842542419,
1.74701493417668E-11));
#22334=CARTESIAN_POINT('Ctrl Pts',(-7.27603390512272,-25.7939842542419,
4.20082013377292));
#22335=CARTESIAN_POINT('Ctrl Pts',(-4.85068927007173,-25.6189842542419,
8.40164026752836));
#22336=CARTESIAN_POINT('Ctrl Pts',(1.5129078685785E-11,-25.4439842542419,
8.40164026751963));
#22337=CARTESIAN_POINT('Ctrl Pts',(4.85068927010198,-25.2689842542419,8.4016402675109));
#22338=CARTESIAN_POINT('Ctrl Pts',(7.27603390513785,-25.0939842542419,4.20082013374672));
#22339=CARTESIAN_POINT('Ctrl Pts',(9.70137854017372,-24.9189842542419,-1.74689612655491E-11));
#22340=CARTESIAN_POINT('Ctrl Pts',(7.27603390512273,-24.7439842542419,-4.20082013377291));
#22341=CARTESIAN_POINT('Ctrl Pts',(4.85068927007173,-24.5689842542419,-8.40164026752836));
#22342=CARTESIAN_POINT('Ctrl Pts',(-1.51301075899711E-11,-24.3939842542419,
-8.40164026751963));
#22343=CARTESIAN_POINT('Ctrl Pts',(-4.85068927010199,-24.2189842542419,
-8.4016402675109));
#22344=CARTESIAN_POINT('Ctrl Pts',(-7.27603390513785,-24.0439842542419,
-4.20082013374671));
#22345=CARTESIAN_POINT('Ctrl Pts',(-9.70137854017372,-23.8689842542419,
1.74701493417668E-11));
#22346=CARTESIAN_POINT('Ctrl Pts',(-7.27603390512272,-23.6939842542419,
4.20082013377292));
#22347=CARTESIAN_POINT('Ctrl Pts',(-4.85068927007173,-23.5189842542419,
8.40164026752836));
#22348=CARTESIAN_POINT('Ctrl Pts',(1.5129078685785E-11,-23.3439842542419,
8.40164026751963));
#22349=CARTESIAN_POINT('Ctrl Pts',(4.85068927010198,-23.1689842542419,8.4016402675109));
#22350=CARTESIAN_POINT('Ctrl Pts',(7.27603390513785,-22.9939842542419,4.20082013374672));
#22351=CARTESIAN_POINT('Ctrl Pts',(9.70137854017372,-22.8189842542419,-1.74689612655491E-11));
#22352=CARTESIAN_POINT('Ctrl Pts',(7.27603390512273,-22.6439842542419,-4.20082013377291));
#22353=CARTESIAN_POINT('Ctrl Pts',(4.85068927007173,-22.4689842542419,-8.40164026752836));
#22354=CARTESIAN_POINT('Ctrl Pts',(-1.51301075899711E-11,-22.2939842542419,
-8.40164026751963));
#22355=CARTESIAN_POINT('Ctrl Pts',(-4.85068927010199,-22.1189842542419,
-8.4016402675109));
#22356=CARTESIAN_POINT('Ctrl Pts',(-7.27603390513785,-21.9439842542419,
-4.20082013374671));
#22357=CARTESIAN_POINT('Ctrl Pts',(-9.70137854017372,-21.7689842542419,
1.74701493417668E-11));
#22358=CARTESIAN_POINT('Ctrl Pts',(-7.27603390512272,-21.5939842542419,
4.20082013377292));
#22359=CARTESIAN_POINT('Ctrl Pts',(-4.85068927007173,-21.4189842542419,
8.40164026752836));
#22360=CARTESIAN_POINT('Ctrl Pts',(1.5129078685785E-11,-21.2439842542419,
8.40164026751963));
#22361=CARTESIAN_POINT('Ctrl Pts',(4.85068927010198,-21.0689842542419,8.4016402675109));
#22362=CARTESIAN_POINT('Ctrl Pts',(7.27603390513785,-20.8939842542419,4.20082013374672));
#22363=CARTESIAN_POINT('Ctrl Pts',(9.70137854017372,-20.7189842542419,-1.74689612655491E-11));
#22364=CARTESIAN_POINT('Ctrl Pts',(7.27603390512273,-20.5439842542419,-4.20082013377291));
#22365=CARTESIAN_POINT('Ctrl Pts',(4.85068927007173,-20.3689842542419,-8.40164026752836));
#22366=CARTESIAN_POINT('Ctrl Pts',(-1.51301075899711E-11,-20.1939842542419,
-8.40164026751963));
#22367=CARTESIAN_POINT('Ctrl Pts',(-4.85068927010199,-20.0189842542419,
-8.4016402675109));
#22368=CARTESIAN_POINT('Ctrl Pts',(-7.27603390513785,-19.8439842542419,
-4.20082013374671));
#22369=CARTESIAN_POINT('Ctrl Pts',(-9.70137854017372,-19.6689842542419,
1.74701493417668E-11));
#22370=CARTESIAN_POINT('Ctrl Pts',(-7.27603390512272,-19.4939842542419,
4.20082013377292));
#22371=CARTESIAN_POINT('Ctrl Pts',(-4.85068927007173,-19.3189842542419,
8.40164026752836));
#22372=CARTESIAN_POINT('Ctrl Pts',(1.5129078685785E-11,-19.1439842542419,
8.40164026751963));
#22373=CARTESIAN_POINT('Ctrl Pts',(4.85068927010198,-18.9689842542419,8.4016402675109));
#22374=CARTESIAN_POINT('Ctrl Pts',(7.27603390513785,-18.7939842542419,4.20082013374672));
#22375=CARTESIAN_POINT('Ctrl Pts',(9.70137854017372,-18.6189842542419,-1.74689612655491E-11));
#22376=CARTESIAN_POINT('Ctrl Pts',(7.27603390512273,-18.4439842542419,-4.20082013377291));
#22377=CARTESIAN_POINT('Ctrl Pts',(4.85068927007173,-18.2689842542419,-8.40164026752836));
#22378=CARTESIAN_POINT('Ctrl Pts',(-1.51301075899711E-11,-18.0939842542419,
-8.40164026751963));
#22379=CARTESIAN_POINT('Ctrl Pts',(-4.85068927010199,-17.9189842542419,
-8.4016402675109));
#22380=CARTESIAN_POINT('Ctrl Pts',(-7.27603390513785,-17.7439842542419,
-4.20082013374671));
#22381=CARTESIAN_POINT('Ctrl Pts',(-9.70137854017372,-17.5689842542419,
1.74701493417668E-11));
#22382=CARTESIAN_POINT('Ctrl Pts',(-7.27603390512272,-17.3939842542419,
4.20082013377292));
#22383=CARTESIAN_POINT('Ctrl Pts',(-4.85068927007173,-17.2189842542419,
8.40164026752836));
#22384=CARTESIAN_POINT('Ctrl Pts',(1.5129078685785E-11,-17.0439842542419,
8.40164026751963));
#22385=CARTESIAN_POINT('Ctrl Pts',(4.85068927010198,-16.8689842542419,8.4016402675109));
#22386=CARTESIAN_POINT('Ctrl Pts',(7.27603390513785,-16.6939842542419,4.20082013374672));
#22387=CARTESIAN_POINT('Ctrl Pts',(9.70137854017372,-16.518984254242,-1.74689612655491E-11));
#22388=CARTESIAN_POINT('Ctrl Pts',(7.27603390512273,-16.3439842542419,-4.20082013377291));
#22389=CARTESIAN_POINT('Ctrl Pts',(4.85068927007173,-16.1689842542419,-8.40164026752836));
#22390=CARTESIAN_POINT('Ctrl Pts',(-1.51301075899711E-11,-15.9939842542419,
-8.40164026751963));
#22391=CARTESIAN_POINT('Ctrl Pts',(-4.85068927010199,-15.8189842542419,
-8.4016402675109));
#22392=CARTESIAN_POINT('Ctrl Pts',(-7.27603390513785,-15.6439842542419,
-4.20082013374671));
#22393=CARTESIAN_POINT('Ctrl Pts',(-9.70137854017372,-15.4689842542419,
1.74701493417668E-11));
#22394=CARTESIAN_POINT('Ctrl Pts',(-7.27603390512272,-15.2939842542419,
4.20082013377292));
#22395=CARTESIAN_POINT('Ctrl Pts',(-4.85068927007173,-15.1189842542419,
8.40164026752836));
#22396=CARTESIAN_POINT('Ctrl Pts',(1.5129078685785E-11,-14.9439842542419,
8.40164026751963));
#22397=CARTESIAN_POINT('Ctrl Pts',(4.85068927010198,-14.7689842542419,8.4016402675109));
#22398=CARTESIAN_POINT('Ctrl Pts',(7.27603390513785,-14.5939842542419,4.20082013374672));
#22399=CARTESIAN_POINT('Ctrl Pts',(9.70137854017372,-14.4189842542419,-1.74689612655491E-11));
#22400=CARTESIAN_POINT('Ctrl Pts',(7.27603390512273,-14.2439842542419,-4.20082013377291));
#22401=CARTESIAN_POINT('Ctrl Pts',(4.85068927007173,-14.0689842542419,-8.40164026752836));
#22402=CARTESIAN_POINT('Ctrl Pts',(-1.51301075899711E-11,-13.8939842542419,
-8.40164026751963));
#22403=CARTESIAN_POINT('Ctrl Pts',(-4.85068927010199,-13.7189842542419,
-8.4016402675109));
#22404=CARTESIAN_POINT('Ctrl Pts',(-7.27603390513785,-13.5439842542419,
-4.20082013374671));
#22405=CARTESIAN_POINT('Ctrl Pts',(-9.70137854017372,-13.3689842542419,
1.74701493417668E-11));
#22406=CARTESIAN_POINT('Ctrl Pts',(-7.27603390512272,-13.193984254242,4.20082013377292));
#22407=CARTESIAN_POINT('Ctrl Pts',(-4.85068927007173,-13.018984254242,8.40164026752836));
#22408=CARTESIAN_POINT('Ctrl Pts',(1.5129078685785E-11,-12.8439842542419,
8.40164026751963));
#22409=CARTESIAN_POINT('Ctrl Pts',(4.85068927010198,-12.668984254242,8.4016402675109));
#22410=CARTESIAN_POINT('Ctrl Pts',(7.27603390513785,-12.4939842542419,4.20082013374672));
#22411=CARTESIAN_POINT('Ctrl Pts',(9.70137854017372,-12.3189842542419,-1.74689612655491E-11));
#22412=CARTESIAN_POINT('Ctrl Pts',(7.27603390512273,-12.143984254242,-4.20082013377291));
#22413=CARTESIAN_POINT('Ctrl Pts',(4.85068927007173,-11.968984254242,-8.40164026752836));
#22414=CARTESIAN_POINT('Ctrl Pts',(-1.51301075899711E-11,-11.7939842542419,
-8.40164026751963));
#22415=CARTESIAN_POINT('Ctrl Pts',(-4.85068927010199,-11.6189842542419,
-8.4016402675109));
#22416=CARTESIAN_POINT('Ctrl Pts',(-7.27603390513785,-11.443984254242,-4.20082013374671));
#22417=CARTESIAN_POINT('Ctrl Pts',(-9.70137854017372,-11.2689842542419,
1.74701493417668E-11));
#22418=CARTESIAN_POINT('Ctrl Pts',(-7.27603390512272,-11.0939842542419,
4.20082013377292));
#22419=CARTESIAN_POINT('Ctrl Pts',(-4.85068927007173,-10.918984254242,8.40164026752836));
#22420=CARTESIAN_POINT('Ctrl Pts',(1.5129078685785E-11,-10.7439842542419,
8.40164026751963));
#22421=CARTESIAN_POINT('Ctrl Pts',(4.85068927010198,-10.5689842542419,8.4016402675109));
#22422=CARTESIAN_POINT('Ctrl Pts',(7.27603390513785,-10.393984254242,4.20082013374672));
#22423=CARTESIAN_POINT('Ctrl Pts',(9.70137854017372,-10.2189842542419,-1.74689612655491E-11));
#22424=CARTESIAN_POINT('Ctrl Pts',(7.27603390512273,-10.0439842542419,-4.20082013377291));
#22425=CARTESIAN_POINT('Ctrl Pts',(4.85068927007173,-9.86898425424196,-8.40164026752836));
#22426=CARTESIAN_POINT('Ctrl Pts',(-1.51301075899711E-11,-9.69398425424195,
-8.40164026751963));
#22427=CARTESIAN_POINT('Ctrl Pts',(-4.85068927010199,-9.51898425424195,
-8.4016402675109));
#22428=CARTESIAN_POINT('Ctrl Pts',(-7.27603390513785,-9.34398425424196,
-4.20082013374671));
#22429=CARTESIAN_POINT('Ctrl Pts',(-9.70137854017372,-9.16898425424195,
1.74701493417668E-11));
#22430=CARTESIAN_POINT('Ctrl Pts',(-7.27603390512272,-8.99398425424194,
4.20082013377292));
#22431=CARTESIAN_POINT('Ctrl Pts',(-4.85068927007173,-8.81898425424197,
8.40164026752836));
#22432=CARTESIAN_POINT('Ctrl Pts',(1.5129078685785E-11,-8.64398425424195,
8.40164026751963));
#22433=CARTESIAN_POINT('Ctrl Pts',(4.85068927010198,-8.46898425424195,8.4016402675109));
#22434=CARTESIAN_POINT('Ctrl Pts',(7.27603390513785,-8.29398425424196,4.20082013374672));
#22435=CARTESIAN_POINT('Ctrl Pts',(9.70137854017372,-8.11898425424196,-1.74689612655491E-11));
#22436=CARTESIAN_POINT('Ctrl Pts',(7.27603390512273,-7.94398425424195,-4.20082013377291));
#22437=CARTESIAN_POINT('Ctrl Pts',(4.85068927007173,-7.76898425424197,-8.40164026752836));
#22438=CARTESIAN_POINT('Ctrl Pts',(-1.51301075899711E-11,-7.59398425424196,
-8.40164026751963));
#22439=CARTESIAN_POINT('Ctrl Pts',(-4.85068927010199,-7.41898425424196,
-8.4016402675109));
#22440=CARTESIAN_POINT('Ctrl Pts',(-7.27603390513785,-7.24398425424194,
-4.20082013374671));
#22441=CARTESIAN_POINT('Ctrl Pts',(-9.70137854017372,-7.06898425424196,
1.74701493417668E-11));
#22442=CARTESIAN_POINT('Ctrl Pts',(-7.27603390512272,-6.89398425424195,
4.20082013377292));
#22443=CARTESIAN_POINT('Ctrl Pts',(-4.85068927007173,-6.71898425424195,
8.40164026752836));
#22444=CARTESIAN_POINT('Ctrl Pts',(1.5129078685785E-11,-6.54398425424196,
8.40164026751963));
#22445=CARTESIAN_POINT('Ctrl Pts',(4.85068927010198,-6.36898425424197,8.4016402675109));
#22446=CARTESIAN_POINT('Ctrl Pts',(7.27603390513785,-6.19398425424195,4.20082013374672));
#22447=CARTESIAN_POINT('Ctrl Pts',(9.70137854017372,-6.01898425424197,-1.74689612655491E-11));
#22448=CARTESIAN_POINT('Ctrl Pts',(7.27603390512273,-5.84398425424196,-4.20082013377291));
#22449=CARTESIAN_POINT('Ctrl Pts',(4.85068927007173,-5.66898425424195,-8.40164026752836));
#22450=CARTESIAN_POINT('Ctrl Pts',(-1.51301075899711E-11,-5.49398425424197,
-8.40164026751963));
#22451=CARTESIAN_POINT('Ctrl Pts',(-4.85068927010199,-5.31898425424197,
-8.4016402675109));
#22452=CARTESIAN_POINT('Ctrl Pts',(-7.27603390513785,-5.14398425424195,
-4.20082013374671));
#22453=CARTESIAN_POINT('Ctrl Pts',(-9.70137854017372,-4.96898425424197,
1.74701493417668E-11));
#22454=CARTESIAN_POINT('Ctrl Pts',(-7.27603390512272,-4.79398425424196,
4.20082013377292));
#22455=CARTESIAN_POINT('Ctrl Pts',(-4.85068927007173,-4.61898425424196,
8.40164026752836));
#22456=CARTESIAN_POINT('Ctrl Pts',(1.5129078685785E-11,-4.44398425424197,
8.40164026751963));
#22457=CARTESIAN_POINT('Ctrl Pts',(4.85068927010198,-4.26898425424197,8.4016402675109));
#22458=CARTESIAN_POINT('Ctrl Pts',(7.27603390513785,-4.09398425424196,4.20082013374672));
#22459=CARTESIAN_POINT('Ctrl Pts',(9.70137854017372,-3.91898425424198,-1.74689612655491E-11));
#22460=CARTESIAN_POINT('Ctrl Pts',(7.27603390512273,-3.74398425424197,-4.20082013377291));
#22461=CARTESIAN_POINT('Ctrl Pts',(4.85068927007173,-3.56898425424196,-8.40164026752836));
#22462=CARTESIAN_POINT('Ctrl Pts',(-1.51301075899711E-11,-3.39398425424198,
-8.40164026751963));
#22463=CARTESIAN_POINT('Ctrl Pts',(-4.85068927010199,-3.21898425424198,
-8.4016402675109));
#22464=CARTESIAN_POINT('Ctrl Pts',(-7.27603390513785,-3.04398425424196,
-4.20082013374671));
#22465=CARTESIAN_POINT('Ctrl Pts',(-9.70137854017372,-2.86898425424196,
1.74701493417668E-11));
#22466=CARTESIAN_POINT('Ctrl Pts',(-7.27603390512272,-2.69398425424197,
4.20082013377292));
#22467=CARTESIAN_POINT('Ctrl Pts',(-4.85068927007173,-2.51898425424196,
8.40164026752836));
#22468=CARTESIAN_POINT('Ctrl Pts',(1.5129078685785E-11,-2.34398425424195,
8.40164026751963));
#22469=CARTESIAN_POINT('Ctrl Pts',(4.85068927010198,-2.16898425424197,8.4016402675109));
#22470=CARTESIAN_POINT('Ctrl Pts',(7.27603390513785,-1.99398425424197,4.20082013374672));
#22471=CARTESIAN_POINT('Ctrl Pts',(9.70137854017372,-1.81898425424196,-1.74689612655491E-11));
#22472=CARTESIAN_POINT('Ctrl Pts',(7.27603390512273,-1.64398425424198,-4.20082013377291));
#22473=CARTESIAN_POINT('Ctrl Pts',(4.85068927007173,-1.46898425424197,-8.40164026752836));
#22474=CARTESIAN_POINT('Ctrl Pts',(-1.51301075899711E-11,-1.29398425424196,
-8.40164026751963));
#22475=CARTESIAN_POINT('Ctrl Pts',(-4.85068927010199,-1.11898425424198,
-8.4016402675109));
#22476=CARTESIAN_POINT('Ctrl Pts',(-7.27603390513785,-0.94398425424197,
-4.20082013374671));
#22477=CARTESIAN_POINT('Ctrl Pts',(-9.70137854017372,-0.768984254241965,
1.74701493417668E-11));
#22478=CARTESIAN_POINT('Ctrl Pts',(-7.27603390512272,-0.59398425424198,
4.20082013377292));
#22479=CARTESIAN_POINT('Ctrl Pts',(-4.85068927007173,-0.418984254241974,
8.40164026752836));
#22480=CARTESIAN_POINT('Ctrl Pts',(1.5129078685785E-11,-0.243984254241963,
8.40164026751963));
#22481=CARTESIAN_POINT('Ctrl Pts',(4.85068927010198,-0.068984254241984,
8.4016402675109));
#22482=CARTESIAN_POINT('Ctrl Pts',(7.27603390513785,0.106015745758026,4.20082013374672));
#22483=CARTESIAN_POINT('Ctrl Pts',(9.70137854017372,0.28101574575803,-1.74689612655491E-11));
#22484=CARTESIAN_POINT('Ctrl Pts',(7.27603390512273,0.456015745758015,-4.20082013377291));
#22485=CARTESIAN_POINT('Ctrl Pts',(4.85068927007173,0.631015745758021,-8.40164026752836));
#22486=CARTESIAN_POINT('Ctrl Pts',(-1.51301075899711E-11,0.806015745758032,
-8.40164026751963));
#22487=CARTESIAN_POINT('Ctrl Pts',(-4.85068927010199,0.981015745758011,
-8.4016402675109));
#22488=CARTESIAN_POINT('Ctrl Pts',(-7.27603390513785,1.15601574575802,-4.20082013374671));
#22489=CARTESIAN_POINT('Ctrl Pts',(-9.70137854017372,1.33101574575803,1.74701493417668E-11));
#22490=CARTESIAN_POINT('Ctrl Pts',(-7.27603390512272,1.50601574575804,4.20082013377292));
#22491=CARTESIAN_POINT('Ctrl Pts',(-4.85068927007173,1.68101574575802,8.40164026752836));
#22492=CARTESIAN_POINT('Ctrl Pts',(1.5129078685785E-11,1.85601574575803,
8.40164026751963));
#22493=CARTESIAN_POINT('Ctrl Pts',(4.85068927010198,2.03101574575803,8.4016402675109));
#22494=CARTESIAN_POINT('Ctrl Pts',(7.27603390513785,2.20601574575802,4.20082013374672));
#22495=CARTESIAN_POINT('Ctrl Pts',(9.70137854017372,2.38101574575802,-1.74689612655491E-11));
#22496=CARTESIAN_POINT('Ctrl Pts',(7.27603390512273,2.55601574575803,-4.20082013377291));
#22497=CARTESIAN_POINT('Ctrl Pts',(4.85068927007173,2.73101574575801,-8.40164026752836));
#22498=CARTESIAN_POINT('Ctrl Pts',(-1.51301075899711E-11,2.90601574575802,
-8.40164026751963));
#22499=CARTESIAN_POINT('Ctrl Pts',(-4.85068927010199,3.08101574575803,-8.4016402675109));
#22500=CARTESIAN_POINT('Ctrl Pts',(-7.27603390513785,3.25601574575801,-4.20082013374671));
#22501=CARTESIAN_POINT('Ctrl Pts',(-9.70137854017372,3.43101574575802,1.74701493417668E-11));
#22502=CARTESIAN_POINT('Ctrl Pts',(-7.27603390512272,3.60601574575803,4.20082013377292));
#22503=CARTESIAN_POINT('Ctrl Pts',(-4.85068927007173,3.78101574575801,8.40164026752836));
#22504=CARTESIAN_POINT('Ctrl Pts',(1.5129078685785E-11,3.95601574575802,
8.40164026751963));
#22505=CARTESIAN_POINT('Ctrl Pts',(4.85068927010198,4.13101574575802,8.4016402675109));
#22506=CARTESIAN_POINT('Ctrl Pts',(7.27603390513785,4.30601574575801,4.20082013374672));
#22507=CARTESIAN_POINT('Ctrl Pts',(9.70137854017372,4.48101574575801,-1.74689612655491E-11));
#22508=CARTESIAN_POINT('Ctrl Pts',(7.27603390512273,4.65601574575802,-4.20082013377291));
#22509=CARTESIAN_POINT('Ctrl Pts',(4.85068927007173,4.831015745758,-8.40164026752836));
#22510=CARTESIAN_POINT('Ctrl Pts',(-1.51301075899711E-11,5.00601574575801,
-8.40164026751963));
#22511=CARTESIAN_POINT('Ctrl Pts',(-4.85068927010199,5.18101574575802,-8.4016402675109));
#22512=CARTESIAN_POINT('Ctrl Pts',(-7.27603390513785,5.356015745758,-4.20082013374671));
#22513=CARTESIAN_POINT('Ctrl Pts',(-9.70137854017372,5.53101574575801,1.74701493417668E-11));
#22514=CARTESIAN_POINT('Ctrl Pts',(-7.27603390512272,5.70601574575802,4.20082013377292));
#22515=CARTESIAN_POINT('Ctrl Pts',(-4.85068927007173,5.881015745758,8.40164026752836));
#22516=CARTESIAN_POINT('Ctrl Pts',(1.5129078685785E-11,6.05601574575801,
8.40164026751963));
#22517=CARTESIAN_POINT('Ctrl Pts',(4.85068927010198,6.23101574575801,8.4016402675109));
#22518=CARTESIAN_POINT('Ctrl Pts',(7.27603390513785,6.40601574575803,4.20082013374672));
#22519=CARTESIAN_POINT('Ctrl Pts',(9.70137854017372,6.581015745758,-1.74689612655491E-11));
#22520=CARTESIAN_POINT('Ctrl Pts',(7.27603390512273,6.75601574575802,-4.20082013377291));
#22521=CARTESIAN_POINT('Ctrl Pts',(4.85068927007173,6.93101574575802,-8.40164026752836));
#22522=CARTESIAN_POINT('Ctrl Pts',(-1.51301075899711E-11,7.106015745758,
-8.40164026751963));
#22523=CARTESIAN_POINT('Ctrl Pts',(-4.85068927010199,7.28101574575801,-8.4016402675109));
#22524=CARTESIAN_POINT('Ctrl Pts',(-7.27603390513785,7.45601574575802,-4.20082013374671));
#22525=CARTESIAN_POINT('Ctrl Pts',(-9.70137854017372,7.631015745758,1.74701493417668E-11));
#22526=CARTESIAN_POINT('Ctrl Pts',(-7.27603390512272,7.80601574575801,4.20082013377292));
#22527=CARTESIAN_POINT('Ctrl Pts',(-4.85068927007173,7.98101574575801,8.40164026752836));
#22528=CARTESIAN_POINT('Ctrl Pts',(1.5129078685785E-11,8.156015745758,8.40164026751963));
#22529=CARTESIAN_POINT('Ctrl Pts',(4.85068927010198,8.331015745758,8.4016402675109));
#22530=CARTESIAN_POINT('Ctrl Pts',(7.27603390513785,8.50601574575802,4.20082013374672));
#22531=CARTESIAN_POINT('Ctrl Pts',(9.70137854017372,8.68101574575799,-1.74689612655491E-11));
#22532=CARTESIAN_POINT('Ctrl Pts',(7.27603390512273,8.85601574575801,-4.20082013377291));
#22533=CARTESIAN_POINT('Ctrl Pts',(4.85068927007173,9.03101574575801,-8.40164026752836));
#22534=CARTESIAN_POINT('Ctrl Pts',(-1.51301075899711E-11,9.20601574575799,
-8.40164026751963));
#22535=CARTESIAN_POINT('Ctrl Pts',(-4.85068927010199,9.381015745758,-8.4016402675109));
#22536=CARTESIAN_POINT('Ctrl Pts',(-7.27603390513785,9.55601574575801,-4.20082013374671));
#22537=CARTESIAN_POINT('Ctrl Pts',(-9.70137854017372,9.73101574575799,1.74701493417668E-11));
#22538=CARTESIAN_POINT('Ctrl Pts',(-7.27603390512272,9.906015745758,4.20082013377292));
#22539=CARTESIAN_POINT('Ctrl Pts',(-4.85068927007173,10.081015745758,8.40164026752836));
#22540=CARTESIAN_POINT('Ctrl Pts',(1.5129078685785E-11,10.256015745758,
8.40164026751963));
#22541=CARTESIAN_POINT('Ctrl Pts',(4.85068927010198,10.431015745758,8.4016402675109));
#22542=CARTESIAN_POINT('Ctrl Pts',(7.27603390513785,10.606015745758,4.20082013374672));
#22543=CARTESIAN_POINT('Ctrl Pts',(9.70137854017372,10.781015745758,-1.74689612655491E-11));
#22544=CARTESIAN_POINT('Ctrl Pts',(7.27603390512273,10.956015745758,-4.20082013377291));
#22545=CARTESIAN_POINT('Ctrl Pts',(4.85068927007173,11.131015745758,-8.40164026752836));
#22546=CARTESIAN_POINT('Ctrl Pts',(-1.51301075899711E-11,11.306015745758,
-8.40164026751963));
#22547=CARTESIAN_POINT('Ctrl Pts',(-4.85068927010199,11.481015745758,-8.4016402675109));
#22548=CARTESIAN_POINT('Ctrl Pts',(-7.27603390513785,11.656015745758,-4.20082013374671));
#22549=CARTESIAN_POINT('Ctrl Pts',(-9.70137854017372,11.831015745758,1.74701493417668E-11));
#22550=CARTESIAN_POINT('Ctrl Pts',(-7.27603390512272,12.006015745758,4.20082013377292));
#22551=CARTESIAN_POINT('Ctrl Pts',(-4.85068927007173,12.181015745758,8.40164026752836));
#22552=CARTESIAN_POINT('Ctrl Pts',(1.5129078685785E-11,12.356015745758,
8.40164026751963));
#22553=CARTESIAN_POINT('Ctrl Pts',(4.85068927010198,12.531015745758,8.4016402675109));
#22554=CARTESIAN_POINT('Ctrl Pts',(7.27603390513785,12.706015745758,4.20082013374672));
#22555=CARTESIAN_POINT('Ctrl Pts',(9.70137854017372,12.881015745758,-1.74689612655491E-11));
#22556=CARTESIAN_POINT('Ctrl Pts',(7.27603390512273,13.056015745758,-4.20082013377291));
#22557=CARTESIAN_POINT('Ctrl Pts',(4.85068927007173,13.231015745758,-8.40164026752836));
#22558=CARTESIAN_POINT('Ctrl Pts',(-1.51301075899711E-11,13.406015745758,
-8.40164026751963));
#22559=CARTESIAN_POINT('Ctrl Pts',(-4.85068927010199,13.581015745758,-8.4016402675109));
#22560=CARTESIAN_POINT('Ctrl Pts',(-7.27603390513785,13.756015745758,-4.20082013374671));
#22561=CARTESIAN_POINT('Ctrl Pts',(-9.70137854017372,13.931015745758,1.74701493417668E-11));
#22562=CARTESIAN_POINT('Ctrl Pts',(-7.27603390512272,14.106015745758,4.20082013377292));
#22563=CARTESIAN_POINT('Ctrl Pts',(-4.85068927007173,14.281015745758,8.40164026752836));
#22564=CARTESIAN_POINT('Ctrl Pts',(1.5129078685785E-11,14.456015745758,
8.40164026751963));
#22565=CARTESIAN_POINT('Ctrl Pts',(4.85068927010198,14.631015745758,8.4016402675109));
#22566=CARTESIAN_POINT('Ctrl Pts',(7.27603390513785,14.806015745758,4.20082013374672));
#22567=CARTESIAN_POINT('Ctrl Pts',(9.70137854017372,14.981015745758,-1.74689612655491E-11));
#22568=CARTESIAN_POINT('Ctrl Pts',(7.27603390512273,15.156015745758,-4.20082013377291));
#22569=CARTESIAN_POINT('Ctrl Pts',(4.85068927007173,15.331015745758,-8.40164026752836));
#22570=CARTESIAN_POINT('Ctrl Pts',(-1.51301075899711E-11,15.506015745758,
-8.40164026751963));
#22571=CARTESIAN_POINT('Ctrl Pts',(-4.85068927010199,15.681015745758,-8.4016402675109));
#22572=CARTESIAN_POINT('Ctrl Pts',(-7.27603390513785,15.856015745758,-4.20082013374671));
#22573=CARTESIAN_POINT('Ctrl Pts',(-9.70137854017372,16.031015745758,1.74701493417668E-11));
#22574=CARTESIAN_POINT('Ctrl Pts',(-7.27603390512272,16.206015745758,4.20082013377292));
#22575=CARTESIAN_POINT('Ctrl Pts',(-4.85068927007173,16.381015745758,8.40164026752836));
#22576=CARTESIAN_POINT('Ctrl Pts',(1.5129078685785E-11,16.556015745758,
8.40164026751963));
#22577=CARTESIAN_POINT('Ctrl Pts',(4.85068927010198,16.731015745758,8.4016402675109));
#22578=CARTESIAN_POINT('Ctrl Pts',(7.27603390513785,16.906015745758,4.20082013374672));
#22579=CARTESIAN_POINT('Ctrl Pts',(9.70137854017372,17.081015745758,-1.74689612655491E-11));
#22580=CARTESIAN_POINT('Ctrl Pts',(7.27603390512273,17.256015745758,-4.20082013377291));
#22581=CARTESIAN_POINT('Ctrl Pts',(4.85068927007173,17.431015745758,-8.40164026752836));
#22582=CARTESIAN_POINT('Ctrl Pts',(-1.51301075899711E-11,17.606015745758,
-8.40164026751963));
#22583=CARTESIAN_POINT('Ctrl Pts',(-4.85068927010199,17.781015745758,-8.4016402675109));
#22584=CARTESIAN_POINT('Ctrl Pts',(-7.27603390513785,17.956015745758,-4.20082013374671));
#22585=CARTESIAN_POINT('Ctrl Pts',(-9.70137854017372,18.131015745758,1.74701493417668E-11));
#22586=CARTESIAN_POINT('Ctrl Pts',(-7.27603390512272,18.306015745758,4.20082013377292));
#22587=CARTESIAN_POINT('Ctrl Pts',(-4.85068927007173,18.481015745758,8.40164026752836));
#22588=CARTESIAN_POINT('Ctrl Pts',(1.5129078685785E-11,18.656015745758,
8.40164026751963));
#22589=CARTESIAN_POINT('Ctrl Pts',(4.85068927010198,18.831015745758,8.4016402675109));
#22590=CARTESIAN_POINT('Ctrl Pts',(7.27603390513785,19.006015745758,4.20082013374672));
#22591=CARTESIAN_POINT('Ctrl Pts',(9.70137854017372,19.181015745758,-1.74689612655491E-11));
#22592=CARTESIAN_POINT('Ctrl Pts',(7.27603390512273,19.356015745758,-4.20082013377291));
#22593=CARTESIAN_POINT('Ctrl Pts',(4.85068927007173,19.531015745758,-8.40164026752836));
#22594=CARTESIAN_POINT('Ctrl Pts',(-1.51301075899711E-11,19.706015745758,
-8.40164026751963));
#22595=CARTESIAN_POINT('Ctrl Pts',(-4.85068927010199,19.881015745758,-8.4016402675109));
#22596=CARTESIAN_POINT('Ctrl Pts',(-7.27603390513785,20.056015745758,-4.20082013374671));
#22597=CARTESIAN_POINT('Ctrl Pts',(-9.70137854017372,20.231015745758,1.74701493417668E-11));
#22598=CARTESIAN_POINT('Ctrl Pts',(-7.27603390512272,20.406015745758,4.20082013377292));
#22599=CARTESIAN_POINT('Ctrl Pts',(-4.85068927007173,20.581015745758,8.40164026752836));
#22600=CARTESIAN_POINT('Ctrl Pts',(1.5129078685785E-11,20.756015745758,
8.40164026751963));
#22601=CARTESIAN_POINT('Ctrl Pts',(4.85068927010198,20.931015745758,8.4016402675109));
#22602=CARTESIAN_POINT('Ctrl Pts',(7.27603390513785,21.106015745758,4.20082013374672));
#22603=CARTESIAN_POINT('Ctrl Pts',(9.70137854017372,21.281015745758,-1.74689612655491E-11));
#22604=CARTESIAN_POINT('Ctrl Pts',(7.27603390512273,21.456015745758,-4.20082013377291));
#22605=CARTESIAN_POINT('Ctrl Pts',(4.85068927007173,21.631015745758,-8.40164026752836));
#22606=CARTESIAN_POINT('Ctrl Pts',(-1.51301075899711E-11,21.806015745758,
-8.40164026751963));
#22607=CARTESIAN_POINT('Ctrl Pts',(-4.85068927010199,21.981015745758,-8.4016402675109));
#22608=CARTESIAN_POINT('Ctrl Pts',(-7.27603390513785,22.156015745758,-4.20082013374671));
#22609=CARTESIAN_POINT('Ctrl Pts',(-9.70137854017372,22.331015745758,1.74701493417668E-11));
#22610=CARTESIAN_POINT('Ctrl Pts',(-7.27603390512272,22.506015745758,4.20082013377292));
#22611=CARTESIAN_POINT('Ctrl Pts',(-4.85068927007173,22.681015745758,8.40164026752836));
#22612=CARTESIAN_POINT('Ctrl Pts',(1.5129078685785E-11,22.856015745758,
8.40164026751963));
#22613=CARTESIAN_POINT('Ctrl Pts',(4.85068927010198,23.031015745758,8.4016402675109));
#22614=CARTESIAN_POINT('Ctrl Pts',(7.27603390513785,23.206015745758,4.20082013374672));
#22615=CARTESIAN_POINT('Ctrl Pts',(9.70137854017372,23.381015745758,-1.74689612655491E-11));
#22616=CARTESIAN_POINT('Ctrl Pts',(7.27603390512273,23.556015745758,-4.20082013377291));
#22617=CARTESIAN_POINT('Ctrl Pts',(4.85068927007173,23.731015745758,-8.40164026752836));
#22618=CARTESIAN_POINT('Ctrl Pts',(-1.51301075899711E-11,23.906015745758,
-8.40164026751963));
#22619=CARTESIAN_POINT('Ctrl Pts',(-4.85068927010199,24.081015745758,-8.4016402675109));
#22620=CARTESIAN_POINT('Ctrl Pts',(-7.27603390513785,24.256015745758,-4.20082013374671));
#22621=CARTESIAN_POINT('Ctrl Pts',(-9.70137854017372,24.431015745758,1.74701493417668E-11));
#22622=CARTESIAN_POINT('Ctrl Pts',(-7.27603390512272,24.606015745758,4.20082013377292));
#22623=CARTESIAN_POINT('Ctrl Pts',(-4.85068927007173,24.781015745758,8.40164026752836));
#22624=CARTESIAN_POINT('Ctrl Pts',(1.5129078685785E-11,24.956015745758,
8.40164026751963));
#22625=CARTESIAN_POINT('Ctrl Pts',(4.85068927010198,25.131015745758,8.4016402675109));
#22626=CARTESIAN_POINT('Ctrl Pts',(7.27603390513785,25.306015745758,4.20082013374672));
#22627=CARTESIAN_POINT('Ctrl Pts',(9.70137854017372,25.481015745758,-1.74689612655491E-11));
#22628=CARTESIAN_POINT('Ctrl Pts',(7.27603390512273,25.656015745758,-4.20082013377291));
#22629=CARTESIAN_POINT('Ctrl Pts',(4.85068927007173,25.831015745758,-8.40164026752836));
#22630=CARTESIAN_POINT('Ctrl Pts',(-1.51301075899711E-11,26.006015745758,
-8.40164026751963));
#22631=CARTESIAN_POINT('Ctrl Pts',(-1.4702867290402E-11,-143.970483118095,
-8.16439679232146));
#22632=CARTESIAN_POINT('Ctrl Pts',(-4.71371668583241,-143.795483118095,
-8.16439679231297));
#22633=CARTESIAN_POINT('Ctrl Pts',(-7.07057502873392,-143.620483118095,
-4.082198396148));
#22634=CARTESIAN_POINT('Ctrl Pts',(-9.42743337163542,-143.445483118095,
1.69768315121407E-11));
#22635=CARTESIAN_POINT('Ctrl Pts',(-7.07057502871922,-143.270483118095,
4.08219839617346));
#22636=CARTESIAN_POINT('Ctrl Pts',(-4.71371668580301,-143.095483118095,
8.16439679232994));
#22637=CARTESIAN_POINT('Ctrl Pts',(1.47018674401621E-11,-142.920483118095,
8.16439679232146));
#22638=CARTESIAN_POINT('Ctrl Pts',(4.71371668583241,-142.745483118095,8.16439679231297));
#22639=CARTESIAN_POINT('Ctrl Pts',(7.07057502873392,-142.570483118095,4.082198396148));
#22640=CARTESIAN_POINT('Ctrl Pts',(9.42743337163542,-142.395483118095,-1.69756769845304E-11));
#22641=CARTESIAN_POINT('Ctrl Pts',(7.07057502871922,-142.220483118095,-4.08219839617346));
#22642=CARTESIAN_POINT('Ctrl Pts',(4.71371668580301,-142.045483118095,-8.16439679232994));
#22643=CARTESIAN_POINT('Ctrl Pts',(-1.4702867290402E-11,-141.870483118095,
-8.16439679232146));
#22644=CARTESIAN_POINT('Ctrl Pts',(-4.71371668583241,-141.695483118095,
-8.16439679231297));
#22645=CARTESIAN_POINT('Ctrl Pts',(-7.07057502873392,-141.520483118095,
-4.082198396148));
#22646=CARTESIAN_POINT('Ctrl Pts',(-9.42743337163542,-141.345483118095,
1.69768315121407E-11));
#22647=CARTESIAN_POINT('Ctrl Pts',(-7.07057502871922,-141.170483118095,
4.08219839617346));
#22648=CARTESIAN_POINT('Ctrl Pts',(-4.71371668580301,-140.995483118095,
8.16439679232994));
#22649=CARTESIAN_POINT('Ctrl Pts',(1.47018674401621E-11,-140.820483118095,
8.16439679232146));
#22650=CARTESIAN_POINT('Ctrl Pts',(4.71371668583241,-140.645483118095,8.16439679231297));
#22651=CARTESIAN_POINT('Ctrl Pts',(7.07057502873392,-140.470483118095,4.082198396148));
#22652=CARTESIAN_POINT('Ctrl Pts',(9.42743337163542,-140.295483118095,-1.69756769845304E-11));
#22653=CARTESIAN_POINT('Ctrl Pts',(7.07057502871922,-140.120483118095,-4.08219839617346));
#22654=CARTESIAN_POINT('Ctrl Pts',(4.71371668580301,-139.945483118095,-8.16439679232994));
#22655=CARTESIAN_POINT('Ctrl Pts',(-1.4702867290402E-11,-139.770483118095,
-8.16439679232146));
#22656=CARTESIAN_POINT('Ctrl Pts',(-4.71371668583241,-139.595483118095,
-8.16439679231297));
#22657=CARTESIAN_POINT('Ctrl Pts',(-7.07057502873392,-139.420483118095,
-4.082198396148));
#22658=CARTESIAN_POINT('Ctrl Pts',(-9.42743337163542,-139.245483118095,
1.69768315121407E-11));
#22659=CARTESIAN_POINT('Ctrl Pts',(-7.07057502871922,-139.070483118095,
4.08219839617346));
#22660=CARTESIAN_POINT('Ctrl Pts',(-4.71371668580301,-138.895483118095,
8.16439679232994));
#22661=CARTESIAN_POINT('Ctrl Pts',(1.47018674401621E-11,-138.720483118095,
8.16439679232146));
#22662=CARTESIAN_POINT('Ctrl Pts',(4.71371668583241,-138.545483118095,8.16439679231297));
#22663=CARTESIAN_POINT('Ctrl Pts',(7.07057502873392,-138.370483118095,4.082198396148));
#22664=CARTESIAN_POINT('Ctrl Pts',(9.42743337163542,-138.195483118095,-1.69756769845304E-11));
#22665=CARTESIAN_POINT('Ctrl Pts',(7.07057502871922,-138.020483118095,-4.08219839617346));
#22666=CARTESIAN_POINT('Ctrl Pts',(4.71371668580301,-137.845483118095,-8.16439679232994));
#22667=CARTESIAN_POINT('Ctrl Pts',(-1.4702867290402E-11,-137.670483118095,
-8.16439679232146));
#22668=CARTESIAN_POINT('Ctrl Pts',(-4.71371668583241,-137.495483118095,
-8.16439679231297));
#22669=CARTESIAN_POINT('Ctrl Pts',(-7.07057502873392,-137.320483118095,
-4.082198396148));
#22670=CARTESIAN_POINT('Ctrl Pts',(-9.42743337163542,-137.145483118095,
1.69768315121407E-11));
#22671=CARTESIAN_POINT('Ctrl Pts',(-7.07057502871922,-136.970483118095,
4.08219839617346));
#22672=CARTESIAN_POINT('Ctrl Pts',(-4.71371668580301,-136.795483118095,
8.16439679232994));
#22673=CARTESIAN_POINT('Ctrl Pts',(1.47018674401621E-11,-136.620483118095,
8.16439679232146));
#22674=CARTESIAN_POINT('Ctrl Pts',(4.71371668583241,-136.445483118095,8.16439679231297));
#22675=CARTESIAN_POINT('Ctrl Pts',(7.07057502873392,-136.270483118095,4.082198396148));
#22676=CARTESIAN_POINT('Ctrl Pts',(9.42743337163542,-136.095483118095,-1.69756769845304E-11));
#22677=CARTESIAN_POINT('Ctrl Pts',(7.07057502871922,-135.920483118095,-4.08219839617346));
#22678=CARTESIAN_POINT('Ctrl Pts',(4.71371668580301,-135.745483118095,-8.16439679232994));
#22679=CARTESIAN_POINT('Ctrl Pts',(-1.4702867290402E-11,-135.570483118095,
-8.16439679232146));
#22680=CARTESIAN_POINT('Ctrl Pts',(-4.71371668583241,-135.395483118095,
-8.16439679231297));
#22681=CARTESIAN_POINT('Ctrl Pts',(-7.07057502873392,-135.220483118095,
-4.082198396148));
#22682=CARTESIAN_POINT('Ctrl Pts',(-9.42743337163542,-135.045483118095,
1.69768315121407E-11));
#22683=CARTESIAN_POINT('Ctrl Pts',(-7.07057502871922,-134.870483118095,
4.08219839617346));
#22684=CARTESIAN_POINT('Ctrl Pts',(-4.71371668580301,-134.695483118095,
8.16439679232994));
#22685=CARTESIAN_POINT('Ctrl Pts',(1.47018674401621E-11,-134.520483118095,
8.16439679232146));
#22686=CARTESIAN_POINT('Ctrl Pts',(4.71371668583241,-134.345483118095,8.16439679231297));
#22687=CARTESIAN_POINT('Ctrl Pts',(7.07057502873392,-134.170483118095,4.082198396148));
#22688=CARTESIAN_POINT('Ctrl Pts',(9.42743337163542,-133.995483118095,-1.69756769845304E-11));
#22689=CARTESIAN_POINT('Ctrl Pts',(7.07057502871922,-133.820483118095,-4.08219839617346));
#22690=CARTESIAN_POINT('Ctrl Pts',(4.71371668580301,-133.645483118095,-8.16439679232994));
#22691=CARTESIAN_POINT('Ctrl Pts',(-1.4702867290402E-11,-133.470483118095,
-8.16439679232146));
#22692=CARTESIAN_POINT('Ctrl Pts',(-4.71371668583241,-133.295483118095,
-8.16439679231297));
#22693=CARTESIAN_POINT('Ctrl Pts',(-7.07057502873392,-133.120483118095,
-4.082198396148));
#22694=CARTESIAN_POINT('Ctrl Pts',(-9.42743337163542,-132.945483118095,
1.69768315121407E-11));
#22695=CARTESIAN_POINT('Ctrl Pts',(-7.07057502871922,-132.770483118095,
4.08219839617346));
#22696=CARTESIAN_POINT('Ctrl Pts',(-4.71371668580301,-132.595483118095,
8.16439679232994));
#22697=CARTESIAN_POINT('Ctrl Pts',(1.47018674401621E-11,-132.420483118095,
8.16439679232146));
#22698=CARTESIAN_POINT('Ctrl Pts',(4.71371668583241,-132.245483118095,8.16439679231297));
#22699=CARTESIAN_POINT('Ctrl Pts',(7.07057502873392,-132.070483118095,4.082198396148));
#22700=CARTESIAN_POINT('Ctrl Pts',(9.42743337163542,-131.895483118095,-1.69756769845304E-11));
#22701=CARTESIAN_POINT('Ctrl Pts',(7.07057502871922,-131.720483118095,-4.08219839617346));
#22702=CARTESIAN_POINT('Ctrl Pts',(4.71371668580301,-131.545483118095,-8.16439679232994));
#22703=CARTESIAN_POINT('Ctrl Pts',(-1.4702867290402E-11,-131.370483118095,
-8.16439679232146));
#22704=CARTESIAN_POINT('Ctrl Pts',(-4.71371668583241,-131.195483118095,
-8.16439679231297));
#22705=CARTESIAN_POINT('Ctrl Pts',(-7.07057502873392,-131.020483118095,
-4.082198396148));
#22706=CARTESIAN_POINT('Ctrl Pts',(-9.42743337163542,-130.845483118095,
1.69768315121407E-11));
#22707=CARTESIAN_POINT('Ctrl Pts',(-7.07057502871922,-130.670483118095,
4.08219839617346));
#22708=CARTESIAN_POINT('Ctrl Pts',(-4.71371668580301,-130.495483118095,
8.16439679232994));
#22709=CARTESIAN_POINT('Ctrl Pts',(1.47018674401621E-11,-130.320483118095,
8.16439679232146));
#22710=CARTESIAN_POINT('Ctrl Pts',(4.71371668583241,-130.145483118095,8.16439679231297));
#22711=CARTESIAN_POINT('Ctrl Pts',(7.07057502873392,-129.970483118095,4.082198396148));
#22712=CARTESIAN_POINT('Ctrl Pts',(9.42743337163542,-129.795483118095,-1.69756769845304E-11));
#22713=CARTESIAN_POINT('Ctrl Pts',(7.07057502871922,-129.620483118095,-4.08219839617346));
#22714=CARTESIAN_POINT('Ctrl Pts',(4.71371668580301,-129.445483118095,-8.16439679232994));
#22715=CARTESIAN_POINT('Ctrl Pts',(-1.4702867290402E-11,-129.270483118095,
-8.16439679232146));
#22716=CARTESIAN_POINT('Ctrl Pts',(-4.71371668583241,-129.095483118095,
-8.16439679231297));
#22717=CARTESIAN_POINT('Ctrl Pts',(-7.07057502873392,-128.920483118095,
-4.082198396148));
#22718=CARTESIAN_POINT('Ctrl Pts',(-9.42743337163542,-128.745483118095,
1.69768315121407E-11));
#22719=CARTESIAN_POINT('Ctrl Pts',(-7.07057502871922,-128.570483118095,
4.08219839617346));
#22720=CARTESIAN_POINT('Ctrl Pts',(-4.71371668580301,-128.395483118095,
8.16439679232994));
#22721=CARTESIAN_POINT('Ctrl Pts',(1.47018674401621E-11,-128.220483118095,
8.16439679232146));
#22722=CARTESIAN_POINT('Ctrl Pts',(4.71371668583241,-128.045483118095,8.16439679231297));
#22723=CARTESIAN_POINT('Ctrl Pts',(7.07057502873392,-127.870483118095,4.082198396148));
#22724=CARTESIAN_POINT('Ctrl Pts',(9.42743337163542,-127.695483118095,-1.69756769845304E-11));
#22725=CARTESIAN_POINT('Ctrl Pts',(7.07057502871922,-127.520483118095,-4.08219839617346));
#22726=CARTESIAN_POINT('Ctrl Pts',(4.71371668580301,-127.345483118095,-8.16439679232994));
#22727=CARTESIAN_POINT('Ctrl Pts',(-1.4702867290402E-11,-127.170483118095,
-8.16439679232146));
#22728=CARTESIAN_POINT('Ctrl Pts',(-4.71371668583241,-126.995483118095,
-8.16439679231297));
#22729=CARTESIAN_POINT('Ctrl Pts',(-7.07057502873392,-126.820483118095,
-4.082198396148));
#22730=CARTESIAN_POINT('Ctrl Pts',(-9.42743337163542,-126.645483118095,
1.69768315121407E-11));
#22731=CARTESIAN_POINT('Ctrl Pts',(-7.07057502871922,-126.470483118095,
4.08219839617346));
#22732=CARTESIAN_POINT('Ctrl Pts',(-4.71371668580301,-126.295483118095,
8.16439679232994));
#22733=CARTESIAN_POINT('Ctrl Pts',(1.47018674401621E-11,-126.120483118095,
8.16439679232146));
#22734=CARTESIAN_POINT('Ctrl Pts',(4.71371668583241,-125.945483118095,8.16439679231297));
#22735=CARTESIAN_POINT('Ctrl Pts',(7.07057502873392,-125.770483118095,4.082198396148));
#22736=CARTESIAN_POINT('Ctrl Pts',(9.42743337163542,-125.595483118095,-1.69756769845304E-11));
#22737=CARTESIAN_POINT('Ctrl Pts',(7.07057502871922,-125.420483118095,-4.08219839617346));
#22738=CARTESIAN_POINT('Ctrl Pts',(4.71371668580301,-125.245483118095,-8.16439679232994));
#22739=CARTESIAN_POINT('Ctrl Pts',(-1.4702867290402E-11,-125.070483118095,
-8.16439679232146));
#22740=CARTESIAN_POINT('Ctrl Pts',(-4.71371668583241,-124.895483118095,
-8.16439679231297));
#22741=CARTESIAN_POINT('Ctrl Pts',(-7.07057502873392,-124.720483118095,
-4.082198396148));
#22742=CARTESIAN_POINT('Ctrl Pts',(-9.42743337163542,-124.545483118095,
1.69768315121407E-11));
#22743=CARTESIAN_POINT('Ctrl Pts',(-7.07057502871922,-124.370483118095,
4.08219839617346));
#22744=CARTESIAN_POINT('Ctrl Pts',(-4.71371668580301,-124.195483118095,
8.16439679232994));
#22745=CARTESIAN_POINT('Ctrl Pts',(1.47018674401621E-11,-124.020483118095,
8.16439679232146));
#22746=CARTESIAN_POINT('Ctrl Pts',(4.71371668583241,-123.845483118095,8.16439679231297));
#22747=CARTESIAN_POINT('Ctrl Pts',(7.07057502873392,-123.670483118095,4.082198396148));
#22748=CARTESIAN_POINT('Ctrl Pts',(9.42743337163542,-123.495483118095,-1.69756769845304E-11));
#22749=CARTESIAN_POINT('Ctrl Pts',(7.07057502871922,-123.320483118095,-4.08219839617346));
#22750=CARTESIAN_POINT('Ctrl Pts',(4.71371668580301,-123.145483118095,-8.16439679232994));
#22751=CARTESIAN_POINT('Ctrl Pts',(-1.4702867290402E-11,-122.970483118095,
-8.16439679232146));
#22752=CARTESIAN_POINT('Ctrl Pts',(-4.71371668583241,-122.795483118095,
-8.16439679231297));
#22753=CARTESIAN_POINT('Ctrl Pts',(-7.07057502873392,-122.620483118095,
-4.082198396148));
#22754=CARTESIAN_POINT('Ctrl Pts',(-9.42743337163542,-122.445483118095,
1.69768315121407E-11));
#22755=CARTESIAN_POINT('Ctrl Pts',(-7.07057502871922,-122.270483118095,
4.08219839617346));
#22756=CARTESIAN_POINT('Ctrl Pts',(-4.71371668580301,-122.095483118095,
8.16439679232994));
#22757=CARTESIAN_POINT('Ctrl Pts',(1.47018674401621E-11,-121.920483118095,
8.16439679232146));
#22758=CARTESIAN_POINT('Ctrl Pts',(4.71371668583241,-121.745483118095,8.16439679231297));
#22759=CARTESIAN_POINT('Ctrl Pts',(7.07057502873392,-121.570483118095,4.082198396148));
#22760=CARTESIAN_POINT('Ctrl Pts',(9.42743337163542,-121.395483118095,-1.69756769845304E-11));
#22761=CARTESIAN_POINT('Ctrl Pts',(7.07057502871922,-121.220483118095,-4.08219839617346));
#22762=CARTESIAN_POINT('Ctrl Pts',(4.71371668580301,-121.045483118095,-8.16439679232994));
#22763=CARTESIAN_POINT('Ctrl Pts',(-1.4702867290402E-11,-120.870483118095,
-8.16439679232146));
#22764=CARTESIAN_POINT('Ctrl Pts',(-4.71371668583241,-120.695483118095,
-8.16439679231297));
#22765=CARTESIAN_POINT('Ctrl Pts',(-7.07057502873392,-120.520483118095,
-4.082198396148));
#22766=CARTESIAN_POINT('Ctrl Pts',(-9.42743337163542,-120.345483118095,
1.69768315121407E-11));
#22767=CARTESIAN_POINT('Ctrl Pts',(-7.07057502871922,-120.170483118095,
4.08219839617346));
#22768=CARTESIAN_POINT('Ctrl Pts',(-4.71371668580301,-119.995483118095,
8.16439679232994));
#22769=CARTESIAN_POINT('Ctrl Pts',(1.47018674401621E-11,-119.820483118095,
8.16439679232146));
#22770=CARTESIAN_POINT('Ctrl Pts',(4.71371668583241,-119.645483118095,8.16439679231297));
#22771=CARTESIAN_POINT('Ctrl Pts',(7.07057502873392,-119.470483118095,4.082198396148));
#22772=CARTESIAN_POINT('Ctrl Pts',(9.42743337163542,-119.295483118095,-1.69756769845304E-11));
#22773=CARTESIAN_POINT('Ctrl Pts',(7.07057502871922,-119.120483118095,-4.08219839617346));
#22774=CARTESIAN_POINT('Ctrl Pts',(4.71371668580301,-118.945483118095,-8.16439679232994));
#22775=CARTESIAN_POINT('Ctrl Pts',(-1.4702867290402E-11,-118.770483118095,
-8.16439679232146));
#22776=CARTESIAN_POINT('Ctrl Pts',(-4.71371668583241,-118.595483118095,
-8.16439679231297));
#22777=CARTESIAN_POINT('Ctrl Pts',(-7.07057502873392,-118.420483118095,
-4.082198396148));
#22778=CARTESIAN_POINT('Ctrl Pts',(-9.42743337163542,-118.245483118095,
1.69768315121407E-11));
#22779=CARTESIAN_POINT('Ctrl Pts',(-7.07057502871922,-118.070483118095,
4.08219839617346));
#22780=CARTESIAN_POINT('Ctrl Pts',(-4.71371668580301,-117.895483118095,
8.16439679232994));
#22781=CARTESIAN_POINT('Ctrl Pts',(1.47018674401621E-11,-117.720483118095,
8.16439679232146));
#22782=CARTESIAN_POINT('Ctrl Pts',(4.71371668583241,-117.545483118095,8.16439679231297));
#22783=CARTESIAN_POINT('Ctrl Pts',(7.07057502873392,-117.370483118095,4.082198396148));
#22784=CARTESIAN_POINT('Ctrl Pts',(9.42743337163542,-117.195483118095,-1.69756769845304E-11));
#22785=CARTESIAN_POINT('Ctrl Pts',(7.07057502871922,-117.020483118095,-4.08219839617346));
#22786=CARTESIAN_POINT('Ctrl Pts',(4.71371668580301,-116.845483118095,-8.16439679232994));
#22787=CARTESIAN_POINT('Ctrl Pts',(-1.4702867290402E-11,-116.670483118095,
-8.16439679232146));
#22788=CARTESIAN_POINT('Ctrl Pts',(-4.71371668583241,-116.495483118095,
-8.16439679231297));
#22789=CARTESIAN_POINT('Ctrl Pts',(-7.07057502873392,-116.320483118095,
-4.082198396148));
#22790=CARTESIAN_POINT('Ctrl Pts',(-9.42743337163542,-116.145483118095,
1.69768315121407E-11));
#22791=CARTESIAN_POINT('Ctrl Pts',(-7.07057502871922,-115.970483118095,
4.08219839617346));
#22792=CARTESIAN_POINT('Ctrl Pts',(-4.71371668580301,-115.795483118095,
8.16439679232994));
#22793=CARTESIAN_POINT('Ctrl Pts',(1.47018674401621E-11,-115.620483118095,
8.16439679232146));
#22794=CARTESIAN_POINT('Ctrl Pts',(4.71371668583241,-115.445483118095,8.16439679231297));
#22795=CARTESIAN_POINT('Ctrl Pts',(7.07057502873392,-115.270483118095,4.082198396148));
#22796=CARTESIAN_POINT('Ctrl Pts',(9.42743337163542,-115.095483118095,-1.69756769845304E-11));
#22797=CARTESIAN_POINT('Ctrl Pts',(7.07057502871922,-114.920483118095,-4.08219839617346));
#22798=CARTESIAN_POINT('Ctrl Pts',(4.71371668580301,-114.745483118095,-8.16439679232994));
#22799=CARTESIAN_POINT('Ctrl Pts',(-1.4702867290402E-11,-114.570483118095,
-8.16439679232146));
#22800=CARTESIAN_POINT('Ctrl Pts',(-4.71371668583241,-114.395483118095,
-8.16439679231297));
#22801=CARTESIAN_POINT('Ctrl Pts',(-7.07057502873392,-114.220483118095,
-4.082198396148));
#22802=CARTESIAN_POINT('Ctrl Pts',(-9.42743337163542,-114.045483118095,
1.69768315121407E-11));
#22803=CARTESIAN_POINT('Ctrl Pts',(-7.07057502871922,-113.870483118095,
4.08219839617346));
#22804=CARTESIAN_POINT('Ctrl Pts',(-4.71371668580301,-113.695483118095,
8.16439679232994));
#22805=CARTESIAN_POINT('Ctrl Pts',(1.47018674401621E-11,-113.520483118095,
8.16439679232146));
#22806=CARTESIAN_POINT('Ctrl Pts',(4.71371668583241,-113.345483118095,8.16439679231297));
#22807=CARTESIAN_POINT('Ctrl Pts',(7.07057502873392,-113.170483118095,4.082198396148));
#22808=CARTESIAN_POINT('Ctrl Pts',(9.42743337163542,-112.995483118095,-1.69756769845304E-11));
#22809=CARTESIAN_POINT('Ctrl Pts',(7.07057502871922,-112.820483118095,-4.08219839617346));
#22810=CARTESIAN_POINT('Ctrl Pts',(4.71371668580301,-112.645483118095,-8.16439679232994));
#22811=CARTESIAN_POINT('Ctrl Pts',(-1.4702867290402E-11,-112.470483118095,
-8.16439679232146));
#22812=CARTESIAN_POINT('Ctrl Pts',(-4.71371668583241,-112.295483118095,
-8.16439679231297));
#22813=CARTESIAN_POINT('Ctrl Pts',(-7.07057502873392,-112.120483118095,
-4.082198396148));
#22814=CARTESIAN_POINT('Ctrl Pts',(-9.42743337163542,-111.945483118095,
1.69768315121407E-11));
#22815=CARTESIAN_POINT('Ctrl Pts',(-7.07057502871922,-111.770483118095,
4.08219839617346));
#22816=CARTESIAN_POINT('Ctrl Pts',(-4.71371668580301,-111.595483118095,
8.16439679232994));
#22817=CARTESIAN_POINT('Ctrl Pts',(1.47018674401621E-11,-111.420483118095,
8.16439679232146));
#22818=CARTESIAN_POINT('Ctrl Pts',(4.71371668583241,-111.245483118095,8.16439679231297));
#22819=CARTESIAN_POINT('Ctrl Pts',(7.07057502873392,-111.070483118095,4.082198396148));
#22820=CARTESIAN_POINT('Ctrl Pts',(9.42743337163542,-110.895483118095,-1.69756769845304E-11));
#22821=CARTESIAN_POINT('Ctrl Pts',(7.07057502871922,-110.720483118095,-4.08219839617346));
#22822=CARTESIAN_POINT('Ctrl Pts',(4.71371668580301,-110.545483118095,-8.16439679232994));
#22823=CARTESIAN_POINT('Ctrl Pts',(-1.4702867290402E-11,-110.370483118095,
-8.16439679232146));
#22824=CARTESIAN_POINT('Ctrl Pts',(-4.71371668583241,-110.195483118095,
-8.16439679231297));
#22825=CARTESIAN_POINT('Ctrl Pts',(-7.07057502873392,-110.020483118095,
-4.082198396148));
#22826=CARTESIAN_POINT('Ctrl Pts',(-9.42743337163542,-109.845483118095,
1.69768315121407E-11));
#22827=CARTESIAN_POINT('Ctrl Pts',(-7.07057502871922,-109.670483118095,
4.08219839617346));
#22828=CARTESIAN_POINT('Ctrl Pts',(-4.71371668580301,-109.495483118095,
8.16439679232994));
#22829=CARTESIAN_POINT('Ctrl Pts',(1.47018674401621E-11,-109.320483118095,
8.16439679232146));
#22830=CARTESIAN_POINT('Ctrl Pts',(4.71371668583241,-109.145483118095,8.16439679231297));
#22831=CARTESIAN_POINT('Ctrl Pts',(7.07057502873392,-108.970483118095,4.082198396148));
#22832=CARTESIAN_POINT('Ctrl Pts',(9.42743337163542,-108.795483118095,-1.69756769845304E-11));
#22833=CARTESIAN_POINT('Ctrl Pts',(7.07057502871922,-108.620483118095,-4.08219839617346));
#22834=CARTESIAN_POINT('Ctrl Pts',(4.71371668580301,-108.445483118095,-8.16439679232994));
#22835=CARTESIAN_POINT('Ctrl Pts',(-1.4702867290402E-11,-108.270483118095,
-8.16439679232146));
#22836=CARTESIAN_POINT('Ctrl Pts',(-4.71371668583241,-108.095483118095,
-8.16439679231297));
#22837=CARTESIAN_POINT('Ctrl Pts',(-7.07057502873392,-107.920483118095,
-4.082198396148));
#22838=CARTESIAN_POINT('Ctrl Pts',(-9.42743337163542,-107.745483118095,
1.69768315121407E-11));
#22839=CARTESIAN_POINT('Ctrl Pts',(-7.07057502871922,-107.570483118095,
4.08219839617346));
#22840=CARTESIAN_POINT('Ctrl Pts',(-4.71371668580301,-107.395483118095,
8.16439679232994));
#22841=CARTESIAN_POINT('Ctrl Pts',(1.47018674401621E-11,-107.220483118095,
8.16439679232146));
#22842=CARTESIAN_POINT('Ctrl Pts',(4.71371668583241,-107.045483118095,8.16439679231297));
#22843=CARTESIAN_POINT('Ctrl Pts',(7.07057502873392,-106.870483118095,4.082198396148));
#22844=CARTESIAN_POINT('Ctrl Pts',(9.42743337163542,-106.695483118095,-1.69756769845304E-11));
#22845=CARTESIAN_POINT('Ctrl Pts',(7.07057502871922,-106.520483118095,-4.08219839617346));
#22846=CARTESIAN_POINT('Ctrl Pts',(4.71371668580301,-106.345483118095,-8.16439679232994));
#22847=CARTESIAN_POINT('Ctrl Pts',(-1.4702867290402E-11,-106.170483118095,
-8.16439679232146));
#22848=CARTESIAN_POINT('Ctrl Pts',(-4.71371668583241,-105.995483118095,
-8.16439679231297));
#22849=CARTESIAN_POINT('Ctrl Pts',(-7.07057502873392,-105.820483118095,
-4.082198396148));
#22850=CARTESIAN_POINT('Ctrl Pts',(-9.42743337163542,-105.645483118095,
1.69768315121407E-11));
#22851=CARTESIAN_POINT('Ctrl Pts',(-7.07057502871922,-105.470483118095,
4.08219839617346));
#22852=CARTESIAN_POINT('Ctrl Pts',(-4.71371668580301,-105.295483118095,
8.16439679232994));
#22853=CARTESIAN_POINT('Ctrl Pts',(1.47018674401621E-11,-105.120483118095,
8.16439679232146));
#22854=CARTESIAN_POINT('Ctrl Pts',(4.71371668583241,-104.945483118095,8.16439679231297));
#22855=CARTESIAN_POINT('Ctrl Pts',(7.07057502873392,-104.770483118095,4.082198396148));
#22856=CARTESIAN_POINT('Ctrl Pts',(9.42743337163542,-104.595483118095,-1.69756769845304E-11));
#22857=CARTESIAN_POINT('Ctrl Pts',(7.07057502871922,-104.420483118095,-4.08219839617346));
#22858=CARTESIAN_POINT('Ctrl Pts',(4.71371668580301,-104.245483118095,-8.16439679232994));
#22859=CARTESIAN_POINT('Ctrl Pts',(-1.4702867290402E-11,-104.070483118095,
-8.16439679232146));
#22860=CARTESIAN_POINT('Ctrl Pts',(-4.71371668583241,-103.895483118095,
-8.16439679231297));
#22861=CARTESIAN_POINT('Ctrl Pts',(-7.07057502873392,-103.720483118095,
-4.082198396148));
#22862=CARTESIAN_POINT('Ctrl Pts',(-9.42743337163542,-103.545483118095,
1.69768315121407E-11));
#22863=CARTESIAN_POINT('Ctrl Pts',(-7.07057502871922,-103.370483118095,
4.08219839617346));
#22864=CARTESIAN_POINT('Ctrl Pts',(-4.71371668580301,-103.195483118095,
8.16439679232994));
#22865=CARTESIAN_POINT('Ctrl Pts',(1.47018674401621E-11,-103.020483118095,
8.16439679232146));
#22866=CARTESIAN_POINT('Ctrl Pts',(4.71371668583241,-102.845483118095,8.16439679231297));
#22867=CARTESIAN_POINT('Ctrl Pts',(7.07057502873392,-102.670483118095,4.082198396148));
#22868=CARTESIAN_POINT('Ctrl Pts',(9.42743337163542,-102.495483118095,-1.69756769845304E-11));
#22869=CARTESIAN_POINT('Ctrl Pts',(7.07057502871922,-102.320483118095,-4.08219839617346));
#22870=CARTESIAN_POINT('Ctrl Pts',(4.71371668580301,-102.145483118095,-8.16439679232994));
#22871=CARTESIAN_POINT('Ctrl Pts',(-1.4702867290402E-11,-101.970483118095,
-8.16439679232146));
#22872=CARTESIAN_POINT('Ctrl Pts',(-4.71371668583241,-101.795483118095,
-8.16439679231297));
#22873=CARTESIAN_POINT('Ctrl Pts',(-7.07057502873392,-101.620483118095,
-4.082198396148));
#22874=CARTESIAN_POINT('Ctrl Pts',(-9.42743337163542,-101.445483118095,
1.69768315121407E-11));
#22875=CARTESIAN_POINT('Ctrl Pts',(-7.07057502871922,-101.270483118095,
4.08219839617346));
#22876=CARTESIAN_POINT('Ctrl Pts',(-4.71371668580301,-101.095483118095,
8.16439679232994));
#22877=CARTESIAN_POINT('Ctrl Pts',(1.47018674401621E-11,-100.920483118095,
8.16439679232146));
#22878=CARTESIAN_POINT('Ctrl Pts',(4.71371668583241,-100.745483118095,8.16439679231297));
#22879=CARTESIAN_POINT('Ctrl Pts',(7.07057502873392,-100.570483118095,4.082198396148));
#22880=CARTESIAN_POINT('Ctrl Pts',(9.42743337163542,-100.395483118095,-1.69756769845304E-11));
#22881=CARTESIAN_POINT('Ctrl Pts',(7.07057502871922,-100.220483118095,-4.08219839617346));
#22882=CARTESIAN_POINT('Ctrl Pts',(4.71371668580301,-100.045483118095,-8.16439679232994));
#22883=CARTESIAN_POINT('Ctrl Pts',(-1.4702867290402E-11,-99.8704831180952,
-8.16439679232146));
#22884=CARTESIAN_POINT('Ctrl Pts',(-4.71371668583241,-99.6954831180952,
-8.16439679231297));
#22885=CARTESIAN_POINT('Ctrl Pts',(-7.07057502873392,-99.5204831180952,
-4.082198396148));
#22886=CARTESIAN_POINT('Ctrl Pts',(-9.42743337163542,-99.3454831180952,
1.69768315121407E-11));
#22887=CARTESIAN_POINT('Ctrl Pts',(-7.07057502871922,-99.1704831180952,
4.08219839617346));
#22888=CARTESIAN_POINT('Ctrl Pts',(-4.71371668580301,-98.9954831180952,
8.16439679232994));
#22889=CARTESIAN_POINT('Ctrl Pts',(1.47018674401621E-11,-98.8204831180952,
8.16439679232146));
#22890=CARTESIAN_POINT('Ctrl Pts',(4.71371668583241,-98.6454831180952,8.16439679231297));
#22891=CARTESIAN_POINT('Ctrl Pts',(7.07057502873392,-98.4704831180952,4.082198396148));
#22892=CARTESIAN_POINT('Ctrl Pts',(9.42743337163542,-98.2954831180952,-1.69756769845304E-11));
#22893=CARTESIAN_POINT('Ctrl Pts',(7.07057502871922,-98.1204831180952,-4.08219839617346));
#22894=CARTESIAN_POINT('Ctrl Pts',(4.71371668580301,-97.9454831180952,-8.16439679232994));
#22895=CARTESIAN_POINT('Ctrl Pts',(-1.4702867290402E-11,-97.7704831180952,
-8.16439679232146));
#22896=CARTESIAN_POINT('Ctrl Pts',(-4.71371668583241,-97.5954831180952,
-8.16439679231297));
#22897=CARTESIAN_POINT('Ctrl Pts',(-7.07057502873392,-97.4204831180952,
-4.082198396148));
#22898=CARTESIAN_POINT('Ctrl Pts',(-9.42743337163542,-97.2454831180952,
1.69768315121407E-11));
#22899=CARTESIAN_POINT('Ctrl Pts',(-7.07057502871922,-97.0704831180952,
4.08219839617346));
#22900=CARTESIAN_POINT('Ctrl Pts',(-4.71371668580301,-96.8954831180952,
8.16439679232994));
#22901=CARTESIAN_POINT('Ctrl Pts',(1.47018674401621E-11,-96.7204831180952,
8.16439679232146));
#22902=CARTESIAN_POINT('Ctrl Pts',(4.71371668583241,-96.5454831180952,8.16439679231297));
#22903=CARTESIAN_POINT('Ctrl Pts',(7.07057502873392,-96.3704831180952,4.082198396148));
#22904=CARTESIAN_POINT('Ctrl Pts',(9.42743337163542,-96.1954831180952,-1.69756769845304E-11));
#22905=CARTESIAN_POINT('Ctrl Pts',(7.07057502871922,-96.0204831180952,-4.08219839617346));
#22906=CARTESIAN_POINT('Ctrl Pts',(4.71371668580301,-95.8454831180952,-8.16439679232994));
#22907=CARTESIAN_POINT('Ctrl Pts',(-1.4702867290402E-11,-95.6704831180952,
-8.16439679232146));
#22908=CARTESIAN_POINT('Ctrl Pts',(-4.71371668583241,-95.4954831180952,
-8.16439679231297));
#22909=CARTESIAN_POINT('Ctrl Pts',(-7.07057502873392,-95.3204831180952,
-4.082198396148));
#22910=CARTESIAN_POINT('Ctrl Pts',(-9.42743337163542,-95.1454831180952,
1.69768315121407E-11));
#22911=CARTESIAN_POINT('Ctrl Pts',(-7.07057502871922,-94.9704831180952,
4.08219839617346));
#22912=CARTESIAN_POINT('Ctrl Pts',(-4.71371668580301,-94.7954831180952,
8.16439679232994));
#22913=CARTESIAN_POINT('Ctrl Pts',(1.47018674401621E-11,-94.6204831180952,
8.16439679232146));
#22914=CARTESIAN_POINT('Ctrl Pts',(4.71371668583241,-94.4454831180952,8.16439679231297));
#22915=CARTESIAN_POINT('Ctrl Pts',(7.07057502873392,-94.2704831180952,4.082198396148));
#22916=CARTESIAN_POINT('Ctrl Pts',(9.42743337163542,-94.0954831180952,-1.69756769845304E-11));
#22917=CARTESIAN_POINT('Ctrl Pts',(7.07057502871922,-93.9204831180952,-4.08219839617346));
#22918=CARTESIAN_POINT('Ctrl Pts',(4.71371668580301,-93.7454831180952,-8.16439679232994));
#22919=CARTESIAN_POINT('Ctrl Pts',(-1.4702867290402E-11,-93.5704831180952,
-8.16439679232146));
#22920=CARTESIAN_POINT('Ctrl Pts',(-4.71371668583241,-93.3954831180952,
-8.16439679231297));
#22921=CARTESIAN_POINT('Ctrl Pts',(-7.07057502873392,-93.2204831180952,
-4.082198396148));
#22922=CARTESIAN_POINT('Ctrl Pts',(-9.42743337163542,-93.0454831180952,
1.69768315121407E-11));
#22923=CARTESIAN_POINT('Ctrl Pts',(-7.07057502871922,-92.8704831180952,
4.08219839617346));
#22924=CARTESIAN_POINT('Ctrl Pts',(-4.71371668580301,-92.6954831180952,
8.16439679232994));
#22925=CARTESIAN_POINT('Ctrl Pts',(1.47018674401621E-11,-92.5204831180952,
8.16439679232146));
#22926=CARTESIAN_POINT('Ctrl Pts',(4.71371668583241,-92.3454831180952,8.16439679231297));
#22927=CARTESIAN_POINT('Ctrl Pts',(7.07057502873392,-92.1704831180952,4.082198396148));
#22928=CARTESIAN_POINT('Ctrl Pts',(9.42743337163542,-91.9954831180952,-1.69756769845304E-11));
#22929=CARTESIAN_POINT('Ctrl Pts',(7.07057502871922,-91.8204831180952,-4.08219839617346));
#22930=CARTESIAN_POINT('Ctrl Pts',(4.71371668580301,-91.6454831180952,-8.16439679232994));
#22931=CARTESIAN_POINT('Ctrl Pts',(-1.4702867290402E-11,-91.4704831180952,
-8.16439679232146));
#22932=CARTESIAN_POINT('Ctrl Pts',(-4.71371668583241,-91.2954831180952,
-8.16439679231297));
#22933=CARTESIAN_POINT('Ctrl Pts',(-7.07057502873392,-91.1204831180952,
-4.082198396148));
#22934=CARTESIAN_POINT('Ctrl Pts',(-9.42743337163542,-90.9454831180952,
1.69768315121407E-11));
#22935=CARTESIAN_POINT('Ctrl Pts',(-7.07057502871922,-90.7704831180952,
4.08219839617346));
#22936=CARTESIAN_POINT('Ctrl Pts',(-4.71371668580301,-90.5954831180952,
8.16439679232994));
#22937=CARTESIAN_POINT('Ctrl Pts',(1.47018674401621E-11,-90.4204831180952,
8.16439679232146));
#22938=CARTESIAN_POINT('Ctrl Pts',(4.71371668583241,-90.2454831180952,8.16439679231297));
#22939=CARTESIAN_POINT('Ctrl Pts',(7.07057502873392,-90.0704831180952,4.082198396148));
#22940=CARTESIAN_POINT('Ctrl Pts',(9.42743337163542,-89.8954831180952,-1.69756769845304E-11));
#22941=CARTESIAN_POINT('Ctrl Pts',(7.07057502871922,-89.7204831180952,-4.08219839617346));
#22942=CARTESIAN_POINT('Ctrl Pts',(4.71371668580301,-89.5454831180952,-8.16439679232994));
#22943=CARTESIAN_POINT('Ctrl Pts',(-1.4702867290402E-11,-89.3704831180952,
-8.16439679232146));
#22944=CARTESIAN_POINT('Ctrl Pts',(-4.71371668583241,-89.1954831180952,
-8.16439679231297));
#22945=CARTESIAN_POINT('Ctrl Pts',(-7.07057502873392,-89.0204831180952,
-4.082198396148));
#22946=CARTESIAN_POINT('Ctrl Pts',(-9.42743337163542,-88.8454831180952,
1.69768315121407E-11));
#22947=CARTESIAN_POINT('Ctrl Pts',(-7.07057502871922,-88.6704831180952,
4.08219839617346));
#22948=CARTESIAN_POINT('Ctrl Pts',(-4.71371668580301,-88.4954831180952,
8.16439679232994));
#22949=CARTESIAN_POINT('Ctrl Pts',(1.47018674401621E-11,-88.3204831180952,
8.16439679232146));
#22950=CARTESIAN_POINT('Ctrl Pts',(4.71371668583241,-88.1454831180952,8.16439679231297));
#22951=CARTESIAN_POINT('Ctrl Pts',(7.07057502873392,-87.9704831180952,4.082198396148));
#22952=CARTESIAN_POINT('Ctrl Pts',(9.42743337163542,-87.7954831180952,-1.69756769845304E-11));
#22953=CARTESIAN_POINT('Ctrl Pts',(7.07057502871922,-87.6204831180952,-4.08219839617346));
#22954=CARTESIAN_POINT('Ctrl Pts',(4.71371668580301,-87.4454831180952,-8.16439679232994));
#22955=CARTESIAN_POINT('Ctrl Pts',(-1.4702867290402E-11,-87.2704831180952,
-8.16439679232146));
#22956=CARTESIAN_POINT('Ctrl Pts',(-4.71371668583241,-87.0954831180952,
-8.16439679231297));
#22957=CARTESIAN_POINT('Ctrl Pts',(-7.07057502873392,-86.9204831180952,
-4.082198396148));
#22958=CARTESIAN_POINT('Ctrl Pts',(-9.42743337163542,-86.7454831180952,
1.69768315121407E-11));
#22959=CARTESIAN_POINT('Ctrl Pts',(-7.07057502871922,-86.5704831180952,
4.08219839617346));
#22960=CARTESIAN_POINT('Ctrl Pts',(-4.71371668580301,-86.3954831180952,
8.16439679232994));
#22961=CARTESIAN_POINT('Ctrl Pts',(1.47018674401621E-11,-86.2204831180952,
8.16439679232146));
#22962=CARTESIAN_POINT('Ctrl Pts',(4.71371668583241,-86.0454831180952,8.16439679231297));
#22963=CARTESIAN_POINT('Ctrl Pts',(7.07057502873392,-85.8704831180952,4.082198396148));
#22964=CARTESIAN_POINT('Ctrl Pts',(9.42743337163542,-85.6954831180952,-1.69756769845304E-11));
#22965=CARTESIAN_POINT('Ctrl Pts',(7.07057502871922,-85.5204831180952,-4.08219839617346));
#22966=CARTESIAN_POINT('Ctrl Pts',(4.71371668580301,-85.3454831180952,-8.16439679232994));
#22967=CARTESIAN_POINT('Ctrl Pts',(-1.4702867290402E-11,-85.1704831180952,
-8.16439679232146));
#22968=CARTESIAN_POINT('Ctrl Pts',(-4.71371668583241,-84.9954831180952,
-8.16439679231297));
#22969=CARTESIAN_POINT('Ctrl Pts',(-7.07057502873392,-84.8204831180952,
-4.082198396148));
#22970=CARTESIAN_POINT('Ctrl Pts',(-9.42743337163542,-84.6454831180952,
1.69768315121407E-11));
#22971=CARTESIAN_POINT('Ctrl Pts',(-7.07057502871922,-84.4704831180952,
4.08219839617346));
#22972=CARTESIAN_POINT('Ctrl Pts',(-4.71371668580301,-84.2954831180952,
8.16439679232994));
#22973=CARTESIAN_POINT('Ctrl Pts',(1.47018674401621E-11,-84.1204831180952,
8.16439679232146));
#22974=CARTESIAN_POINT('Ctrl Pts',(4.71371668583241,-83.9454831180952,8.16439679231297));
#22975=CARTESIAN_POINT('Ctrl Pts',(7.07057502873392,-83.7704831180952,4.082198396148));
#22976=CARTESIAN_POINT('Ctrl Pts',(9.42743337163542,-83.5954831180952,-1.69756769845304E-11));
#22977=CARTESIAN_POINT('Ctrl Pts',(7.07057502871922,-83.4204831180952,-4.08219839617346));
#22978=CARTESIAN_POINT('Ctrl Pts',(4.71371668580301,-83.2454831180952,-8.16439679232994));
#22979=CARTESIAN_POINT('Ctrl Pts',(-1.4702867290402E-11,-83.0704831180952,
-8.16439679232146));
#22980=CARTESIAN_POINT('Ctrl Pts',(-4.71371668583241,-82.8954831180952,
-8.16439679231297));
#22981=CARTESIAN_POINT('Ctrl Pts',(-7.07057502873392,-82.7204831180952,
-4.082198396148));
#22982=CARTESIAN_POINT('Ctrl Pts',(-9.42743337163542,-82.5454831180952,
1.69768315121407E-11));
#22983=CARTESIAN_POINT('Ctrl Pts',(-7.07057502871922,-82.3704831180952,
4.08219839617346));
#22984=CARTESIAN_POINT('Ctrl Pts',(-4.71371668580301,-82.1954831180952,
8.16439679232994));
#22985=CARTESIAN_POINT('Ctrl Pts',(1.47018674401621E-11,-82.0204831180952,
8.16439679232146));
#22986=CARTESIAN_POINT('Ctrl Pts',(4.71371668583241,-81.8454831180952,8.16439679231297));
#22987=CARTESIAN_POINT('Ctrl Pts',(7.07057502873392,-81.6704831180952,4.082198396148));
#22988=CARTESIAN_POINT('Ctrl Pts',(9.42743337163542,-81.4954831180952,-1.69756769845304E-11));
#22989=CARTESIAN_POINT('Ctrl Pts',(7.07057502871922,-81.3204831180952,-4.08219839617346));
#22990=CARTESIAN_POINT('Ctrl Pts',(4.71371668580301,-81.1454831180953,-8.16439679232994));
#22991=CARTESIAN_POINT('Ctrl Pts',(-1.4702867290402E-11,-80.9704831180952,
-8.16439679232146));
#22992=CARTESIAN_POINT('Ctrl Pts',(-4.71371668583241,-80.7954831180952,
-8.16439679231297));
#22993=CARTESIAN_POINT('Ctrl Pts',(-7.07057502873392,-80.6204831180952,
-4.082198396148));
#22994=CARTESIAN_POINT('Ctrl Pts',(-9.42743337163542,-80.4454831180952,
1.69768315121407E-11));
#22995=CARTESIAN_POINT('Ctrl Pts',(-7.07057502871922,-80.2704831180952,
4.08219839617346));
#22996=CARTESIAN_POINT('Ctrl Pts',(-4.71371668580301,-80.0954831180952,
8.16439679232994));
#22997=CARTESIAN_POINT('Ctrl Pts',(1.47018674401621E-11,-79.9204831180952,
8.16439679232146));
#22998=CARTESIAN_POINT('Ctrl Pts',(4.71371668583241,-79.7454831180953,8.16439679231297));
#22999=CARTESIAN_POINT('Ctrl Pts',(7.07057502873392,-79.5704831180952,4.082198396148));
#23000=CARTESIAN_POINT('Ctrl Pts',(9.42743337163542,-79.3954831180952,-1.69756769845304E-11));
#23001=CARTESIAN_POINT('Ctrl Pts',(7.07057502871922,-79.2204831180952,-4.08219839617346));
#23002=CARTESIAN_POINT('Ctrl Pts',(4.71371668580301,-79.0454831180952,-8.16439679232994));
#23003=CARTESIAN_POINT('Ctrl Pts',(-1.4702867290402E-11,-78.8704831180952,
-8.16439679232146));
#23004=CARTESIAN_POINT('Ctrl Pts',(-4.71371668583241,-78.6954831180953,
-8.16439679231297));
#23005=CARTESIAN_POINT('Ctrl Pts',(-7.07057502873392,-78.5204831180952,
-4.082198396148));
#23006=CARTESIAN_POINT('Ctrl Pts',(-9.42743337163542,-78.3454831180952,
1.69768315121407E-11));
#23007=CARTESIAN_POINT('Ctrl Pts',(-7.07057502871922,-78.1704831180953,
4.08219839617346));
#23008=CARTESIAN_POINT('Ctrl Pts',(-4.71371668580301,-77.9954831180953,
8.16439679232994));
#23009=CARTESIAN_POINT('Ctrl Pts',(1.47018674401621E-11,-77.8204831180952,
8.16439679232146));
#23010=CARTESIAN_POINT('Ctrl Pts',(4.71371668583241,-77.6454831180953,8.16439679231297));
#23011=CARTESIAN_POINT('Ctrl Pts',(7.07057502873392,-77.4704831180952,4.082198396148));
#23012=CARTESIAN_POINT('Ctrl Pts',(9.42743337163542,-77.2954831180952,-1.69756769845304E-11));
#23013=CARTESIAN_POINT('Ctrl Pts',(7.07057502871922,-77.1204831180952,-4.08219839617346));
#23014=CARTESIAN_POINT('Ctrl Pts',(4.71371668580301,-76.9454831180952,-8.16439679232994));
#23015=CARTESIAN_POINT('Ctrl Pts',(-1.4702867290402E-11,-76.7704831180952,
-8.16439679232146));
#23016=CARTESIAN_POINT('Ctrl Pts',(-4.71371668583241,-76.5954831180953,
-8.16439679231297));
#23017=CARTESIAN_POINT('Ctrl Pts',(-7.07057502873392,-76.4204831180952,
-4.082198396148));
#23018=CARTESIAN_POINT('Ctrl Pts',(-9.42743337163542,-76.2454831180952,
1.69768315121407E-11));
#23019=CARTESIAN_POINT('Ctrl Pts',(-7.07057502871922,-76.0704831180952,
4.08219839617346));
#23020=CARTESIAN_POINT('Ctrl Pts',(-4.71371668580301,-75.8954831180952,
8.16439679232994));
#23021=CARTESIAN_POINT('Ctrl Pts',(1.47018674401621E-11,-75.7204831180952,
8.16439679232146));
#23022=CARTESIAN_POINT('Ctrl Pts',(4.71371668583241,-75.5454831180952,8.16439679231297));
#23023=CARTESIAN_POINT('Ctrl Pts',(7.07057502873392,-75.3704831180952,4.082198396148));
#23024=CARTESIAN_POINT('Ctrl Pts',(9.42743337163542,-75.1954831180952,-1.69756769845304E-11));
#23025=CARTESIAN_POINT('Ctrl Pts',(7.07057502871922,-75.0204831180952,-4.08219839617346));
#23026=CARTESIAN_POINT('Ctrl Pts',(4.71371668580301,-74.8454831180952,-8.16439679232994));
#23027=CARTESIAN_POINT('Ctrl Pts',(-1.4702867290402E-11,-74.6704831180952,
-8.16439679232146));
#23028=CARTESIAN_POINT('Ctrl Pts',(-4.71371668583241,-74.4954831180953,
-8.16439679231297));
#23029=CARTESIAN_POINT('Ctrl Pts',(-7.07057502873392,-74.3204831180952,
-4.082198396148));
#23030=CARTESIAN_POINT('Ctrl Pts',(-9.42743337163542,-74.1454831180952,
1.69768315121407E-11));
#23031=CARTESIAN_POINT('Ctrl Pts',(-7.07057502871922,-73.9704831180952,
4.08219839617346));
#23032=CARTESIAN_POINT('Ctrl Pts',(-4.71371668580301,-73.7954831180952,
8.16439679232994));
#23033=CARTESIAN_POINT('Ctrl Pts',(1.47018674401621E-11,-73.6204831180952,
8.16439679232146));
#23034=CARTESIAN_POINT('Ctrl Pts',(4.71371668583241,-73.4454831180953,8.16439679231297));
#23035=CARTESIAN_POINT('Ctrl Pts',(7.07057502873392,-73.2704831180952,4.082198396148));
#23036=CARTESIAN_POINT('Ctrl Pts',(9.42743337163542,-73.0954831180953,-1.69756769845304E-11));
#23037=CARTESIAN_POINT('Ctrl Pts',(7.07057502871922,-72.9204831180952,-4.08219839617346));
#23038=CARTESIAN_POINT('Ctrl Pts',(4.71371668580301,-72.7454831180952,-8.16439679232994));
#23039=CARTESIAN_POINT('Ctrl Pts',(-1.4702867290402E-11,-72.5704831180953,
-8.16439679232146));
#23040=CARTESIAN_POINT('Ctrl Pts',(-4.71371668583241,-72.3954831180953,
-8.16439679231297));
#23041=CARTESIAN_POINT('Ctrl Pts',(-7.07057502873392,-72.2204831180952,
-4.082198396148));
#23042=CARTESIAN_POINT('Ctrl Pts',(-9.42743337163542,-72.0454831180953,
1.69768315121407E-11));
#23043=CARTESIAN_POINT('Ctrl Pts',(-7.07057502871922,-71.8704831180952,
4.08219839617346));
#23044=CARTESIAN_POINT('Ctrl Pts',(-4.71371668580301,-71.6954831180952,
8.16439679232994));
#23045=CARTESIAN_POINT('Ctrl Pts',(1.47018674401621E-11,-71.5204831180953,
8.16439679232146));
#23046=CARTESIAN_POINT('Ctrl Pts',(4.71371668583241,-71.3454831180952,8.16439679231297));
#23047=CARTESIAN_POINT('Ctrl Pts',(7.07057502873392,-71.1704831180952,4.082198396148));
#23048=CARTESIAN_POINT('Ctrl Pts',(9.42743337163542,-70.9954831180953,-1.69756769845304E-11));
#23049=CARTESIAN_POINT('Ctrl Pts',(7.07057502871922,-70.8204831180952,-4.08219839617346));
#23050=CARTESIAN_POINT('Ctrl Pts',(4.71371668580301,-70.6454831180952,-8.16439679232994));
#23051=CARTESIAN_POINT('Ctrl Pts',(-1.4702867290402E-11,-70.4704831180953,
-8.16439679232146));
#23052=CARTESIAN_POINT('Ctrl Pts',(-4.71371668583241,-70.2954831180952,
-8.16439679231297));
#23053=CARTESIAN_POINT('Ctrl Pts',(-7.07057502873392,-70.1204831180952,
-4.082198396148));
#23054=CARTESIAN_POINT('Ctrl Pts',(-9.42743337163542,-69.9454831180953,
1.69768315121407E-11));
#23055=CARTESIAN_POINT('Ctrl Pts',(-7.07057502871922,-69.7704831180953,
4.08219839617346));
#23056=CARTESIAN_POINT('Ctrl Pts',(-4.71371668580301,-69.5954831180952,
8.16439679232994));
#23057=CARTESIAN_POINT('Ctrl Pts',(1.47018674401621E-11,-69.4204831180953,
8.16439679232146));
#23058=CARTESIAN_POINT('Ctrl Pts',(4.71371668583241,-69.2454831180953,8.16439679231297));
#23059=CARTESIAN_POINT('Ctrl Pts',(7.07057502873392,-69.0704831180953,4.082198396148));
#23060=CARTESIAN_POINT('Ctrl Pts',(9.42743337163542,-68.8954831180953,-1.69756769845304E-11));
#23061=CARTESIAN_POINT('Ctrl Pts',(7.07057502871922,-68.7204831180952,-4.08219839617346));
#23062=CARTESIAN_POINT('Ctrl Pts',(4.71371668580301,-68.5454831180952,-8.16439679232994));
#23063=CARTESIAN_POINT('Ctrl Pts',(-1.4702867290402E-11,-68.3704831180953,
-8.16439679232146));
#23064=CARTESIAN_POINT('Ctrl Pts',(-4.71371668583241,-68.1954831180952,
-8.16439679231297));
#23065=CARTESIAN_POINT('Ctrl Pts',(-7.07057502873392,-68.0204831180953,
-4.082198396148));
#23066=CARTESIAN_POINT('Ctrl Pts',(-9.42743337163542,-67.8454831180953,
1.69768315121407E-11));
#23067=CARTESIAN_POINT('Ctrl Pts',(-7.07057502871922,-67.6704831180952,
4.08219839617346));
#23068=CARTESIAN_POINT('Ctrl Pts',(-4.71371668580301,-67.4954831180953,
8.16439679232994));
#23069=CARTESIAN_POINT('Ctrl Pts',(1.47018674401621E-11,-67.3204831180953,
8.16439679232146));
#23070=CARTESIAN_POINT('Ctrl Pts',(4.71371668583241,-67.1454831180952,8.16439679231297));
#23071=CARTESIAN_POINT('Ctrl Pts',(7.07057502873392,-66.9704831180952,4.082198396148));
#23072=CARTESIAN_POINT('Ctrl Pts',(9.42743337163542,-66.7954831180953,-1.69756769845304E-11));
#23073=CARTESIAN_POINT('Ctrl Pts',(7.07057502871922,-66.6204831180952,-4.08219839617346));
#23074=CARTESIAN_POINT('Ctrl Pts',(4.71371668580301,-66.4454831180952,-8.16439679232994));
#23075=CARTESIAN_POINT('Ctrl Pts',(-1.4702867290402E-11,-66.2704831180953,
-8.16439679232146));
#23076=CARTESIAN_POINT('Ctrl Pts',(-4.71371668583241,-66.0954831180952,
-8.16439679231297));
#23077=CARTESIAN_POINT('Ctrl Pts',(-7.07057502873392,-65.9204831180952,
-4.082198396148));
#23078=CARTESIAN_POINT('Ctrl Pts',(-9.42743337163542,-65.7454831180953,
1.69768315121407E-11));
#23079=CARTESIAN_POINT('Ctrl Pts',(-7.07057502871922,-65.5704831180953,
4.08219839617346));
#23080=CARTESIAN_POINT('Ctrl Pts',(-4.71371668580301,-65.3954831180953,
8.16439679232994));
#23081=CARTESIAN_POINT('Ctrl Pts',(1.47018674401621E-11,-65.2204831180952,
8.16439679232146));
#23082=CARTESIAN_POINT('Ctrl Pts',(4.71371668583241,-65.0454831180952,8.16439679231297));
#23083=CARTESIAN_POINT('Ctrl Pts',(7.07057502873392,-64.8704831180953,4.082198396148));
#23084=CARTESIAN_POINT('Ctrl Pts',(9.42743337163542,-64.6954831180953,-1.69756769845304E-11));
#23085=CARTESIAN_POINT('Ctrl Pts',(7.07057502871922,-64.5204831180953,-4.08219839617346));
#23086=CARTESIAN_POINT('Ctrl Pts',(4.71371668580301,-64.3454831180953,-8.16439679232994));
#23087=CARTESIAN_POINT('Ctrl Pts',(-1.4702867290402E-11,-64.1704831180952,
-8.16439679232146));
#23088=CARTESIAN_POINT('Ctrl Pts',(-4.71371668583241,-63.9954831180953,
-8.16439679231297));
#23089=CARTESIAN_POINT('Ctrl Pts',(-7.07057502873392,-63.8204831180953,
-4.082198396148));
#23090=CARTESIAN_POINT('Ctrl Pts',(-9.42743337163542,-63.6454831180953,
1.69768315121407E-11));
#23091=CARTESIAN_POINT('Ctrl Pts',(-7.07057502871922,-63.4704831180953,
4.08219839617346));
#23092=CARTESIAN_POINT('Ctrl Pts',(-4.71371668580301,-63.2954831180953,
8.16439679232994));
#23093=CARTESIAN_POINT('Ctrl Pts',(1.47018674401621E-11,-63.1204831180953,
8.16439679232146));
#23094=CARTESIAN_POINT('Ctrl Pts',(4.71371668583241,-62.9454831180952,8.16439679231297));
#23095=CARTESIAN_POINT('Ctrl Pts',(7.07057502873392,-62.7704831180953,4.082198396148));
#23096=CARTESIAN_POINT('Ctrl Pts',(9.42743337163542,-62.5954831180953,-1.69756769845304E-11));
#23097=CARTESIAN_POINT('Ctrl Pts',(7.07057502871922,-62.4204831180953,-4.08219839617346));
#23098=CARTESIAN_POINT('Ctrl Pts',(4.71371668580301,-62.2454831180953,-8.16439679232994));
#23099=CARTESIAN_POINT('Ctrl Pts',(-1.4702867290402E-11,-62.0704831180953,
-8.16439679232146));
#23100=CARTESIAN_POINT('Ctrl Pts',(-4.71371668583241,-61.8954831180952,
-8.16439679231297));
#23101=CARTESIAN_POINT('Ctrl Pts',(-7.07057502873392,-61.7204831180953,
-4.082198396148));
#23102=CARTESIAN_POINT('Ctrl Pts',(-9.42743337163542,-61.5454831180953,
1.69768315121407E-11));
#23103=CARTESIAN_POINT('Ctrl Pts',(-7.07057502871922,-61.3704831180953,
4.08219839617346));
#23104=CARTESIAN_POINT('Ctrl Pts',(-4.71371668580301,-61.1954831180953,
8.16439679232994));
#23105=CARTESIAN_POINT('Ctrl Pts',(1.47018674401621E-11,-61.0204831180953,
8.16439679232146));
#23106=CARTESIAN_POINT('Ctrl Pts',(4.71371668583241,-60.8454831180953,8.16439679231297));
#23107=CARTESIAN_POINT('Ctrl Pts',(7.07057502873392,-60.6704831180953,4.082198396148));
#23108=CARTESIAN_POINT('Ctrl Pts',(9.42743337163542,-60.4954831180953,-1.69756769845304E-11));
#23109=CARTESIAN_POINT('Ctrl Pts',(7.07057502871922,-60.3204831180953,-4.08219839617346));
#23110=CARTESIAN_POINT('Ctrl Pts',(4.71371668580301,-60.1454831180953,-8.16439679232994));
#23111=CARTESIAN_POINT('Ctrl Pts',(-1.4702867290402E-11,-59.9704831180953,
-8.16439679232146));
#23112=CARTESIAN_POINT('Ctrl Pts',(-4.71371668583241,-59.7954831180953,
-8.16439679231297));
#23113=CARTESIAN_POINT('Ctrl Pts',(-7.07057502873392,-59.6204831180953,
-4.082198396148));
#23114=CARTESIAN_POINT('Ctrl Pts',(-9.42743337163542,-59.4454831180953,
1.69768315121407E-11));
#23115=CARTESIAN_POINT('Ctrl Pts',(-7.07057502871922,-59.2704831180953,
4.08219839617346));
#23116=CARTESIAN_POINT('Ctrl Pts',(-4.71371668580301,-59.0954831180953,
8.16439679232994));
#23117=CARTESIAN_POINT('Ctrl Pts',(1.47018674401621E-11,-58.9204831180953,
8.16439679232146));
#23118=CARTESIAN_POINT('Ctrl Pts',(4.71371668583241,-58.7454831180953,8.16439679231297));
#23119=CARTESIAN_POINT('Ctrl Pts',(7.07057502873392,-58.5704831180953,4.082198396148));
#23120=CARTESIAN_POINT('Ctrl Pts',(9.42743337163542,-58.3954831180953,-1.69756769845304E-11));
#23121=CARTESIAN_POINT('Ctrl Pts',(7.07057502871922,-58.2204831180953,-4.08219839617346));
#23122=CARTESIAN_POINT('Ctrl Pts',(4.71371668580301,-58.0454831180953,-8.16439679232994));
#23123=CARTESIAN_POINT('Ctrl Pts',(-1.4702867290402E-11,-57.8704831180952,
-8.16439679232146));
#23124=CARTESIAN_POINT('Ctrl Pts',(-4.71371668583241,-57.6954831180953,
-8.16439679231297));
#23125=CARTESIAN_POINT('Ctrl Pts',(-7.07057502873392,-57.5204831180953,
-4.082198396148));
#23126=CARTESIAN_POINT('Ctrl Pts',(-9.42743337163542,-57.3454831180953,
1.69768315121407E-11));
#23127=CARTESIAN_POINT('Ctrl Pts',(-7.07057502871922,-57.1704831180953,
4.08219839617346));
#23128=CARTESIAN_POINT('Ctrl Pts',(-4.71371668580301,-56.9954831180953,
8.16439679232994));
#23129=CARTESIAN_POINT('Ctrl Pts',(1.47018674401621E-11,-56.8204831180953,
8.16439679232146));
#23130=CARTESIAN_POINT('Ctrl Pts',(4.71371668583241,-56.6454831180953,8.16439679231297));
#23131=CARTESIAN_POINT('Ctrl Pts',(7.07057502873392,-56.4704831180953,4.082198396148));
#23132=CARTESIAN_POINT('Ctrl Pts',(9.42743337163542,-56.2954831180953,-1.69756769845304E-11));
#23133=CARTESIAN_POINT('Ctrl Pts',(7.07057502871922,-56.1204831180953,-4.08219839617346));
#23134=CARTESIAN_POINT('Ctrl Pts',(4.71371668580301,-55.9454831180953,-8.16439679232994));
#23135=CARTESIAN_POINT('Ctrl Pts',(-1.4702867290402E-11,-55.7704831180953,
-8.16439679232146));
#23136=CARTESIAN_POINT('Ctrl Pts',(-4.71371668583241,-55.5954831180953,
-8.16439679231297));
#23137=CARTESIAN_POINT('Ctrl Pts',(-7.07057502873392,-55.4204831180953,
-4.082198396148));
#23138=CARTESIAN_POINT('Ctrl Pts',(-9.42743337163542,-55.2454831180953,
1.69768315121407E-11));
#23139=CARTESIAN_POINT('Ctrl Pts',(-7.07057502871922,-55.0704831180953,
4.08219839617346));
#23140=CARTESIAN_POINT('Ctrl Pts',(-4.71371668580301,-54.8954831180953,
8.16439679232994));
#23141=CARTESIAN_POINT('Ctrl Pts',(1.47018674401621E-11,-54.7204831180953,
8.16439679232146));
#23142=CARTESIAN_POINT('Ctrl Pts',(4.71371668583241,-54.5454831180953,8.16439679231297));
#23143=CARTESIAN_POINT('Ctrl Pts',(7.07057502873392,-54.3704831180953,4.082198396148));
#23144=CARTESIAN_POINT('Ctrl Pts',(9.42743337163542,-54.1954831180953,-1.69756769845304E-11));
#23145=CARTESIAN_POINT('Ctrl Pts',(7.07057502871922,-54.0204831180953,-4.08219839617346));
#23146=CARTESIAN_POINT('Ctrl Pts',(4.71371668580301,-53.8454831180953,-8.16439679232994));
#23147=CARTESIAN_POINT('Ctrl Pts',(-1.4702867290402E-11,-53.6704831180953,
-8.16439679232146));
#23148=CARTESIAN_POINT('Ctrl Pts',(-4.71371668583241,-53.4954831180953,
-8.16439679231297));
#23149=CARTESIAN_POINT('Ctrl Pts',(-7.07057502873392,-53.3204831180953,
-4.082198396148));
#23150=CARTESIAN_POINT('Ctrl Pts',(-9.42743337163542,-53.1454831180953,
1.69768315121407E-11));
#23151=CARTESIAN_POINT('Ctrl Pts',(-7.07057502871922,-52.9704831180953,
4.08219839617346));
#23152=CARTESIAN_POINT('Ctrl Pts',(-4.71371668580301,-52.7954831180953,
8.16439679232994));
#23153=CARTESIAN_POINT('Ctrl Pts',(1.47018674401621E-11,-52.6204831180953,
8.16439679232146));
#23154=CARTESIAN_POINT('Ctrl Pts',(4.71371668583241,-52.4454831180953,8.16439679231297));
#23155=CARTESIAN_POINT('Ctrl Pts',(7.07057502873392,-52.2704831180953,4.082198396148));
#23156=CARTESIAN_POINT('Ctrl Pts',(9.42743337163542,-52.0954831180953,-1.69756769845304E-11));
#23157=CARTESIAN_POINT('Ctrl Pts',(7.07057502871922,-51.9204831180953,-4.08219839617346));
#23158=CARTESIAN_POINT('Ctrl Pts',(4.71371668580301,-51.7454831180953,-8.16439679232994));
#23159=CARTESIAN_POINT('Ctrl Pts',(-1.4702867290402E-11,-51.5704831180953,
-8.16439679232146));
#23160=CARTESIAN_POINT('Ctrl Pts',(-4.71371668583241,-51.3954831180953,
-8.16439679231297));
#23161=CARTESIAN_POINT('Ctrl Pts',(-7.07057502873392,-51.2204831180953,
-4.082198396148));
#23162=CARTESIAN_POINT('Ctrl Pts',(-9.42743337163542,-51.0454831180953,
1.69768315121407E-11));
#23163=CARTESIAN_POINT('Ctrl Pts',(-7.07057502871922,-50.8704831180953,
4.08219839617346));
#23164=CARTESIAN_POINT('Ctrl Pts',(-4.71371668580301,-50.6954831180953,
8.16439679232994));
#23165=CARTESIAN_POINT('Ctrl Pts',(1.47018674401621E-11,-50.5204831180953,
8.16439679232146));
#23166=CARTESIAN_POINT('Ctrl Pts',(4.71371668583241,-50.3454831180953,8.16439679231297));
#23167=CARTESIAN_POINT('Ctrl Pts',(7.07057502873392,-50.1704831180953,4.082198396148));
#23168=CARTESIAN_POINT('Ctrl Pts',(9.42743337163542,-49.9954831180953,-1.69756769845304E-11));
#23169=CARTESIAN_POINT('Ctrl Pts',(7.07057502871922,-49.8204831180953,-4.08219839617346));
#23170=CARTESIAN_POINT('Ctrl Pts',(4.71371668580301,-49.6454831180953,-8.16439679232994));
#23171=CARTESIAN_POINT('Ctrl Pts',(-1.4702867290402E-11,-49.4704831180953,
-8.16439679232146));
#23172=CARTESIAN_POINT('Ctrl Pts',(-4.71371668583241,-49.2954831180953,
-8.16439679231297));
#23173=CARTESIAN_POINT('Ctrl Pts',(-7.07057502873392,-49.1204831180953,
-4.082198396148));
#23174=CARTESIAN_POINT('Ctrl Pts',(-9.42743337163542,-48.9454831180953,
1.69768315121407E-11));
#23175=CARTESIAN_POINT('Ctrl Pts',(-7.07057502871922,-48.7704831180953,
4.08219839617346));
#23176=CARTESIAN_POINT('Ctrl Pts',(-4.71371668580301,-48.5954831180953,
8.16439679232994));
#23177=CARTESIAN_POINT('Ctrl Pts',(1.47018674401621E-11,-48.4204831180953,
8.16439679232146));
#23178=CARTESIAN_POINT('Ctrl Pts',(4.71371668583241,-48.2454831180953,8.16439679231297));
#23179=CARTESIAN_POINT('Ctrl Pts',(7.07057502873392,-48.0704831180953,4.082198396148));
#23180=CARTESIAN_POINT('Ctrl Pts',(9.42743337163542,-47.8954831180953,-1.69756769845304E-11));
#23181=CARTESIAN_POINT('Ctrl Pts',(7.07057502871922,-47.7204831180953,-4.08219839617346));
#23182=CARTESIAN_POINT('Ctrl Pts',(4.71371668580301,-47.5454831180953,-8.16439679232994));
#23183=CARTESIAN_POINT('Ctrl Pts',(-1.4702867290402E-11,-47.3704831180953,
-8.16439679232146));
#23184=CARTESIAN_POINT('Ctrl Pts',(-4.71371668583241,-47.1954831180953,
-8.16439679231297));
#23185=CARTESIAN_POINT('Ctrl Pts',(-7.07057502873392,-47.0204831180953,
-4.082198396148));
#23186=CARTESIAN_POINT('Ctrl Pts',(-9.42743337163542,-46.8454831180953,
1.69768315121407E-11));
#23187=CARTESIAN_POINT('Ctrl Pts',(-7.07057502871922,-46.6704831180953,
4.08219839617346));
#23188=CARTESIAN_POINT('Ctrl Pts',(-4.71371668580301,-46.4954831180953,
8.16439679232994));
#23189=CARTESIAN_POINT('Ctrl Pts',(1.47018674401621E-11,-46.3204831180953,
8.16439679232146));
#23190=CARTESIAN_POINT('Ctrl Pts',(4.71371668583241,-46.1454831180953,8.16439679231297));
#23191=CARTESIAN_POINT('Ctrl Pts',(7.07057502873392,-45.9704831180953,4.082198396148));
#23192=CARTESIAN_POINT('Ctrl Pts',(9.42743337163542,-45.7954831180953,-1.69756769845304E-11));
#23193=CARTESIAN_POINT('Ctrl Pts',(7.07057502871922,-45.6204831180953,-4.08219839617346));
#23194=CARTESIAN_POINT('Ctrl Pts',(4.71371668580301,-45.4454831180953,-8.16439679232994));
#23195=CARTESIAN_POINT('Ctrl Pts',(-1.4702867290402E-11,-45.2704831180953,
-8.16439679232146));
#23196=CARTESIAN_POINT('Ctrl Pts',(-4.71371668583241,-45.0954831180953,
-8.16439679231297));
#23197=CARTESIAN_POINT('Ctrl Pts',(-7.07057502873392,-44.9204831180953,
-4.082198396148));
#23198=CARTESIAN_POINT('Ctrl Pts',(-9.42743337163542,-44.7454831180953,
1.69768315121407E-11));
#23199=CARTESIAN_POINT('Ctrl Pts',(-7.07057502871922,-44.5704831180953,
4.08219839617346));
#23200=CARTESIAN_POINT('Ctrl Pts',(-4.71371668580301,-44.3954831180953,
8.16439679232994));
#23201=CARTESIAN_POINT('Ctrl Pts',(1.47018674401621E-11,-44.2204831180953,
8.16439679232146));
#23202=CARTESIAN_POINT('Ctrl Pts',(4.71371668583241,-44.0454831180953,8.16439679231297));
#23203=CARTESIAN_POINT('Ctrl Pts',(7.07057502873392,-43.8704831180953,4.082198396148));
#23204=CARTESIAN_POINT('Ctrl Pts',(9.42743337163542,-43.6954831180953,-1.69756769845304E-11));
#23205=CARTESIAN_POINT('Ctrl Pts',(7.07057502871922,-43.5204831180953,-4.08219839617346));
#23206=CARTESIAN_POINT('Ctrl Pts',(4.71371668580301,-43.3454831180953,-8.16439679232994));
#23207=CARTESIAN_POINT('Ctrl Pts',(-1.4702867290402E-11,-43.1704831180953,
-8.16439679232146));
#23208=CARTESIAN_POINT('Ctrl Pts',(-4.71371668583241,-42.9954831180953,
-8.16439679231297));
#23209=CARTESIAN_POINT('Ctrl Pts',(-7.07057502873392,-42.8204831180953,
-4.082198396148));
#23210=CARTESIAN_POINT('Ctrl Pts',(-9.42743337163542,-42.6454831180953,
1.69768315121407E-11));
#23211=CARTESIAN_POINT('Ctrl Pts',(-7.07057502871922,-42.4704831180953,
4.08219839617346));
#23212=CARTESIAN_POINT('Ctrl Pts',(-4.71371668580301,-42.2954831180953,
8.16439679232994));
#23213=CARTESIAN_POINT('Ctrl Pts',(1.47018674401621E-11,-42.1204831180953,
8.16439679232146));
#23214=CARTESIAN_POINT('Ctrl Pts',(4.71371668583241,-41.9454831180953,8.16439679231297));
#23215=CARTESIAN_POINT('Ctrl Pts',(7.07057502873392,-41.7704831180953,4.082198396148));
#23216=CARTESIAN_POINT('Ctrl Pts',(9.42743337163542,-41.5954831180953,-1.69756769845304E-11));
#23217=CARTESIAN_POINT('Ctrl Pts',(7.07057502871922,-41.4204831180953,-4.08219839617346));
#23218=CARTESIAN_POINT('Ctrl Pts',(4.71371668580301,-41.2454831180953,-8.16439679232994));
#23219=CARTESIAN_POINT('Ctrl Pts',(-1.4702867290402E-11,-41.0704831180953,
-8.16439679232146));
#23220=CARTESIAN_POINT('Ctrl Pts',(-4.71371668583241,-40.8954831180953,
-8.16439679231297));
#23221=CARTESIAN_POINT('Ctrl Pts',(-7.07057502873392,-40.7204831180953,
-4.082198396148));
#23222=CARTESIAN_POINT('Ctrl Pts',(-9.42743337163542,-40.5454831180953,
1.69768315121407E-11));
#23223=CARTESIAN_POINT('Ctrl Pts',(-7.07057502871922,-40.3704831180953,
4.08219839617346));
#23224=CARTESIAN_POINT('Ctrl Pts',(-4.71371668580301,-40.1954831180953,
8.16439679232994));
#23225=CARTESIAN_POINT('Ctrl Pts',(1.47018674401621E-11,-40.0204831180953,
8.16439679232146));
#23226=CARTESIAN_POINT('Ctrl Pts',(4.71371668583241,-39.8454831180953,8.16439679231297));
#23227=CARTESIAN_POINT('Ctrl Pts',(7.07057502873392,-39.6704831180953,4.082198396148));
#23228=CARTESIAN_POINT('Ctrl Pts',(9.42743337163542,-39.4954831180953,-1.69756769845304E-11));
#23229=CARTESIAN_POINT('Ctrl Pts',(7.07057502871922,-39.3204831180953,-4.08219839617346));
#23230=CARTESIAN_POINT('Ctrl Pts',(4.71371668580301,-39.1454831180953,-8.16439679232994));
#23231=CARTESIAN_POINT('Ctrl Pts',(-1.4702867290402E-11,-38.9704831180953,
-8.16439679232146));
#23232=CARTESIAN_POINT('Ctrl Pts',(-4.71371668583241,-38.7954831180953,
-8.16439679231297));
#23233=CARTESIAN_POINT('Ctrl Pts',(-7.07057502873392,-38.6204831180953,
-4.082198396148));
#23234=CARTESIAN_POINT('Ctrl Pts',(-9.42743337163542,-38.4454831180953,
1.69768315121407E-11));
#23235=CARTESIAN_POINT('Ctrl Pts',(-7.07057502871922,-38.2704831180953,
4.08219839617346));
#23236=CARTESIAN_POINT('Ctrl Pts',(-4.71371668580301,-38.0954831180953,
8.16439679232994));
#23237=CARTESIAN_POINT('Ctrl Pts',(1.47018674401621E-11,-37.9204831180953,
8.16439679232146));
#23238=CARTESIAN_POINT('Ctrl Pts',(4.71371668583241,-37.7454831180953,8.16439679231297));
#23239=CARTESIAN_POINT('Ctrl Pts',(7.07057502873392,-37.5704831180953,4.082198396148));
#23240=CARTESIAN_POINT('Ctrl Pts',(9.42743337163542,-37.3954831180953,-1.69756769845304E-11));
#23241=CARTESIAN_POINT('Ctrl Pts',(7.07057502871922,-37.2204831180953,-4.08219839617346));
#23242=CARTESIAN_POINT('Ctrl Pts',(4.71371668580301,-37.0454831180953,-8.16439679232994));
#23243=CARTESIAN_POINT('Ctrl Pts',(-1.4702867290402E-11,-36.8704831180953,
-8.16439679232146));
#23244=CARTESIAN_POINT('Ctrl Pts',(-4.71371668583241,-36.6954831180953,
-8.16439679231297));
#23245=CARTESIAN_POINT('Ctrl Pts',(-7.07057502873392,-36.5204831180953,
-4.082198396148));
#23246=CARTESIAN_POINT('Ctrl Pts',(-9.42743337163542,-36.3454831180953,
1.69768315121407E-11));
#23247=CARTESIAN_POINT('Ctrl Pts',(-7.07057502871922,-36.1704831180953,
4.08219839617346));
#23248=CARTESIAN_POINT('Ctrl Pts',(-4.71371668580301,-35.9954831180953,
8.16439679232994));
#23249=CARTESIAN_POINT('Ctrl Pts',(1.47018674401621E-11,-35.8204831180953,
8.16439679232146));
#23250=CARTESIAN_POINT('Ctrl Pts',(4.71371668583241,-35.6454831180953,8.16439679231297));
#23251=CARTESIAN_POINT('Ctrl Pts',(7.07057502873392,-35.4704831180953,4.082198396148));
#23252=CARTESIAN_POINT('Ctrl Pts',(9.42743337163542,-35.2954831180953,-1.69756769845304E-11));
#23253=CARTESIAN_POINT('Ctrl Pts',(7.07057502871922,-35.1204831180953,-4.08219839617346));
#23254=CARTESIAN_POINT('Ctrl Pts',(4.71371668580301,-34.9454831180953,-8.16439679232994));
#23255=CARTESIAN_POINT('Ctrl Pts',(-1.4702867290402E-11,-34.7704831180953,
-8.16439679232146));
#23256=CARTESIAN_POINT('Ctrl Pts',(-4.71371668583241,-34.5954831180953,
-8.16439679231297));
#23257=CARTESIAN_POINT('Ctrl Pts',(-7.07057502873392,-34.4204831180953,
-4.082198396148));
#23258=CARTESIAN_POINT('Ctrl Pts',(-9.42743337163542,-34.2454831180953,
1.69768315121407E-11));
#23259=CARTESIAN_POINT('Ctrl Pts',(-7.07057502871922,-34.0704831180953,
4.08219839617346));
#23260=CARTESIAN_POINT('Ctrl Pts',(-4.71371668580301,-33.8954831180953,
8.16439679232994));
#23261=CARTESIAN_POINT('Ctrl Pts',(1.47018674401621E-11,-33.7204831180953,
8.16439679232146));
#23262=CARTESIAN_POINT('Ctrl Pts',(4.71371668583241,-33.5454831180953,8.16439679231297));
#23263=CARTESIAN_POINT('Ctrl Pts',(7.07057502873392,-33.3704831180953,4.082198396148));
#23264=CARTESIAN_POINT('Ctrl Pts',(9.42743337163542,-33.1954831180953,-1.69756769845304E-11));
#23265=CARTESIAN_POINT('Ctrl Pts',(7.07057502871922,-33.0204831180953,-4.08219839617346));
#23266=CARTESIAN_POINT('Ctrl Pts',(4.71371668580301,-32.8454831180953,-8.16439679232994));
#23267=CARTESIAN_POINT('Ctrl Pts',(-1.4702867290402E-11,-32.6704831180953,
-8.16439679232146));
#23268=CARTESIAN_POINT('Ctrl Pts',(-4.71371668583241,-32.4954831180953,
-8.16439679231297));
#23269=CARTESIAN_POINT('Ctrl Pts',(-7.07057502873392,-32.3204831180953,
-4.082198396148));
#23270=CARTESIAN_POINT('Ctrl Pts',(-9.42743337163542,-32.1454831180953,
1.69768315121407E-11));
#23271=CARTESIAN_POINT('Ctrl Pts',(-7.07057502871922,-31.9704831180953,
4.08219839617346));
#23272=CARTESIAN_POINT('Ctrl Pts',(-4.71371668580301,-31.7954831180953,
8.16439679232994));
#23273=CARTESIAN_POINT('Ctrl Pts',(1.47018674401621E-11,-31.6204831180953,
8.16439679232146));
#23274=CARTESIAN_POINT('Ctrl Pts',(4.71371668583241,-31.4454831180953,8.16439679231297));
#23275=CARTESIAN_POINT('Ctrl Pts',(7.07057502873392,-31.2704831180953,4.082198396148));
#23276=CARTESIAN_POINT('Ctrl Pts',(9.42743337163542,-31.0954831180953,-1.69756769845304E-11));
#23277=CARTESIAN_POINT('Ctrl Pts',(7.07057502871922,-30.9204831180953,-4.08219839617346));
#23278=CARTESIAN_POINT('Ctrl Pts',(4.71371668580301,-30.7454831180953,-8.16439679232994));
#23279=CARTESIAN_POINT('Ctrl Pts',(-1.4702867290402E-11,-30.5704831180953,
-8.16439679232146));
#23280=CARTESIAN_POINT('Ctrl Pts',(-4.71371668583241,-30.3954831180953,
-8.16439679231297));
#23281=CARTESIAN_POINT('Ctrl Pts',(-7.07057502873392,-30.2204831180953,
-4.082198396148));
#23282=CARTESIAN_POINT('Ctrl Pts',(-9.42743337163542,-30.0454831180953,
1.69768315121407E-11));
#23283=CARTESIAN_POINT('Ctrl Pts',(-7.07057502871922,-29.8704831180953,
4.08219839617346));
#23284=CARTESIAN_POINT('Ctrl Pts',(-4.71371668580301,-29.6954831180953,
8.16439679232994));
#23285=CARTESIAN_POINT('Ctrl Pts',(1.47018674401621E-11,-29.5204831180953,
8.16439679232146));
#23286=CARTESIAN_POINT('Ctrl Pts',(4.71371668583241,-29.3454831180953,8.16439679231297));
#23287=CARTESIAN_POINT('Ctrl Pts',(7.07057502873392,-29.1704831180953,4.082198396148));
#23288=CARTESIAN_POINT('Ctrl Pts',(9.42743337163542,-28.9954831180954,-1.69756769845304E-11));
#23289=CARTESIAN_POINT('Ctrl Pts',(7.07057502871922,-28.8204831180953,-4.08219839617346));
#23290=CARTESIAN_POINT('Ctrl Pts',(4.71371668580301,-28.6454831180953,-8.16439679232994));
#23291=CARTESIAN_POINT('Ctrl Pts',(-1.4702867290402E-11,-28.4704831180953,
-8.16439679232146));
#23292=CARTESIAN_POINT('Ctrl Pts',(-4.71371668583241,-28.2954831180953,
-8.16439679231297));
#23293=CARTESIAN_POINT('Ctrl Pts',(-7.07057502873392,-28.1204831180953,
-4.082198396148));
#23294=CARTESIAN_POINT('Ctrl Pts',(-9.42743337163542,-27.9454831180954,
1.69768315121407E-11));
#23295=CARTESIAN_POINT('Ctrl Pts',(-7.07057502871922,-27.7704831180953,
4.08219839617346));
#23296=CARTESIAN_POINT('Ctrl Pts',(-4.71371668580301,-27.5954831180953,
8.16439679232994));
#23297=CARTESIAN_POINT('Ctrl Pts',(1.47018674401621E-11,-27.4204831180953,
8.16439679232146));
#23298=CARTESIAN_POINT('Ctrl Pts',(4.71371668583241,-27.2454831180954,8.16439679231297));
#23299=CARTESIAN_POINT('Ctrl Pts',(7.07057502873392,-27.0704831180953,4.082198396148));
#23300=CARTESIAN_POINT('Ctrl Pts',(9.42743337163542,-26.8954831180954,-1.69756769845304E-11));
#23301=CARTESIAN_POINT('Ctrl Pts',(7.07057502871922,-26.7204831180953,-4.08219839617346));
#23302=CARTESIAN_POINT('Ctrl Pts',(4.71371668580301,-26.5454831180953,-8.16439679232994));
#23303=CARTESIAN_POINT('Ctrl Pts',(-1.4702867290402E-11,-26.3704831180953,
-8.16439679232146));
#23304=CARTESIAN_POINT('Ctrl Pts',(-4.71371668583241,-26.1954831180954,
-8.16439679231297));
#23305=CARTESIAN_POINT('Ctrl Pts',(-7.07057502873392,-26.0204831180953,
-4.082198396148));
#23306=CARTESIAN_POINT('Ctrl Pts',(-9.42743337163542,-25.8454831180953,
1.69768315121407E-11));
#23307=CARTESIAN_POINT('Ctrl Pts',(-7.07057502871922,-25.6704831180953,
4.08219839617346));
#23308=CARTESIAN_POINT('Ctrl Pts',(-4.71371668580301,-25.4954831180954,
8.16439679232994));
#23309=CARTESIAN_POINT('Ctrl Pts',(1.47018674401621E-11,-25.3204831180953,
8.16439679232146));
#23310=CARTESIAN_POINT('Ctrl Pts',(4.71371668583241,-25.1454831180954,8.16439679231297));
#23311=CARTESIAN_POINT('Ctrl Pts',(7.07057502873392,-24.9704831180954,4.082198396148));
#23312=CARTESIAN_POINT('Ctrl Pts',(9.42743337163542,-24.7954831180953,-1.69756769845304E-11));
#23313=CARTESIAN_POINT('Ctrl Pts',(7.07057502871922,-24.6204831180954,-4.08219839617346));
#23314=CARTESIAN_POINT('Ctrl Pts',(4.71371668580301,-24.4454831180954,-8.16439679232994));
#23315=CARTESIAN_POINT('Ctrl Pts',(-1.4702867290402E-11,-24.2704831180953,
-8.16439679232146));
#23316=CARTESIAN_POINT('Ctrl Pts',(-4.71371668583241,-24.0954831180954,
-8.16439679231297));
#23317=CARTESIAN_POINT('Ctrl Pts',(-7.07057502873392,-23.9204831180953,
-4.082198396148));
#23318=CARTESIAN_POINT('Ctrl Pts',(-9.42743337163542,-23.7454831180954,
1.69768315121407E-11));
#23319=CARTESIAN_POINT('Ctrl Pts',(-7.07057502871922,-23.5704831180954,
4.08219839617346));
#23320=CARTESIAN_POINT('Ctrl Pts',(-4.71371668580301,-23.3954831180954,
8.16439679232994));
#23321=CARTESIAN_POINT('Ctrl Pts',(1.47018674401621E-11,-23.2204831180953,
8.16439679232146));
#23322=CARTESIAN_POINT('Ctrl Pts',(4.71371668583241,-23.0454831180954,8.16439679231297));
#23323=CARTESIAN_POINT('Ctrl Pts',(7.07057502873392,-22.8704831180954,4.082198396148));
#23324=CARTESIAN_POINT('Ctrl Pts',(9.42743337163542,-22.6954831180954,-1.69756769845304E-11));
#23325=CARTESIAN_POINT('Ctrl Pts',(7.07057502871922,-22.5204831180954,-4.08219839617346));
#23326=CARTESIAN_POINT('Ctrl Pts',(4.71371668580301,-22.3454831180954,-8.16439679232994));
#23327=CARTESIAN_POINT('Ctrl Pts',(-1.4702867290402E-11,-22.1704831180954,
-8.16439679232146));
#23328=CARTESIAN_POINT('Ctrl Pts',(-4.71371668583241,-21.9954831180954,
-8.16439679231297));
#23329=CARTESIAN_POINT('Ctrl Pts',(-7.07057502873392,-21.8204831180954,
-4.082198396148));
#23330=CARTESIAN_POINT('Ctrl Pts',(-9.42743337163542,-21.6454831180954,
1.69768315121407E-11));
#23331=CARTESIAN_POINT('Ctrl Pts',(-7.07057502871922,-21.4704831180953,
4.08219839617346));
#23332=CARTESIAN_POINT('Ctrl Pts',(-4.71371668580301,-21.2954831180954,
8.16439679232994));
#23333=CARTESIAN_POINT('Ctrl Pts',(1.47018674401621E-11,-21.1204831180954,
8.16439679232146));
#23334=CARTESIAN_POINT('Ctrl Pts',(4.71371668583241,-20.9454831180954,8.16439679231297));
#23335=CARTESIAN_POINT('Ctrl Pts',(7.07057502873392,-20.7704831180954,4.082198396148));
#23336=CARTESIAN_POINT('Ctrl Pts',(9.42743337163542,-20.5954831180954,-1.69756769845304E-11));
#23337=CARTESIAN_POINT('Ctrl Pts',(7.07057502871922,-20.4204831180954,-4.08219839617346));
#23338=CARTESIAN_POINT('Ctrl Pts',(4.71371668580301,-20.2454831180954,-8.16439679232994));
#23339=CARTESIAN_POINT('Ctrl Pts',(-1.4702867290402E-11,-20.0704831180954,
-8.16439679232146));
#23340=CARTESIAN_POINT('Ctrl Pts',(-4.71371668583241,-19.8954831180954,
-8.16439679231297));
#23341=CARTESIAN_POINT('Ctrl Pts',(-7.07057502873392,-19.7204831180954,
-4.082198396148));
#23342=CARTESIAN_POINT('Ctrl Pts',(-9.42743337163542,-19.5454831180954,
1.69768315121407E-11));
#23343=CARTESIAN_POINT('Ctrl Pts',(-7.07057502871922,-19.3704831180954,
4.08219839617346));
#23344=CARTESIAN_POINT('Ctrl Pts',(-4.71371668580301,-19.1954831180954,
8.16439679232994));
#23345=CARTESIAN_POINT('Ctrl Pts',(1.47018674401621E-11,-19.0204831180954,
8.16439679232146));
#23346=CARTESIAN_POINT('Ctrl Pts',(4.71371668583241,-18.8454831180954,8.16439679231297));
#23347=CARTESIAN_POINT('Ctrl Pts',(7.07057502873392,-18.6704831180954,4.082198396148));
#23348=CARTESIAN_POINT('Ctrl Pts',(9.42743337163542,-18.4954831180954,-1.69756769845304E-11));
#23349=CARTESIAN_POINT('Ctrl Pts',(7.07057502871922,-18.3204831180954,-4.08219839617346));
#23350=CARTESIAN_POINT('Ctrl Pts',(4.71371668580301,-18.1454831180954,-8.16439679232994));
#23351=CARTESIAN_POINT('Ctrl Pts',(-1.4702867290402E-11,-17.9704831180954,
-8.16439679232146));
#23352=CARTESIAN_POINT('Ctrl Pts',(-4.71371668583241,-17.7954831180954,
-8.16439679231297));
#23353=CARTESIAN_POINT('Ctrl Pts',(-7.07057502873392,-17.6204831180954,
-4.082198396148));
#23354=CARTESIAN_POINT('Ctrl Pts',(-9.42743337163542,-17.4454831180954,
1.69768315121407E-11));
#23355=CARTESIAN_POINT('Ctrl Pts',(-7.07057502871922,-17.2704831180954,
4.08219839617346));
#23356=CARTESIAN_POINT('Ctrl Pts',(-4.71371668580301,-17.0954831180954,
8.16439679232994));
#23357=CARTESIAN_POINT('Ctrl Pts',(1.47018674401621E-11,-16.9204831180954,
8.16439679232146));
#23358=CARTESIAN_POINT('Ctrl Pts',(4.71371668583241,-16.7454831180954,8.16439679231297));
#23359=CARTESIAN_POINT('Ctrl Pts',(7.07057502873392,-16.5704831180954,4.082198396148));
#23360=CARTESIAN_POINT('Ctrl Pts',(9.42743337163542,-16.3954831180954,-1.69756769845304E-11));
#23361=CARTESIAN_POINT('Ctrl Pts',(7.07057502871922,-16.2204831180954,-4.08219839617346));
#23362=CARTESIAN_POINT('Ctrl Pts',(4.71371668580301,-16.0454831180954,-8.16439679232994));
#23363=CARTESIAN_POINT('Ctrl Pts',(-1.4702867290402E-11,-15.8704831180954,
-8.16439679232146));
#23364=CARTESIAN_POINT('Ctrl Pts',(-4.71371668583241,-15.6954831180954,
-8.16439679231297));
#23365=CARTESIAN_POINT('Ctrl Pts',(-7.07057502873392,-15.5204831180954,
-4.082198396148));
#23366=CARTESIAN_POINT('Ctrl Pts',(-9.42743337163542,-15.3454831180954,
1.69768315121407E-11));
#23367=CARTESIAN_POINT('Ctrl Pts',(-7.07057502871922,-15.1704831180954,
4.08219839617346));
#23368=CARTESIAN_POINT('Ctrl Pts',(-4.71371668580301,-14.9954831180954,
8.16439679232994));
#23369=CARTESIAN_POINT('Ctrl Pts',(1.47018674401621E-11,-14.8204831180954,
8.16439679232146));
#23370=CARTESIAN_POINT('Ctrl Pts',(4.71371668583241,-14.6454831180954,8.16439679231297));
#23371=CARTESIAN_POINT('Ctrl Pts',(7.07057502873392,-14.4704831180954,4.082198396148));
#23372=CARTESIAN_POINT('Ctrl Pts',(9.42743337163542,-14.2954831180954,-1.69756769845304E-11));
#23373=CARTESIAN_POINT('Ctrl Pts',(7.07057502871922,-14.1204831180954,-4.08219839617346));
#23374=CARTESIAN_POINT('Ctrl Pts',(4.71371668580301,-13.9454831180954,-8.16439679232994));
#23375=CARTESIAN_POINT('Ctrl Pts',(-1.4702867290402E-11,-13.7704831180954,
-8.16439679232146));
#23376=CARTESIAN_POINT('Ctrl Pts',(-4.71371668583241,-13.5954831180954,
-8.16439679231297));
#23377=CARTESIAN_POINT('Ctrl Pts',(-7.07057502873392,-13.4204831180954,
-4.082198396148));
#23378=CARTESIAN_POINT('Ctrl Pts',(-9.42743337163542,-13.2454831180954,
1.69768315121407E-11));
#23379=CARTESIAN_POINT('Ctrl Pts',(-7.07057502871922,-13.0704831180954,
4.08219839617346));
#23380=CARTESIAN_POINT('Ctrl Pts',(-4.71371668580301,-12.8954831180954,
8.16439679232994));
#23381=CARTESIAN_POINT('Ctrl Pts',(1.47018674401621E-11,-12.7204831180954,
8.16439679232146));
#23382=CARTESIAN_POINT('Ctrl Pts',(4.71371668583241,-12.5454831180954,8.16439679231297));
#23383=CARTESIAN_POINT('Ctrl Pts',(7.07057502873392,-12.3704831180954,4.082198396148));
#23384=CARTESIAN_POINT('Ctrl Pts',(9.42743337163542,-12.1954831180954,-1.69756769845304E-11));
#23385=CARTESIAN_POINT('Ctrl Pts',(7.07057502871922,-12.0204831180954,-4.08219839617346));
#23386=CARTESIAN_POINT('Ctrl Pts',(4.71371668580301,-11.8454831180954,-8.16439679232994));
#23387=CARTESIAN_POINT('Ctrl Pts',(-1.4702867290402E-11,-11.6704831180954,
-8.16439679232146));
#23388=CARTESIAN_POINT('Ctrl Pts',(-4.71371668583241,-11.4954831180954,
-8.16439679231297));
#23389=CARTESIAN_POINT('Ctrl Pts',(-7.07057502873392,-11.3204831180954,
-4.082198396148));
#23390=CARTESIAN_POINT('Ctrl Pts',(-9.42743337163542,-11.1454831180954,
1.69768315121407E-11));
#23391=CARTESIAN_POINT('Ctrl Pts',(-7.07057502871922,-10.9704831180954,
4.08219839617346));
#23392=CARTESIAN_POINT('Ctrl Pts',(-4.71371668580301,-10.7954831180954,
8.16439679232994));
#23393=CARTESIAN_POINT('Ctrl Pts',(1.47018674401621E-11,-10.6204831180954,
8.16439679232146));
#23394=CARTESIAN_POINT('Ctrl Pts',(4.71371668583241,-10.4454831180954,8.16439679231297));
#23395=CARTESIAN_POINT('Ctrl Pts',(7.07057502873392,-10.2704831180954,4.082198396148));
#23396=CARTESIAN_POINT('Ctrl Pts',(9.42743337163542,-10.0954831180954,-1.69756769845304E-11));
#23397=CARTESIAN_POINT('Ctrl Pts',(7.07057502871922,-9.92048311809537,-4.08219839617346));
#23398=CARTESIAN_POINT('Ctrl Pts',(4.71371668580301,-9.74548311809539,-8.16439679232994));
#23399=CARTESIAN_POINT('Ctrl Pts',(-1.4702867290402E-11,-9.57048311809539,
-8.16439679232146));
#23400=CARTESIAN_POINT('Ctrl Pts',(-4.71371668583241,-9.39548311809538,
-8.16439679231297));
#23401=CARTESIAN_POINT('Ctrl Pts',(-7.07057502873392,-9.22048311809539,
-4.082198396148));
#23402=CARTESIAN_POINT('Ctrl Pts',(-9.42743337163542,-9.04548311809539,
1.69768315121407E-11));
#23403=CARTESIAN_POINT('Ctrl Pts',(-7.07057502871922,-8.87048311809537,
4.08219839617346));
#23404=CARTESIAN_POINT('Ctrl Pts',(-4.71371668580301,-8.6954831180954,8.16439679232994));
#23405=CARTESIAN_POINT('Ctrl Pts',(1.47018674401621E-11,-8.52048311809539,
8.16439679232146));
#23406=CARTESIAN_POINT('Ctrl Pts',(4.71371668583241,-8.34548311809539,8.16439679231297));
#23407=CARTESIAN_POINT('Ctrl Pts',(7.07057502873392,-8.1704831180954,4.082198396148));
#23408=CARTESIAN_POINT('Ctrl Pts',(9.42743337163542,-7.9954831180954,-1.69756769845304E-11));
#23409=CARTESIAN_POINT('Ctrl Pts',(7.07057502871922,-7.82048311809538,-4.08219839617346));
#23410=CARTESIAN_POINT('Ctrl Pts',(4.71371668580301,-7.64548311809541,-8.16439679232994));
#23411=CARTESIAN_POINT('Ctrl Pts',(-1.4702867290402E-11,-7.47048311809539,
-8.16439679232146));
#23412=CARTESIAN_POINT('Ctrl Pts',(-4.71371668583241,-7.29548311809539,
-8.16439679231297));
#23413=CARTESIAN_POINT('Ctrl Pts',(-7.07057502873392,-7.12048311809538,
-4.082198396148));
#23414=CARTESIAN_POINT('Ctrl Pts',(-9.42743337163542,-6.94548311809541,
1.69768315121407E-11));
#23415=CARTESIAN_POINT('Ctrl Pts',(-7.07057502871922,-6.77048311809538,
4.08219839617346));
#23416=CARTESIAN_POINT('Ctrl Pts',(-4.71371668580301,-6.59548311809539,
8.16439679232994));
#23417=CARTESIAN_POINT('Ctrl Pts',(1.47018674401621E-11,-6.4204831180954,
8.16439679232146));
#23418=CARTESIAN_POINT('Ctrl Pts',(4.71371668583241,-6.24548311809539,8.16439679231297));
#23419=CARTESIAN_POINT('Ctrl Pts',(7.07057502873392,-6.07048311809538,4.082198396148));
#23420=CARTESIAN_POINT('Ctrl Pts',(9.42743337163542,-5.89548311809541,-1.69756769845304E-11));
#23421=CARTESIAN_POINT('Ctrl Pts',(7.07057502871922,-5.72048311809538,-4.08219839617346));
#23422=CARTESIAN_POINT('Ctrl Pts',(4.71371668580301,-5.54548311809539,-8.16439679232994));
#23423=CARTESIAN_POINT('Ctrl Pts',(-1.4702867290402E-11,-5.3704831180954,
-8.16439679232146));
#23424=CARTESIAN_POINT('Ctrl Pts',(-4.71371668583241,-5.19548311809541,
-8.16439679231297));
#23425=CARTESIAN_POINT('Ctrl Pts',(-7.07057502873392,-5.02048311809538,
-4.082198396148));
#23426=CARTESIAN_POINT('Ctrl Pts',(-9.42743337163542,-4.84548311809541,
1.69768315121407E-11));
#23427=CARTESIAN_POINT('Ctrl Pts',(-7.07057502871922,-4.6704831180954,4.08219839617346));
#23428=CARTESIAN_POINT('Ctrl Pts',(-4.71371668580301,-4.49548311809539,
8.16439679232994));
#23429=CARTESIAN_POINT('Ctrl Pts',(1.47018674401621E-11,-4.3204831180954,
8.16439679232146));
#23430=CARTESIAN_POINT('Ctrl Pts',(4.71371668583241,-4.14548311809541,8.16439679231297));
#23431=CARTESIAN_POINT('Ctrl Pts',(7.07057502873392,-3.97048311809539,4.082198396148));
#23432=CARTESIAN_POINT('Ctrl Pts',(9.42743337163542,-3.79548311809541,-1.69756769845304E-11));
#23433=CARTESIAN_POINT('Ctrl Pts',(7.07057502871922,-3.6204831180954,-4.08219839617346));
#23434=CARTESIAN_POINT('Ctrl Pts',(4.71371668580301,-3.44548311809539,-8.16439679232994));
#23435=CARTESIAN_POINT('Ctrl Pts',(-1.4702867290402E-11,-3.27048311809541,
-8.16439679232146));
#23436=CARTESIAN_POINT('Ctrl Pts',(-4.71371668583241,-3.09548311809541,
-8.16439679231297));
#23437=CARTESIAN_POINT('Ctrl Pts',(-7.07057502873392,-2.92048311809539,
-4.082198396148));
#23438=CARTESIAN_POINT('Ctrl Pts',(-9.42743337163542,-2.74548311809539,
1.69768315121407E-11));
#23439=CARTESIAN_POINT('Ctrl Pts',(-7.07057502871922,-2.5704831180954,4.08219839617346));
#23440=CARTESIAN_POINT('Ctrl Pts',(-4.71371668580301,-2.3954831180954,8.16439679232994));
#23441=CARTESIAN_POINT('Ctrl Pts',(1.47018674401621E-11,-2.22048311809539,
8.16439679232146));
#23442=CARTESIAN_POINT('Ctrl Pts',(4.71371668583241,-2.04548311809541,8.16439679231297));
#23443=CARTESIAN_POINT('Ctrl Pts',(7.07057502873392,-1.87048311809539,4.082198396148));
#23444=CARTESIAN_POINT('Ctrl Pts',(9.42743337163542,-1.69548311809539,-1.69756769845304E-11));
#23445=CARTESIAN_POINT('Ctrl Pts',(7.07057502871922,-1.52048311809541,-4.08219839617346));
#23446=CARTESIAN_POINT('Ctrl Pts',(4.71371668580301,-1.34548311809541,-8.16439679232994));
#23447=CARTESIAN_POINT('Ctrl Pts',(-1.4702867290402E-11,-1.17048311809539,
-8.16439679232146));
#23448=CARTESIAN_POINT('Ctrl Pts',(-4.71371668583241,-0.995483118095416,
-8.16439679231297));
#23449=CARTESIAN_POINT('Ctrl Pts',(-7.07057502873392,-0.820483118095406,
-4.082198396148));
#23450=CARTESIAN_POINT('Ctrl Pts',(-9.42743337163542,-0.645483118095396,
1.69768315121407E-11));
#23451=CARTESIAN_POINT('Ctrl Pts',(-7.07057502871922,-0.47048311809541,
4.08219839617346));
#23452=CARTESIAN_POINT('Ctrl Pts',(-4.71371668580301,-0.295483118095414,
8.16439679232994));
#23453=CARTESIAN_POINT('Ctrl Pts',(1.47018674401621E-11,-0.120483118095393,
8.16439679232146));
#23454=CARTESIAN_POINT('Ctrl Pts',(4.71371668583241,0.054516881904581,8.16439679231297));
#23455=CARTESIAN_POINT('Ctrl Pts',(7.07057502873392,0.229516881904591,4.082198396148));
#23456=CARTESIAN_POINT('Ctrl Pts',(9.42743337163542,0.404516881904601,-1.69756769845304E-11));
#23457=CARTESIAN_POINT('Ctrl Pts',(7.07057502871922,0.579516881904587,-4.08219839617346));
#23458=CARTESIAN_POINT('Ctrl Pts',(4.71371668580301,0.754516881904583,-8.16439679232994));
#23459=CARTESIAN_POINT('Ctrl Pts',(-1.4702867290402E-11,0.929516881904604,
-8.16439679232146));
#23460=CARTESIAN_POINT('Ctrl Pts',(-4.71371668583241,1.10451688190458,-8.16439679231297));
#23461=CARTESIAN_POINT('Ctrl Pts',(-7.07057502873392,1.27951688190459,-4.082198396148));
#23462=CARTESIAN_POINT('Ctrl Pts',(-9.42743337163542,1.4545168819046,1.69768315121407E-11));
#23463=CARTESIAN_POINT('Ctrl Pts',(-7.07057502871922,1.62951688190461,4.08219839617346));
#23464=CARTESIAN_POINT('Ctrl Pts',(-4.71371668580301,1.80451688190458,8.16439679232994));
#23465=CARTESIAN_POINT('Ctrl Pts',(1.47018674401621E-11,1.9795168819046,
8.16439679232146));
#23466=CARTESIAN_POINT('Ctrl Pts',(4.71371668583241,2.1545168819046,8.16439679231297));
#23467=CARTESIAN_POINT('Ctrl Pts',(7.07057502873392,2.32951688190458,4.082198396148));
#23468=CARTESIAN_POINT('Ctrl Pts',(9.42743337163542,2.50451688190458,-1.69756769845304E-11));
#23469=CARTESIAN_POINT('Ctrl Pts',(7.07057502871922,2.6795168819046,-4.08219839617346));
#23470=CARTESIAN_POINT('Ctrl Pts',(4.71371668580301,2.85451688190458,-8.16439679232994));
#23471=CARTESIAN_POINT('Ctrl Pts',(-1.4702867290402E-11,3.02951688190459,
-8.16439679232146));
#23472=CARTESIAN_POINT('Ctrl Pts',(-4.71371668583241,3.2045168819046,-8.16439679231297));
#23473=CARTESIAN_POINT('Ctrl Pts',(-7.07057502873392,3.37951688190458,-4.082198396148));
#23474=CARTESIAN_POINT('Ctrl Pts',(-9.42743337163542,3.55451688190458,1.69768315121407E-11));
#23475=CARTESIAN_POINT('Ctrl Pts',(-7.07057502871922,3.7295168819046,4.08219839617346));
#23476=CARTESIAN_POINT('Ctrl Pts',(-4.71371668580301,3.90451688190458,8.16439679232994));
#23477=CARTESIAN_POINT('Ctrl Pts',(1.47018674401621E-11,4.07951688190458,
8.16439679232146));
#23478=CARTESIAN_POINT('Ctrl Pts',(4.71371668583241,4.2545168819046,8.16439679231297));
#23479=CARTESIAN_POINT('Ctrl Pts',(7.07057502873392,4.42951688190458,4.082198396148));
#23480=CARTESIAN_POINT('Ctrl Pts',(9.42743337163542,4.60451688190458,-1.69756769845304E-11));
#23481=CARTESIAN_POINT('Ctrl Pts',(7.07057502871922,4.7795168819046,-4.08219839617346));
#23482=CARTESIAN_POINT('Ctrl Pts',(4.71371668580301,4.95451688190457,-8.16439679232994));
#23483=CARTESIAN_POINT('Ctrl Pts',(-1.4702867290402E-11,5.12951688190458,
-8.16439679232146));
#23484=CARTESIAN_POINT('Ctrl Pts',(-4.71371668583241,5.30451688190459,-8.16439679231297));
#23485=CARTESIAN_POINT('Ctrl Pts',(-7.07057502873392,5.47951688190458,-4.082198396148));
#23486=CARTESIAN_POINT('Ctrl Pts',(-9.42743337163542,5.65451688190458,1.69768315121407E-11));
#23487=CARTESIAN_POINT('Ctrl Pts',(-7.07057502871922,5.82951688190459,4.08219839617346));
#23488=CARTESIAN_POINT('Ctrl Pts',(-4.71371668580301,6.00451688190457,8.16439679232994));
#23489=CARTESIAN_POINT('Ctrl Pts',(1.47018674401621E-11,6.17951688190458,
8.16439679232146));
#23490=CARTESIAN_POINT('Ctrl Pts',(4.71371668583241,6.35451688190459,8.16439679231297));
#23491=CARTESIAN_POINT('Ctrl Pts',(7.07057502873392,6.52951688190459,4.082198396148));
#23492=CARTESIAN_POINT('Ctrl Pts',(9.42743337163542,6.70451688190457,-1.69756769845304E-11));
#23493=CARTESIAN_POINT('Ctrl Pts',(7.07057502871922,6.87951688190458,-4.08219839617346));
#23494=CARTESIAN_POINT('Ctrl Pts',(4.71371668580301,7.05451688190459,-8.16439679232994));
#23495=CARTESIAN_POINT('Ctrl Pts',(-1.4702867290402E-11,7.22951688190457,
-8.16439679232146));
#23496=CARTESIAN_POINT('Ctrl Pts',(-4.71371668583241,7.40451688190458,-8.16439679231297));
#23497=CARTESIAN_POINT('Ctrl Pts',(-7.07057502873392,7.57951688190459,-4.082198396148));
#23498=CARTESIAN_POINT('Ctrl Pts',(-9.42743337163542,7.75451688190457,1.69768315121407E-11));
#23499=CARTESIAN_POINT('Ctrl Pts',(-7.07057502871922,7.92951688190458,4.08219839617346));
#23500=CARTESIAN_POINT('Ctrl Pts',(-4.71371668580301,8.10451688190458,8.16439679232994));
#23501=CARTESIAN_POINT('Ctrl Pts',(1.47018674401621E-11,8.27951688190457,
8.16439679232146));
#23502=CARTESIAN_POINT('Ctrl Pts',(4.71371668583241,8.45451688190457,8.16439679231297));
#23503=CARTESIAN_POINT('Ctrl Pts',(7.07057502873392,8.62951688190459,4.082198396148));
#23504=CARTESIAN_POINT('Ctrl Pts',(9.42743337163542,8.80451688190457,-1.69756769845304E-11));
#23505=CARTESIAN_POINT('Ctrl Pts',(7.07057502871922,8.97951688190457,-4.08219839617346));
#23506=CARTESIAN_POINT('Ctrl Pts',(4.71371668580301,9.15451688190458,-8.16439679232994));
#23507=CARTESIAN_POINT('Ctrl Pts',(-1.4702867290402E-11,9.32951688190457,
-8.16439679232146));
#23508=CARTESIAN_POINT('Ctrl Pts',(-4.71371668583241,9.50451688190457,-8.16439679231297));
#23509=CARTESIAN_POINT('Ctrl Pts',(-7.07057502873392,9.67951688190458,-4.082198396148));
#23510=CARTESIAN_POINT('Ctrl Pts',(-9.42743337163542,9.85451688190457,1.69768315121407E-11));
#23511=CARTESIAN_POINT('Ctrl Pts',(-7.07057502871922,10.0295168819046,4.08219839617346));
#23512=CARTESIAN_POINT('Ctrl Pts',(-4.71371668580301,10.2045168819046,8.16439679232994));
#23513=CARTESIAN_POINT('Ctrl Pts',(1.47018674401621E-11,10.3795168819046,
8.16439679232146));
#23514=CARTESIAN_POINT('Ctrl Pts',(4.71371668583241,10.5545168819046,8.16439679231297));
#23515=CARTESIAN_POINT('Ctrl Pts',(7.07057502873392,10.7295168819046,4.082198396148));
#23516=CARTESIAN_POINT('Ctrl Pts',(9.42743337163542,10.9045168819046,-1.69756769845304E-11));
#23517=CARTESIAN_POINT('Ctrl Pts',(7.07057502871922,11.0795168819046,-4.08219839617346));
#23518=CARTESIAN_POINT('Ctrl Pts',(4.71371668580301,11.2545168819046,-8.16439679232994));
#23519=CARTESIAN_POINT('Ctrl Pts',(-1.4702867290402E-11,11.4295168819046,
-8.16439679232146));
#23520=CARTESIAN_POINT('Ctrl Pts',(-4.71371668583241,11.6045168819046,-8.16439679231297));
#23521=CARTESIAN_POINT('Ctrl Pts',(-7.07057502873392,11.7795168819046,-4.082198396148));
#23522=CARTESIAN_POINT('Ctrl Pts',(-9.42743337163542,11.9545168819046,1.69768315121407E-11));
#23523=CARTESIAN_POINT('Ctrl Pts',(-7.07057502871922,12.1295168819046,4.08219839617346));
#23524=CARTESIAN_POINT('Ctrl Pts',(-4.71371668580301,12.3045168819046,8.16439679232994));
#23525=CARTESIAN_POINT('Ctrl Pts',(1.47018674401621E-11,12.4795168819046,
8.16439679232146));
#23526=CARTESIAN_POINT('Ctrl Pts',(4.71371668583241,12.6545168819046,8.16439679231297));
#23527=CARTESIAN_POINT('Ctrl Pts',(7.07057502873392,12.8295168819046,4.082198396148));
#23528=CARTESIAN_POINT('Ctrl Pts',(9.42743337163542,13.0045168819046,-1.69756769845304E-11));
#23529=CARTESIAN_POINT('Ctrl Pts',(7.07057502871922,13.1795168819046,-4.08219839617346));
#23530=CARTESIAN_POINT('Ctrl Pts',(4.71371668580301,13.3545168819046,-8.16439679232994));
#23531=CARTESIAN_POINT('Ctrl Pts',(-1.4702867290402E-11,13.5295168819046,
-8.16439679232146));
#23532=CARTESIAN_POINT('Ctrl Pts',(-4.71371668583241,13.7045168819046,-8.16439679231297));
#23533=CARTESIAN_POINT('Ctrl Pts',(-7.07057502873392,13.8795168819046,-4.082198396148));
#23534=CARTESIAN_POINT('Ctrl Pts',(-9.42743337163542,14.0545168819046,1.69768315121407E-11));
#23535=CARTESIAN_POINT('Ctrl Pts',(-7.07057502871922,14.2295168819046,4.08219839617346));
#23536=CARTESIAN_POINT('Ctrl Pts',(-4.71371668580301,14.4045168819046,8.16439679232994));
#23537=CARTESIAN_POINT('Ctrl Pts',(1.47018674401621E-11,14.5795168819046,
8.16439679232146));
#23538=CARTESIAN_POINT('Ctrl Pts',(4.71371668583241,14.7545168819045,8.16439679231297));
#23539=CARTESIAN_POINT('Ctrl Pts',(7.07057502873392,14.9295168819046,4.082198396148));
#23540=CARTESIAN_POINT('Ctrl Pts',(9.42743337163542,15.1045168819046,-1.69756769845304E-11));
#23541=CARTESIAN_POINT('Ctrl Pts',(7.07057502871922,15.2795168819046,-4.08219839617346));
#23542=CARTESIAN_POINT('Ctrl Pts',(4.71371668580301,15.4545168819046,-8.16439679232994));
#23543=CARTESIAN_POINT('Ctrl Pts',(-1.4702867290402E-11,15.6295168819046,
-8.16439679232146));
#23544=CARTESIAN_POINT('Ctrl Pts',(-4.71371668583241,15.8045168819046,-8.16439679231297));
#23545=CARTESIAN_POINT('Ctrl Pts',(-7.07057502873392,15.9795168819046,-4.082198396148));
#23546=CARTESIAN_POINT('Ctrl Pts',(-9.42743337163542,16.1545168819046,1.69768315121407E-11));
#23547=CARTESIAN_POINT('Ctrl Pts',(-7.07057502871922,16.3295168819046,4.08219839617346));
#23548=CARTESIAN_POINT('Ctrl Pts',(-4.71371668580301,16.5045168819046,8.16439679232994));
#23549=CARTESIAN_POINT('Ctrl Pts',(1.47018674401621E-11,16.6795168819046,
8.16439679232146));
#23550=CARTESIAN_POINT('Ctrl Pts',(4.71371668583241,16.8545168819046,8.16439679231297));
#23551=CARTESIAN_POINT('Ctrl Pts',(7.07057502873392,17.0295168819046,4.082198396148));
#23552=CARTESIAN_POINT('Ctrl Pts',(9.42743337163542,17.2045168819045,-1.69756769845304E-11));
#23553=CARTESIAN_POINT('Ctrl Pts',(7.07057502871922,17.3795168819046,-4.08219839617346));
#23554=CARTESIAN_POINT('Ctrl Pts',(4.71371668580301,17.5545168819045,-8.16439679232994));
#23555=CARTESIAN_POINT('Ctrl Pts',(-1.4702867290402E-11,17.7295168819046,
-8.16439679232146));
#23556=CARTESIAN_POINT('Ctrl Pts',(-4.71371668583241,17.9045168819046,-8.16439679231297));
#23557=CARTESIAN_POINT('Ctrl Pts',(-7.07057502873392,18.0795168819045,-4.082198396148));
#23558=CARTESIAN_POINT('Ctrl Pts',(-9.42743337163542,18.2545168819045,1.69768315121407E-11));
#23559=CARTESIAN_POINT('Ctrl Pts',(-7.07057502871922,18.4295168819046,4.08219839617346));
#23560=CARTESIAN_POINT('Ctrl Pts',(-4.71371668580301,18.6045168819045,8.16439679232994));
#23561=CARTESIAN_POINT('Ctrl Pts',(1.47018674401621E-11,18.7795168819046,
8.16439679232146));
#23562=CARTESIAN_POINT('Ctrl Pts',(4.71371668583241,18.9545168819045,8.16439679231297));
#23563=CARTESIAN_POINT('Ctrl Pts',(7.07057502873392,19.1295168819045,4.082198396148));
#23564=CARTESIAN_POINT('Ctrl Pts',(9.42743337163542,19.3045168819045,-1.69756769845304E-11));
#23565=CARTESIAN_POINT('Ctrl Pts',(7.07057502871922,19.4795168819046,-4.08219839617346));
#23566=CARTESIAN_POINT('Ctrl Pts',(4.71371668580301,19.6545168819046,-8.16439679232994));
#23567=CARTESIAN_POINT('Ctrl Pts',(-1.4702867290402E-11,19.8295168819045,
-8.16439679232146));
#23568=CARTESIAN_POINT('Ctrl Pts',(-4.71371668583241,20.0045168819045,-8.16439679231297));
#23569=CARTESIAN_POINT('Ctrl Pts',(-7.07057502873392,20.1795168819046,-4.082198396148));
#23570=CARTESIAN_POINT('Ctrl Pts',(-9.42743337163542,20.3545168819045,1.69768315121407E-11));
#23571=CARTESIAN_POINT('Ctrl Pts',(-7.07057502871922,20.5295168819046,4.08219839617346));
#23572=CARTESIAN_POINT('Ctrl Pts',(-4.71371668580301,20.7045168819046,8.16439679232994));
#23573=CARTESIAN_POINT('Ctrl Pts',(1.47018674401621E-11,20.8795168819045,
8.16439679232146));
#23574=CARTESIAN_POINT('Ctrl Pts',(4.71371668583241,21.0545168819045,8.16439679231297));
#23575=CARTESIAN_POINT('Ctrl Pts',(7.07057502873392,21.2295168819046,4.082198396148));
#23576=CARTESIAN_POINT('Ctrl Pts',(9.42743337163542,21.4045168819045,-1.69756769845304E-11));
#23577=CARTESIAN_POINT('Ctrl Pts',(7.07057502871922,21.5795168819045,-4.08219839617346));
#23578=CARTESIAN_POINT('Ctrl Pts',(4.71371668580301,21.7545168819045,-8.16439679232994));
#23579=CARTESIAN_POINT('Ctrl Pts',(-1.4702867290402E-11,21.9295168819045,
-8.16439679232146));
#23580=CARTESIAN_POINT('Ctrl Pts',(-4.71371668583241,22.1045168819045,-8.16439679231297));
#23581=CARTESIAN_POINT('Ctrl Pts',(-7.07057502873392,22.2795168819046,-4.082198396148));
#23582=CARTESIAN_POINT('Ctrl Pts',(-9.42743337163542,22.4545168819045,1.69768315121407E-11));
#23583=CARTESIAN_POINT('Ctrl Pts',(-7.07057502871922,22.6295168819045,4.08219839617346));
#23584=CARTESIAN_POINT('Ctrl Pts',(-4.71371668580301,22.8045168819045,8.16439679232994));
#23585=CARTESIAN_POINT('Ctrl Pts',(1.47018674401621E-11,22.9795168819045,
8.16439679232146));
#23586=CARTESIAN_POINT('Ctrl Pts',(4.71371668583241,23.1545168819045,8.16439679231297));
#23587=CARTESIAN_POINT('Ctrl Pts',(7.07057502873392,23.3295168819046,4.082198396148));
#23588=CARTESIAN_POINT('Ctrl Pts',(9.42743337163542,23.5045168819045,-1.69756769845304E-11));
#23589=CARTESIAN_POINT('Ctrl Pts',(7.07057502871922,23.6795168819045,-4.08219839617346));
#23590=CARTESIAN_POINT('Ctrl Pts',(4.71371668580301,23.8545168819045,-8.16439679232994));
#23591=CARTESIAN_POINT('Ctrl Pts',(-1.4702867290402E-11,24.0295168819045,
-8.16439679232146));
#23592=CARTESIAN_POINT('Ctrl Pts',(-4.71371668583241,24.2045168819045,-8.16439679231297));
#23593=CARTESIAN_POINT('Ctrl Pts',(-7.07057502873392,24.3795168819046,-4.082198396148));
#23594=CARTESIAN_POINT('Ctrl Pts',(-9.42743337163542,24.5545168819046,1.69768315121407E-11));
#23595=CARTESIAN_POINT('Ctrl Pts',(-7.07057502871922,24.7295168819045,4.08219839617346));
#23596=CARTESIAN_POINT('Ctrl Pts',(-4.71371668580301,24.9045168819045,8.16439679232994));
#23597=CARTESIAN_POINT('Ctrl Pts',(1.47018674401621E-11,25.0795168819046,
8.16439679232146));
#23598=CARTESIAN_POINT('Ctrl Pts',(4.71371668583241,25.2545168819045,8.16439679231297));
#23599=CARTESIAN_POINT('Ctrl Pts',(7.07057502873392,25.4295168819045,4.082198396148));
#23600=CARTESIAN_POINT('Ctrl Pts',(9.42743337163542,25.6045168819045,-1.69756769845304E-11));
#23601=CARTESIAN_POINT('Ctrl Pts',(7.07057502871922,25.7795168819045,-4.08219839617346));
#23602=CARTESIAN_POINT('Ctrl Pts',(4.71371668580301,25.9545168819045,-8.16439679232994));
#23603=CARTESIAN_POINT('Ctrl Pts',(-1.4702867290402E-11,26.1295168819045,
-8.16439679232146));
#23604=CARTESIAN_POINT('Ctrl Pts',(-1.4702867290402E-11,-143.703019107145,
-8.16439679232146));
#23605=CARTESIAN_POINT('Ctrl Pts',(-4.71371668583241,-143.528019107145,
-8.16439679231297));
#23606=CARTESIAN_POINT('Ctrl Pts',(-7.07057502873392,-143.353019107145,
-4.082198396148));
#23607=CARTESIAN_POINT('Ctrl Pts',(-9.42743337163542,-143.178019107145,
1.69768315121407E-11));
#23608=CARTESIAN_POINT('Ctrl Pts',(-7.07057502871922,-143.003019107145,
4.08219839617346));
#23609=CARTESIAN_POINT('Ctrl Pts',(-4.71371668580301,-142.828019107145,
8.16439679232994));
#23610=CARTESIAN_POINT('Ctrl Pts',(1.47018674401621E-11,-142.653019107145,
8.16439679232146));
#23611=CARTESIAN_POINT('Ctrl Pts',(4.71371668583241,-142.478019107145,8.16439679231297));
#23612=CARTESIAN_POINT('Ctrl Pts',(7.07057502873392,-142.303019107145,4.082198396148));
#23613=CARTESIAN_POINT('Ctrl Pts',(9.42743337163542,-142.128019107145,-1.69756769845304E-11));
#23614=CARTESIAN_POINT('Ctrl Pts',(7.07057502871922,-141.953019107145,-4.08219839617346));
#23615=CARTESIAN_POINT('Ctrl Pts',(4.71371668580301,-141.778019107145,-8.16439679232994));
#23616=CARTESIAN_POINT('Ctrl Pts',(-1.4702867290402E-11,-141.603019107145,
-8.16439679232146));
#23617=CARTESIAN_POINT('Ctrl Pts',(-4.71371668583241,-141.428019107145,
-8.16439679231297));
#23618=CARTESIAN_POINT('Ctrl Pts',(-7.07057502873392,-141.253019107145,
-4.082198396148));
#23619=CARTESIAN_POINT('Ctrl Pts',(-9.42743337163542,-141.078019107145,
1.69768315121407E-11));
#23620=CARTESIAN_POINT('Ctrl Pts',(-7.07057502871922,-140.903019107145,
4.08219839617346));
#23621=CARTESIAN_POINT('Ctrl Pts',(-4.71371668580301,-140.728019107145,
8.16439679232994));
#23622=CARTESIAN_POINT('Ctrl Pts',(1.47018674401621E-11,-140.553019107145,
8.16439679232146));
#23623=CARTESIAN_POINT('Ctrl Pts',(4.71371668583241,-140.378019107145,8.16439679231297));
#23624=CARTESIAN_POINT('Ctrl Pts',(7.07057502873392,-140.203019107145,4.082198396148));
#23625=CARTESIAN_POINT('Ctrl Pts',(9.42743337163542,-140.028019107145,-1.69756769845304E-11));
#23626=CARTESIAN_POINT('Ctrl Pts',(7.07057502871922,-139.853019107145,-4.08219839617346));
#23627=CARTESIAN_POINT('Ctrl Pts',(4.71371668580301,-139.678019107145,-8.16439679232994));
#23628=CARTESIAN_POINT('Ctrl Pts',(-1.4702867290402E-11,-139.503019107145,
-8.16439679232146));
#23629=CARTESIAN_POINT('Ctrl Pts',(-4.71371668583241,-139.328019107145,
-8.16439679231297));
#23630=CARTESIAN_POINT('Ctrl Pts',(-7.07057502873392,-139.153019107145,
-4.082198396148));
#23631=CARTESIAN_POINT('Ctrl Pts',(-9.42743337163542,-138.978019107145,
1.69768315121407E-11));
#23632=CARTESIAN_POINT('Ctrl Pts',(-7.07057502871922,-138.803019107145,
4.08219839617346));
#23633=CARTESIAN_POINT('Ctrl Pts',(-4.71371668580301,-138.628019107145,
8.16439679232994));
#23634=CARTESIAN_POINT('Ctrl Pts',(1.47018674401621E-11,-138.453019107145,
8.16439679232146));
#23635=CARTESIAN_POINT('Ctrl Pts',(4.71371668583241,-138.278019107145,8.16439679231297));
#23636=CARTESIAN_POINT('Ctrl Pts',(7.07057502873392,-138.103019107145,4.082198396148));
#23637=CARTESIAN_POINT('Ctrl Pts',(9.42743337163542,-137.928019107145,-1.69756769845304E-11));
#23638=CARTESIAN_POINT('Ctrl Pts',(7.07057502871922,-137.753019107145,-4.08219839617346));
#23639=CARTESIAN_POINT('Ctrl Pts',(4.71371668580301,-137.578019107145,-8.16439679232994));
#23640=CARTESIAN_POINT('Ctrl Pts',(-1.4702867290402E-11,-137.403019107145,
-8.16439679232146));
#23641=CARTESIAN_POINT('Ctrl Pts',(-4.71371668583241,-137.228019107145,
-8.16439679231297));
#23642=CARTESIAN_POINT('Ctrl Pts',(-7.07057502873392,-137.053019107145,
-4.082198396148));
#23643=CARTESIAN_POINT('Ctrl Pts',(-9.42743337163542,-136.878019107145,
1.69768315121407E-11));
#23644=CARTESIAN_POINT('Ctrl Pts',(-7.07057502871922,-136.703019107145,
4.08219839617346));
#23645=CARTESIAN_POINT('Ctrl Pts',(-4.71371668580301,-136.528019107145,
8.16439679232994));
#23646=CARTESIAN_POINT('Ctrl Pts',(1.47018674401621E-11,-136.353019107145,
8.16439679232146));
#23647=CARTESIAN_POINT('Ctrl Pts',(4.71371668583241,-136.178019107145,8.16439679231297));
#23648=CARTESIAN_POINT('Ctrl Pts',(7.07057502873392,-136.003019107145,4.082198396148));
#23649=CARTESIAN_POINT('Ctrl Pts',(9.42743337163542,-135.828019107145,-1.69756769845304E-11));
#23650=CARTESIAN_POINT('Ctrl Pts',(7.07057502871922,-135.653019107145,-4.08219839617346));
#23651=CARTESIAN_POINT('Ctrl Pts',(4.71371668580301,-135.478019107145,-8.16439679232994));
#23652=CARTESIAN_POINT('Ctrl Pts',(-1.4702867290402E-11,-135.303019107145,
-8.16439679232146));
#23653=CARTESIAN_POINT('Ctrl Pts',(-4.71371668583241,-135.128019107145,
-8.16439679231297));
#23654=CARTESIAN_POINT('Ctrl Pts',(-7.07057502873392,-134.953019107145,
-4.082198396148));
#23655=CARTESIAN_POINT('Ctrl Pts',(-9.42743337163542,-134.778019107145,
1.69768315121407E-11));
#23656=CARTESIAN_POINT('Ctrl Pts',(-7.07057502871922,-134.603019107145,
4.08219839617346));
#23657=CARTESIAN_POINT('Ctrl Pts',(-4.71371668580301,-134.428019107145,
8.16439679232994));
#23658=CARTESIAN_POINT('Ctrl Pts',(1.47018674401621E-11,-134.253019107145,
8.16439679232146));
#23659=CARTESIAN_POINT('Ctrl Pts',(4.71371668583241,-134.078019107145,8.16439679231297));
#23660=CARTESIAN_POINT('Ctrl Pts',(7.07057502873392,-133.903019107145,4.082198396148));
#23661=CARTESIAN_POINT('Ctrl Pts',(9.42743337163542,-133.728019107145,-1.69756769845304E-11));
#23662=CARTESIAN_POINT('Ctrl Pts',(7.07057502871922,-133.553019107145,-4.08219839617346));
#23663=CARTESIAN_POINT('Ctrl Pts',(4.71371668580301,-133.378019107145,-8.16439679232994));
#23664=CARTESIAN_POINT('Ctrl Pts',(-1.4702867290402E-11,-133.203019107145,
-8.16439679232146));
#23665=CARTESIAN_POINT('Ctrl Pts',(-4.71371668583241,-133.028019107145,
-8.16439679231297));
#23666=CARTESIAN_POINT('Ctrl Pts',(-7.07057502873392,-132.853019107145,
-4.082198396148));
#23667=CARTESIAN_POINT('Ctrl Pts',(-9.42743337163542,-132.678019107145,
1.69768315121407E-11));
#23668=CARTESIAN_POINT('Ctrl Pts',(-7.07057502871922,-132.503019107145,
4.08219839617346));
#23669=CARTESIAN_POINT('Ctrl Pts',(-4.71371668580301,-132.328019107145,
8.16439679232994));
#23670=CARTESIAN_POINT('Ctrl Pts',(1.47018674401621E-11,-132.153019107145,
8.16439679232146));
#23671=CARTESIAN_POINT('Ctrl Pts',(4.71371668583241,-131.978019107145,8.16439679231297));
#23672=CARTESIAN_POINT('Ctrl Pts',(7.07057502873392,-131.803019107145,4.082198396148));
#23673=CARTESIAN_POINT('Ctrl Pts',(9.42743337163542,-131.628019107145,-1.69756769845304E-11));
#23674=CARTESIAN_POINT('Ctrl Pts',(7.07057502871922,-131.453019107145,-4.08219839617346));
#23675=CARTESIAN_POINT('Ctrl Pts',(4.71371668580301,-131.278019107145,-8.16439679232994));
#23676=CARTESIAN_POINT('Ctrl Pts',(-1.4702867290402E-11,-131.103019107145,
-8.16439679232146));
#23677=CARTESIAN_POINT('Ctrl Pts',(-4.71371668583241,-130.928019107145,
-8.16439679231297));
#23678=CARTESIAN_POINT('Ctrl Pts',(-7.07057502873392,-130.753019107145,
-4.082198396148));
#23679=CARTESIAN_POINT('Ctrl Pts',(-9.42743337163542,-130.578019107145,
1.69768315121407E-11));
#23680=CARTESIAN_POINT('Ctrl Pts',(-7.07057502871922,-130.403019107145,
4.08219839617346));
#23681=CARTESIAN_POINT('Ctrl Pts',(-4.71371668580301,-130.228019107145,
8.16439679232994));
#23682=CARTESIAN_POINT('Ctrl Pts',(1.47018674401621E-11,-130.053019107145,
8.16439679232146));
#23683=CARTESIAN_POINT('Ctrl Pts',(4.71371668583241,-129.878019107145,8.16439679231297));
#23684=CARTESIAN_POINT('Ctrl Pts',(7.07057502873392,-129.703019107145,4.082198396148));
#23685=CARTESIAN_POINT('Ctrl Pts',(9.42743337163542,-129.528019107145,-1.69756769845304E-11));
#23686=CARTESIAN_POINT('Ctrl Pts',(7.07057502871922,-129.353019107145,-4.08219839617346));
#23687=CARTESIAN_POINT('Ctrl Pts',(4.71371668580301,-129.178019107145,-8.16439679232994));
#23688=CARTESIAN_POINT('Ctrl Pts',(-1.4702867290402E-11,-129.003019107145,
-8.16439679232146));
#23689=CARTESIAN_POINT('Ctrl Pts',(-4.71371668583241,-128.828019107145,
-8.16439679231297));
#23690=CARTESIAN_POINT('Ctrl Pts',(-7.07057502873392,-128.653019107145,
-4.082198396148));
#23691=CARTESIAN_POINT('Ctrl Pts',(-9.42743337163542,-128.478019107145,
1.69768315121407E-11));
#23692=CARTESIAN_POINT('Ctrl Pts',(-7.07057502871922,-128.303019107145,
4.08219839617346));
#23693=CARTESIAN_POINT('Ctrl Pts',(-4.71371668580301,-128.128019107145,
8.16439679232994));
#23694=CARTESIAN_POINT('Ctrl Pts',(1.47018674401621E-11,-127.953019107145,
8.16439679232146));
#23695=CARTESIAN_POINT('Ctrl Pts',(4.71371668583241,-127.778019107145,8.16439679231297));
#23696=CARTESIAN_POINT('Ctrl Pts',(7.07057502873392,-127.603019107145,4.082198396148));
#23697=CARTESIAN_POINT('Ctrl Pts',(9.42743337163542,-127.428019107145,-1.69756769845304E-11));
#23698=CARTESIAN_POINT('Ctrl Pts',(7.07057502871922,-127.253019107145,-4.08219839617346));
#23699=CARTESIAN_POINT('Ctrl Pts',(4.71371668580301,-127.078019107145,-8.16439679232994));
#23700=CARTESIAN_POINT('Ctrl Pts',(-1.4702867290402E-11,-126.903019107145,
-8.16439679232146));
#23701=CARTESIAN_POINT('Ctrl Pts',(-4.71371668583241,-126.728019107145,
-8.16439679231297));
#23702=CARTESIAN_POINT('Ctrl Pts',(-7.07057502873392,-126.553019107145,
-4.082198396148));
#23703=CARTESIAN_POINT('Ctrl Pts',(-9.42743337163542,-126.378019107145,
1.69768315121407E-11));
#23704=CARTESIAN_POINT('Ctrl Pts',(-7.07057502871922,-126.203019107145,
4.08219839617346));
#23705=CARTESIAN_POINT('Ctrl Pts',(-4.71371668580301,-126.028019107145,
8.16439679232994));
#23706=CARTESIAN_POINT('Ctrl Pts',(1.47018674401621E-11,-125.853019107145,
8.16439679232146));
#23707=CARTESIAN_POINT('Ctrl Pts',(4.71371668583241,-125.678019107145,8.16439679231297));
#23708=CARTESIAN_POINT('Ctrl Pts',(7.07057502873392,-125.503019107145,4.082198396148));
#23709=CARTESIAN_POINT('Ctrl Pts',(9.42743337163542,-125.328019107145,-1.69756769845304E-11));
#23710=CARTESIAN_POINT('Ctrl Pts',(7.07057502871922,-125.153019107145,-4.08219839617346));
#23711=CARTESIAN_POINT('Ctrl Pts',(4.71371668580301,-124.978019107145,-8.16439679232994));
#23712=CARTESIAN_POINT('Ctrl Pts',(-1.4702867290402E-11,-124.803019107145,
-8.16439679232146));
#23713=CARTESIAN_POINT('Ctrl Pts',(-4.71371668583241,-124.628019107145,
-8.16439679231297));
#23714=CARTESIAN_POINT('Ctrl Pts',(-7.07057502873392,-124.453019107145,
-4.082198396148));
#23715=CARTESIAN_POINT('Ctrl Pts',(-9.42743337163542,-124.278019107145,
1.69768315121407E-11));
#23716=CARTESIAN_POINT('Ctrl Pts',(-7.07057502871922,-124.103019107145,
4.08219839617346));
#23717=CARTESIAN_POINT('Ctrl Pts',(-4.71371668580301,-123.928019107145,
8.16439679232994));
#23718=CARTESIAN_POINT('Ctrl Pts',(1.47018674401621E-11,-123.753019107145,
8.16439679232146));
#23719=CARTESIAN_POINT('Ctrl Pts',(4.71371668583241,-123.578019107145,8.16439679231297));
#23720=CARTESIAN_POINT('Ctrl Pts',(7.07057502873392,-123.403019107145,4.082198396148));
#23721=CARTESIAN_POINT('Ctrl Pts',(9.42743337163542,-123.228019107145,-1.69756769845304E-11));
#23722=CARTESIAN_POINT('Ctrl Pts',(7.07057502871922,-123.053019107145,-4.08219839617346));
#23723=CARTESIAN_POINT('Ctrl Pts',(4.71371668580301,-122.878019107145,-8.16439679232994));
#23724=CARTESIAN_POINT('Ctrl Pts',(-1.4702867290402E-11,-122.703019107145,
-8.16439679232146));
#23725=CARTESIAN_POINT('Ctrl Pts',(-4.71371668583241,-122.528019107145,
-8.16439679231297));
#23726=CARTESIAN_POINT('Ctrl Pts',(-7.07057502873392,-122.353019107145,
-4.082198396148));
#23727=CARTESIAN_POINT('Ctrl Pts',(-9.42743337163542,-122.178019107145,
1.69768315121407E-11));
#23728=CARTESIAN_POINT('Ctrl Pts',(-7.07057502871922,-122.003019107145,
4.08219839617346));
#23729=CARTESIAN_POINT('Ctrl Pts',(-4.71371668580301,-121.828019107145,
8.16439679232994));
#23730=CARTESIAN_POINT('Ctrl Pts',(1.47018674401621E-11,-121.653019107145,
8.16439679232146));
#23731=CARTESIAN_POINT('Ctrl Pts',(4.71371668583241,-121.478019107145,8.16439679231297));
#23732=CARTESIAN_POINT('Ctrl Pts',(7.07057502873392,-121.303019107145,4.082198396148));
#23733=CARTESIAN_POINT('Ctrl Pts',(9.42743337163542,-121.128019107145,-1.69756769845304E-11));
#23734=CARTESIAN_POINT('Ctrl Pts',(7.07057502871922,-120.953019107145,-4.08219839617346));
#23735=CARTESIAN_POINT('Ctrl Pts',(4.71371668580301,-120.778019107145,-8.16439679232994));
#23736=CARTESIAN_POINT('Ctrl Pts',(-1.4702867290402E-11,-120.603019107145,
-8.16439679232146));
#23737=CARTESIAN_POINT('Ctrl Pts',(-4.71371668583241,-120.428019107145,
-8.16439679231297));
#23738=CARTESIAN_POINT('Ctrl Pts',(-7.07057502873392,-120.253019107145,
-4.082198396148));
#23739=CARTESIAN_POINT('Ctrl Pts',(-9.42743337163542,-120.078019107145,
1.69768315121407E-11));
#23740=CARTESIAN_POINT('Ctrl Pts',(-7.07057502871922,-119.903019107145,
4.08219839617346));
#23741=CARTESIAN_POINT('Ctrl Pts',(-4.71371668580301,-119.728019107145,
8.16439679232994));
#23742=CARTESIAN_POINT('Ctrl Pts',(1.47018674401621E-11,-119.553019107145,
8.16439679232146));
#23743=CARTESIAN_POINT('Ctrl Pts',(4.71371668583241,-119.378019107145,8.16439679231297));
#23744=CARTESIAN_POINT('Ctrl Pts',(7.07057502873392,-119.203019107145,4.082198396148));
#23745=CARTESIAN_POINT('Ctrl Pts',(9.42743337163542,-119.028019107145,-1.69756769845304E-11));
#23746=CARTESIAN_POINT('Ctrl Pts',(7.07057502871922,-118.853019107145,-4.08219839617346));
#23747=CARTESIAN_POINT('Ctrl Pts',(4.71371668580301,-118.678019107145,-8.16439679232994));
#23748=CARTESIAN_POINT('Ctrl Pts',(-1.4702867290402E-11,-118.503019107145,
-8.16439679232146));
#23749=CARTESIAN_POINT('Ctrl Pts',(-4.71371668583241,-118.328019107145,
-8.16439679231297));
#23750=CARTESIAN_POINT('Ctrl Pts',(-7.07057502873392,-118.153019107145,
-4.082198396148));
#23751=CARTESIAN_POINT('Ctrl Pts',(-9.42743337163542,-117.978019107145,
1.69768315121407E-11));
#23752=CARTESIAN_POINT('Ctrl Pts',(-7.07057502871922,-117.803019107145,
4.08219839617346));
#23753=CARTESIAN_POINT('Ctrl Pts',(-4.71371668580301,-117.628019107145,
8.16439679232994));
#23754=CARTESIAN_POINT('Ctrl Pts',(1.47018674401621E-11,-117.453019107145,
8.16439679232146));
#23755=CARTESIAN_POINT('Ctrl Pts',(4.71371668583241,-117.278019107145,8.16439679231297));
#23756=CARTESIAN_POINT('Ctrl Pts',(7.07057502873392,-117.103019107145,4.082198396148));
#23757=CARTESIAN_POINT('Ctrl Pts',(9.42743337163542,-116.928019107145,-1.69756769845304E-11));
#23758=CARTESIAN_POINT('Ctrl Pts',(7.07057502871922,-116.753019107145,-4.08219839617346));
#23759=CARTESIAN_POINT('Ctrl Pts',(4.71371668580301,-116.578019107145,-8.16439679232994));
#23760=CARTESIAN_POINT('Ctrl Pts',(-1.4702867290402E-11,-116.403019107145,
-8.16439679232146));
#23761=CARTESIAN_POINT('Ctrl Pts',(-4.71371668583241,-116.228019107145,
-8.16439679231297));
#23762=CARTESIAN_POINT('Ctrl Pts',(-7.07057502873392,-116.053019107145,
-4.082198396148));
#23763=CARTESIAN_POINT('Ctrl Pts',(-9.42743337163542,-115.878019107145,
1.69768315121407E-11));
#23764=CARTESIAN_POINT('Ctrl Pts',(-7.07057502871922,-115.703019107145,
4.08219839617346));
#23765=CARTESIAN_POINT('Ctrl Pts',(-4.71371668580301,-115.528019107145,
8.16439679232994));
#23766=CARTESIAN_POINT('Ctrl Pts',(1.47018674401621E-11,-115.353019107145,
8.16439679232146));
#23767=CARTESIAN_POINT('Ctrl Pts',(4.71371668583241,-115.178019107145,8.16439679231297));
#23768=CARTESIAN_POINT('Ctrl Pts',(7.07057502873392,-115.003019107145,4.082198396148));
#23769=CARTESIAN_POINT('Ctrl Pts',(9.42743337163542,-114.828019107145,-1.69756769845304E-11));
#23770=CARTESIAN_POINT('Ctrl Pts',(7.07057502871922,-114.653019107145,-4.08219839617346));
#23771=CARTESIAN_POINT('Ctrl Pts',(4.71371668580301,-114.478019107145,-8.16439679232994));
#23772=CARTESIAN_POINT('Ctrl Pts',(-1.4702867290402E-11,-114.303019107145,
-8.16439679232146));
#23773=CARTESIAN_POINT('Ctrl Pts',(-4.71371668583241,-114.128019107145,
-8.16439679231297));
#23774=CARTESIAN_POINT('Ctrl Pts',(-7.07057502873392,-113.953019107145,
-4.082198396148));
#23775=CARTESIAN_POINT('Ctrl Pts',(-9.42743337163542,-113.778019107145,
1.69768315121407E-11));
#23776=CARTESIAN_POINT('Ctrl Pts',(-7.07057502871922,-113.603019107145,
4.08219839617346));
#23777=CARTESIAN_POINT('Ctrl Pts',(-4.71371668580301,-113.428019107145,
8.16439679232994));
#23778=CARTESIAN_POINT('Ctrl Pts',(1.47018674401621E-11,-113.253019107145,
8.16439679232146));
#23779=CARTESIAN_POINT('Ctrl Pts',(4.71371668583241,-113.078019107145,8.16439679231297));
#23780=CARTESIAN_POINT('Ctrl Pts',(7.07057502873392,-112.903019107145,4.082198396148));
#23781=CARTESIAN_POINT('Ctrl Pts',(9.42743337163542,-112.728019107145,-1.69756769845304E-11));
#23782=CARTESIAN_POINT('Ctrl Pts',(7.07057502871922,-112.553019107145,-4.08219839617346));
#23783=CARTESIAN_POINT('Ctrl Pts',(4.71371668580301,-112.378019107145,-8.16439679232994));
#23784=CARTESIAN_POINT('Ctrl Pts',(-1.4702867290402E-11,-112.203019107145,
-8.16439679232146));
#23785=CARTESIAN_POINT('Ctrl Pts',(-4.71371668583241,-112.028019107145,
-8.16439679231297));
#23786=CARTESIAN_POINT('Ctrl Pts',(-7.07057502873392,-111.853019107145,
-4.082198396148));
#23787=CARTESIAN_POINT('Ctrl Pts',(-9.42743337163542,-111.678019107145,
1.69768315121407E-11));
#23788=CARTESIAN_POINT('Ctrl Pts',(-7.07057502871922,-111.503019107145,
4.08219839617346));
#23789=CARTESIAN_POINT('Ctrl Pts',(-4.71371668580301,-111.328019107145,
8.16439679232994));
#23790=CARTESIAN_POINT('Ctrl Pts',(1.47018674401621E-11,-111.153019107145,
8.16439679232146));
#23791=CARTESIAN_POINT('Ctrl Pts',(4.71371668583241,-110.978019107145,8.16439679231297));
#23792=CARTESIAN_POINT('Ctrl Pts',(7.07057502873392,-110.803019107145,4.082198396148));
#23793=CARTESIAN_POINT('Ctrl Pts',(9.42743337163542,-110.628019107145,-1.69756769845304E-11));
#23794=CARTESIAN_POINT('Ctrl Pts',(7.07057502871922,-110.453019107145,-4.08219839617346));
#23795=CARTESIAN_POINT('Ctrl Pts',(4.71371668580301,-110.278019107145,-8.16439679232994));
#23796=CARTESIAN_POINT('Ctrl Pts',(-1.4702867290402E-11,-110.103019107145,
-8.16439679232146));
#23797=CARTESIAN_POINT('Ctrl Pts',(-4.71371668583241,-109.928019107145,
-8.16439679231297));
#23798=CARTESIAN_POINT('Ctrl Pts',(-7.07057502873392,-109.753019107145,
-4.082198396148));
#23799=CARTESIAN_POINT('Ctrl Pts',(-9.42743337163542,-109.578019107145,
1.69768315121407E-11));
#23800=CARTESIAN_POINT('Ctrl Pts',(-7.07057502871922,-109.403019107145,
4.08219839617346));
#23801=CARTESIAN_POINT('Ctrl Pts',(-4.71371668580301,-109.228019107145,
8.16439679232994));
#23802=CARTESIAN_POINT('Ctrl Pts',(1.47018674401621E-11,-109.053019107145,
8.16439679232146));
#23803=CARTESIAN_POINT('Ctrl Pts',(4.71371668583241,-108.878019107145,8.16439679231297));
#23804=CARTESIAN_POINT('Ctrl Pts',(7.07057502873392,-108.703019107145,4.082198396148));
#23805=CARTESIAN_POINT('Ctrl Pts',(9.42743337163542,-108.528019107145,-1.69756769845304E-11));
#23806=CARTESIAN_POINT('Ctrl Pts',(7.07057502871922,-108.353019107145,-4.08219839617346));
#23807=CARTESIAN_POINT('Ctrl Pts',(4.71371668580301,-108.178019107145,-8.16439679232994));
#23808=CARTESIAN_POINT('Ctrl Pts',(-1.4702867290402E-11,-108.003019107145,
-8.16439679232146));
#23809=CARTESIAN_POINT('Ctrl Pts',(-4.71371668583241,-107.828019107145,
-8.16439679231297));
#23810=CARTESIAN_POINT('Ctrl Pts',(-7.07057502873392,-107.653019107145,
-4.082198396148));
#23811=CARTESIAN_POINT('Ctrl Pts',(-9.42743337163542,-107.478019107145,
1.69768315121407E-11));
#23812=CARTESIAN_POINT('Ctrl Pts',(-7.07057502871922,-107.303019107145,
4.08219839617346));
#23813=CARTESIAN_POINT('Ctrl Pts',(-4.71371668580301,-107.128019107145,
8.16439679232994));
#23814=CARTESIAN_POINT('Ctrl Pts',(1.47018674401621E-11,-106.953019107145,
8.16439679232146));
#23815=CARTESIAN_POINT('Ctrl Pts',(4.71371668583241,-106.778019107145,8.16439679231297));
#23816=CARTESIAN_POINT('Ctrl Pts',(7.07057502873392,-106.603019107145,4.082198396148));
#23817=CARTESIAN_POINT('Ctrl Pts',(9.42743337163542,-106.428019107145,-1.69756769845304E-11));
#23818=CARTESIAN_POINT('Ctrl Pts',(7.07057502871922,-106.253019107145,-4.08219839617346));
#23819=CARTESIAN_POINT('Ctrl Pts',(4.71371668580301,-106.078019107145,-8.16439679232994));
#23820=CARTESIAN_POINT('Ctrl Pts',(-1.4702867290402E-11,-105.903019107145,
-8.16439679232146));
#23821=CARTESIAN_POINT('Ctrl Pts',(-4.71371668583241,-105.728019107145,
-8.16439679231297));
#23822=CARTESIAN_POINT('Ctrl Pts',(-7.07057502873392,-105.553019107145,
-4.082198396148));
#23823=CARTESIAN_POINT('Ctrl Pts',(-9.42743337163542,-105.378019107145,
1.69768315121407E-11));
#23824=CARTESIAN_POINT('Ctrl Pts',(-7.07057502871922,-105.203019107145,
4.08219839617346));
#23825=CARTESIAN_POINT('Ctrl Pts',(-4.71371668580301,-105.028019107145,
8.16439679232994));
#23826=CARTESIAN_POINT('Ctrl Pts',(1.47018674401621E-11,-104.853019107145,
8.16439679232146));
#23827=CARTESIAN_POINT('Ctrl Pts',(4.71371668583241,-104.678019107145,8.16439679231297));
#23828=CARTESIAN_POINT('Ctrl Pts',(7.07057502873392,-104.503019107145,4.082198396148));
#23829=CARTESIAN_POINT('Ctrl Pts',(9.42743337163542,-104.328019107145,-1.69756769845304E-11));
#23830=CARTESIAN_POINT('Ctrl Pts',(7.07057502871922,-104.153019107145,-4.08219839617346));
#23831=CARTESIAN_POINT('Ctrl Pts',(4.71371668580301,-103.978019107145,-8.16439679232994));
#23832=CARTESIAN_POINT('Ctrl Pts',(-1.4702867290402E-11,-103.803019107145,
-8.16439679232146));
#23833=CARTESIAN_POINT('Ctrl Pts',(-4.71371668583241,-103.628019107145,
-8.16439679231297));
#23834=CARTESIAN_POINT('Ctrl Pts',(-7.07057502873392,-103.453019107145,
-4.082198396148));
#23835=CARTESIAN_POINT('Ctrl Pts',(-9.42743337163542,-103.278019107145,
1.69768315121407E-11));
#23836=CARTESIAN_POINT('Ctrl Pts',(-7.07057502871922,-103.103019107145,
4.08219839617346));
#23837=CARTESIAN_POINT('Ctrl Pts',(-4.71371668580301,-102.928019107145,
8.16439679232994));
#23838=CARTESIAN_POINT('Ctrl Pts',(1.47018674401621E-11,-102.753019107145,
8.16439679232146));
#23839=CARTESIAN_POINT('Ctrl Pts',(4.71371668583241,-102.578019107145,8.16439679231297));
#23840=CARTESIAN_POINT('Ctrl Pts',(7.07057502873392,-102.403019107145,4.082198396148));
#23841=CARTESIAN_POINT('Ctrl Pts',(9.42743337163542,-102.228019107145,-1.69756769845304E-11));
#23842=CARTESIAN_POINT('Ctrl Pts',(7.07057502871922,-102.053019107145,-4.08219839617346));
#23843=CARTESIAN_POINT('Ctrl Pts',(4.71371668580301,-101.878019107145,-8.16439679232994));
#23844=CARTESIAN_POINT('Ctrl Pts',(-1.4702867290402E-11,-101.703019107145,
-8.16439679232146));
#23845=CARTESIAN_POINT('Ctrl Pts',(-4.71371668583241,-101.528019107145,
-8.16439679231297));
#23846=CARTESIAN_POINT('Ctrl Pts',(-7.07057502873392,-101.353019107145,
-4.082198396148));
#23847=CARTESIAN_POINT('Ctrl Pts',(-9.42743337163542,-101.178019107145,
1.69768315121407E-11));
#23848=CARTESIAN_POINT('Ctrl Pts',(-7.07057502871922,-101.003019107145,
4.08219839617346));
#23849=CARTESIAN_POINT('Ctrl Pts',(-4.71371668580301,-100.828019107145,
8.16439679232994));
#23850=CARTESIAN_POINT('Ctrl Pts',(1.47018674401621E-11,-100.653019107145,
8.16439679232146));
#23851=CARTESIAN_POINT('Ctrl Pts',(4.71371668583241,-100.478019107145,8.16439679231297));
#23852=CARTESIAN_POINT('Ctrl Pts',(7.07057502873392,-100.303019107145,4.082198396148));
#23853=CARTESIAN_POINT('Ctrl Pts',(9.42743337163542,-100.128019107145,-1.69756769845304E-11));
#23854=CARTESIAN_POINT('Ctrl Pts',(7.07057502871922,-99.953019107145,-4.08219839617346));
#23855=CARTESIAN_POINT('Ctrl Pts',(4.71371668580301,-99.7780191071449,-8.16439679232994));
#23856=CARTESIAN_POINT('Ctrl Pts',(-1.4702867290402E-11,-99.6030191071449,
-8.16439679232146));
#23857=CARTESIAN_POINT('Ctrl Pts',(-4.71371668583241,-99.4280191071449,
-8.16439679231297));
#23858=CARTESIAN_POINT('Ctrl Pts',(-7.07057502873392,-99.253019107145,-4.082198396148));
#23859=CARTESIAN_POINT('Ctrl Pts',(-9.42743337163542,-99.078019107145,1.69768315121407E-11));
#23860=CARTESIAN_POINT('Ctrl Pts',(-7.07057502871922,-98.903019107145,4.08219839617346));
#23861=CARTESIAN_POINT('Ctrl Pts',(-4.71371668580301,-98.7280191071449,
8.16439679232994));
#23862=CARTESIAN_POINT('Ctrl Pts',(1.47018674401621E-11,-98.5530191071449,
8.16439679232146));
#23863=CARTESIAN_POINT('Ctrl Pts',(4.71371668583241,-98.378019107145,8.16439679231297));
#23864=CARTESIAN_POINT('Ctrl Pts',(7.07057502873392,-98.2030191071449,4.082198396148));
#23865=CARTESIAN_POINT('Ctrl Pts',(9.42743337163542,-98.0280191071449,-1.69756769845304E-11));
#23866=CARTESIAN_POINT('Ctrl Pts',(7.07057502871922,-97.8530191071449,-4.08219839617346));
#23867=CARTESIAN_POINT('Ctrl Pts',(4.71371668580301,-97.6780191071449,-8.16439679232994));
#23868=CARTESIAN_POINT('Ctrl Pts',(-1.4702867290402E-11,-97.503019107145,
-8.16439679232146));
#23869=CARTESIAN_POINT('Ctrl Pts',(-4.71371668583241,-97.328019107145,-8.16439679231297));
#23870=CARTESIAN_POINT('Ctrl Pts',(-7.07057502873392,-97.153019107145,-4.082198396148));
#23871=CARTESIAN_POINT('Ctrl Pts',(-9.42743337163542,-96.978019107145,1.69768315121407E-11));
#23872=CARTESIAN_POINT('Ctrl Pts',(-7.07057502871922,-96.803019107145,4.08219839617346));
#23873=CARTESIAN_POINT('Ctrl Pts',(-4.71371668580301,-96.6280191071449,
8.16439679232994));
#23874=CARTESIAN_POINT('Ctrl Pts',(1.47018674401621E-11,-96.453019107145,
8.16439679232146));
#23875=CARTESIAN_POINT('Ctrl Pts',(4.71371668583241,-96.278019107145,8.16439679231297));
#23876=CARTESIAN_POINT('Ctrl Pts',(7.07057502873392,-96.103019107145,4.082198396148));
#23877=CARTESIAN_POINT('Ctrl Pts',(9.42743337163542,-95.928019107145,-1.69756769845304E-11));
#23878=CARTESIAN_POINT('Ctrl Pts',(7.07057502871922,-95.753019107145,-4.08219839617346));
#23879=CARTESIAN_POINT('Ctrl Pts',(4.71371668580301,-95.5780191071449,-8.16439679232994));
#23880=CARTESIAN_POINT('Ctrl Pts',(-1.4702867290402E-11,-95.403019107145,
-8.16439679232146));
#23881=CARTESIAN_POINT('Ctrl Pts',(-4.71371668583241,-95.228019107145,-8.16439679231297));
#23882=CARTESIAN_POINT('Ctrl Pts',(-7.07057502873392,-95.053019107145,-4.082198396148));
#23883=CARTESIAN_POINT('Ctrl Pts',(-9.42743337163542,-94.8780191071449,
1.69768315121407E-11));
#23884=CARTESIAN_POINT('Ctrl Pts',(-7.07057502871922,-94.703019107145,4.08219839617346));
#23885=CARTESIAN_POINT('Ctrl Pts',(-4.71371668580301,-94.528019107145,8.16439679232994));
#23886=CARTESIAN_POINT('Ctrl Pts',(1.47018674401621E-11,-94.3530191071449,
8.16439679232146));
#23887=CARTESIAN_POINT('Ctrl Pts',(4.71371668583241,-94.178019107145,8.16439679231297));
#23888=CARTESIAN_POINT('Ctrl Pts',(7.07057502873392,-94.003019107145,4.082198396148));
#23889=CARTESIAN_POINT('Ctrl Pts',(9.42743337163542,-93.8280191071449,-1.69756769845304E-11));
#23890=CARTESIAN_POINT('Ctrl Pts',(7.07057502871922,-93.6530191071449,-4.08219839617346));
#23891=CARTESIAN_POINT('Ctrl Pts',(4.71371668580301,-93.4780191071449,-8.16439679232994));
#23892=CARTESIAN_POINT('Ctrl Pts',(-1.4702867290402E-11,-93.3030191071449,
-8.16439679232146));
#23893=CARTESIAN_POINT('Ctrl Pts',(-4.71371668583241,-93.128019107145,-8.16439679231297));
#23894=CARTESIAN_POINT('Ctrl Pts',(-7.07057502873392,-92.953019107145,-4.082198396148));
#23895=CARTESIAN_POINT('Ctrl Pts',(-9.42743337163542,-92.7780191071449,
1.69768315121407E-11));
#23896=CARTESIAN_POINT('Ctrl Pts',(-7.07057502871922,-92.6030191071449,
4.08219839617346));
#23897=CARTESIAN_POINT('Ctrl Pts',(-4.71371668580301,-92.428019107145,8.16439679232994));
#23898=CARTESIAN_POINT('Ctrl Pts',(1.47018674401621E-11,-92.253019107145,
8.16439679232146));
#23899=CARTESIAN_POINT('Ctrl Pts',(4.71371668583241,-92.0780191071449,8.16439679231297));
#23900=CARTESIAN_POINT('Ctrl Pts',(7.07057502873392,-91.903019107145,4.082198396148));
#23901=CARTESIAN_POINT('Ctrl Pts',(9.42743337163542,-91.728019107145,-1.69756769845304E-11));
#23902=CARTESIAN_POINT('Ctrl Pts',(7.07057502871922,-91.553019107145,-4.08219839617346));
#23903=CARTESIAN_POINT('Ctrl Pts',(4.71371668580301,-91.378019107145,-8.16439679232994));
#23904=CARTESIAN_POINT('Ctrl Pts',(-1.4702867290402E-11,-91.203019107145,
-8.16439679232146));
#23905=CARTESIAN_POINT('Ctrl Pts',(-4.71371668583241,-91.028019107145,-8.16439679231297));
#23906=CARTESIAN_POINT('Ctrl Pts',(-7.07057502873392,-90.853019107145,-4.082198396148));
#23907=CARTESIAN_POINT('Ctrl Pts',(-9.42743337163542,-90.678019107145,1.69768315121407E-11));
#23908=CARTESIAN_POINT('Ctrl Pts',(-7.07057502871922,-90.503019107145,4.08219839617346));
#23909=CARTESIAN_POINT('Ctrl Pts',(-4.71371668580301,-90.328019107145,8.16439679232994));
#23910=CARTESIAN_POINT('Ctrl Pts',(1.47018674401621E-11,-90.153019107145,
8.16439679232146));
#23911=CARTESIAN_POINT('Ctrl Pts',(4.71371668583241,-89.978019107145,8.16439679231297));
#23912=CARTESIAN_POINT('Ctrl Pts',(7.07057502873392,-89.803019107145,4.082198396148));
#23913=CARTESIAN_POINT('Ctrl Pts',(9.42743337163542,-89.628019107145,-1.69756769845304E-11));
#23914=CARTESIAN_POINT('Ctrl Pts',(7.07057502871922,-89.4530191071449,-4.08219839617346));
#23915=CARTESIAN_POINT('Ctrl Pts',(4.71371668580301,-89.278019107145,-8.16439679232994));
#23916=CARTESIAN_POINT('Ctrl Pts',(-1.4702867290402E-11,-89.103019107145,
-8.16439679232146));
#23917=CARTESIAN_POINT('Ctrl Pts',(-4.71371668583241,-88.9280191071449,
-8.16439679231297));
#23918=CARTESIAN_POINT('Ctrl Pts',(-7.07057502873392,-88.753019107145,-4.082198396148));
#23919=CARTESIAN_POINT('Ctrl Pts',(-9.42743337163542,-88.578019107145,1.69768315121407E-11));
#23920=CARTESIAN_POINT('Ctrl Pts',(-7.07057502871922,-88.403019107145,4.08219839617346));
#23921=CARTESIAN_POINT('Ctrl Pts',(-4.71371668580301,-88.228019107145,8.16439679232994));
#23922=CARTESIAN_POINT('Ctrl Pts',(1.47018674401621E-11,-88.053019107145,
8.16439679232146));
#23923=CARTESIAN_POINT('Ctrl Pts',(4.71371668583241,-87.878019107145,8.16439679231297));
#23924=CARTESIAN_POINT('Ctrl Pts',(7.07057502873392,-87.703019107145,4.082198396148));
#23925=CARTESIAN_POINT('Ctrl Pts',(9.42743337163542,-87.528019107145,-1.69756769845304E-11));
#23926=CARTESIAN_POINT('Ctrl Pts',(7.07057502871922,-87.353019107145,-4.08219839617346));
#23927=CARTESIAN_POINT('Ctrl Pts',(4.71371668580301,-87.178019107145,-8.16439679232994));
#23928=CARTESIAN_POINT('Ctrl Pts',(-1.4702867290402E-11,-87.003019107145,
-8.16439679232146));
#23929=CARTESIAN_POINT('Ctrl Pts',(-4.71371668583241,-86.828019107145,-8.16439679231297));
#23930=CARTESIAN_POINT('Ctrl Pts',(-7.07057502873392,-86.653019107145,-4.082198396148));
#23931=CARTESIAN_POINT('Ctrl Pts',(-9.42743337163542,-86.478019107145,1.69768315121407E-11));
#23932=CARTESIAN_POINT('Ctrl Pts',(-7.07057502871922,-86.303019107145,4.08219839617346));
#23933=CARTESIAN_POINT('Ctrl Pts',(-4.71371668580301,-86.128019107145,8.16439679232994));
#23934=CARTESIAN_POINT('Ctrl Pts',(1.47018674401621E-11,-85.953019107145,
8.16439679232146));
#23935=CARTESIAN_POINT('Ctrl Pts',(4.71371668583241,-85.778019107145,8.16439679231297));
#23936=CARTESIAN_POINT('Ctrl Pts',(7.07057502873392,-85.603019107145,4.082198396148));
#23937=CARTESIAN_POINT('Ctrl Pts',(9.42743337163542,-85.428019107145,-1.69756769845304E-11));
#23938=CARTESIAN_POINT('Ctrl Pts',(7.07057502871922,-85.253019107145,-4.08219839617346));
#23939=CARTESIAN_POINT('Ctrl Pts',(4.71371668580301,-85.078019107145,-8.16439679232994));
#23940=CARTESIAN_POINT('Ctrl Pts',(-1.4702867290402E-11,-84.903019107145,
-8.16439679232146));
#23941=CARTESIAN_POINT('Ctrl Pts',(-4.71371668583241,-84.728019107145,-8.16439679231297));
#23942=CARTESIAN_POINT('Ctrl Pts',(-7.07057502873392,-84.553019107145,-4.082198396148));
#23943=CARTESIAN_POINT('Ctrl Pts',(-9.42743337163542,-84.378019107145,1.69768315121407E-11));
#23944=CARTESIAN_POINT('Ctrl Pts',(-7.07057502871922,-84.203019107145,4.08219839617346));
#23945=CARTESIAN_POINT('Ctrl Pts',(-4.71371668580301,-84.028019107145,8.16439679232994));
#23946=CARTESIAN_POINT('Ctrl Pts',(1.47018674401621E-11,-83.853019107145,
8.16439679232146));
#23947=CARTESIAN_POINT('Ctrl Pts',(4.71371668583241,-83.678019107145,8.16439679231297));
#23948=CARTESIAN_POINT('Ctrl Pts',(7.07057502873392,-83.503019107145,4.082198396148));
#23949=CARTESIAN_POINT('Ctrl Pts',(9.42743337163542,-83.328019107145,-1.69756769845304E-11));
#23950=CARTESIAN_POINT('Ctrl Pts',(7.07057502871922,-83.153019107145,-4.08219839617346));
#23951=CARTESIAN_POINT('Ctrl Pts',(4.71371668580301,-82.978019107145,-8.16439679232994));
#23952=CARTESIAN_POINT('Ctrl Pts',(-1.4702867290402E-11,-82.803019107145,
-8.16439679232146));
#23953=CARTESIAN_POINT('Ctrl Pts',(-4.71371668583241,-82.628019107145,-8.16439679231297));
#23954=CARTESIAN_POINT('Ctrl Pts',(-7.07057502873392,-82.453019107145,-4.082198396148));
#23955=CARTESIAN_POINT('Ctrl Pts',(-9.42743337163542,-82.278019107145,1.69768315121407E-11));
#23956=CARTESIAN_POINT('Ctrl Pts',(-7.07057502871922,-82.103019107145,4.08219839617346));
#23957=CARTESIAN_POINT('Ctrl Pts',(-4.71371668580301,-81.928019107145,8.16439679232994));
#23958=CARTESIAN_POINT('Ctrl Pts',(1.47018674401621E-11,-81.753019107145,
8.16439679232146));
#23959=CARTESIAN_POINT('Ctrl Pts',(4.71371668583241,-81.578019107145,8.16439679231297));
#23960=CARTESIAN_POINT('Ctrl Pts',(7.07057502873392,-81.403019107145,4.082198396148));
#23961=CARTESIAN_POINT('Ctrl Pts',(9.42743337163542,-81.228019107145,-1.69756769845304E-11));
#23962=CARTESIAN_POINT('Ctrl Pts',(7.07057502871922,-81.053019107145,-4.08219839617346));
#23963=CARTESIAN_POINT('Ctrl Pts',(4.71371668580301,-80.878019107145,-8.16439679232994));
#23964=CARTESIAN_POINT('Ctrl Pts',(-1.4702867290402E-11,-80.703019107145,
-8.16439679232146));
#23965=CARTESIAN_POINT('Ctrl Pts',(-4.71371668583241,-80.528019107145,-8.16439679231297));
#23966=CARTESIAN_POINT('Ctrl Pts',(-7.07057502873392,-80.353019107145,-4.082198396148));
#23967=CARTESIAN_POINT('Ctrl Pts',(-9.42743337163542,-80.178019107145,1.69768315121407E-11));
#23968=CARTESIAN_POINT('Ctrl Pts',(-7.07057502871922,-80.003019107145,4.08219839617346));
#23969=CARTESIAN_POINT('Ctrl Pts',(-4.71371668580301,-79.828019107145,8.16439679232994));
#23970=CARTESIAN_POINT('Ctrl Pts',(1.47018674401621E-11,-79.653019107145,
8.16439679232146));
#23971=CARTESIAN_POINT('Ctrl Pts',(4.71371668583241,-79.478019107145,8.16439679231297));
#23972=CARTESIAN_POINT('Ctrl Pts',(7.07057502873392,-79.303019107145,4.082198396148));
#23973=CARTESIAN_POINT('Ctrl Pts',(9.42743337163542,-79.128019107145,-1.69756769845304E-11));
#23974=CARTESIAN_POINT('Ctrl Pts',(7.07057502871922,-78.953019107145,-4.08219839617346));
#23975=CARTESIAN_POINT('Ctrl Pts',(4.71371668580301,-78.778019107145,-8.16439679232994));
#23976=CARTESIAN_POINT('Ctrl Pts',(-1.4702867290402E-11,-78.603019107145,
-8.16439679232146));
#23977=CARTESIAN_POINT('Ctrl Pts',(-4.71371668583241,-78.428019107145,-8.16439679231297));
#23978=CARTESIAN_POINT('Ctrl Pts',(-7.07057502873392,-78.253019107145,-4.082198396148));
#23979=CARTESIAN_POINT('Ctrl Pts',(-9.42743337163542,-78.078019107145,1.69768315121407E-11));
#23980=CARTESIAN_POINT('Ctrl Pts',(-7.07057502871922,-77.903019107145,4.08219839617346));
#23981=CARTESIAN_POINT('Ctrl Pts',(-4.71371668580301,-77.728019107145,8.16439679232994));
#23982=CARTESIAN_POINT('Ctrl Pts',(1.47018674401621E-11,-77.553019107145,
8.16439679232146));
#23983=CARTESIAN_POINT('Ctrl Pts',(4.71371668583241,-77.378019107145,8.16439679231297));
#23984=CARTESIAN_POINT('Ctrl Pts',(7.07057502873392,-77.203019107145,4.082198396148));
#23985=CARTESIAN_POINT('Ctrl Pts',(9.42743337163542,-77.028019107145,-1.69756769845304E-11));
#23986=CARTESIAN_POINT('Ctrl Pts',(7.07057502871922,-76.853019107145,-4.08219839617346));
#23987=CARTESIAN_POINT('Ctrl Pts',(4.71371668580301,-76.678019107145,-8.16439679232994));
#23988=CARTESIAN_POINT('Ctrl Pts',(-1.4702867290402E-11,-76.503019107145,
-8.16439679232146));
#23989=CARTESIAN_POINT('Ctrl Pts',(-4.71371668583241,-76.328019107145,-8.16439679231297));
#23990=CARTESIAN_POINT('Ctrl Pts',(-7.07057502873392,-76.153019107145,-4.082198396148));
#23991=CARTESIAN_POINT('Ctrl Pts',(-9.42743337163542,-75.978019107145,1.69768315121407E-11));
#23992=CARTESIAN_POINT('Ctrl Pts',(-7.07057502871922,-75.803019107145,4.08219839617346));
#23993=CARTESIAN_POINT('Ctrl Pts',(-4.71371668580301,-75.628019107145,8.16439679232994));
#23994=CARTESIAN_POINT('Ctrl Pts',(1.47018674401621E-11,-75.453019107145,
8.16439679232146));
#23995=CARTESIAN_POINT('Ctrl Pts',(4.71371668583241,-75.278019107145,8.16439679231297));
#23996=CARTESIAN_POINT('Ctrl Pts',(7.07057502873392,-75.103019107145,4.082198396148));
#23997=CARTESIAN_POINT('Ctrl Pts',(9.42743337163542,-74.928019107145,-1.69756769845304E-11));
#23998=CARTESIAN_POINT('Ctrl Pts',(7.07057502871922,-74.753019107145,-4.08219839617346));
#23999=CARTESIAN_POINT('Ctrl Pts',(4.71371668580301,-74.578019107145,-8.16439679232994));
#24000=CARTESIAN_POINT('Ctrl Pts',(-1.4702867290402E-11,-74.403019107145,
-8.16439679232146));
#24001=CARTESIAN_POINT('Ctrl Pts',(-4.71371668583241,-74.228019107145,-8.16439679231297));
#24002=CARTESIAN_POINT('Ctrl Pts',(-7.07057502873392,-74.053019107145,-4.082198396148));
#24003=CARTESIAN_POINT('Ctrl Pts',(-9.42743337163542,-73.878019107145,1.69768315121407E-11));
#24004=CARTESIAN_POINT('Ctrl Pts',(-7.07057502871922,-73.703019107145,4.08219839617346));
#24005=CARTESIAN_POINT('Ctrl Pts',(-4.71371668580301,-73.528019107145,8.16439679232994));
#24006=CARTESIAN_POINT('Ctrl Pts',(1.47018674401621E-11,-73.353019107145,
8.16439679232146));
#24007=CARTESIAN_POINT('Ctrl Pts',(4.71371668583241,-73.178019107145,8.16439679231297));
#24008=CARTESIAN_POINT('Ctrl Pts',(7.07057502873392,-73.003019107145,4.082198396148));
#24009=CARTESIAN_POINT('Ctrl Pts',(9.42743337163542,-72.828019107145,-1.69756769845304E-11));
#24010=CARTESIAN_POINT('Ctrl Pts',(7.07057502871922,-72.653019107145,-4.08219839617346));
#24011=CARTESIAN_POINT('Ctrl Pts',(4.71371668580301,-72.478019107145,-8.16439679232994));
#24012=CARTESIAN_POINT('Ctrl Pts',(-1.4702867290402E-11,-72.303019107145,
-8.16439679232146));
#24013=CARTESIAN_POINT('Ctrl Pts',(-4.71371668583241,-72.128019107145,-8.16439679231297));
#24014=CARTESIAN_POINT('Ctrl Pts',(-7.07057502873392,-71.953019107145,-4.082198396148));
#24015=CARTESIAN_POINT('Ctrl Pts',(-9.42743337163542,-71.778019107145,1.69768315121407E-11));
#24016=CARTESIAN_POINT('Ctrl Pts',(-7.07057502871922,-71.603019107145,4.08219839617346));
#24017=CARTESIAN_POINT('Ctrl Pts',(-4.71371668580301,-71.428019107145,8.16439679232994));
#24018=CARTESIAN_POINT('Ctrl Pts',(1.47018674401621E-11,-71.253019107145,
8.16439679232146));
#24019=CARTESIAN_POINT('Ctrl Pts',(4.71371668583241,-71.078019107145,8.16439679231297));
#24020=CARTESIAN_POINT('Ctrl Pts',(7.07057502873392,-70.903019107145,4.082198396148));
#24021=CARTESIAN_POINT('Ctrl Pts',(9.42743337163542,-70.728019107145,-1.69756769845304E-11));
#24022=CARTESIAN_POINT('Ctrl Pts',(7.07057502871922,-70.553019107145,-4.08219839617346));
#24023=CARTESIAN_POINT('Ctrl Pts',(4.71371668580301,-70.378019107145,-8.16439679232994));
#24024=CARTESIAN_POINT('Ctrl Pts',(-1.4702867290402E-11,-70.203019107145,
-8.16439679232146));
#24025=CARTESIAN_POINT('Ctrl Pts',(-4.71371668583241,-70.028019107145,-8.16439679231297));
#24026=CARTESIAN_POINT('Ctrl Pts',(-7.07057502873392,-69.853019107145,-4.082198396148));
#24027=CARTESIAN_POINT('Ctrl Pts',(-9.42743337163542,-69.678019107145,1.69768315121407E-11));
#24028=CARTESIAN_POINT('Ctrl Pts',(-7.07057502871922,-69.503019107145,4.08219839617346));
#24029=CARTESIAN_POINT('Ctrl Pts',(-4.71371668580301,-69.328019107145,8.16439679232994));
#24030=CARTESIAN_POINT('Ctrl Pts',(1.47018674401621E-11,-69.153019107145,
8.16439679232146));
#24031=CARTESIAN_POINT('Ctrl Pts',(4.71371668583241,-68.978019107145,8.16439679231297));
#24032=CARTESIAN_POINT('Ctrl Pts',(7.07057502873392,-68.803019107145,4.082198396148));
#24033=CARTESIAN_POINT('Ctrl Pts',(9.42743337163542,-68.6280191071451,-1.69756769845304E-11));
#24034=CARTESIAN_POINT('Ctrl Pts',(7.07057502871922,-68.453019107145,-4.08219839617346));
#24035=CARTESIAN_POINT('Ctrl Pts',(4.71371668580301,-68.278019107145,-8.16439679232994));
#24036=CARTESIAN_POINT('Ctrl Pts',(-1.4702867290402E-11,-68.103019107145,
-8.16439679232146));
#24037=CARTESIAN_POINT('Ctrl Pts',(-4.71371668583241,-67.928019107145,-8.16439679231297));
#24038=CARTESIAN_POINT('Ctrl Pts',(-7.07057502873392,-67.753019107145,-4.082198396148));
#24039=CARTESIAN_POINT('Ctrl Pts',(-9.42743337163542,-67.5780191071451,
1.69768315121407E-11));
#24040=CARTESIAN_POINT('Ctrl Pts',(-7.07057502871922,-67.403019107145,4.08219839617346));
#24041=CARTESIAN_POINT('Ctrl Pts',(-4.71371668580301,-67.228019107145,8.16439679232994));
#24042=CARTESIAN_POINT('Ctrl Pts',(1.47018674401621E-11,-67.053019107145,
8.16439679232146));
#24043=CARTESIAN_POINT('Ctrl Pts',(4.71371668583241,-66.878019107145,8.16439679231297));
#24044=CARTESIAN_POINT('Ctrl Pts',(7.07057502873392,-66.703019107145,4.082198396148));
#24045=CARTESIAN_POINT('Ctrl Pts',(9.42743337163542,-66.5280191071451,-1.69756769845304E-11));
#24046=CARTESIAN_POINT('Ctrl Pts',(7.07057502871922,-66.353019107145,-4.08219839617346));
#24047=CARTESIAN_POINT('Ctrl Pts',(4.71371668580301,-66.178019107145,-8.16439679232994));
#24048=CARTESIAN_POINT('Ctrl Pts',(-1.4702867290402E-11,-66.003019107145,
-8.16439679232146));
#24049=CARTESIAN_POINT('Ctrl Pts',(-4.71371668583241,-65.828019107145,-8.16439679231297));
#24050=CARTESIAN_POINT('Ctrl Pts',(-7.07057502873392,-65.653019107145,-4.082198396148));
#24051=CARTESIAN_POINT('Ctrl Pts',(-9.42743337163542,-65.478019107145,1.69768315121407E-11));
#24052=CARTESIAN_POINT('Ctrl Pts',(-7.07057502871922,-65.303019107145,4.08219839617346));
#24053=CARTESIAN_POINT('Ctrl Pts',(-4.71371668580301,-65.1280191071451,
8.16439679232994));
#24054=CARTESIAN_POINT('Ctrl Pts',(1.47018674401621E-11,-64.953019107145,
8.16439679232146));
#24055=CARTESIAN_POINT('Ctrl Pts',(4.71371668583241,-64.778019107145,8.16439679231297));
#24056=CARTESIAN_POINT('Ctrl Pts',(7.07057502873392,-64.603019107145,4.082198396148));
#24057=CARTESIAN_POINT('Ctrl Pts',(9.42743337163542,-64.428019107145,-1.69756769845304E-11));
#24058=CARTESIAN_POINT('Ctrl Pts',(7.07057502871922,-64.253019107145,-4.08219839617346));
#24059=CARTESIAN_POINT('Ctrl Pts',(4.71371668580301,-64.0780191071451,-8.16439679232994));
#24060=CARTESIAN_POINT('Ctrl Pts',(-1.4702867290402E-11,-63.903019107145,
-8.16439679232146));
#24061=CARTESIAN_POINT('Ctrl Pts',(-4.71371668583241,-63.728019107145,-8.16439679231297));
#24062=CARTESIAN_POINT('Ctrl Pts',(-7.07057502873392,-63.553019107145,-4.082198396148));
#24063=CARTESIAN_POINT('Ctrl Pts',(-9.42743337163542,-63.378019107145,1.69768315121407E-11));
#24064=CARTESIAN_POINT('Ctrl Pts',(-7.07057502871922,-63.203019107145,4.08219839617346));
#24065=CARTESIAN_POINT('Ctrl Pts',(-4.71371668580301,-63.028019107145,8.16439679232994));
#24066=CARTESIAN_POINT('Ctrl Pts',(1.47018674401621E-11,-62.853019107145,
8.16439679232146));
#24067=CARTESIAN_POINT('Ctrl Pts',(4.71371668583241,-62.678019107145,8.16439679231297));
#24068=CARTESIAN_POINT('Ctrl Pts',(7.07057502873392,-62.503019107145,4.082198396148));
#24069=CARTESIAN_POINT('Ctrl Pts',(9.42743337163542,-62.328019107145,-1.69756769845304E-11));
#24070=CARTESIAN_POINT('Ctrl Pts',(7.07057502871922,-62.153019107145,-4.08219839617346));
#24071=CARTESIAN_POINT('Ctrl Pts',(4.71371668580301,-61.978019107145,-8.16439679232994));
#24072=CARTESIAN_POINT('Ctrl Pts',(-1.4702867290402E-11,-61.803019107145,
-8.16439679232146));
#24073=CARTESIAN_POINT('Ctrl Pts',(-4.71371668583241,-61.628019107145,-8.16439679231297));
#24074=CARTESIAN_POINT('Ctrl Pts',(-7.07057502873392,-61.453019107145,-4.082198396148));
#24075=CARTESIAN_POINT('Ctrl Pts',(-9.42743337163542,-61.278019107145,1.69768315121407E-11));
#24076=CARTESIAN_POINT('Ctrl Pts',(-7.07057502871922,-61.103019107145,4.08219839617346));
#24077=CARTESIAN_POINT('Ctrl Pts',(-4.71371668580301,-60.9280191071451,
8.16439679232994));
#24078=CARTESIAN_POINT('Ctrl Pts',(1.47018674401621E-11,-60.753019107145,
8.16439679232146));
#24079=CARTESIAN_POINT('Ctrl Pts',(4.71371668583241,-60.578019107145,8.16439679231297));
#24080=CARTESIAN_POINT('Ctrl Pts',(7.07057502873392,-60.403019107145,4.082198396148));
#24081=CARTESIAN_POINT('Ctrl Pts',(9.42743337163542,-60.228019107145,-1.69756769845304E-11));
#24082=CARTESIAN_POINT('Ctrl Pts',(7.07057502871922,-60.053019107145,-4.08219839617346));
#24083=CARTESIAN_POINT('Ctrl Pts',(4.71371668580301,-59.8780191071451,-8.16439679232994));
#24084=CARTESIAN_POINT('Ctrl Pts',(-1.4702867290402E-11,-59.703019107145,
-8.16439679232146));
#24085=CARTESIAN_POINT('Ctrl Pts',(-4.71371668583241,-59.528019107145,-8.16439679231297));
#24086=CARTESIAN_POINT('Ctrl Pts',(-7.07057502873392,-59.3530191071451,
-4.082198396148));
#24087=CARTESIAN_POINT('Ctrl Pts',(-9.42743337163542,-59.178019107145,1.69768315121407E-11));
#24088=CARTESIAN_POINT('Ctrl Pts',(-7.07057502871922,-59.003019107145,4.08219839617346));
#24089=CARTESIAN_POINT('Ctrl Pts',(-4.71371668580301,-58.8280191071451,
8.16439679232994));
#24090=CARTESIAN_POINT('Ctrl Pts',(1.47018674401621E-11,-58.653019107145,
8.16439679232146));
#24091=CARTESIAN_POINT('Ctrl Pts',(4.71371668583241,-58.478019107145,8.16439679231297));
#24092=CARTESIAN_POINT('Ctrl Pts',(7.07057502873392,-58.303019107145,4.082198396148));
#24093=CARTESIAN_POINT('Ctrl Pts',(9.42743337163542,-58.128019107145,-1.69756769845304E-11));
#24094=CARTESIAN_POINT('Ctrl Pts',(7.07057502871922,-57.953019107145,-4.08219839617346));
#24095=CARTESIAN_POINT('Ctrl Pts',(4.71371668580301,-57.7780191071451,-8.16439679232994));
#24096=CARTESIAN_POINT('Ctrl Pts',(-1.4702867290402E-11,-57.603019107145,
-8.16439679232146));
#24097=CARTESIAN_POINT('Ctrl Pts',(-4.71371668583241,-57.428019107145,-8.16439679231297));
#24098=CARTESIAN_POINT('Ctrl Pts',(-7.07057502873392,-57.253019107145,-4.082198396148));
#24099=CARTESIAN_POINT('Ctrl Pts',(-9.42743337163542,-57.078019107145,1.69768315121407E-11));
#24100=CARTESIAN_POINT('Ctrl Pts',(-7.07057502871922,-56.903019107145,4.08219839617346));
#24101=CARTESIAN_POINT('Ctrl Pts',(-4.71371668580301,-56.728019107145,8.16439679232994));
#24102=CARTESIAN_POINT('Ctrl Pts',(1.47018674401621E-11,-56.553019107145,
8.16439679232146));
#24103=CARTESIAN_POINT('Ctrl Pts',(4.71371668583241,-56.3780191071451,8.16439679231297));
#24104=CARTESIAN_POINT('Ctrl Pts',(7.07057502873392,-56.203019107145,4.082198396148));
#24105=CARTESIAN_POINT('Ctrl Pts',(9.42743337163542,-56.028019107145,-1.69756769845304E-11));
#24106=CARTESIAN_POINT('Ctrl Pts',(7.07057502871922,-55.8530191071451,-4.08219839617346));
#24107=CARTESIAN_POINT('Ctrl Pts',(4.71371668580301,-55.678019107145,-8.16439679232994));
#24108=CARTESIAN_POINT('Ctrl Pts',(-1.4702867290402E-11,-55.503019107145,
-8.16439679232146));
#24109=CARTESIAN_POINT('Ctrl Pts',(-4.71371668583241,-55.3280191071451,
-8.16439679231297));
#24110=CARTESIAN_POINT('Ctrl Pts',(-7.07057502873392,-55.153019107145,-4.082198396148));
#24111=CARTESIAN_POINT('Ctrl Pts',(-9.42743337163542,-54.9780191071451,
1.69768315121407E-11));
#24112=CARTESIAN_POINT('Ctrl Pts',(-7.07057502871922,-54.8030191071451,
4.08219839617346));
#24113=CARTESIAN_POINT('Ctrl Pts',(-4.71371668580301,-54.628019107145,8.16439679232994));
#24114=CARTESIAN_POINT('Ctrl Pts',(1.47018674401621E-11,-54.453019107145,
8.16439679232146));
#24115=CARTESIAN_POINT('Ctrl Pts',(4.71371668583241,-54.278019107145,8.16439679231297));
#24116=CARTESIAN_POINT('Ctrl Pts',(7.07057502873392,-54.1030191071451,4.082198396148));
#24117=CARTESIAN_POINT('Ctrl Pts',(9.42743337163542,-53.9280191071451,-1.69756769845304E-11));
#24118=CARTESIAN_POINT('Ctrl Pts',(7.07057502871922,-53.7530191071451,-4.08219839617346));
#24119=CARTESIAN_POINT('Ctrl Pts',(4.71371668580301,-53.5780191071451,-8.16439679232994));
#24120=CARTESIAN_POINT('Ctrl Pts',(-1.4702867290402E-11,-53.403019107145,
-8.16439679232146));
#24121=CARTESIAN_POINT('Ctrl Pts',(-4.71371668583241,-53.228019107145,-8.16439679231297));
#24122=CARTESIAN_POINT('Ctrl Pts',(-7.07057502873392,-53.0530191071451,
-4.082198396148));
#24123=CARTESIAN_POINT('Ctrl Pts',(-9.42743337163542,-52.878019107145,1.69768315121407E-11));
#24124=CARTESIAN_POINT('Ctrl Pts',(-7.07057502871922,-52.703019107145,4.08219839617346));
#24125=CARTESIAN_POINT('Ctrl Pts',(-4.71371668580301,-52.528019107145,8.16439679232994));
#24126=CARTESIAN_POINT('Ctrl Pts',(1.47018674401621E-11,-52.3530191071451,
8.16439679232146));
#24127=CARTESIAN_POINT('Ctrl Pts',(4.71371668583241,-52.178019107145,8.16439679231297));
#24128=CARTESIAN_POINT('Ctrl Pts',(7.07057502873392,-52.0030191071451,4.082198396148));
#24129=CARTESIAN_POINT('Ctrl Pts',(9.42743337163542,-51.828019107145,-1.69756769845304E-11));
#24130=CARTESIAN_POINT('Ctrl Pts',(7.07057502871922,-51.6530191071451,-4.08219839617346));
#24131=CARTESIAN_POINT('Ctrl Pts',(4.71371668580301,-51.4780191071451,-8.16439679232994));
#24132=CARTESIAN_POINT('Ctrl Pts',(-1.4702867290402E-11,-51.303019107145,
-8.16439679232146));
#24133=CARTESIAN_POINT('Ctrl Pts',(-4.71371668583241,-51.1280191071451,
-8.16439679231297));
#24134=CARTESIAN_POINT('Ctrl Pts',(-7.07057502873392,-50.9530191071451,
-4.082198396148));
#24135=CARTESIAN_POINT('Ctrl Pts',(-9.42743337163542,-50.778019107145,1.69768315121407E-11));
#24136=CARTESIAN_POINT('Ctrl Pts',(-7.07057502871922,-50.6030191071451,
4.08219839617346));
#24137=CARTESIAN_POINT('Ctrl Pts',(-4.71371668580301,-50.4280191071451,
8.16439679232994));
#24138=CARTESIAN_POINT('Ctrl Pts',(1.47018674401621E-11,-50.253019107145,
8.16439679232146));
#24139=CARTESIAN_POINT('Ctrl Pts',(4.71371668583241,-50.0780191071451,8.16439679231297));
#24140=CARTESIAN_POINT('Ctrl Pts',(7.07057502873392,-49.9030191071451,4.082198396148));
#24141=CARTESIAN_POINT('Ctrl Pts',(9.42743337163542,-49.728019107145,-1.69756769845304E-11));
#24142=CARTESIAN_POINT('Ctrl Pts',(7.07057502871922,-49.5530191071451,-4.08219839617346));
#24143=CARTESIAN_POINT('Ctrl Pts',(4.71371668580301,-49.3780191071451,-8.16439679232994));
#24144=CARTESIAN_POINT('Ctrl Pts',(-1.4702867290402E-11,-49.2030191071451,
-8.16439679232146));
#24145=CARTESIAN_POINT('Ctrl Pts',(-4.71371668583241,-49.028019107145,-8.16439679231297));
#24146=CARTESIAN_POINT('Ctrl Pts',(-7.07057502873392,-48.853019107145,-4.082198396148));
#24147=CARTESIAN_POINT('Ctrl Pts',(-9.42743337163542,-48.6780191071451,
1.69768315121407E-11));
#24148=CARTESIAN_POINT('Ctrl Pts',(-7.07057502871922,-48.5030191071451,
4.08219839617346));
#24149=CARTESIAN_POINT('Ctrl Pts',(-4.71371668580301,-48.3280191071451,
8.16439679232994));
#24150=CARTESIAN_POINT('Ctrl Pts',(1.47018674401621E-11,-48.1530191071451,
8.16439679232146));
#24151=CARTESIAN_POINT('Ctrl Pts',(4.71371668583241,-47.9780191071451,8.16439679231297));
#24152=CARTESIAN_POINT('Ctrl Pts',(7.07057502873392,-47.8030191071451,4.082198396148));
#24153=CARTESIAN_POINT('Ctrl Pts',(9.42743337163542,-47.6280191071451,-1.69756769845304E-11));
#24154=CARTESIAN_POINT('Ctrl Pts',(7.07057502871922,-47.4530191071451,-4.08219839617346));
#24155=CARTESIAN_POINT('Ctrl Pts',(4.71371668580301,-47.2780191071451,-8.16439679232994));
#24156=CARTESIAN_POINT('Ctrl Pts',(-1.4702867290402E-11,-47.1030191071451,
-8.16439679232146));
#24157=CARTESIAN_POINT('Ctrl Pts',(-4.71371668583241,-46.9280191071451,
-8.16439679231297));
#24158=CARTESIAN_POINT('Ctrl Pts',(-7.07057502873392,-46.7530191071451,
-4.082198396148));
#24159=CARTESIAN_POINT('Ctrl Pts',(-9.42743337163542,-46.5780191071451,
1.69768315121407E-11));
#24160=CARTESIAN_POINT('Ctrl Pts',(-7.07057502871922,-46.4030191071451,
4.08219839617346));
#24161=CARTESIAN_POINT('Ctrl Pts',(-4.71371668580301,-46.2280191071451,
8.16439679232994));
#24162=CARTESIAN_POINT('Ctrl Pts',(1.47018674401621E-11,-46.0530191071451,
8.16439679232146));
#24163=CARTESIAN_POINT('Ctrl Pts',(4.71371668583241,-45.8780191071451,8.16439679231297));
#24164=CARTESIAN_POINT('Ctrl Pts',(7.07057502873392,-45.7030191071451,4.082198396148));
#24165=CARTESIAN_POINT('Ctrl Pts',(9.42743337163542,-45.5280191071451,-1.69756769845304E-11));
#24166=CARTESIAN_POINT('Ctrl Pts',(7.07057502871922,-45.3530191071451,-4.08219839617346));
#24167=CARTESIAN_POINT('Ctrl Pts',(4.71371668580301,-45.1780191071451,-8.16439679232994));
#24168=CARTESIAN_POINT('Ctrl Pts',(-1.4702867290402E-11,-45.0030191071451,
-8.16439679232146));
#24169=CARTESIAN_POINT('Ctrl Pts',(-4.71371668583241,-44.8280191071451,
-8.16439679231297));
#24170=CARTESIAN_POINT('Ctrl Pts',(-7.07057502873392,-44.6530191071451,
-4.082198396148));
#24171=CARTESIAN_POINT('Ctrl Pts',(-9.42743337163542,-44.4780191071451,
1.69768315121407E-11));
#24172=CARTESIAN_POINT('Ctrl Pts',(-7.07057502871922,-44.3030191071451,
4.08219839617346));
#24173=CARTESIAN_POINT('Ctrl Pts',(-4.71371668580301,-44.1280191071451,
8.16439679232994));
#24174=CARTESIAN_POINT('Ctrl Pts',(1.47018674401621E-11,-43.9530191071451,
8.16439679232146));
#24175=CARTESIAN_POINT('Ctrl Pts',(4.71371668583241,-43.7780191071451,8.16439679231297));
#24176=CARTESIAN_POINT('Ctrl Pts',(7.07057502873392,-43.6030191071451,4.082198396148));
#24177=CARTESIAN_POINT('Ctrl Pts',(9.42743337163542,-43.4280191071451,-1.69756769845304E-11));
#24178=CARTESIAN_POINT('Ctrl Pts',(7.07057502871922,-43.2530191071451,-4.08219839617346));
#24179=CARTESIAN_POINT('Ctrl Pts',(4.71371668580301,-43.0780191071451,-8.16439679232994));
#24180=CARTESIAN_POINT('Ctrl Pts',(-1.4702867290402E-11,-42.9030191071451,
-8.16439679232146));
#24181=CARTESIAN_POINT('Ctrl Pts',(-4.71371668583241,-42.7280191071451,
-8.16439679231297));
#24182=CARTESIAN_POINT('Ctrl Pts',(-7.07057502873392,-42.5530191071451,
-4.082198396148));
#24183=CARTESIAN_POINT('Ctrl Pts',(-9.42743337163542,-42.3780191071451,
1.69768315121407E-11));
#24184=CARTESIAN_POINT('Ctrl Pts',(-7.07057502871922,-42.2030191071451,
4.08219839617346));
#24185=CARTESIAN_POINT('Ctrl Pts',(-4.71371668580301,-42.0280191071451,
8.16439679232994));
#24186=CARTESIAN_POINT('Ctrl Pts',(1.47018674401621E-11,-41.8530191071451,
8.16439679232146));
#24187=CARTESIAN_POINT('Ctrl Pts',(4.71371668583241,-41.6780191071451,8.16439679231297));
#24188=CARTESIAN_POINT('Ctrl Pts',(7.07057502873392,-41.5030191071451,4.082198396148));
#24189=CARTESIAN_POINT('Ctrl Pts',(9.42743337163542,-41.3280191071451,-1.69756769845304E-11));
#24190=CARTESIAN_POINT('Ctrl Pts',(7.07057502871922,-41.1530191071451,-4.08219839617346));
#24191=CARTESIAN_POINT('Ctrl Pts',(4.71371668580301,-40.9780191071451,-8.16439679232994));
#24192=CARTESIAN_POINT('Ctrl Pts',(-1.4702867290402E-11,-40.8030191071451,
-8.16439679232146));
#24193=CARTESIAN_POINT('Ctrl Pts',(-4.71371668583241,-40.6280191071451,
-8.16439679231297));
#24194=CARTESIAN_POINT('Ctrl Pts',(-7.07057502873392,-40.4530191071451,
-4.082198396148));
#24195=CARTESIAN_POINT('Ctrl Pts',(-9.42743337163542,-40.2780191071451,
1.69768315121407E-11));
#24196=CARTESIAN_POINT('Ctrl Pts',(-7.07057502871922,-40.1030191071451,
4.08219839617346));
#24197=CARTESIAN_POINT('Ctrl Pts',(-4.71371668580301,-39.9280191071451,
8.16439679232994));
#24198=CARTESIAN_POINT('Ctrl Pts',(1.47018674401621E-11,-39.7530191071451,
8.16439679232146));
#24199=CARTESIAN_POINT('Ctrl Pts',(4.71371668583241,-39.5780191071451,8.16439679231297));
#24200=CARTESIAN_POINT('Ctrl Pts',(7.07057502873392,-39.4030191071451,4.082198396148));
#24201=CARTESIAN_POINT('Ctrl Pts',(9.42743337163542,-39.2280191071451,-1.69756769845304E-11));
#24202=CARTESIAN_POINT('Ctrl Pts',(7.07057502871922,-39.0530191071451,-4.08219839617346));
#24203=CARTESIAN_POINT('Ctrl Pts',(4.71371668580301,-38.8780191071451,-8.16439679232994));
#24204=CARTESIAN_POINT('Ctrl Pts',(-1.4702867290402E-11,-38.7030191071451,
-8.16439679232146));
#24205=CARTESIAN_POINT('Ctrl Pts',(-4.71371668583241,-38.5280191071451,
-8.16439679231297));
#24206=CARTESIAN_POINT('Ctrl Pts',(-7.07057502873392,-38.3530191071451,
-4.082198396148));
#24207=CARTESIAN_POINT('Ctrl Pts',(-9.42743337163542,-38.1780191071451,
1.69768315121407E-11));
#24208=CARTESIAN_POINT('Ctrl Pts',(-7.07057502871922,-38.0030191071451,
4.08219839617346));
#24209=CARTESIAN_POINT('Ctrl Pts',(-4.71371668580301,-37.8280191071451,
8.16439679232994));
#24210=CARTESIAN_POINT('Ctrl Pts',(1.47018674401621E-11,-37.6530191071451,
8.16439679232146));
#24211=CARTESIAN_POINT('Ctrl Pts',(4.71371668583241,-37.4780191071451,8.16439679231297));
#24212=CARTESIAN_POINT('Ctrl Pts',(7.07057502873392,-37.3030191071451,4.082198396148));
#24213=CARTESIAN_POINT('Ctrl Pts',(9.42743337163542,-37.1280191071451,-1.69756769845304E-11));
#24214=CARTESIAN_POINT('Ctrl Pts',(7.07057502871922,-36.9530191071451,-4.08219839617346));
#24215=CARTESIAN_POINT('Ctrl Pts',(4.71371668580301,-36.7780191071451,-8.16439679232994));
#24216=CARTESIAN_POINT('Ctrl Pts',(-1.4702867290402E-11,-36.6030191071451,
-8.16439679232146));
#24217=CARTESIAN_POINT('Ctrl Pts',(-4.71371668583241,-36.4280191071451,
-8.16439679231297));
#24218=CARTESIAN_POINT('Ctrl Pts',(-7.07057502873392,-36.2530191071451,
-4.082198396148));
#24219=CARTESIAN_POINT('Ctrl Pts',(-9.42743337163542,-36.0780191071451,
1.69768315121407E-11));
#24220=CARTESIAN_POINT('Ctrl Pts',(-7.07057502871922,-35.9030191071451,
4.08219839617346));
#24221=CARTESIAN_POINT('Ctrl Pts',(-4.71371668580301,-35.7280191071451,
8.16439679232994));
#24222=CARTESIAN_POINT('Ctrl Pts',(1.47018674401621E-11,-35.5530191071451,
8.16439679232146));
#24223=CARTESIAN_POINT('Ctrl Pts',(4.71371668583241,-35.3780191071451,8.16439679231297));
#24224=CARTESIAN_POINT('Ctrl Pts',(7.07057502873392,-35.2030191071451,4.082198396148));
#24225=CARTESIAN_POINT('Ctrl Pts',(9.42743337163542,-35.0280191071451,-1.69756769845304E-11));
#24226=CARTESIAN_POINT('Ctrl Pts',(7.07057502871922,-34.8530191071451,-4.08219839617346));
#24227=CARTESIAN_POINT('Ctrl Pts',(4.71371668580301,-34.6780191071451,-8.16439679232994));
#24228=CARTESIAN_POINT('Ctrl Pts',(-1.4702867290402E-11,-34.5030191071451,
-8.16439679232146));
#24229=CARTESIAN_POINT('Ctrl Pts',(-4.71371668583241,-34.3280191071451,
-8.16439679231297));
#24230=CARTESIAN_POINT('Ctrl Pts',(-7.07057502873392,-34.1530191071451,
-4.082198396148));
#24231=CARTESIAN_POINT('Ctrl Pts',(-9.42743337163542,-33.9780191071451,
1.69768315121407E-11));
#24232=CARTESIAN_POINT('Ctrl Pts',(-7.07057502871922,-33.8030191071451,
4.08219839617346));
#24233=CARTESIAN_POINT('Ctrl Pts',(-4.71371668580301,-33.6280191071451,
8.16439679232994));
#24234=CARTESIAN_POINT('Ctrl Pts',(1.47018674401621E-11,-33.4530191071451,
8.16439679232146));
#24235=CARTESIAN_POINT('Ctrl Pts',(4.71371668583241,-33.2780191071451,8.16439679231297));
#24236=CARTESIAN_POINT('Ctrl Pts',(7.07057502873392,-33.1030191071451,4.082198396148));
#24237=CARTESIAN_POINT('Ctrl Pts',(9.42743337163542,-32.9280191071451,-1.69756769845304E-11));
#24238=CARTESIAN_POINT('Ctrl Pts',(7.07057502871922,-32.7530191071451,-4.08219839617346));
#24239=CARTESIAN_POINT('Ctrl Pts',(4.71371668580301,-32.5780191071451,-8.16439679232994));
#24240=CARTESIAN_POINT('Ctrl Pts',(-1.4702867290402E-11,-32.4030191071451,
-8.16439679232146));
#24241=CARTESIAN_POINT('Ctrl Pts',(-4.71371668583241,-32.2280191071451,
-8.16439679231297));
#24242=CARTESIAN_POINT('Ctrl Pts',(-7.07057502873392,-32.0530191071451,
-4.082198396148));
#24243=CARTESIAN_POINT('Ctrl Pts',(-9.42743337163542,-31.8780191071451,
1.69768315121407E-11));
#24244=CARTESIAN_POINT('Ctrl Pts',(-7.07057502871922,-31.7030191071451,
4.08219839617346));
#24245=CARTESIAN_POINT('Ctrl Pts',(-4.71371668580301,-31.5280191071451,
8.16439679232994));
#24246=CARTESIAN_POINT('Ctrl Pts',(1.47018674401621E-11,-31.3530191071451,
8.16439679232146));
#24247=CARTESIAN_POINT('Ctrl Pts',(4.71371668583241,-31.1780191071451,8.16439679231297));
#24248=CARTESIAN_POINT('Ctrl Pts',(7.07057502873392,-31.0030191071451,4.082198396148));
#24249=CARTESIAN_POINT('Ctrl Pts',(9.42743337163542,-30.8280191071451,-1.69756769845304E-11));
#24250=CARTESIAN_POINT('Ctrl Pts',(7.07057502871922,-30.6530191071451,-4.08219839617346));
#24251=CARTESIAN_POINT('Ctrl Pts',(4.71371668580301,-30.4780191071451,-8.16439679232994));
#24252=CARTESIAN_POINT('Ctrl Pts',(-1.4702867290402E-11,-30.3030191071451,
-8.16439679232146));
#24253=CARTESIAN_POINT('Ctrl Pts',(-4.71371668583241,-30.1280191071451,
-8.16439679231297));
#24254=CARTESIAN_POINT('Ctrl Pts',(-7.07057502873392,-29.9530191071451,
-4.082198396148));
#24255=CARTESIAN_POINT('Ctrl Pts',(-9.42743337163542,-29.7780191071451,
1.69768315121407E-11));
#24256=CARTESIAN_POINT('Ctrl Pts',(-7.07057502871922,-29.6030191071451,
4.08219839617346));
#24257=CARTESIAN_POINT('Ctrl Pts',(-4.71371668580301,-29.4280191071451,
8.16439679232994));
#24258=CARTESIAN_POINT('Ctrl Pts',(1.47018674401621E-11,-29.2530191071451,
8.16439679232146));
#24259=CARTESIAN_POINT('Ctrl Pts',(4.71371668583241,-29.0780191071451,8.16439679231297));
#24260=CARTESIAN_POINT('Ctrl Pts',(7.07057502873392,-28.9030191071451,4.082198396148));
#24261=CARTESIAN_POINT('Ctrl Pts',(9.42743337163542,-28.7280191071451,-1.69756769845304E-11));
#24262=CARTESIAN_POINT('Ctrl Pts',(7.07057502871922,-28.5530191071451,-4.08219839617346));
#24263=CARTESIAN_POINT('Ctrl Pts',(4.71371668580301,-28.3780191071451,-8.16439679232994));
#24264=CARTESIAN_POINT('Ctrl Pts',(-1.4702867290402E-11,-28.2030191071451,
-8.16439679232146));
#24265=CARTESIAN_POINT('Ctrl Pts',(-4.71371668583241,-28.0280191071451,
-8.16439679231297));
#24266=CARTESIAN_POINT('Ctrl Pts',(-7.07057502873392,-27.8530191071451,
-4.082198396148));
#24267=CARTESIAN_POINT('Ctrl Pts',(-9.42743337163542,-27.6780191071451,
1.69768315121407E-11));
#24268=CARTESIAN_POINT('Ctrl Pts',(-7.07057502871922,-27.5030191071451,
4.08219839617346));
#24269=CARTESIAN_POINT('Ctrl Pts',(-4.71371668580301,-27.3280191071451,
8.16439679232994));
#24270=CARTESIAN_POINT('Ctrl Pts',(1.47018674401621E-11,-27.1530191071451,
8.16439679232146));
#24271=CARTESIAN_POINT('Ctrl Pts',(4.71371668583241,-26.9780191071451,8.16439679231297));
#24272=CARTESIAN_POINT('Ctrl Pts',(7.07057502873392,-26.8030191071451,4.082198396148));
#24273=CARTESIAN_POINT('Ctrl Pts',(9.42743337163542,-26.6280191071451,-1.69756769845304E-11));
#24274=CARTESIAN_POINT('Ctrl Pts',(7.07057502871922,-26.4530191071451,-4.08219839617346));
#24275=CARTESIAN_POINT('Ctrl Pts',(4.71371668580301,-26.2780191071451,-8.16439679232994));
#24276=CARTESIAN_POINT('Ctrl Pts',(-1.4702867290402E-11,-26.1030191071451,
-8.16439679232146));
#24277=CARTESIAN_POINT('Ctrl Pts',(-4.71371668583241,-25.9280191071451,
-8.16439679231297));
#24278=CARTESIAN_POINT('Ctrl Pts',(-7.07057502873392,-25.7530191071451,
-4.082198396148));
#24279=CARTESIAN_POINT('Ctrl Pts',(-9.42743337163542,-25.5780191071451,
1.69768315121407E-11));
#24280=CARTESIAN_POINT('Ctrl Pts',(-7.07057502871922,-25.4030191071451,
4.08219839617346));
#24281=CARTESIAN_POINT('Ctrl Pts',(-4.71371668580301,-25.2280191071451,
8.16439679232994));
#24282=CARTESIAN_POINT('Ctrl Pts',(1.47018674401621E-11,-25.0530191071451,
8.16439679232146));
#24283=CARTESIAN_POINT('Ctrl Pts',(4.71371668583241,-24.8780191071451,8.16439679231297));
#24284=CARTESIAN_POINT('Ctrl Pts',(7.07057502873392,-24.7030191071451,4.082198396148));
#24285=CARTESIAN_POINT('Ctrl Pts',(9.42743337163542,-24.5280191071451,-1.69756769845304E-11));
#24286=CARTESIAN_POINT('Ctrl Pts',(7.07057502871922,-24.3530191071451,-4.08219839617346));
#24287=CARTESIAN_POINT('Ctrl Pts',(4.71371668580301,-24.1780191071451,-8.16439679232994));
#24288=CARTESIAN_POINT('Ctrl Pts',(-1.4702867290402E-11,-24.0030191071451,
-8.16439679232146));
#24289=CARTESIAN_POINT('Ctrl Pts',(-4.71371668583241,-23.8280191071451,
-8.16439679231297));
#24290=CARTESIAN_POINT('Ctrl Pts',(-7.07057502873392,-23.6530191071451,
-4.082198396148));
#24291=CARTESIAN_POINT('Ctrl Pts',(-9.42743337163542,-23.4780191071451,
1.69768315121407E-11));
#24292=CARTESIAN_POINT('Ctrl Pts',(-7.07057502871922,-23.3030191071451,
4.08219839617346));
#24293=CARTESIAN_POINT('Ctrl Pts',(-4.71371668580301,-23.1280191071451,
8.16439679232994));
#24294=CARTESIAN_POINT('Ctrl Pts',(1.47018674401621E-11,-22.9530191071451,
8.16439679232146));
#24295=CARTESIAN_POINT('Ctrl Pts',(4.71371668583241,-22.7780191071451,8.16439679231297));
#24296=CARTESIAN_POINT('Ctrl Pts',(7.07057502873392,-22.6030191071451,4.082198396148));
#24297=CARTESIAN_POINT('Ctrl Pts',(9.42743337163542,-22.4280191071451,-1.69756769845304E-11));
#24298=CARTESIAN_POINT('Ctrl Pts',(7.07057502871922,-22.2530191071451,-4.08219839617346));
#24299=CARTESIAN_POINT('Ctrl Pts',(4.71371668580301,-22.0780191071451,-8.16439679232994));
#24300=CARTESIAN_POINT('Ctrl Pts',(-1.4702867290402E-11,-21.9030191071451,
-8.16439679232146));
#24301=CARTESIAN_POINT('Ctrl Pts',(-4.71371668583241,-21.7280191071451,
-8.16439679231297));
#24302=CARTESIAN_POINT('Ctrl Pts',(-7.07057502873392,-21.5530191071451,
-4.082198396148));
#24303=CARTESIAN_POINT('Ctrl Pts',(-9.42743337163542,-21.3780191071451,
1.69768315121407E-11));
#24304=CARTESIAN_POINT('Ctrl Pts',(-7.07057502871922,-21.2030191071451,
4.08219839617346));
#24305=CARTESIAN_POINT('Ctrl Pts',(-4.71371668580301,-21.0280191071451,
8.16439679232994));
#24306=CARTESIAN_POINT('Ctrl Pts',(1.47018674401621E-11,-20.8530191071451,
8.16439679232146));
#24307=CARTESIAN_POINT('Ctrl Pts',(4.71371668583241,-20.6780191071451,8.16439679231297));
#24308=CARTESIAN_POINT('Ctrl Pts',(7.07057502873392,-20.5030191071451,4.082198396148));
#24309=CARTESIAN_POINT('Ctrl Pts',(9.42743337163542,-20.3280191071451,-1.69756769845304E-11));
#24310=CARTESIAN_POINT('Ctrl Pts',(7.07057502871922,-20.1530191071451,-4.08219839617346));
#24311=CARTESIAN_POINT('Ctrl Pts',(4.71371668580301,-19.9780191071451,-8.16439679232994));
#24312=CARTESIAN_POINT('Ctrl Pts',(-1.4702867290402E-11,-19.8030191071451,
-8.16439679232146));
#24313=CARTESIAN_POINT('Ctrl Pts',(-4.71371668583241,-19.6280191071451,
-8.16439679231297));
#24314=CARTESIAN_POINT('Ctrl Pts',(-7.07057502873392,-19.4530191071451,
-4.082198396148));
#24315=CARTESIAN_POINT('Ctrl Pts',(-9.42743337163542,-19.2780191071451,
1.69768315121407E-11));
#24316=CARTESIAN_POINT('Ctrl Pts',(-7.07057502871922,-19.1030191071451,
4.08219839617346));
#24317=CARTESIAN_POINT('Ctrl Pts',(-4.71371668580301,-18.9280191071451,
8.16439679232994));
#24318=CARTESIAN_POINT('Ctrl Pts',(1.47018674401621E-11,-18.7530191071451,
8.16439679232146));
#24319=CARTESIAN_POINT('Ctrl Pts',(4.71371668583241,-18.5780191071451,8.16439679231297));
#24320=CARTESIAN_POINT('Ctrl Pts',(7.07057502873392,-18.4030191071451,4.082198396148));
#24321=CARTESIAN_POINT('Ctrl Pts',(9.42743337163542,-18.2280191071451,-1.69756769845304E-11));
#24322=CARTESIAN_POINT('Ctrl Pts',(7.07057502871922,-18.0530191071451,-4.08219839617346));
#24323=CARTESIAN_POINT('Ctrl Pts',(4.71371668580301,-17.8780191071451,-8.16439679232994));
#24324=CARTESIAN_POINT('Ctrl Pts',(-1.4702867290402E-11,-17.7030191071451,
-8.16439679232146));
#24325=CARTESIAN_POINT('Ctrl Pts',(-4.71371668583241,-17.5280191071451,
-8.16439679231297));
#24326=CARTESIAN_POINT('Ctrl Pts',(-7.07057502873392,-17.3530191071451,
-4.082198396148));
#24327=CARTESIAN_POINT('Ctrl Pts',(-9.42743337163542,-17.1780191071451,
1.69768315121407E-11));
#24328=CARTESIAN_POINT('Ctrl Pts',(-7.07057502871922,-17.0030191071451,
4.08219839617346));
#24329=CARTESIAN_POINT('Ctrl Pts',(-4.71371668580301,-16.8280191071451,
8.16439679232994));
#24330=CARTESIAN_POINT('Ctrl Pts',(1.47018674401621E-11,-16.6530191071451,
8.16439679232146));
#24331=CARTESIAN_POINT('Ctrl Pts',(4.71371668583241,-16.4780191071451,8.16439679231297));
#24332=CARTESIAN_POINT('Ctrl Pts',(7.07057502873392,-16.3030191071451,4.082198396148));
#24333=CARTESIAN_POINT('Ctrl Pts',(9.42743337163542,-16.1280191071451,-1.69756769845304E-11));
#24334=CARTESIAN_POINT('Ctrl Pts',(7.07057502871922,-15.9530191071451,-4.08219839617346));
#24335=CARTESIAN_POINT('Ctrl Pts',(4.71371668580301,-15.7780191071451,-8.16439679232994));
#24336=CARTESIAN_POINT('Ctrl Pts',(-1.4702867290402E-11,-15.6030191071451,
-8.16439679232146));
#24337=CARTESIAN_POINT('Ctrl Pts',(-4.71371668583241,-15.4280191071451,
-8.16439679231297));
#24338=CARTESIAN_POINT('Ctrl Pts',(-7.07057502873392,-15.2530191071451,
-4.082198396148));
#24339=CARTESIAN_POINT('Ctrl Pts',(-9.42743337163542,-15.0780191071451,
1.69768315121407E-11));
#24340=CARTESIAN_POINT('Ctrl Pts',(-7.07057502871922,-14.9030191071451,
4.08219839617346));
#24341=CARTESIAN_POINT('Ctrl Pts',(-4.71371668580301,-14.7280191071451,
8.16439679232994));
#24342=CARTESIAN_POINT('Ctrl Pts',(1.47018674401621E-11,-14.5530191071451,
8.16439679232146));
#24343=CARTESIAN_POINT('Ctrl Pts',(4.71371668583241,-14.3780191071451,8.16439679231297));
#24344=CARTESIAN_POINT('Ctrl Pts',(7.07057502873392,-14.2030191071451,4.082198396148));
#24345=CARTESIAN_POINT('Ctrl Pts',(9.42743337163542,-14.0280191071451,-1.69756769845304E-11));
#24346=CARTESIAN_POINT('Ctrl Pts',(7.07057502871922,-13.8530191071451,-4.08219839617346));
#24347=CARTESIAN_POINT('Ctrl Pts',(4.71371668580301,-13.6780191071451,-8.16439679232994));
#24348=CARTESIAN_POINT('Ctrl Pts',(-1.4702867290402E-11,-13.5030191071451,
-8.16439679232146));
#24349=CARTESIAN_POINT('Ctrl Pts',(-4.71371668583241,-13.3280191071452,
-8.16439679231297));
#24350=CARTESIAN_POINT('Ctrl Pts',(-7.07057502873392,-13.1530191071451,
-4.082198396148));
#24351=CARTESIAN_POINT('Ctrl Pts',(-9.42743337163542,-12.9780191071451,
1.69768315121407E-11));
#24352=CARTESIAN_POINT('Ctrl Pts',(-7.07057502871922,-12.8030191071452,
4.08219839617346));
#24353=CARTESIAN_POINT('Ctrl Pts',(-4.71371668580301,-12.6280191071451,
8.16439679232994));
#24354=CARTESIAN_POINT('Ctrl Pts',(1.47018674401621E-11,-12.4530191071451,
8.16439679232146));
#24355=CARTESIAN_POINT('Ctrl Pts',(4.71371668583241,-12.2780191071452,8.16439679231297));
#24356=CARTESIAN_POINT('Ctrl Pts',(7.07057502873392,-12.1030191071451,4.082198396148));
#24357=CARTESIAN_POINT('Ctrl Pts',(9.42743337163542,-11.9280191071451,-1.69756769845304E-11));
#24358=CARTESIAN_POINT('Ctrl Pts',(7.07057502871922,-11.7530191071452,-4.08219839617346));
#24359=CARTESIAN_POINT('Ctrl Pts',(4.71371668580301,-11.5780191071452,-8.16439679232994));
#24360=CARTESIAN_POINT('Ctrl Pts',(-1.4702867290402E-11,-11.4030191071451,
-8.16439679232146));
#24361=CARTESIAN_POINT('Ctrl Pts',(-4.71371668583241,-11.2280191071451,
-8.16439679231297));
#24362=CARTESIAN_POINT('Ctrl Pts',(-7.07057502873392,-11.0530191071452,
-4.082198396148));
#24363=CARTESIAN_POINT('Ctrl Pts',(-9.42743337163542,-10.8780191071451,
1.69768315121407E-11));
#24364=CARTESIAN_POINT('Ctrl Pts',(-7.07057502871922,-10.7030191071451,
4.08219839617346));
#24365=CARTESIAN_POINT('Ctrl Pts',(-4.71371668580301,-10.5280191071452,
8.16439679232994));
#24366=CARTESIAN_POINT('Ctrl Pts',(1.47018674401621E-11,-10.3530191071451,
8.16439679232146));
#24367=CARTESIAN_POINT('Ctrl Pts',(4.71371668583241,-10.1780191071451,8.16439679231297));
#24368=CARTESIAN_POINT('Ctrl Pts',(7.07057502873392,-10.0030191071452,4.082198396148));
#24369=CARTESIAN_POINT('Ctrl Pts',(9.42743337163542,-9.82801910714514,-1.69756769845304E-11));
#24370=CARTESIAN_POINT('Ctrl Pts',(7.07057502871922,-9.65301910714514,-4.08219839617346));
#24371=CARTESIAN_POINT('Ctrl Pts',(4.71371668580301,-9.47801910714516,-8.16439679232994));
#24372=CARTESIAN_POINT('Ctrl Pts',(-1.4702867290402E-11,-9.30301910714514,
-8.16439679232146));
#24373=CARTESIAN_POINT('Ctrl Pts',(-4.71371668583241,-9.12801910714515,
-8.16439679231297));
#24374=CARTESIAN_POINT('Ctrl Pts',(-7.07057502873392,-8.95301910714516,
-4.082198396148));
#24375=CARTESIAN_POINT('Ctrl Pts',(-9.42743337163542,-8.77801910714516,
1.69768315121407E-11));
#24376=CARTESIAN_POINT('Ctrl Pts',(-7.07057502871922,-8.60301910714514,
4.08219839617346));
#24377=CARTESIAN_POINT('Ctrl Pts',(-4.71371668580301,-8.42801910714516,
8.16439679232994));
#24378=CARTESIAN_POINT('Ctrl Pts',(1.47018674401621E-11,-8.25301910714516,
8.16439679232146));
#24379=CARTESIAN_POINT('Ctrl Pts',(4.71371668583241,-8.07801910714515,8.16439679231297));
#24380=CARTESIAN_POINT('Ctrl Pts',(7.07057502873392,-7.90301910714516,4.082198396148));
#24381=CARTESIAN_POINT('Ctrl Pts',(9.42743337163542,-7.72801910714516,-1.69756769845304E-11));
#24382=CARTESIAN_POINT('Ctrl Pts',(7.07057502871922,-7.55301910714514,-4.08219839617346));
#24383=CARTESIAN_POINT('Ctrl Pts',(4.71371668580301,-7.37801910714516,-8.16439679232994));
#24384=CARTESIAN_POINT('Ctrl Pts',(-1.4702867290402E-11,-7.20301910714516,
-8.16439679232146));
#24385=CARTESIAN_POINT('Ctrl Pts',(-4.71371668583241,-7.02801910714516,
-8.16439679231297));
#24386=CARTESIAN_POINT('Ctrl Pts',(-7.07057502873392,-6.85301910714514,
-4.082198396148));
#24387=CARTESIAN_POINT('Ctrl Pts',(-9.42743337163542,-6.67801910714516,
1.69768315121407E-11));
#24388=CARTESIAN_POINT('Ctrl Pts',(-7.07057502871922,-6.50301910714514,
4.08219839617346));
#24389=CARTESIAN_POINT('Ctrl Pts',(-4.71371668580301,-6.32801910714515,
8.16439679232994));
#24390=CARTESIAN_POINT('Ctrl Pts',(1.47018674401621E-11,-6.15301910714516,
8.16439679232146));
#24391=CARTESIAN_POINT('Ctrl Pts',(4.71371668583241,-5.97801910714516,8.16439679231297));
#24392=CARTESIAN_POINT('Ctrl Pts',(7.07057502873392,-5.80301910714515,4.082198396148));
#24393=CARTESIAN_POINT('Ctrl Pts',(9.42743337163542,-5.62801910714516,-1.69756769845304E-11));
#24394=CARTESIAN_POINT('Ctrl Pts',(7.07057502871922,-5.45301910714515,-4.08219839617346));
#24395=CARTESIAN_POINT('Ctrl Pts',(4.71371668580301,-5.27801910714516,-8.16439679232994));
#24396=CARTESIAN_POINT('Ctrl Pts',(-1.4702867290402E-11,-5.10301910714516,
-8.16439679232146));
#24397=CARTESIAN_POINT('Ctrl Pts',(-4.71371668583241,-4.92801910714516,
-8.16439679231297));
#24398=CARTESIAN_POINT('Ctrl Pts',(-7.07057502873392,-4.75301910714515,
-4.082198396148));
#24399=CARTESIAN_POINT('Ctrl Pts',(-9.42743337163542,-4.57801910714517,
1.69768315121407E-11));
#24400=CARTESIAN_POINT('Ctrl Pts',(-7.07057502871922,-4.40301910714516,
4.08219839617346));
#24401=CARTESIAN_POINT('Ctrl Pts',(-4.71371668580301,-4.22801910714516,
8.16439679232994));
#24402=CARTESIAN_POINT('Ctrl Pts',(1.47018674401621E-11,-4.05301910714517,
8.16439679232146));
#24403=CARTESIAN_POINT('Ctrl Pts',(4.71371668583241,-3.87801910714518,8.16439679231297));
#24404=CARTESIAN_POINT('Ctrl Pts',(7.07057502873392,-3.70301910714515,4.082198396148));
#24405=CARTESIAN_POINT('Ctrl Pts',(9.42743337163542,-3.52801910714518,-1.69756769845304E-11));
#24406=CARTESIAN_POINT('Ctrl Pts',(7.07057502871922,-3.35301910714517,-4.08219839617346));
#24407=CARTESIAN_POINT('Ctrl Pts',(4.71371668580301,-3.17801910714516,-8.16439679232994));
#24408=CARTESIAN_POINT('Ctrl Pts',(-1.4702867290402E-11,-3.00301910714517,
-8.16439679232146));
#24409=CARTESIAN_POINT('Ctrl Pts',(-4.71371668583241,-2.82801910714518,
-8.16439679231297));
#24410=CARTESIAN_POINT('Ctrl Pts',(-7.07057502873392,-2.65301910714515,
-4.082198396148));
#24411=CARTESIAN_POINT('Ctrl Pts',(-9.42743337163542,-2.47801910714516,
1.69768315121407E-11));
#24412=CARTESIAN_POINT('Ctrl Pts',(-7.07057502871922,-2.30301910714517,
4.08219839617346));
#24413=CARTESIAN_POINT('Ctrl Pts',(-4.71371668580301,-2.12801910714516,
8.16439679232994));
#24414=CARTESIAN_POINT('Ctrl Pts',(1.47018674401621E-11,-1.95301910714515,
8.16439679232146));
#24415=CARTESIAN_POINT('Ctrl Pts',(4.71371668583241,-1.77801910714518,8.16439679231297));
#24416=CARTESIAN_POINT('Ctrl Pts',(7.07057502873392,-1.60301910714516,4.082198396148));
#24417=CARTESIAN_POINT('Ctrl Pts',(9.42743337163542,-1.42801910714516,-1.69756769845304E-11));
#24418=CARTESIAN_POINT('Ctrl Pts',(7.07057502871922,-1.25301910714517,-4.08219839617346));
#24419=CARTESIAN_POINT('Ctrl Pts',(4.71371668580301,-1.07801910714517,-8.16439679232994));
#24420=CARTESIAN_POINT('Ctrl Pts',(-1.4702867290402E-11,-0.903019107145155,
-8.16439679232146));
#24421=CARTESIAN_POINT('Ctrl Pts',(-4.71371668583241,-0.728019107145183,
-8.16439679231297));
#24422=CARTESIAN_POINT('Ctrl Pts',(-7.07057502873392,-0.553019107145171,
-4.082198396148));
#24423=CARTESIAN_POINT('Ctrl Pts',(-9.42743337163542,-0.378019107145163,
1.69768315121407E-11));
#24424=CARTESIAN_POINT('Ctrl Pts',(-7.07057502871922,-0.203019107145175,
4.08219839617346));
#24425=CARTESIAN_POINT('Ctrl Pts',(-4.71371668580301,-0.0280191071451809,
8.16439679232994));
#24426=CARTESIAN_POINT('Ctrl Pts',(1.47018674401621E-11,0.146980892854842,
8.16439679232146));
#24427=CARTESIAN_POINT('Ctrl Pts',(4.71371668583241,0.321980892854814,8.16439679231297));
#24428=CARTESIAN_POINT('Ctrl Pts',(7.07057502873392,0.496980892854826,4.082198396148));
#24429=CARTESIAN_POINT('Ctrl Pts',(9.42743337163542,0.671980892854834,-1.69756769845304E-11));
#24430=CARTESIAN_POINT('Ctrl Pts',(7.07057502871922,0.846980892854822,-4.08219839617346));
#24431=CARTESIAN_POINT('Ctrl Pts',(4.71371668580301,1.02198089285482,-8.16439679232994));
#24432=CARTESIAN_POINT('Ctrl Pts',(-1.4702867290402E-11,1.19698089285484,
-8.16439679232146));
#24433=CARTESIAN_POINT('Ctrl Pts',(-4.71371668583241,1.37198089285481,-8.16439679231297));
#24434=CARTESIAN_POINT('Ctrl Pts',(-7.07057502873392,1.54698089285482,-4.082198396148));
#24435=CARTESIAN_POINT('Ctrl Pts',(-9.42743337163542,1.72198089285483,1.69768315121407E-11));
#24436=CARTESIAN_POINT('Ctrl Pts',(-7.07057502871922,1.89698089285484,4.08219839617346));
#24437=CARTESIAN_POINT('Ctrl Pts',(-4.71371668580301,2.07198089285481,8.16439679232994));
#24438=CARTESIAN_POINT('Ctrl Pts',(1.47018674401621E-11,2.24698089285484,
8.16439679232146));
#24439=CARTESIAN_POINT('Ctrl Pts',(4.71371668583241,2.42198089285483,8.16439679231297));
#24440=CARTESIAN_POINT('Ctrl Pts',(7.07057502873392,2.59698089285482,4.082198396148));
#24441=CARTESIAN_POINT('Ctrl Pts',(9.42743337163542,2.77198089285483,-1.69756769845304E-11));
#24442=CARTESIAN_POINT('Ctrl Pts',(7.07057502871922,2.94698089285484,-4.08219839617346));
#24443=CARTESIAN_POINT('Ctrl Pts',(4.71371668580301,3.12198089285481,-8.16439679232994));
#24444=CARTESIAN_POINT('Ctrl Pts',(-1.4702867290402E-11,3.29698089285482,
-8.16439679232146));
#24445=CARTESIAN_POINT('Ctrl Pts',(-4.71371668583241,3.47198089285483,-8.16439679231297));
#24446=CARTESIAN_POINT('Ctrl Pts',(-7.07057502873392,3.64698089285482,-4.082198396148));
#24447=CARTESIAN_POINT('Ctrl Pts',(-9.42743337163542,3.82198089285481,1.69768315121407E-11));
#24448=CARTESIAN_POINT('Ctrl Pts',(-7.07057502871922,3.99698089285483,4.08219839617346));
#24449=CARTESIAN_POINT('Ctrl Pts',(-4.71371668580301,4.17198089285481,8.16439679232994));
#24450=CARTESIAN_POINT('Ctrl Pts',(1.47018674401621E-11,4.34698089285482,
8.16439679232146));
#24451=CARTESIAN_POINT('Ctrl Pts',(4.71371668583241,4.52198089285483,8.16439679231297));
#24452=CARTESIAN_POINT('Ctrl Pts',(7.07057502873392,4.69698089285481,4.082198396148));
#24453=CARTESIAN_POINT('Ctrl Pts',(9.42743337163542,4.87198089285481,-1.69756769845304E-11));
#24454=CARTESIAN_POINT('Ctrl Pts',(7.07057502871922,5.04698089285483,-4.08219839617346));
#24455=CARTESIAN_POINT('Ctrl Pts',(4.71371668580301,5.22198089285481,-8.16439679232994));
#24456=CARTESIAN_POINT('Ctrl Pts',(-1.4702867290402E-11,5.39698089285482,
-8.16439679232146));
#24457=CARTESIAN_POINT('Ctrl Pts',(-4.71371668583241,5.57198089285483,-8.16439679231297));
#24458=CARTESIAN_POINT('Ctrl Pts',(-7.07057502873392,5.74698089285481,-4.082198396148));
#24459=CARTESIAN_POINT('Ctrl Pts',(-9.42743337163542,5.92198089285481,1.69768315121407E-11));
#24460=CARTESIAN_POINT('Ctrl Pts',(-7.07057502871922,6.09698089285483,4.08219839617346));
#24461=CARTESIAN_POINT('Ctrl Pts',(-4.71371668580301,6.2719808928548,8.16439679232994));
#24462=CARTESIAN_POINT('Ctrl Pts',(1.47018674401621E-11,6.44698089285481,
8.16439679232146));
#24463=CARTESIAN_POINT('Ctrl Pts',(4.71371668583241,6.62198089285482,8.16439679231297));
#24464=CARTESIAN_POINT('Ctrl Pts',(7.07057502873392,6.79698089285483,4.082198396148));
#24465=CARTESIAN_POINT('Ctrl Pts',(9.42743337163542,6.97198089285481,-1.69756769845304E-11));
#24466=CARTESIAN_POINT('Ctrl Pts',(7.07057502871922,7.14698089285482,-4.08219839617346));
#24467=CARTESIAN_POINT('Ctrl Pts',(4.71371668580301,7.32198089285482,-8.16439679232994));
#24468=CARTESIAN_POINT('Ctrl Pts',(-1.4702867290402E-11,7.49698089285481,
-8.16439679232146));
#24469=CARTESIAN_POINT('Ctrl Pts',(-4.71371668583241,7.67198089285481,-8.16439679231297));
#24470=CARTESIAN_POINT('Ctrl Pts',(-7.07057502873392,7.84698089285483,-4.082198396148));
#24471=CARTESIAN_POINT('Ctrl Pts',(-9.42743337163542,8.0219808928548,1.69768315121407E-11));
#24472=CARTESIAN_POINT('Ctrl Pts',(-7.07057502871922,8.19698089285481,4.08219839617346));
#24473=CARTESIAN_POINT('Ctrl Pts',(-4.71371668580301,8.37198089285483,8.16439679232994));
#24474=CARTESIAN_POINT('Ctrl Pts',(1.47018674401621E-11,8.54698089285481,
8.16439679232146));
#24475=CARTESIAN_POINT('Ctrl Pts',(4.71371668583241,8.72198089285481,8.16439679231297));
#24476=CARTESIAN_POINT('Ctrl Pts',(7.07057502873392,8.89698089285482,4.082198396148));
#24477=CARTESIAN_POINT('Ctrl Pts',(9.42743337163542,9.0719808928548,-1.69756769845304E-11));
#24478=CARTESIAN_POINT('Ctrl Pts',(7.07057502871922,9.24698089285481,-4.08219839617346));
#24479=CARTESIAN_POINT('Ctrl Pts',(4.71371668580301,9.42198089285482,-8.16439679232994));
#24480=CARTESIAN_POINT('Ctrl Pts',(-1.4702867290402E-11,9.5969808928548,
-8.16439679232146));
#24481=CARTESIAN_POINT('Ctrl Pts',(-4.71371668583241,9.7719808928548,-8.16439679231297));
#24482=CARTESIAN_POINT('Ctrl Pts',(-7.07057502873392,9.94698089285482,-4.082198396148));
#24483=CARTESIAN_POINT('Ctrl Pts',(-9.42743337163542,10.1219808928548,1.69768315121407E-11));
#24484=CARTESIAN_POINT('Ctrl Pts',(-7.07057502871922,10.2969808928548,4.08219839617346));
#24485=CARTESIAN_POINT('Ctrl Pts',(-4.71371668580301,10.4719808928548,8.16439679232994));
#24486=CARTESIAN_POINT('Ctrl Pts',(1.47018674401621E-11,10.6469808928548,
8.16439679232146));
#24487=CARTESIAN_POINT('Ctrl Pts',(4.71371668583241,10.8219808928548,8.16439679231297));
#24488=CARTESIAN_POINT('Ctrl Pts',(7.07057502873392,10.9969808928548,4.082198396148));
#24489=CARTESIAN_POINT('Ctrl Pts',(9.42743337163542,11.1719808928548,-1.69756769845304E-11));
#24490=CARTESIAN_POINT('Ctrl Pts',(7.07057502871922,11.3469808928548,-4.08219839617346));
#24491=CARTESIAN_POINT('Ctrl Pts',(4.71371668580301,11.5219808928548,-8.16439679232994));
#24492=CARTESIAN_POINT('Ctrl Pts',(-1.4702867290402E-11,11.6969808928548,
-8.16439679232146));
#24493=CARTESIAN_POINT('Ctrl Pts',(-4.71371668583241,11.8719808928548,-8.16439679231297));
#24494=CARTESIAN_POINT('Ctrl Pts',(-7.07057502873392,12.0469808928548,-4.082198396148));
#24495=CARTESIAN_POINT('Ctrl Pts',(-9.42743337163542,12.2219808928548,1.69768315121407E-11));
#24496=CARTESIAN_POINT('Ctrl Pts',(-7.07057502871922,12.3969808928548,4.08219839617346));
#24497=CARTESIAN_POINT('Ctrl Pts',(-4.71371668580301,12.5719808928548,8.16439679232994));
#24498=CARTESIAN_POINT('Ctrl Pts',(1.47018674401621E-11,12.7469808928548,
8.16439679232146));
#24499=CARTESIAN_POINT('Ctrl Pts',(4.71371668583241,12.9219808928548,8.16439679231297));
#24500=CARTESIAN_POINT('Ctrl Pts',(7.07057502873392,13.0969808928548,4.082198396148));
#24501=CARTESIAN_POINT('Ctrl Pts',(9.42743337163542,13.2719808928548,-1.69756769845304E-11));
#24502=CARTESIAN_POINT('Ctrl Pts',(7.07057502871922,13.4469808928548,-4.08219839617346));
#24503=CARTESIAN_POINT('Ctrl Pts',(4.71371668580301,13.6219808928548,-8.16439679232994));
#24504=CARTESIAN_POINT('Ctrl Pts',(-1.4702867290402E-11,13.7969808928548,
-8.16439679232146));
#24505=CARTESIAN_POINT('Ctrl Pts',(-4.71371668583241,13.9719808928548,-8.16439679231297));
#24506=CARTESIAN_POINT('Ctrl Pts',(-7.07057502873392,14.1469808928548,-4.082198396148));
#24507=CARTESIAN_POINT('Ctrl Pts',(-9.42743337163542,14.3219808928548,1.69768315121407E-11));
#24508=CARTESIAN_POINT('Ctrl Pts',(-7.07057502871922,14.4969808928548,4.08219839617346));
#24509=CARTESIAN_POINT('Ctrl Pts',(-4.71371668580301,14.6719808928548,8.16439679232994));
#24510=CARTESIAN_POINT('Ctrl Pts',(1.47018674401621E-11,14.8469808928548,
8.16439679232146));
#24511=CARTESIAN_POINT('Ctrl Pts',(4.71371668583241,15.0219808928548,8.16439679231297));
#24512=CARTESIAN_POINT('Ctrl Pts',(7.07057502873392,15.1969808928548,4.082198396148));
#24513=CARTESIAN_POINT('Ctrl Pts',(9.42743337163542,15.3719808928548,-1.69756769845304E-11));
#24514=CARTESIAN_POINT('Ctrl Pts',(7.07057502871922,15.5469808928548,-4.08219839617346));
#24515=CARTESIAN_POINT('Ctrl Pts',(4.71371668580301,15.7219808928548,-8.16439679232994));
#24516=CARTESIAN_POINT('Ctrl Pts',(-1.4702867290402E-11,15.8969808928548,
-8.16439679232146));
#24517=CARTESIAN_POINT('Ctrl Pts',(-4.71371668583241,16.0719808928548,-8.16439679231297));
#24518=CARTESIAN_POINT('Ctrl Pts',(-7.07057502873392,16.2469808928548,-4.082198396148));
#24519=CARTESIAN_POINT('Ctrl Pts',(-9.42743337163542,16.4219808928548,1.69768315121407E-11));
#24520=CARTESIAN_POINT('Ctrl Pts',(-7.07057502871922,16.5969808928548,4.08219839617346));
#24521=CARTESIAN_POINT('Ctrl Pts',(-4.71371668580301,16.7719808928548,8.16439679232994));
#24522=CARTESIAN_POINT('Ctrl Pts',(1.47018674401621E-11,16.9469808928548,
8.16439679232146));
#24523=CARTESIAN_POINT('Ctrl Pts',(4.71371668583241,17.1219808928548,8.16439679231297));
#24524=CARTESIAN_POINT('Ctrl Pts',(7.07057502873392,17.2969808928548,4.082198396148));
#24525=CARTESIAN_POINT('Ctrl Pts',(9.42743337163542,17.4719808928548,-1.69756769845304E-11));
#24526=CARTESIAN_POINT('Ctrl Pts',(7.07057502871922,17.6469808928548,-4.08219839617346));
#24527=CARTESIAN_POINT('Ctrl Pts',(4.71371668580301,17.8219808928548,-8.16439679232994));
#24528=CARTESIAN_POINT('Ctrl Pts',(-1.4702867290402E-11,17.9969808928548,
-8.16439679232146));
#24529=CARTESIAN_POINT('Ctrl Pts',(-4.71371668583241,18.1719808928548,-8.16439679231297));
#24530=CARTESIAN_POINT('Ctrl Pts',(-7.07057502873392,18.3469808928548,-4.082198396148));
#24531=CARTESIAN_POINT('Ctrl Pts',(-9.42743337163542,18.5219808928548,1.69768315121407E-11));
#24532=CARTESIAN_POINT('Ctrl Pts',(-7.07057502871922,18.6969808928548,4.08219839617346));
#24533=CARTESIAN_POINT('Ctrl Pts',(-4.71371668580301,18.8719808928548,8.16439679232994));
#24534=CARTESIAN_POINT('Ctrl Pts',(1.47018674401621E-11,19.0469808928548,
8.16439679232146));
#24535=CARTESIAN_POINT('Ctrl Pts',(4.71371668583241,19.2219808928548,8.16439679231297));
#24536=CARTESIAN_POINT('Ctrl Pts',(7.07057502873392,19.3969808928548,4.082198396148));
#24537=CARTESIAN_POINT('Ctrl Pts',(9.42743337163542,19.5719808928548,-1.69756769845304E-11));
#24538=CARTESIAN_POINT('Ctrl Pts',(7.07057502871922,19.7469808928548,-4.08219839617346));
#24539=CARTESIAN_POINT('Ctrl Pts',(4.71371668580301,19.9219808928548,-8.16439679232994));
#24540=CARTESIAN_POINT('Ctrl Pts',(-1.4702867290402E-11,20.0969808928548,
-8.16439679232146));
#24541=CARTESIAN_POINT('Ctrl Pts',(-4.71371668583241,20.2719808928548,-8.16439679231297));
#24542=CARTESIAN_POINT('Ctrl Pts',(-7.07057502873392,20.4469808928548,-4.082198396148));
#24543=CARTESIAN_POINT('Ctrl Pts',(-9.42743337163542,20.6219808928548,1.69768315121407E-11));
#24544=CARTESIAN_POINT('Ctrl Pts',(-7.07057502871922,20.7969808928548,4.08219839617346));
#24545=CARTESIAN_POINT('Ctrl Pts',(-4.71371668580301,20.9719808928548,8.16439679232994));
#24546=CARTESIAN_POINT('Ctrl Pts',(1.47018674401621E-11,21.1469808928548,
8.16439679232146));
#24547=CARTESIAN_POINT('Ctrl Pts',(4.71371668583241,21.3219808928548,8.16439679231297));
#24548=CARTESIAN_POINT('Ctrl Pts',(7.07057502873392,21.4969808928548,4.082198396148));
#24549=CARTESIAN_POINT('Ctrl Pts',(9.42743337163542,21.6719808928548,-1.69756769845304E-11));
#24550=CARTESIAN_POINT('Ctrl Pts',(7.07057502871922,21.8469808928548,-4.08219839617346));
#24551=CARTESIAN_POINT('Ctrl Pts',(4.71371668580301,22.0219808928548,-8.16439679232994));
#24552=CARTESIAN_POINT('Ctrl Pts',(-1.4702867290402E-11,22.1969808928548,
-8.16439679232146));
#24553=CARTESIAN_POINT('Ctrl Pts',(-4.71371668583241,22.3719808928548,-8.16439679231297));
#24554=CARTESIAN_POINT('Ctrl Pts',(-7.07057502873392,22.5469808928548,-4.082198396148));
#24555=CARTESIAN_POINT('Ctrl Pts',(-9.42743337163542,22.7219808928548,1.69768315121407E-11));
#24556=CARTESIAN_POINT('Ctrl Pts',(-7.07057502871922,22.8969808928548,4.08219839617346));
#24557=CARTESIAN_POINT('Ctrl Pts',(-4.71371668580301,23.0719808928548,8.16439679232994));
#24558=CARTESIAN_POINT('Ctrl Pts',(1.47018674401621E-11,23.2469808928548,
8.16439679232146));
#24559=CARTESIAN_POINT('Ctrl Pts',(4.71371668583241,23.4219808928548,8.16439679231297));
#24560=CARTESIAN_POINT('Ctrl Pts',(7.07057502873392,23.5969808928548,4.082198396148));
#24561=CARTESIAN_POINT('Ctrl Pts',(9.42743337163542,23.7719808928548,-1.69756769845304E-11));
#24562=CARTESIAN_POINT('Ctrl Pts',(7.07057502871922,23.9469808928548,-4.08219839617346));
#24563=CARTESIAN_POINT('Ctrl Pts',(4.71371668580301,24.1219808928548,-8.16439679232994));
#24564=CARTESIAN_POINT('Ctrl Pts',(-1.4702867290402E-11,24.2969808928548,
-8.16439679232146));
#24565=CARTESIAN_POINT('Ctrl Pts',(-4.71371668583241,24.4719808928548,-8.16439679231297));
#24566=CARTESIAN_POINT('Ctrl Pts',(-7.07057502873392,24.6469808928548,-4.082198396148));
#24567=CARTESIAN_POINT('Ctrl Pts',(-9.42743337163542,24.8219808928548,1.69768315121407E-11));
#24568=CARTESIAN_POINT('Ctrl Pts',(-7.07057502871922,24.9969808928548,4.08219839617346));
#24569=CARTESIAN_POINT('Ctrl Pts',(-4.71371668580301,25.1719808928548,8.16439679232994));
#24570=CARTESIAN_POINT('Ctrl Pts',(1.47018674401621E-11,25.3469808928548,
8.16439679232146));
#24571=CARTESIAN_POINT('Ctrl Pts',(4.71371668583241,25.5219808928548,8.16439679231297));
#24572=CARTESIAN_POINT('Ctrl Pts',(7.07057502873392,25.6969808928548,4.082198396148));
#24573=CARTESIAN_POINT('Ctrl Pts',(9.42743337163542,25.8719808928548,-1.69756769845304E-11));
#24574=CARTESIAN_POINT('Ctrl Pts',(7.07057502871922,26.0469808928548,-4.08219839617346));
#24575=CARTESIAN_POINT('Ctrl Pts',(4.71371668580301,26.2219808928548,-8.16439679232994));
#24576=CARTESIAN_POINT('Ctrl Pts',(-1.4702867290402E-11,26.3969808928548,
-8.16439679232146));
#24577=CARTESIAN_POINT('Ctrl Pts',(-1.51301075899711E-11,-143.579517970998,
-8.40164026751963));
#24578=CARTESIAN_POINT('Ctrl Pts',(-4.85068927010199,-143.404517970998,
-8.4016402675109));
#24579=CARTESIAN_POINT('Ctrl Pts',(-7.27603390513785,-143.229517970998,
-4.20082013374671));
#24580=CARTESIAN_POINT('Ctrl Pts',(-9.70137854017372,-143.054517970998,
1.74701493417668E-11));
#24581=CARTESIAN_POINT('Ctrl Pts',(-7.27603390512272,-142.879517970998,
4.20082013377292));
#24582=CARTESIAN_POINT('Ctrl Pts',(-4.85068927007173,-142.704517970998,
8.40164026752836));
#24583=CARTESIAN_POINT('Ctrl Pts',(1.5129078685785E-11,-142.529517970998,
8.40164026751963));
#24584=CARTESIAN_POINT('Ctrl Pts',(4.85068927010198,-142.354517970998,8.4016402675109));
#24585=CARTESIAN_POINT('Ctrl Pts',(7.27603390513785,-142.179517970998,4.20082013374672));
#24586=CARTESIAN_POINT('Ctrl Pts',(9.70137854017372,-142.004517970998,-1.74689612655491E-11));
#24587=CARTESIAN_POINT('Ctrl Pts',(7.27603390512273,-141.829517970998,-4.20082013377291));
#24588=CARTESIAN_POINT('Ctrl Pts',(4.85068927007173,-141.654517970998,-8.40164026752836));
#24589=CARTESIAN_POINT('Ctrl Pts',(-1.51301075899711E-11,-141.479517970998,
-8.40164026751963));
#24590=CARTESIAN_POINT('Ctrl Pts',(-4.85068927010199,-141.304517970998,
-8.4016402675109));
#24591=CARTESIAN_POINT('Ctrl Pts',(-7.27603390513785,-141.129517970998,
-4.20082013374671));
#24592=CARTESIAN_POINT('Ctrl Pts',(-9.70137854017372,-140.954517970998,
1.74701493417668E-11));
#24593=CARTESIAN_POINT('Ctrl Pts',(-7.27603390512272,-140.779517970998,
4.20082013377292));
#24594=CARTESIAN_POINT('Ctrl Pts',(-4.85068927007173,-140.604517970998,
8.40164026752836));
#24595=CARTESIAN_POINT('Ctrl Pts',(1.5129078685785E-11,-140.429517970998,
8.40164026751963));
#24596=CARTESIAN_POINT('Ctrl Pts',(4.85068927010198,-140.254517970998,8.4016402675109));
#24597=CARTESIAN_POINT('Ctrl Pts',(7.27603390513785,-140.079517970998,4.20082013374672));
#24598=CARTESIAN_POINT('Ctrl Pts',(9.70137854017372,-139.904517970998,-1.74689612655491E-11));
#24599=CARTESIAN_POINT('Ctrl Pts',(7.27603390512273,-139.729517970998,-4.20082013377291));
#24600=CARTESIAN_POINT('Ctrl Pts',(4.85068927007173,-139.554517970998,-8.40164026752836));
#24601=CARTESIAN_POINT('Ctrl Pts',(-1.51301075899711E-11,-139.379517970998,
-8.40164026751963));
#24602=CARTESIAN_POINT('Ctrl Pts',(-4.85068927010199,-139.204517970998,
-8.4016402675109));
#24603=CARTESIAN_POINT('Ctrl Pts',(-7.27603390513785,-139.029517970998,
-4.20082013374671));
#24604=CARTESIAN_POINT('Ctrl Pts',(-9.70137854017372,-138.854517970998,
1.74701493417668E-11));
#24605=CARTESIAN_POINT('Ctrl Pts',(-7.27603390512272,-138.679517970998,
4.20082013377292));
#24606=CARTESIAN_POINT('Ctrl Pts',(-4.85068927007173,-138.504517970998,
8.40164026752836));
#24607=CARTESIAN_POINT('Ctrl Pts',(1.5129078685785E-11,-138.329517970998,
8.40164026751963));
#24608=CARTESIAN_POINT('Ctrl Pts',(4.85068927010198,-138.154517970998,8.4016402675109));
#24609=CARTESIAN_POINT('Ctrl Pts',(7.27603390513785,-137.979517970998,4.20082013374672));
#24610=CARTESIAN_POINT('Ctrl Pts',(9.70137854017372,-137.804517970998,-1.74689612655491E-11));
#24611=CARTESIAN_POINT('Ctrl Pts',(7.27603390512273,-137.629517970998,-4.20082013377291));
#24612=CARTESIAN_POINT('Ctrl Pts',(4.85068927007173,-137.454517970998,-8.40164026752836));
#24613=CARTESIAN_POINT('Ctrl Pts',(-1.51301075899711E-11,-137.279517970998,
-8.40164026751963));
#24614=CARTESIAN_POINT('Ctrl Pts',(-4.85068927010199,-137.104517970998,
-8.4016402675109));
#24615=CARTESIAN_POINT('Ctrl Pts',(-7.27603390513785,-136.929517970998,
-4.20082013374671));
#24616=CARTESIAN_POINT('Ctrl Pts',(-9.70137854017372,-136.754517970998,
1.74701493417668E-11));
#24617=CARTESIAN_POINT('Ctrl Pts',(-7.27603390512272,-136.579517970998,
4.20082013377292));
#24618=CARTESIAN_POINT('Ctrl Pts',(-4.85068927007173,-136.404517970998,
8.40164026752836));
#24619=CARTESIAN_POINT('Ctrl Pts',(1.5129078685785E-11,-136.229517970998,
8.40164026751963));
#24620=CARTESIAN_POINT('Ctrl Pts',(4.85068927010198,-136.054517970998,8.4016402675109));
#24621=CARTESIAN_POINT('Ctrl Pts',(7.27603390513785,-135.879517970998,4.20082013374672));
#24622=CARTESIAN_POINT('Ctrl Pts',(9.70137854017372,-135.704517970998,-1.74689612655491E-11));
#24623=CARTESIAN_POINT('Ctrl Pts',(7.27603390512273,-135.529517970998,-4.20082013377291));
#24624=CARTESIAN_POINT('Ctrl Pts',(4.85068927007173,-135.354517970998,-8.40164026752836));
#24625=CARTESIAN_POINT('Ctrl Pts',(-1.51301075899711E-11,-135.179517970998,
-8.40164026751963));
#24626=CARTESIAN_POINT('Ctrl Pts',(-4.85068927010199,-135.004517970998,
-8.4016402675109));
#24627=CARTESIAN_POINT('Ctrl Pts',(-7.27603390513785,-134.829517970998,
-4.20082013374671));
#24628=CARTESIAN_POINT('Ctrl Pts',(-9.70137854017372,-134.654517970998,
1.74701493417668E-11));
#24629=CARTESIAN_POINT('Ctrl Pts',(-7.27603390512272,-134.479517970998,
4.20082013377292));
#24630=CARTESIAN_POINT('Ctrl Pts',(-4.85068927007173,-134.304517970998,
8.40164026752836));
#24631=CARTESIAN_POINT('Ctrl Pts',(1.5129078685785E-11,-134.129517970998,
8.40164026751963));
#24632=CARTESIAN_POINT('Ctrl Pts',(4.85068927010198,-133.954517970998,8.4016402675109));
#24633=CARTESIAN_POINT('Ctrl Pts',(7.27603390513785,-133.779517970998,4.20082013374672));
#24634=CARTESIAN_POINT('Ctrl Pts',(9.70137854017372,-133.604517970998,-1.74689612655491E-11));
#24635=CARTESIAN_POINT('Ctrl Pts',(7.27603390512273,-133.429517970998,-4.20082013377291));
#24636=CARTESIAN_POINT('Ctrl Pts',(4.85068927007173,-133.254517970998,-8.40164026752836));
#24637=CARTESIAN_POINT('Ctrl Pts',(-1.51301075899711E-11,-133.079517970998,
-8.40164026751963));
#24638=CARTESIAN_POINT('Ctrl Pts',(-4.85068927010199,-132.904517970998,
-8.4016402675109));
#24639=CARTESIAN_POINT('Ctrl Pts',(-7.27603390513785,-132.729517970998,
-4.20082013374671));
#24640=CARTESIAN_POINT('Ctrl Pts',(-9.70137854017372,-132.554517970998,
1.74701493417668E-11));
#24641=CARTESIAN_POINT('Ctrl Pts',(-7.27603390512272,-132.379517970998,
4.20082013377292));
#24642=CARTESIAN_POINT('Ctrl Pts',(-4.85068927007173,-132.204517970998,
8.40164026752836));
#24643=CARTESIAN_POINT('Ctrl Pts',(1.5129078685785E-11,-132.029517970998,
8.40164026751963));
#24644=CARTESIAN_POINT('Ctrl Pts',(4.85068927010198,-131.854517970998,8.4016402675109));
#24645=CARTESIAN_POINT('Ctrl Pts',(7.27603390513785,-131.679517970998,4.20082013374672));
#24646=CARTESIAN_POINT('Ctrl Pts',(9.70137854017372,-131.504517970998,-1.74689612655491E-11));
#24647=CARTESIAN_POINT('Ctrl Pts',(7.27603390512273,-131.329517970998,-4.20082013377291));
#24648=CARTESIAN_POINT('Ctrl Pts',(4.85068927007173,-131.154517970998,-8.40164026752836));
#24649=CARTESIAN_POINT('Ctrl Pts',(-1.51301075899711E-11,-130.979517970998,
-8.40164026751963));
#24650=CARTESIAN_POINT('Ctrl Pts',(-4.85068927010199,-130.804517970998,
-8.4016402675109));
#24651=CARTESIAN_POINT('Ctrl Pts',(-7.27603390513785,-130.629517970998,
-4.20082013374671));
#24652=CARTESIAN_POINT('Ctrl Pts',(-9.70137854017372,-130.454517970998,
1.74701493417668E-11));
#24653=CARTESIAN_POINT('Ctrl Pts',(-7.27603390512272,-130.279517970998,
4.20082013377292));
#24654=CARTESIAN_POINT('Ctrl Pts',(-4.85068927007173,-130.104517970998,
8.40164026752836));
#24655=CARTESIAN_POINT('Ctrl Pts',(1.5129078685785E-11,-129.929517970998,
8.40164026751963));
#24656=CARTESIAN_POINT('Ctrl Pts',(4.85068927010198,-129.754517970998,8.4016402675109));
#24657=CARTESIAN_POINT('Ctrl Pts',(7.27603390513785,-129.579517970998,4.20082013374672));
#24658=CARTESIAN_POINT('Ctrl Pts',(9.70137854017372,-129.404517970998,-1.74689612655491E-11));
#24659=CARTESIAN_POINT('Ctrl Pts',(7.27603390512273,-129.229517970998,-4.20082013377291));
#24660=CARTESIAN_POINT('Ctrl Pts',(4.85068927007173,-129.054517970998,-8.40164026752836));
#24661=CARTESIAN_POINT('Ctrl Pts',(-1.51301075899711E-11,-128.879517970998,
-8.40164026751963));
#24662=CARTESIAN_POINT('Ctrl Pts',(-4.85068927010199,-128.704517970998,
-8.4016402675109));
#24663=CARTESIAN_POINT('Ctrl Pts',(-7.27603390513785,-128.529517970998,
-4.20082013374671));
#24664=CARTESIAN_POINT('Ctrl Pts',(-9.70137854017372,-128.354517970998,
1.74701493417668E-11));
#24665=CARTESIAN_POINT('Ctrl Pts',(-7.27603390512272,-128.179517970998,
4.20082013377292));
#24666=CARTESIAN_POINT('Ctrl Pts',(-4.85068927007173,-128.004517970998,
8.40164026752836));
#24667=CARTESIAN_POINT('Ctrl Pts',(1.5129078685785E-11,-127.829517970998,
8.40164026751963));
#24668=CARTESIAN_POINT('Ctrl Pts',(4.85068927010198,-127.654517970998,8.4016402675109));
#24669=CARTESIAN_POINT('Ctrl Pts',(7.27603390513785,-127.479517970998,4.20082013374672));
#24670=CARTESIAN_POINT('Ctrl Pts',(9.70137854017372,-127.304517970998,-1.74689612655491E-11));
#24671=CARTESIAN_POINT('Ctrl Pts',(7.27603390512273,-127.129517970998,-4.20082013377291));
#24672=CARTESIAN_POINT('Ctrl Pts',(4.85068927007173,-126.954517970998,-8.40164026752836));
#24673=CARTESIAN_POINT('Ctrl Pts',(-1.51301075899711E-11,-126.779517970998,
-8.40164026751963));
#24674=CARTESIAN_POINT('Ctrl Pts',(-4.85068927010199,-126.604517970998,
-8.4016402675109));
#24675=CARTESIAN_POINT('Ctrl Pts',(-7.27603390513785,-126.429517970998,
-4.20082013374671));
#24676=CARTESIAN_POINT('Ctrl Pts',(-9.70137854017372,-126.254517970998,
1.74701493417668E-11));
#24677=CARTESIAN_POINT('Ctrl Pts',(-7.27603390512272,-126.079517970998,
4.20082013377292));
#24678=CARTESIAN_POINT('Ctrl Pts',(-4.85068927007173,-125.904517970998,
8.40164026752836));
#24679=CARTESIAN_POINT('Ctrl Pts',(1.5129078685785E-11,-125.729517970998,
8.40164026751963));
#24680=CARTESIAN_POINT('Ctrl Pts',(4.85068927010198,-125.554517970998,8.4016402675109));
#24681=CARTESIAN_POINT('Ctrl Pts',(7.27603390513785,-125.379517970998,4.20082013374672));
#24682=CARTESIAN_POINT('Ctrl Pts',(9.70137854017372,-125.204517970998,-1.74689612655491E-11));
#24683=CARTESIAN_POINT('Ctrl Pts',(7.27603390512273,-125.029517970998,-4.20082013377291));
#24684=CARTESIAN_POINT('Ctrl Pts',(4.85068927007173,-124.854517970998,-8.40164026752836));
#24685=CARTESIAN_POINT('Ctrl Pts',(-1.51301075899711E-11,-124.679517970998,
-8.40164026751963));
#24686=CARTESIAN_POINT('Ctrl Pts',(-4.85068927010199,-124.504517970998,
-8.4016402675109));
#24687=CARTESIAN_POINT('Ctrl Pts',(-7.27603390513785,-124.329517970998,
-4.20082013374671));
#24688=CARTESIAN_POINT('Ctrl Pts',(-9.70137854017372,-124.154517970998,
1.74701493417668E-11));
#24689=CARTESIAN_POINT('Ctrl Pts',(-7.27603390512272,-123.979517970998,
4.20082013377292));
#24690=CARTESIAN_POINT('Ctrl Pts',(-4.85068927007173,-123.804517970998,
8.40164026752836));
#24691=CARTESIAN_POINT('Ctrl Pts',(1.5129078685785E-11,-123.629517970998,
8.40164026751963));
#24692=CARTESIAN_POINT('Ctrl Pts',(4.85068927010198,-123.454517970998,8.4016402675109));
#24693=CARTESIAN_POINT('Ctrl Pts',(7.27603390513785,-123.279517970998,4.20082013374672));
#24694=CARTESIAN_POINT('Ctrl Pts',(9.70137854017372,-123.104517970998,-1.74689612655491E-11));
#24695=CARTESIAN_POINT('Ctrl Pts',(7.27603390512273,-122.929517970998,-4.20082013377291));
#24696=CARTESIAN_POINT('Ctrl Pts',(4.85068927007173,-122.754517970998,-8.40164026752836));
#24697=CARTESIAN_POINT('Ctrl Pts',(-1.51301075899711E-11,-122.579517970998,
-8.40164026751963));
#24698=CARTESIAN_POINT('Ctrl Pts',(-4.85068927010199,-122.404517970998,
-8.4016402675109));
#24699=CARTESIAN_POINT('Ctrl Pts',(-7.27603390513785,-122.229517970998,
-4.20082013374671));
#24700=CARTESIAN_POINT('Ctrl Pts',(-9.70137854017372,-122.054517970998,
1.74701493417668E-11));
#24701=CARTESIAN_POINT('Ctrl Pts',(-7.27603390512272,-121.879517970998,
4.20082013377292));
#24702=CARTESIAN_POINT('Ctrl Pts',(-4.85068927007173,-121.704517970998,
8.40164026752836));
#24703=CARTESIAN_POINT('Ctrl Pts',(1.5129078685785E-11,-121.529517970998,
8.40164026751963));
#24704=CARTESIAN_POINT('Ctrl Pts',(4.85068927010198,-121.354517970998,8.4016402675109));
#24705=CARTESIAN_POINT('Ctrl Pts',(7.27603390513785,-121.179517970998,4.20082013374672));
#24706=CARTESIAN_POINT('Ctrl Pts',(9.70137854017372,-121.004517970998,-1.74689612655491E-11));
#24707=CARTESIAN_POINT('Ctrl Pts',(7.27603390512273,-120.829517970998,-4.20082013377291));
#24708=CARTESIAN_POINT('Ctrl Pts',(4.85068927007173,-120.654517970998,-8.40164026752836));
#24709=CARTESIAN_POINT('Ctrl Pts',(-1.51301075899711E-11,-120.479517970998,
-8.40164026751963));
#24710=CARTESIAN_POINT('Ctrl Pts',(-4.85068927010199,-120.304517970998,
-8.4016402675109));
#24711=CARTESIAN_POINT('Ctrl Pts',(-7.27603390513785,-120.129517970998,
-4.20082013374671));
#24712=CARTESIAN_POINT('Ctrl Pts',(-9.70137854017372,-119.954517970998,
1.74701493417668E-11));
#24713=CARTESIAN_POINT('Ctrl Pts',(-7.27603390512272,-119.779517970998,
4.20082013377292));
#24714=CARTESIAN_POINT('Ctrl Pts',(-4.85068927007173,-119.604517970998,
8.40164026752836));
#24715=CARTESIAN_POINT('Ctrl Pts',(1.5129078685785E-11,-119.429517970998,
8.40164026751963));
#24716=CARTESIAN_POINT('Ctrl Pts',(4.85068927010198,-119.254517970998,8.4016402675109));
#24717=CARTESIAN_POINT('Ctrl Pts',(7.27603390513785,-119.079517970998,4.20082013374672));
#24718=CARTESIAN_POINT('Ctrl Pts',(9.70137854017372,-118.904517970998,-1.74689612655491E-11));
#24719=CARTESIAN_POINT('Ctrl Pts',(7.27603390512273,-118.729517970998,-4.20082013377291));
#24720=CARTESIAN_POINT('Ctrl Pts',(4.85068927007173,-118.554517970998,-8.40164026752836));
#24721=CARTESIAN_POINT('Ctrl Pts',(-1.51301075899711E-11,-118.379517970998,
-8.40164026751963));
#24722=CARTESIAN_POINT('Ctrl Pts',(-4.85068927010199,-118.204517970998,
-8.4016402675109));
#24723=CARTESIAN_POINT('Ctrl Pts',(-7.27603390513785,-118.029517970998,
-4.20082013374671));
#24724=CARTESIAN_POINT('Ctrl Pts',(-9.70137854017372,-117.854517970998,
1.74701493417668E-11));
#24725=CARTESIAN_POINT('Ctrl Pts',(-7.27603390512272,-117.679517970998,
4.20082013377292));
#24726=CARTESIAN_POINT('Ctrl Pts',(-4.85068927007173,-117.504517970998,
8.40164026752836));
#24727=CARTESIAN_POINT('Ctrl Pts',(1.5129078685785E-11,-117.329517970998,
8.40164026751963));
#24728=CARTESIAN_POINT('Ctrl Pts',(4.85068927010198,-117.154517970998,8.4016402675109));
#24729=CARTESIAN_POINT('Ctrl Pts',(7.27603390513785,-116.979517970998,4.20082013374672));
#24730=CARTESIAN_POINT('Ctrl Pts',(9.70137854017372,-116.804517970998,-1.74689612655491E-11));
#24731=CARTESIAN_POINT('Ctrl Pts',(7.27603390512273,-116.629517970998,-4.20082013377291));
#24732=CARTESIAN_POINT('Ctrl Pts',(4.85068927007173,-116.454517970998,-8.40164026752836));
#24733=CARTESIAN_POINT('Ctrl Pts',(-1.51301075899711E-11,-116.279517970998,
-8.40164026751963));
#24734=CARTESIAN_POINT('Ctrl Pts',(-4.85068927010199,-116.104517970998,
-8.4016402675109));
#24735=CARTESIAN_POINT('Ctrl Pts',(-7.27603390513785,-115.929517970998,
-4.20082013374671));
#24736=CARTESIAN_POINT('Ctrl Pts',(-9.70137854017372,-115.754517970998,
1.74701493417668E-11));
#24737=CARTESIAN_POINT('Ctrl Pts',(-7.27603390512272,-115.579517970998,
4.20082013377292));
#24738=CARTESIAN_POINT('Ctrl Pts',(-4.85068927007173,-115.404517970998,
8.40164026752836));
#24739=CARTESIAN_POINT('Ctrl Pts',(1.5129078685785E-11,-115.229517970998,
8.40164026751963));
#24740=CARTESIAN_POINT('Ctrl Pts',(4.85068927010198,-115.054517970998,8.4016402675109));
#24741=CARTESIAN_POINT('Ctrl Pts',(7.27603390513785,-114.879517970998,4.20082013374672));
#24742=CARTESIAN_POINT('Ctrl Pts',(9.70137854017372,-114.704517970998,-1.74689612655491E-11));
#24743=CARTESIAN_POINT('Ctrl Pts',(7.27603390512273,-114.529517970998,-4.20082013377291));
#24744=CARTESIAN_POINT('Ctrl Pts',(4.85068927007173,-114.354517970998,-8.40164026752836));
#24745=CARTESIAN_POINT('Ctrl Pts',(-1.51301075899711E-11,-114.179517970998,
-8.40164026751963));
#24746=CARTESIAN_POINT('Ctrl Pts',(-4.85068927010199,-114.004517970998,
-8.4016402675109));
#24747=CARTESIAN_POINT('Ctrl Pts',(-7.27603390513785,-113.829517970998,
-4.20082013374671));
#24748=CARTESIAN_POINT('Ctrl Pts',(-9.70137854017372,-113.654517970998,
1.74701493417668E-11));
#24749=CARTESIAN_POINT('Ctrl Pts',(-7.27603390512272,-113.479517970998,
4.20082013377292));
#24750=CARTESIAN_POINT('Ctrl Pts',(-4.85068927007173,-113.304517970998,
8.40164026752836));
#24751=CARTESIAN_POINT('Ctrl Pts',(1.5129078685785E-11,-113.129517970998,
8.40164026751963));
#24752=CARTESIAN_POINT('Ctrl Pts',(4.85068927010198,-112.954517970998,8.4016402675109));
#24753=CARTESIAN_POINT('Ctrl Pts',(7.27603390513785,-112.779517970998,4.20082013374672));
#24754=CARTESIAN_POINT('Ctrl Pts',(9.70137854017372,-112.604517970998,-1.74689612655491E-11));
#24755=CARTESIAN_POINT('Ctrl Pts',(7.27603390512273,-112.429517970998,-4.20082013377291));
#24756=CARTESIAN_POINT('Ctrl Pts',(4.85068927007173,-112.254517970998,-8.40164026752836));
#24757=CARTESIAN_POINT('Ctrl Pts',(-1.51301075899711E-11,-112.079517970998,
-8.40164026751963));
#24758=CARTESIAN_POINT('Ctrl Pts',(-4.85068927010199,-111.904517970998,
-8.4016402675109));
#24759=CARTESIAN_POINT('Ctrl Pts',(-7.27603390513785,-111.729517970998,
-4.20082013374671));
#24760=CARTESIAN_POINT('Ctrl Pts',(-9.70137854017372,-111.554517970998,
1.74701493417668E-11));
#24761=CARTESIAN_POINT('Ctrl Pts',(-7.27603390512272,-111.379517970998,
4.20082013377292));
#24762=CARTESIAN_POINT('Ctrl Pts',(-4.85068927007173,-111.204517970998,
8.40164026752836));
#24763=CARTESIAN_POINT('Ctrl Pts',(1.5129078685785E-11,-111.029517970998,
8.40164026751963));
#24764=CARTESIAN_POINT('Ctrl Pts',(4.85068927010198,-110.854517970998,8.4016402675109));
#24765=CARTESIAN_POINT('Ctrl Pts',(7.27603390513785,-110.679517970998,4.20082013374672));
#24766=CARTESIAN_POINT('Ctrl Pts',(9.70137854017372,-110.504517970998,-1.74689612655491E-11));
#24767=CARTESIAN_POINT('Ctrl Pts',(7.27603390512273,-110.329517970998,-4.20082013377291));
#24768=CARTESIAN_POINT('Ctrl Pts',(4.85068927007173,-110.154517970998,-8.40164026752836));
#24769=CARTESIAN_POINT('Ctrl Pts',(-1.51301075899711E-11,-109.979517970998,
-8.40164026751963));
#24770=CARTESIAN_POINT('Ctrl Pts',(-4.85068927010199,-109.804517970998,
-8.4016402675109));
#24771=CARTESIAN_POINT('Ctrl Pts',(-7.27603390513785,-109.629517970998,
-4.20082013374671));
#24772=CARTESIAN_POINT('Ctrl Pts',(-9.70137854017372,-109.454517970998,
1.74701493417668E-11));
#24773=CARTESIAN_POINT('Ctrl Pts',(-7.27603390512272,-109.279517970998,
4.20082013377292));
#24774=CARTESIAN_POINT('Ctrl Pts',(-4.85068927007173,-109.104517970998,
8.40164026752836));
#24775=CARTESIAN_POINT('Ctrl Pts',(1.5129078685785E-11,-108.929517970998,
8.40164026751963));
#24776=CARTESIAN_POINT('Ctrl Pts',(4.85068927010198,-108.754517970998,8.4016402675109));
#24777=CARTESIAN_POINT('Ctrl Pts',(7.27603390513785,-108.579517970998,4.20082013374672));
#24778=CARTESIAN_POINT('Ctrl Pts',(9.70137854017372,-108.404517970998,-1.74689612655491E-11));
#24779=CARTESIAN_POINT('Ctrl Pts',(7.27603390512273,-108.229517970998,-4.20082013377291));
#24780=CARTESIAN_POINT('Ctrl Pts',(4.85068927007173,-108.054517970998,-8.40164026752836));
#24781=CARTESIAN_POINT('Ctrl Pts',(-1.51301075899711E-11,-107.879517970998,
-8.40164026751963));
#24782=CARTESIAN_POINT('Ctrl Pts',(-4.85068927010199,-107.704517970998,
-8.4016402675109));
#24783=CARTESIAN_POINT('Ctrl Pts',(-7.27603390513785,-107.529517970998,
-4.20082013374671));
#24784=CARTESIAN_POINT('Ctrl Pts',(-9.70137854017372,-107.354517970998,
1.74701493417668E-11));
#24785=CARTESIAN_POINT('Ctrl Pts',(-7.27603390512272,-107.179517970998,
4.20082013377292));
#24786=CARTESIAN_POINT('Ctrl Pts',(-4.85068927007173,-107.004517970998,
8.40164026752836));
#24787=CARTESIAN_POINT('Ctrl Pts',(1.5129078685785E-11,-106.829517970998,
8.40164026751963));
#24788=CARTESIAN_POINT('Ctrl Pts',(4.85068927010198,-106.654517970998,8.4016402675109));
#24789=CARTESIAN_POINT('Ctrl Pts',(7.27603390513785,-106.479517970998,4.20082013374672));
#24790=CARTESIAN_POINT('Ctrl Pts',(9.70137854017372,-106.304517970998,-1.74689612655491E-11));
#24791=CARTESIAN_POINT('Ctrl Pts',(7.27603390512273,-106.129517970998,-4.20082013377291));
#24792=CARTESIAN_POINT('Ctrl Pts',(4.85068927007173,-105.954517970998,-8.40164026752836));
#24793=CARTESIAN_POINT('Ctrl Pts',(-1.51301075899711E-11,-105.779517970998,
-8.40164026751963));
#24794=CARTESIAN_POINT('Ctrl Pts',(-4.85068927010199,-105.604517970998,
-8.4016402675109));
#24795=CARTESIAN_POINT('Ctrl Pts',(-7.27603390513785,-105.429517970998,
-4.20082013374671));
#24796=CARTESIAN_POINT('Ctrl Pts',(-9.70137854017372,-105.254517970998,
1.74701493417668E-11));
#24797=CARTESIAN_POINT('Ctrl Pts',(-7.27603390512272,-105.079517970998,
4.20082013377292));
#24798=CARTESIAN_POINT('Ctrl Pts',(-4.85068927007173,-104.904517970998,
8.40164026752836));
#24799=CARTESIAN_POINT('Ctrl Pts',(1.5129078685785E-11,-104.729517970998,
8.40164026751963));
#24800=CARTESIAN_POINT('Ctrl Pts',(4.85068927010198,-104.554517970998,8.4016402675109));
#24801=CARTESIAN_POINT('Ctrl Pts',(7.27603390513785,-104.379517970998,4.20082013374672));
#24802=CARTESIAN_POINT('Ctrl Pts',(9.70137854017372,-104.204517970998,-1.74689612655491E-11));
#24803=CARTESIAN_POINT('Ctrl Pts',(7.27603390512273,-104.029517970998,-4.20082013377291));
#24804=CARTESIAN_POINT('Ctrl Pts',(4.85068927007173,-103.854517970998,-8.40164026752836));
#24805=CARTESIAN_POINT('Ctrl Pts',(-1.51301075899711E-11,-103.679517970998,
-8.40164026751963));
#24806=CARTESIAN_POINT('Ctrl Pts',(-4.85068927010199,-103.504517970998,
-8.4016402675109));
#24807=CARTESIAN_POINT('Ctrl Pts',(-7.27603390513785,-103.329517970998,
-4.20082013374671));
#24808=CARTESIAN_POINT('Ctrl Pts',(-9.70137854017372,-103.154517970998,
1.74701493417668E-11));
#24809=CARTESIAN_POINT('Ctrl Pts',(-7.27603390512272,-102.979517970998,
4.20082013377292));
#24810=CARTESIAN_POINT('Ctrl Pts',(-4.85068927007173,-102.804517970998,
8.40164026752836));
#24811=CARTESIAN_POINT('Ctrl Pts',(1.5129078685785E-11,-102.629517970998,
8.40164026751963));
#24812=CARTESIAN_POINT('Ctrl Pts',(4.85068927010198,-102.454517970998,8.4016402675109));
#24813=CARTESIAN_POINT('Ctrl Pts',(7.27603390513785,-102.279517970998,4.20082013374672));
#24814=CARTESIAN_POINT('Ctrl Pts',(9.70137854017372,-102.104517970998,-1.74689612655491E-11));
#24815=CARTESIAN_POINT('Ctrl Pts',(7.27603390512273,-101.929517970998,-4.20082013377291));
#24816=CARTESIAN_POINT('Ctrl Pts',(4.85068927007173,-101.754517970998,-8.40164026752836));
#24817=CARTESIAN_POINT('Ctrl Pts',(-1.51301075899711E-11,-101.579517970998,
-8.40164026751963));
#24818=CARTESIAN_POINT('Ctrl Pts',(-4.85068927010199,-101.404517970998,
-8.4016402675109));
#24819=CARTESIAN_POINT('Ctrl Pts',(-7.27603390513785,-101.229517970998,
-4.20082013374671));
#24820=CARTESIAN_POINT('Ctrl Pts',(-9.70137854017372,-101.054517970998,
1.74701493417668E-11));
#24821=CARTESIAN_POINT('Ctrl Pts',(-7.27603390512272,-100.879517970998,
4.20082013377292));
#24822=CARTESIAN_POINT('Ctrl Pts',(-4.85068927007173,-100.704517970998,
8.40164026752836));
#24823=CARTESIAN_POINT('Ctrl Pts',(1.5129078685785E-11,-100.529517970998,
8.40164026751963));
#24824=CARTESIAN_POINT('Ctrl Pts',(4.85068927010198,-100.354517970998,8.4016402675109));
#24825=CARTESIAN_POINT('Ctrl Pts',(7.27603390513785,-100.179517970998,4.20082013374672));
#24826=CARTESIAN_POINT('Ctrl Pts',(9.70137854017372,-100.004517970998,-1.74689612655491E-11));
#24827=CARTESIAN_POINT('Ctrl Pts',(7.27603390512273,-99.8295179709984,-4.20082013377291));
#24828=CARTESIAN_POINT('Ctrl Pts',(4.85068927007173,-99.6545179709984,-8.40164026752836));
#24829=CARTESIAN_POINT('Ctrl Pts',(-1.51301075899711E-11,-99.4795179709984,
-8.40164026751963));
#24830=CARTESIAN_POINT('Ctrl Pts',(-4.85068927010199,-99.3045179709984,
-8.4016402675109));
#24831=CARTESIAN_POINT('Ctrl Pts',(-7.27603390513785,-99.1295179709984,
-4.20082013374671));
#24832=CARTESIAN_POINT('Ctrl Pts',(-9.70137854017372,-98.9545179709984,
1.74701493417668E-11));
#24833=CARTESIAN_POINT('Ctrl Pts',(-7.27603390512272,-98.7795179709984,
4.20082013377292));
#24834=CARTESIAN_POINT('Ctrl Pts',(-4.85068927007173,-98.6045179709984,
8.40164026752836));
#24835=CARTESIAN_POINT('Ctrl Pts',(1.5129078685785E-11,-98.4295179709984,
8.40164026751963));
#24836=CARTESIAN_POINT('Ctrl Pts',(4.85068927010198,-98.2545179709984,8.4016402675109));
#24837=CARTESIAN_POINT('Ctrl Pts',(7.27603390513785,-98.0795179709984,4.20082013374672));
#24838=CARTESIAN_POINT('Ctrl Pts',(9.70137854017372,-97.9045179709984,-1.74689612655491E-11));
#24839=CARTESIAN_POINT('Ctrl Pts',(7.27603390512273,-97.7295179709984,-4.20082013377291));
#24840=CARTESIAN_POINT('Ctrl Pts',(4.85068927007173,-97.5545179709984,-8.40164026752836));
#24841=CARTESIAN_POINT('Ctrl Pts',(-1.51301075899711E-11,-97.3795179709984,
-8.40164026751963));
#24842=CARTESIAN_POINT('Ctrl Pts',(-4.85068927010199,-97.2045179709984,
-8.4016402675109));
#24843=CARTESIAN_POINT('Ctrl Pts',(-7.27603390513785,-97.0295179709984,
-4.20082013374671));
#24844=CARTESIAN_POINT('Ctrl Pts',(-9.70137854017372,-96.8545179709984,
1.74701493417668E-11));
#24845=CARTESIAN_POINT('Ctrl Pts',(-7.27603390512272,-96.6795179709984,
4.20082013377292));
#24846=CARTESIAN_POINT('Ctrl Pts',(-4.85068927007173,-96.5045179709984,
8.40164026752836));
#24847=CARTESIAN_POINT('Ctrl Pts',(1.5129078685785E-11,-96.3295179709984,
8.40164026751963));
#24848=CARTESIAN_POINT('Ctrl Pts',(4.85068927010198,-96.1545179709984,8.4016402675109));
#24849=CARTESIAN_POINT('Ctrl Pts',(7.27603390513785,-95.9795179709984,4.20082013374672));
#24850=CARTESIAN_POINT('Ctrl Pts',(9.70137854017372,-95.8045179709984,-1.74689612655491E-11));
#24851=CARTESIAN_POINT('Ctrl Pts',(7.27603390512273,-95.6295179709984,-4.20082013377291));
#24852=CARTESIAN_POINT('Ctrl Pts',(4.85068927007173,-95.4545179709984,-8.40164026752836));
#24853=CARTESIAN_POINT('Ctrl Pts',(-1.51301075899711E-11,-95.2795179709984,
-8.40164026751963));
#24854=CARTESIAN_POINT('Ctrl Pts',(-4.85068927010199,-95.1045179709984,
-8.4016402675109));
#24855=CARTESIAN_POINT('Ctrl Pts',(-7.27603390513785,-94.9295179709984,
-4.20082013374671));
#24856=CARTESIAN_POINT('Ctrl Pts',(-9.70137854017372,-94.7545179709984,
1.74701493417668E-11));
#24857=CARTESIAN_POINT('Ctrl Pts',(-7.27603390512272,-94.5795179709984,
4.20082013377292));
#24858=CARTESIAN_POINT('Ctrl Pts',(-4.85068927007173,-94.4045179709984,
8.40164026752836));
#24859=CARTESIAN_POINT('Ctrl Pts',(1.5129078685785E-11,-94.2295179709984,
8.40164026751963));
#24860=CARTESIAN_POINT('Ctrl Pts',(4.85068927010198,-94.0545179709984,8.4016402675109));
#24861=CARTESIAN_POINT('Ctrl Pts',(7.27603390513785,-93.8795179709984,4.20082013374672));
#24862=CARTESIAN_POINT('Ctrl Pts',(9.70137854017372,-93.7045179709984,-1.74689612655491E-11));
#24863=CARTESIAN_POINT('Ctrl Pts',(7.27603390512273,-93.5295179709984,-4.20082013377291));
#24864=CARTESIAN_POINT('Ctrl Pts',(4.85068927007173,-93.3545179709984,-8.40164026752836));
#24865=CARTESIAN_POINT('Ctrl Pts',(-1.51301075899711E-11,-93.1795179709984,
-8.40164026751963));
#24866=CARTESIAN_POINT('Ctrl Pts',(-4.85068927010199,-93.0045179709984,
-8.4016402675109));
#24867=CARTESIAN_POINT('Ctrl Pts',(-7.27603390513785,-92.8295179709984,
-4.20082013374671));
#24868=CARTESIAN_POINT('Ctrl Pts',(-9.70137854017372,-92.6545179709984,
1.74701493417668E-11));
#24869=CARTESIAN_POINT('Ctrl Pts',(-7.27603390512272,-92.4795179709984,
4.20082013377292));
#24870=CARTESIAN_POINT('Ctrl Pts',(-4.85068927007173,-92.3045179709984,
8.40164026752836));
#24871=CARTESIAN_POINT('Ctrl Pts',(1.5129078685785E-11,-92.1295179709984,
8.40164026751963));
#24872=CARTESIAN_POINT('Ctrl Pts',(4.85068927010198,-91.9545179709984,8.4016402675109));
#24873=CARTESIAN_POINT('Ctrl Pts',(7.27603390513785,-91.7795179709984,4.20082013374672));
#24874=CARTESIAN_POINT('Ctrl Pts',(9.70137854017372,-91.6045179709984,-1.74689612655491E-11));
#24875=CARTESIAN_POINT('Ctrl Pts',(7.27603390512273,-91.4295179709984,-4.20082013377291));
#24876=CARTESIAN_POINT('Ctrl Pts',(4.85068927007173,-91.2545179709984,-8.40164026752836));
#24877=CARTESIAN_POINT('Ctrl Pts',(-1.51301075899711E-11,-91.0795179709984,
-8.40164026751963));
#24878=CARTESIAN_POINT('Ctrl Pts',(-4.85068927010199,-90.9045179709984,
-8.4016402675109));
#24879=CARTESIAN_POINT('Ctrl Pts',(-7.27603390513785,-90.7295179709984,
-4.20082013374671));
#24880=CARTESIAN_POINT('Ctrl Pts',(-9.70137854017372,-90.5545179709984,
1.74701493417668E-11));
#24881=CARTESIAN_POINT('Ctrl Pts',(-7.27603390512272,-90.3795179709984,
4.20082013377292));
#24882=CARTESIAN_POINT('Ctrl Pts',(-4.85068927007173,-90.2045179709984,
8.40164026752836));
#24883=CARTESIAN_POINT('Ctrl Pts',(1.5129078685785E-11,-90.0295179709984,
8.40164026751963));
#24884=CARTESIAN_POINT('Ctrl Pts',(4.85068927010198,-89.8545179709984,8.4016402675109));
#24885=CARTESIAN_POINT('Ctrl Pts',(7.27603390513785,-89.6795179709984,4.20082013374672));
#24886=CARTESIAN_POINT('Ctrl Pts',(9.70137854017372,-89.5045179709984,-1.74689612655491E-11));
#24887=CARTESIAN_POINT('Ctrl Pts',(7.27603390512273,-89.3295179709984,-4.20082013377291));
#24888=CARTESIAN_POINT('Ctrl Pts',(4.85068927007173,-89.1545179709984,-8.40164026752836));
#24889=CARTESIAN_POINT('Ctrl Pts',(-1.51301075899711E-11,-88.9795179709984,
-8.40164026751963));
#24890=CARTESIAN_POINT('Ctrl Pts',(-4.85068927010199,-88.8045179709984,
-8.4016402675109));
#24891=CARTESIAN_POINT('Ctrl Pts',(-7.27603390513785,-88.6295179709984,
-4.20082013374671));
#24892=CARTESIAN_POINT('Ctrl Pts',(-9.70137854017372,-88.4545179709984,
1.74701493417668E-11));
#24893=CARTESIAN_POINT('Ctrl Pts',(-7.27603390512272,-88.2795179709984,
4.20082013377292));
#24894=CARTESIAN_POINT('Ctrl Pts',(-4.85068927007173,-88.1045179709984,
8.40164026752836));
#24895=CARTESIAN_POINT('Ctrl Pts',(1.5129078685785E-11,-87.9295179709984,
8.40164026751963));
#24896=CARTESIAN_POINT('Ctrl Pts',(4.85068927010198,-87.7545179709984,8.4016402675109));
#24897=CARTESIAN_POINT('Ctrl Pts',(7.27603390513785,-87.5795179709984,4.20082013374672));
#24898=CARTESIAN_POINT('Ctrl Pts',(9.70137854017372,-87.4045179709984,-1.74689612655491E-11));
#24899=CARTESIAN_POINT('Ctrl Pts',(7.27603390512273,-87.2295179709984,-4.20082013377291));
#24900=CARTESIAN_POINT('Ctrl Pts',(4.85068927007173,-87.0545179709984,-8.40164026752836));
#24901=CARTESIAN_POINT('Ctrl Pts',(-1.51301075899711E-11,-86.8795179709984,
-8.40164026751963));
#24902=CARTESIAN_POINT('Ctrl Pts',(-4.85068927010199,-86.7045179709984,
-8.4016402675109));
#24903=CARTESIAN_POINT('Ctrl Pts',(-7.27603390513785,-86.5295179709984,
-4.20082013374671));
#24904=CARTESIAN_POINT('Ctrl Pts',(-9.70137854017372,-86.3545179709984,
1.74701493417668E-11));
#24905=CARTESIAN_POINT('Ctrl Pts',(-7.27603390512272,-86.1795179709984,
4.20082013377292));
#24906=CARTESIAN_POINT('Ctrl Pts',(-4.85068927007173,-86.0045179709984,
8.40164026752836));
#24907=CARTESIAN_POINT('Ctrl Pts',(1.5129078685785E-11,-85.8295179709984,
8.40164026751963));
#24908=CARTESIAN_POINT('Ctrl Pts',(4.85068927010198,-85.6545179709984,8.4016402675109));
#24909=CARTESIAN_POINT('Ctrl Pts',(7.27603390513785,-85.4795179709984,4.20082013374672));
#24910=CARTESIAN_POINT('Ctrl Pts',(9.70137854017372,-85.3045179709984,-1.74689612655491E-11));
#24911=CARTESIAN_POINT('Ctrl Pts',(7.27603390512273,-85.1295179709984,-4.20082013377291));
#24912=CARTESIAN_POINT('Ctrl Pts',(4.85068927007173,-84.9545179709984,-8.40164026752836));
#24913=CARTESIAN_POINT('Ctrl Pts',(-1.51301075899711E-11,-84.7795179709984,
-8.40164026751963));
#24914=CARTESIAN_POINT('Ctrl Pts',(-4.85068927010199,-84.6045179709984,
-8.4016402675109));
#24915=CARTESIAN_POINT('Ctrl Pts',(-7.27603390513785,-84.4295179709984,
-4.20082013374671));
#24916=CARTESIAN_POINT('Ctrl Pts',(-9.70137854017372,-84.2545179709984,
1.74701493417668E-11));
#24917=CARTESIAN_POINT('Ctrl Pts',(-7.27603390512272,-84.0795179709984,
4.20082013377292));
#24918=CARTESIAN_POINT('Ctrl Pts',(-4.85068927007173,-83.9045179709984,
8.40164026752836));
#24919=CARTESIAN_POINT('Ctrl Pts',(1.5129078685785E-11,-83.7295179709984,
8.40164026751963));
#24920=CARTESIAN_POINT('Ctrl Pts',(4.85068927010198,-83.5545179709984,8.4016402675109));
#24921=CARTESIAN_POINT('Ctrl Pts',(7.27603390513785,-83.3795179709984,4.20082013374672));
#24922=CARTESIAN_POINT('Ctrl Pts',(9.70137854017372,-83.2045179709984,-1.74689612655491E-11));
#24923=CARTESIAN_POINT('Ctrl Pts',(7.27603390512273,-83.0295179709984,-4.20082013377291));
#24924=CARTESIAN_POINT('Ctrl Pts',(4.85068927007173,-82.8545179709984,-8.40164026752836));
#24925=CARTESIAN_POINT('Ctrl Pts',(-1.51301075899711E-11,-82.6795179709984,
-8.40164026751963));
#24926=CARTESIAN_POINT('Ctrl Pts',(-4.85068927010199,-82.5045179709984,
-8.4016402675109));
#24927=CARTESIAN_POINT('Ctrl Pts',(-7.27603390513785,-82.3295179709984,
-4.20082013374671));
#24928=CARTESIAN_POINT('Ctrl Pts',(-9.70137854017372,-82.1545179709984,
1.74701493417668E-11));
#24929=CARTESIAN_POINT('Ctrl Pts',(-7.27603390512272,-81.9795179709984,
4.20082013377292));
#24930=CARTESIAN_POINT('Ctrl Pts',(-4.85068927007173,-81.8045179709984,
8.40164026752836));
#24931=CARTESIAN_POINT('Ctrl Pts',(1.5129078685785E-11,-81.6295179709984,
8.40164026751963));
#24932=CARTESIAN_POINT('Ctrl Pts',(4.85068927010198,-81.4545179709984,8.4016402675109));
#24933=CARTESIAN_POINT('Ctrl Pts',(7.27603390513785,-81.2795179709984,4.20082013374672));
#24934=CARTESIAN_POINT('Ctrl Pts',(9.70137854017372,-81.1045179709984,-1.74689612655491E-11));
#24935=CARTESIAN_POINT('Ctrl Pts',(7.27603390512273,-80.9295179709984,-4.20082013377291));
#24936=CARTESIAN_POINT('Ctrl Pts',(4.85068927007173,-80.7545179709984,-8.40164026752836));
#24937=CARTESIAN_POINT('Ctrl Pts',(-1.51301075899711E-11,-80.5795179709984,
-8.40164026751963));
#24938=CARTESIAN_POINT('Ctrl Pts',(-4.85068927010199,-80.4045179709985,
-8.4016402675109));
#24939=CARTESIAN_POINT('Ctrl Pts',(-7.27603390513785,-80.2295179709984,
-4.20082013374671));
#24940=CARTESIAN_POINT('Ctrl Pts',(-9.70137854017372,-80.0545179709984,
1.74701493417668E-11));
#24941=CARTESIAN_POINT('Ctrl Pts',(-7.27603390512272,-79.8795179709984,
4.20082013377292));
#24942=CARTESIAN_POINT('Ctrl Pts',(-4.85068927007173,-79.7045179709984,
8.40164026752836));
#24943=CARTESIAN_POINT('Ctrl Pts',(1.5129078685785E-11,-79.5295179709984,
8.40164026751963));
#24944=CARTESIAN_POINT('Ctrl Pts',(4.85068927010198,-79.3545179709984,8.4016402675109));
#24945=CARTESIAN_POINT('Ctrl Pts',(7.27603390513785,-79.1795179709984,4.20082013374672));
#24946=CARTESIAN_POINT('Ctrl Pts',(9.70137854017372,-79.0045179709984,-1.74689612655491E-11));
#24947=CARTESIAN_POINT('Ctrl Pts',(7.27603390512273,-78.8295179709984,-4.20082013377291));
#24948=CARTESIAN_POINT('Ctrl Pts',(4.85068927007173,-78.6545179709984,-8.40164026752836));
#24949=CARTESIAN_POINT('Ctrl Pts',(-1.51301075899711E-11,-78.4795179709984,
-8.40164026751963));
#24950=CARTESIAN_POINT('Ctrl Pts',(-4.85068927010199,-78.3045179709985,
-8.4016402675109));
#24951=CARTESIAN_POINT('Ctrl Pts',(-7.27603390513785,-78.1295179709984,
-4.20082013374671));
#24952=CARTESIAN_POINT('Ctrl Pts',(-9.70137854017372,-77.9545179709984,
1.74701493417668E-11));
#24953=CARTESIAN_POINT('Ctrl Pts',(-7.27603390512272,-77.7795179709984,
4.20082013377292));
#24954=CARTESIAN_POINT('Ctrl Pts',(-4.85068927007173,-77.6045179709984,
8.40164026752836));
#24955=CARTESIAN_POINT('Ctrl Pts',(1.5129078685785E-11,-77.4295179709984,
8.40164026751963));
#24956=CARTESIAN_POINT('Ctrl Pts',(4.85068927010198,-77.2545179709984,8.4016402675109));
#24957=CARTESIAN_POINT('Ctrl Pts',(7.27603390513785,-77.0795179709984,4.20082013374672));
#24958=CARTESIAN_POINT('Ctrl Pts',(9.70137854017372,-76.9045179709984,-1.74689612655491E-11));
#24959=CARTESIAN_POINT('Ctrl Pts',(7.27603390512273,-76.7295179709984,-4.20082013377291));
#24960=CARTESIAN_POINT('Ctrl Pts',(4.85068927007173,-76.5545179709984,-8.40164026752836));
#24961=CARTESIAN_POINT('Ctrl Pts',(-1.51301075899711E-11,-76.3795179709984,
-8.40164026751963));
#24962=CARTESIAN_POINT('Ctrl Pts',(-4.85068927010199,-76.2045179709985,
-8.4016402675109));
#24963=CARTESIAN_POINT('Ctrl Pts',(-7.27603390513785,-76.0295179709984,
-4.20082013374671));
#24964=CARTESIAN_POINT('Ctrl Pts',(-9.70137854017372,-75.8545179709985,
1.74701493417668E-11));
#24965=CARTESIAN_POINT('Ctrl Pts',(-7.27603390512272,-75.6795179709984,
4.20082013377292));
#24966=CARTESIAN_POINT('Ctrl Pts',(-4.85068927007173,-75.5045179709984,
8.40164026752836));
#24967=CARTESIAN_POINT('Ctrl Pts',(1.5129078685785E-11,-75.3295179709984,
8.40164026751963));
#24968=CARTESIAN_POINT('Ctrl Pts',(4.85068927010198,-75.1545179709984,8.4016402675109));
#24969=CARTESIAN_POINT('Ctrl Pts',(7.27603390513785,-74.9795179709984,4.20082013374672));
#24970=CARTESIAN_POINT('Ctrl Pts',(9.70137854017372,-74.8045179709984,-1.74689612655491E-11));
#24971=CARTESIAN_POINT('Ctrl Pts',(7.27603390512273,-74.6295179709984,-4.20082013377291));
#24972=CARTESIAN_POINT('Ctrl Pts',(4.85068927007173,-74.4545179709984,-8.40164026752836));
#24973=CARTESIAN_POINT('Ctrl Pts',(-1.51301075899711E-11,-74.2795179709984,
-8.40164026751963));
#24974=CARTESIAN_POINT('Ctrl Pts',(-4.85068927010199,-74.1045179709984,
-8.4016402675109));
#24975=CARTESIAN_POINT('Ctrl Pts',(-7.27603390513785,-73.9295179709984,
-4.20082013374671));
#24976=CARTESIAN_POINT('Ctrl Pts',(-9.70137854017372,-73.7545179709984,
1.74701493417668E-11));
#24977=CARTESIAN_POINT('Ctrl Pts',(-7.27603390512272,-73.5795179709984,
4.20082013377292));
#24978=CARTESIAN_POINT('Ctrl Pts',(-4.85068927007173,-73.4045179709984,
8.40164026752836));
#24979=CARTESIAN_POINT('Ctrl Pts',(1.5129078685785E-11,-73.2295179709984,
8.40164026751963));
#24980=CARTESIAN_POINT('Ctrl Pts',(4.85068927010198,-73.0545179709984,8.4016402675109));
#24981=CARTESIAN_POINT('Ctrl Pts',(7.27603390513785,-72.8795179709984,4.20082013374672));
#24982=CARTESIAN_POINT('Ctrl Pts',(9.70137854017372,-72.7045179709984,-1.74689612655491E-11));
#24983=CARTESIAN_POINT('Ctrl Pts',(7.27603390512273,-72.5295179709984,-4.20082013377291));
#24984=CARTESIAN_POINT('Ctrl Pts',(4.85068927007173,-72.3545179709984,-8.40164026752836));
#24985=CARTESIAN_POINT('Ctrl Pts',(-1.51301075899711E-11,-72.1795179709984,
-8.40164026751963));
#24986=CARTESIAN_POINT('Ctrl Pts',(-4.85068927010199,-72.0045179709984,
-8.4016402675109));
#24987=CARTESIAN_POINT('Ctrl Pts',(-7.27603390513785,-71.8295179709984,
-4.20082013374671));
#24988=CARTESIAN_POINT('Ctrl Pts',(-9.70137854017372,-71.6545179709985,
1.74701493417668E-11));
#24989=CARTESIAN_POINT('Ctrl Pts',(-7.27603390512272,-71.4795179709984,
4.20082013377292));
#24990=CARTESIAN_POINT('Ctrl Pts',(-4.85068927007173,-71.3045179709984,
8.40164026752836));
#24991=CARTESIAN_POINT('Ctrl Pts',(1.5129078685785E-11,-71.1295179709984,
8.40164026751963));
#24992=CARTESIAN_POINT('Ctrl Pts',(4.85068927010198,-70.9545179709984,8.4016402675109));
#24993=CARTESIAN_POINT('Ctrl Pts',(7.27603390513785,-70.7795179709984,4.20082013374672));
#24994=CARTESIAN_POINT('Ctrl Pts',(9.70137854017372,-70.6045179709985,-1.74689612655491E-11));
#24995=CARTESIAN_POINT('Ctrl Pts',(7.27603390512273,-70.4295179709984,-4.20082013377291));
#24996=CARTESIAN_POINT('Ctrl Pts',(4.85068927007173,-70.2545179709984,-8.40164026752836));
#24997=CARTESIAN_POINT('Ctrl Pts',(-1.51301075899711E-11,-70.0795179709985,
-8.40164026751963));
#24998=CARTESIAN_POINT('Ctrl Pts',(-4.85068927010199,-69.9045179709984,
-8.4016402675109));
#24999=CARTESIAN_POINT('Ctrl Pts',(-7.27603390513785,-69.7295179709984,
-4.20082013374671));
#25000=CARTESIAN_POINT('Ctrl Pts',(-9.70137854017372,-69.5545179709985,
1.74701493417668E-11));
#25001=CARTESIAN_POINT('Ctrl Pts',(-7.27603390512272,-69.3795179709984,
4.20082013377292));
#25002=CARTESIAN_POINT('Ctrl Pts',(-4.85068927007173,-69.2045179709985,
8.40164026752836));
#25003=CARTESIAN_POINT('Ctrl Pts',(1.5129078685785E-11,-69.0295179709985,
8.40164026751963));
#25004=CARTESIAN_POINT('Ctrl Pts',(4.85068927010198,-68.8545179709984,8.4016402675109));
#25005=CARTESIAN_POINT('Ctrl Pts',(7.27603390513785,-68.6795179709985,4.20082013374672));
#25006=CARTESIAN_POINT('Ctrl Pts',(9.70137854017372,-68.5045179709985,-1.74689612655491E-11));
#25007=CARTESIAN_POINT('Ctrl Pts',(7.27603390512273,-68.3295179709984,-4.20082013377291));
#25008=CARTESIAN_POINT('Ctrl Pts',(4.85068927007173,-68.1545179709985,-8.40164026752836));
#25009=CARTESIAN_POINT('Ctrl Pts',(-1.51301075899711E-11,-67.9795179709985,
-8.40164026751963));
#25010=CARTESIAN_POINT('Ctrl Pts',(-4.85068927010199,-67.8045179709984,
-8.4016402675109));
#25011=CARTESIAN_POINT('Ctrl Pts',(-7.27603390513785,-67.6295179709984,
-4.20082013374671));
#25012=CARTESIAN_POINT('Ctrl Pts',(-9.70137854017372,-67.4545179709985,
1.74701493417668E-11));
#25013=CARTESIAN_POINT('Ctrl Pts',(-7.27603390512272,-67.2795179709984,
4.20082013377292));
#25014=CARTESIAN_POINT('Ctrl Pts',(-4.85068927007173,-67.1045179709985,
8.40164026752836));
#25015=CARTESIAN_POINT('Ctrl Pts',(1.5129078685785E-11,-66.9295179709985,
8.40164026751963));
#25016=CARTESIAN_POINT('Ctrl Pts',(4.85068927010198,-66.7545179709984,8.4016402675109));
#25017=CARTESIAN_POINT('Ctrl Pts',(7.27603390513785,-66.5795179709985,4.20082013374672));
#25018=CARTESIAN_POINT('Ctrl Pts',(9.70137854017372,-66.4045179709985,-1.74689612655491E-11));
#25019=CARTESIAN_POINT('Ctrl Pts',(7.27603390512273,-66.2295179709984,-4.20082013377291));
#25020=CARTESIAN_POINT('Ctrl Pts',(4.85068927007173,-66.0545179709985,-8.40164026752836));
#25021=CARTESIAN_POINT('Ctrl Pts',(-1.51301075899711E-11,-65.8795179709984,
-8.40164026751963));
#25022=CARTESIAN_POINT('Ctrl Pts',(-4.85068927010199,-65.7045179709985,
-8.4016402675109));
#25023=CARTESIAN_POINT('Ctrl Pts',(-7.27603390513785,-65.5295179709985,
-4.20082013374671));
#25024=CARTESIAN_POINT('Ctrl Pts',(-9.70137854017372,-65.3545179709984,
1.74701493417668E-11));
#25025=CARTESIAN_POINT('Ctrl Pts',(-7.27603390512272,-65.1795179709984,
4.20082013377292));
#25026=CARTESIAN_POINT('Ctrl Pts',(-4.85068927007173,-65.0045179709985,
8.40164026752836));
#25027=CARTESIAN_POINT('Ctrl Pts',(1.5129078685785E-11,-64.8295179709985,
8.40164026751963));
#25028=CARTESIAN_POINT('Ctrl Pts',(4.85068927010198,-64.6545179709985,8.4016402675109));
#25029=CARTESIAN_POINT('Ctrl Pts',(7.27603390513785,-64.4795179709985,4.20082013374672));
#25030=CARTESIAN_POINT('Ctrl Pts',(9.70137854017372,-64.3045179709985,-1.74689612655491E-11));
#25031=CARTESIAN_POINT('Ctrl Pts',(7.27603390512273,-64.1295179709984,-4.20082013377291));
#25032=CARTESIAN_POINT('Ctrl Pts',(4.85068927007173,-63.9545179709985,-8.40164026752836));
#25033=CARTESIAN_POINT('Ctrl Pts',(-1.51301075899711E-11,-63.7795179709985,
-8.40164026751963));
#25034=CARTESIAN_POINT('Ctrl Pts',(-4.85068927010199,-63.6045179709985,
-8.4016402675109));
#25035=CARTESIAN_POINT('Ctrl Pts',(-7.27603390513785,-63.4295179709985,
-4.20082013374671));
#25036=CARTESIAN_POINT('Ctrl Pts',(-9.70137854017372,-63.2545179709985,
1.74701493417668E-11));
#25037=CARTESIAN_POINT('Ctrl Pts',(-7.27603390512272,-63.0795179709985,
4.20082013377292));
#25038=CARTESIAN_POINT('Ctrl Pts',(-4.85068927007173,-62.9045179709985,
8.40164026752836));
#25039=CARTESIAN_POINT('Ctrl Pts',(1.5129078685785E-11,-62.7295179709985,
8.40164026751963));
#25040=CARTESIAN_POINT('Ctrl Pts',(4.85068927010198,-62.5545179709985,8.4016402675109));
#25041=CARTESIAN_POINT('Ctrl Pts',(7.27603390513785,-62.3795179709985,4.20082013374672));
#25042=CARTESIAN_POINT('Ctrl Pts',(9.70137854017372,-62.2045179709985,-1.74689612655491E-11));
#25043=CARTESIAN_POINT('Ctrl Pts',(7.27603390512273,-62.0295179709985,-4.20082013377291));
#25044=CARTESIAN_POINT('Ctrl Pts',(4.85068927007173,-61.8545179709985,-8.40164026752836));
#25045=CARTESIAN_POINT('Ctrl Pts',(-1.51301075899711E-11,-61.6795179709985,
-8.40164026751963));
#25046=CARTESIAN_POINT('Ctrl Pts',(-4.85068927010199,-61.5045179709985,
-8.4016402675109));
#25047=CARTESIAN_POINT('Ctrl Pts',(-7.27603390513785,-61.3295179709985,
-4.20082013374671));
#25048=CARTESIAN_POINT('Ctrl Pts',(-9.70137854017372,-61.1545179709985,
1.74701493417668E-11));
#25049=CARTESIAN_POINT('Ctrl Pts',(-7.27603390512272,-60.9795179709985,
4.20082013377292));
#25050=CARTESIAN_POINT('Ctrl Pts',(-4.85068927007173,-60.8045179709985,
8.40164026752836));
#25051=CARTESIAN_POINT('Ctrl Pts',(1.5129078685785E-11,-60.6295179709985,
8.40164026751963));
#25052=CARTESIAN_POINT('Ctrl Pts',(4.85068927010198,-60.4545179709985,8.4016402675109));
#25053=CARTESIAN_POINT('Ctrl Pts',(7.27603390513785,-60.2795179709985,4.20082013374672));
#25054=CARTESIAN_POINT('Ctrl Pts',(9.70137854017372,-60.1045179709985,-1.74689612655491E-11));
#25055=CARTESIAN_POINT('Ctrl Pts',(7.27603390512273,-59.9295179709985,-4.20082013377291));
#25056=CARTESIAN_POINT('Ctrl Pts',(4.85068927007173,-59.7545179709985,-8.40164026752836));
#25057=CARTESIAN_POINT('Ctrl Pts',(-1.51301075899711E-11,-59.5795179709985,
-8.40164026751963));
#25058=CARTESIAN_POINT('Ctrl Pts',(-4.85068927010199,-59.4045179709985,
-8.4016402675109));
#25059=CARTESIAN_POINT('Ctrl Pts',(-7.27603390513785,-59.2295179709985,
-4.20082013374671));
#25060=CARTESIAN_POINT('Ctrl Pts',(-9.70137854017372,-59.0545179709985,
1.74701493417668E-11));
#25061=CARTESIAN_POINT('Ctrl Pts',(-7.27603390512272,-58.8795179709985,
4.20082013377292));
#25062=CARTESIAN_POINT('Ctrl Pts',(-4.85068927007173,-58.7045179709985,
8.40164026752836));
#25063=CARTESIAN_POINT('Ctrl Pts',(1.5129078685785E-11,-58.5295179709984,
8.40164026751963));
#25064=CARTESIAN_POINT('Ctrl Pts',(4.85068927010198,-58.3545179709985,8.4016402675109));
#25065=CARTESIAN_POINT('Ctrl Pts',(7.27603390513785,-58.1795179709985,4.20082013374672));
#25066=CARTESIAN_POINT('Ctrl Pts',(9.70137854017372,-58.0045179709985,-1.74689612655491E-11));
#25067=CARTESIAN_POINT('Ctrl Pts',(7.27603390512273,-57.8295179709985,-4.20082013377291));
#25068=CARTESIAN_POINT('Ctrl Pts',(4.85068927007173,-57.6545179709985,-8.40164026752836));
#25069=CARTESIAN_POINT('Ctrl Pts',(-1.51301075899711E-11,-57.4795179709985,
-8.40164026751963));
#25070=CARTESIAN_POINT('Ctrl Pts',(-4.85068927010199,-57.3045179709985,
-8.4016402675109));
#25071=CARTESIAN_POINT('Ctrl Pts',(-7.27603390513785,-57.1295179709985,
-4.20082013374671));
#25072=CARTESIAN_POINT('Ctrl Pts',(-9.70137854017372,-56.9545179709985,
1.74701493417668E-11));
#25073=CARTESIAN_POINT('Ctrl Pts',(-7.27603390512272,-56.7795179709985,
4.20082013377292));
#25074=CARTESIAN_POINT('Ctrl Pts',(-4.85068927007173,-56.6045179709985,
8.40164026752836));
#25075=CARTESIAN_POINT('Ctrl Pts',(1.5129078685785E-11,-56.4295179709985,
8.40164026751963));
#25076=CARTESIAN_POINT('Ctrl Pts',(4.85068927010198,-56.2545179709985,8.4016402675109));
#25077=CARTESIAN_POINT('Ctrl Pts',(7.27603390513785,-56.0795179709985,4.20082013374672));
#25078=CARTESIAN_POINT('Ctrl Pts',(9.70137854017372,-55.9045179709985,-1.74689612655491E-11));
#25079=CARTESIAN_POINT('Ctrl Pts',(7.27603390512273,-55.7295179709985,-4.20082013377291));
#25080=CARTESIAN_POINT('Ctrl Pts',(4.85068927007173,-55.5545179709985,-8.40164026752836));
#25081=CARTESIAN_POINT('Ctrl Pts',(-1.51301075899711E-11,-55.3795179709985,
-8.40164026751963));
#25082=CARTESIAN_POINT('Ctrl Pts',(-4.85068927010199,-55.2045179709985,
-8.4016402675109));
#25083=CARTESIAN_POINT('Ctrl Pts',(-7.27603390513785,-55.0295179709985,
-4.20082013374671));
#25084=CARTESIAN_POINT('Ctrl Pts',(-9.70137854017372,-54.8545179709985,
1.74701493417668E-11));
#25085=CARTESIAN_POINT('Ctrl Pts',(-7.27603390512272,-54.6795179709985,
4.20082013377292));
#25086=CARTESIAN_POINT('Ctrl Pts',(-4.85068927007173,-54.5045179709985,
8.40164026752836));
#25087=CARTESIAN_POINT('Ctrl Pts',(1.5129078685785E-11,-54.3295179709985,
8.40164026751963));
#25088=CARTESIAN_POINT('Ctrl Pts',(4.85068927010198,-54.1545179709985,8.4016402675109));
#25089=CARTESIAN_POINT('Ctrl Pts',(7.27603390513785,-53.9795179709985,4.20082013374672));
#25090=CARTESIAN_POINT('Ctrl Pts',(9.70137854017372,-53.8045179709985,-1.74689612655491E-11));
#25091=CARTESIAN_POINT('Ctrl Pts',(7.27603390512273,-53.6295179709985,-4.20082013377291));
#25092=CARTESIAN_POINT('Ctrl Pts',(4.85068927007173,-53.4545179709985,-8.40164026752836));
#25093=CARTESIAN_POINT('Ctrl Pts',(-1.51301075899711E-11,-53.2795179709985,
-8.40164026751963));
#25094=CARTESIAN_POINT('Ctrl Pts',(-4.85068927010199,-53.1045179709985,
-8.4016402675109));
#25095=CARTESIAN_POINT('Ctrl Pts',(-7.27603390513785,-52.9295179709985,
-4.20082013374671));
#25096=CARTESIAN_POINT('Ctrl Pts',(-9.70137854017372,-52.7545179709985,
1.74701493417668E-11));
#25097=CARTESIAN_POINT('Ctrl Pts',(-7.27603390512272,-52.5795179709985,
4.20082013377292));
#25098=CARTESIAN_POINT('Ctrl Pts',(-4.85068927007173,-52.4045179709985,
8.40164026752836));
#25099=CARTESIAN_POINT('Ctrl Pts',(1.5129078685785E-11,-52.2295179709985,
8.40164026751963));
#25100=CARTESIAN_POINT('Ctrl Pts',(4.85068927010198,-52.0545179709985,8.4016402675109));
#25101=CARTESIAN_POINT('Ctrl Pts',(7.27603390513785,-51.8795179709985,4.20082013374672));
#25102=CARTESIAN_POINT('Ctrl Pts',(9.70137854017372,-51.7045179709985,-1.74689612655491E-11));
#25103=CARTESIAN_POINT('Ctrl Pts',(7.27603390512273,-51.5295179709985,-4.20082013377291));
#25104=CARTESIAN_POINT('Ctrl Pts',(4.85068927007173,-51.3545179709985,-8.40164026752836));
#25105=CARTESIAN_POINT('Ctrl Pts',(-1.51301075899711E-11,-51.1795179709985,
-8.40164026751963));
#25106=CARTESIAN_POINT('Ctrl Pts',(-4.85068927010199,-51.0045179709985,
-8.4016402675109));
#25107=CARTESIAN_POINT('Ctrl Pts',(-7.27603390513785,-50.8295179709985,
-4.20082013374671));
#25108=CARTESIAN_POINT('Ctrl Pts',(-9.70137854017372,-50.6545179709985,
1.74701493417668E-11));
#25109=CARTESIAN_POINT('Ctrl Pts',(-7.27603390512272,-50.4795179709985,
4.20082013377292));
#25110=CARTESIAN_POINT('Ctrl Pts',(-4.85068927007173,-50.3045179709985,
8.40164026752836));
#25111=CARTESIAN_POINT('Ctrl Pts',(1.5129078685785E-11,-50.1295179709985,
8.40164026751963));
#25112=CARTESIAN_POINT('Ctrl Pts',(4.85068927010198,-49.9545179709985,8.4016402675109));
#25113=CARTESIAN_POINT('Ctrl Pts',(7.27603390513785,-49.7795179709985,4.20082013374672));
#25114=CARTESIAN_POINT('Ctrl Pts',(9.70137854017372,-49.6045179709985,-1.74689612655491E-11));
#25115=CARTESIAN_POINT('Ctrl Pts',(7.27603390512273,-49.4295179709985,-4.20082013377291));
#25116=CARTESIAN_POINT('Ctrl Pts',(4.85068927007173,-49.2545179709985,-8.40164026752836));
#25117=CARTESIAN_POINT('Ctrl Pts',(-1.51301075899711E-11,-49.0795179709985,
-8.40164026751963));
#25118=CARTESIAN_POINT('Ctrl Pts',(-4.85068927010199,-48.9045179709985,
-8.4016402675109));
#25119=CARTESIAN_POINT('Ctrl Pts',(-7.27603390513785,-48.7295179709985,
-4.20082013374671));
#25120=CARTESIAN_POINT('Ctrl Pts',(-9.70137854017372,-48.5545179709985,
1.74701493417668E-11));
#25121=CARTESIAN_POINT('Ctrl Pts',(-7.27603390512272,-48.3795179709985,
4.20082013377292));
#25122=CARTESIAN_POINT('Ctrl Pts',(-4.85068927007173,-48.2045179709985,
8.40164026752836));
#25123=CARTESIAN_POINT('Ctrl Pts',(1.5129078685785E-11,-48.0295179709985,
8.40164026751963));
#25124=CARTESIAN_POINT('Ctrl Pts',(4.85068927010198,-47.8545179709985,8.4016402675109));
#25125=CARTESIAN_POINT('Ctrl Pts',(7.27603390513785,-47.6795179709985,4.20082013374672));
#25126=CARTESIAN_POINT('Ctrl Pts',(9.70137854017372,-47.5045179709985,-1.74689612655491E-11));
#25127=CARTESIAN_POINT('Ctrl Pts',(7.27603390512273,-47.3295179709985,-4.20082013377291));
#25128=CARTESIAN_POINT('Ctrl Pts',(4.85068927007173,-47.1545179709985,-8.40164026752836));
#25129=CARTESIAN_POINT('Ctrl Pts',(-1.51301075899711E-11,-46.9795179709985,
-8.40164026751963));
#25130=CARTESIAN_POINT('Ctrl Pts',(-4.85068927010199,-46.8045179709985,
-8.4016402675109));
#25131=CARTESIAN_POINT('Ctrl Pts',(-7.27603390513785,-46.6295179709985,
-4.20082013374671));
#25132=CARTESIAN_POINT('Ctrl Pts',(-9.70137854017372,-46.4545179709985,
1.74701493417668E-11));
#25133=CARTESIAN_POINT('Ctrl Pts',(-7.27603390512272,-46.2795179709985,
4.20082013377292));
#25134=CARTESIAN_POINT('Ctrl Pts',(-4.85068927007173,-46.1045179709985,
8.40164026752836));
#25135=CARTESIAN_POINT('Ctrl Pts',(1.5129078685785E-11,-45.9295179709985,
8.40164026751963));
#25136=CARTESIAN_POINT('Ctrl Pts',(4.85068927010198,-45.7545179709985,8.4016402675109));
#25137=CARTESIAN_POINT('Ctrl Pts',(7.27603390513785,-45.5795179709985,4.20082013374672));
#25138=CARTESIAN_POINT('Ctrl Pts',(9.70137854017372,-45.4045179709985,-1.74689612655491E-11));
#25139=CARTESIAN_POINT('Ctrl Pts',(7.27603390512273,-45.2295179709985,-4.20082013377291));
#25140=CARTESIAN_POINT('Ctrl Pts',(4.85068927007173,-45.0545179709985,-8.40164026752836));
#25141=CARTESIAN_POINT('Ctrl Pts',(-1.51301075899711E-11,-44.8795179709985,
-8.40164026751963));
#25142=CARTESIAN_POINT('Ctrl Pts',(-4.85068927010199,-44.7045179709985,
-8.4016402675109));
#25143=CARTESIAN_POINT('Ctrl Pts',(-7.27603390513785,-44.5295179709985,
-4.20082013374671));
#25144=CARTESIAN_POINT('Ctrl Pts',(-9.70137854017372,-44.3545179709985,
1.74701493417668E-11));
#25145=CARTESIAN_POINT('Ctrl Pts',(-7.27603390512272,-44.1795179709985,
4.20082013377292));
#25146=CARTESIAN_POINT('Ctrl Pts',(-4.85068927007173,-44.0045179709985,
8.40164026752836));
#25147=CARTESIAN_POINT('Ctrl Pts',(1.5129078685785E-11,-43.8295179709985,
8.40164026751963));
#25148=CARTESIAN_POINT('Ctrl Pts',(4.85068927010198,-43.6545179709985,8.4016402675109));
#25149=CARTESIAN_POINT('Ctrl Pts',(7.27603390513785,-43.4795179709985,4.20082013374672));
#25150=CARTESIAN_POINT('Ctrl Pts',(9.70137854017372,-43.3045179709985,-1.74689612655491E-11));
#25151=CARTESIAN_POINT('Ctrl Pts',(7.27603390512273,-43.1295179709985,-4.20082013377291));
#25152=CARTESIAN_POINT('Ctrl Pts',(4.85068927007173,-42.9545179709985,-8.40164026752836));
#25153=CARTESIAN_POINT('Ctrl Pts',(-1.51301075899711E-11,-42.7795179709985,
-8.40164026751963));
#25154=CARTESIAN_POINT('Ctrl Pts',(-4.85068927010199,-42.6045179709985,
-8.4016402675109));
#25155=CARTESIAN_POINT('Ctrl Pts',(-7.27603390513785,-42.4295179709985,
-4.20082013374671));
#25156=CARTESIAN_POINT('Ctrl Pts',(-9.70137854017372,-42.2545179709985,
1.74701493417668E-11));
#25157=CARTESIAN_POINT('Ctrl Pts',(-7.27603390512272,-42.0795179709985,
4.20082013377292));
#25158=CARTESIAN_POINT('Ctrl Pts',(-4.85068927007173,-41.9045179709985,
8.40164026752836));
#25159=CARTESIAN_POINT('Ctrl Pts',(1.5129078685785E-11,-41.7295179709985,
8.40164026751963));
#25160=CARTESIAN_POINT('Ctrl Pts',(4.85068927010198,-41.5545179709985,8.4016402675109));
#25161=CARTESIAN_POINT('Ctrl Pts',(7.27603390513785,-41.3795179709985,4.20082013374672));
#25162=CARTESIAN_POINT('Ctrl Pts',(9.70137854017372,-41.2045179709985,-1.74689612655491E-11));
#25163=CARTESIAN_POINT('Ctrl Pts',(7.27603390512273,-41.0295179709985,-4.20082013377291));
#25164=CARTESIAN_POINT('Ctrl Pts',(4.85068927007173,-40.8545179709985,-8.40164026752836));
#25165=CARTESIAN_POINT('Ctrl Pts',(-1.51301075899711E-11,-40.6795179709985,
-8.40164026751963));
#25166=CARTESIAN_POINT('Ctrl Pts',(-4.85068927010199,-40.5045179709985,
-8.4016402675109));
#25167=CARTESIAN_POINT('Ctrl Pts',(-7.27603390513785,-40.3295179709985,
-4.20082013374671));
#25168=CARTESIAN_POINT('Ctrl Pts',(-9.70137854017372,-40.1545179709985,
1.74701493417668E-11));
#25169=CARTESIAN_POINT('Ctrl Pts',(-7.27603390512272,-39.9795179709985,
4.20082013377292));
#25170=CARTESIAN_POINT('Ctrl Pts',(-4.85068927007173,-39.8045179709985,
8.40164026752836));
#25171=CARTESIAN_POINT('Ctrl Pts',(1.5129078685785E-11,-39.6295179709985,
8.40164026751963));
#25172=CARTESIAN_POINT('Ctrl Pts',(4.85068927010198,-39.4545179709985,8.4016402675109));
#25173=CARTESIAN_POINT('Ctrl Pts',(7.27603390513785,-39.2795179709985,4.20082013374672));
#25174=CARTESIAN_POINT('Ctrl Pts',(9.70137854017372,-39.1045179709985,-1.74689612655491E-11));
#25175=CARTESIAN_POINT('Ctrl Pts',(7.27603390512273,-38.9295179709985,-4.20082013377291));
#25176=CARTESIAN_POINT('Ctrl Pts',(4.85068927007173,-38.7545179709985,-8.40164026752836));
#25177=CARTESIAN_POINT('Ctrl Pts',(-1.51301075899711E-11,-38.5795179709985,
-8.40164026751963));
#25178=CARTESIAN_POINT('Ctrl Pts',(-4.85068927010199,-38.4045179709985,
-8.4016402675109));
#25179=CARTESIAN_POINT('Ctrl Pts',(-7.27603390513785,-38.2295179709985,
-4.20082013374671));
#25180=CARTESIAN_POINT('Ctrl Pts',(-9.70137854017372,-38.0545179709985,
1.74701493417668E-11));
#25181=CARTESIAN_POINT('Ctrl Pts',(-7.27603390512272,-37.8795179709985,
4.20082013377292));
#25182=CARTESIAN_POINT('Ctrl Pts',(-4.85068927007173,-37.7045179709985,
8.40164026752836));
#25183=CARTESIAN_POINT('Ctrl Pts',(1.5129078685785E-11,-37.5295179709985,
8.40164026751963));
#25184=CARTESIAN_POINT('Ctrl Pts',(4.85068927010198,-37.3545179709985,8.4016402675109));
#25185=CARTESIAN_POINT('Ctrl Pts',(7.27603390513785,-37.1795179709985,4.20082013374672));
#25186=CARTESIAN_POINT('Ctrl Pts',(9.70137854017372,-37.0045179709985,-1.74689612655491E-11));
#25187=CARTESIAN_POINT('Ctrl Pts',(7.27603390512273,-36.8295179709985,-4.20082013377291));
#25188=CARTESIAN_POINT('Ctrl Pts',(4.85068927007173,-36.6545179709985,-8.40164026752836));
#25189=CARTESIAN_POINT('Ctrl Pts',(-1.51301075899711E-11,-36.4795179709985,
-8.40164026751963));
#25190=CARTESIAN_POINT('Ctrl Pts',(-4.85068927010199,-36.3045179709985,
-8.4016402675109));
#25191=CARTESIAN_POINT('Ctrl Pts',(-7.27603390513785,-36.1295179709985,
-4.20082013374671));
#25192=CARTESIAN_POINT('Ctrl Pts',(-9.70137854017372,-35.9545179709985,
1.74701493417668E-11));
#25193=CARTESIAN_POINT('Ctrl Pts',(-7.27603390512272,-35.7795179709985,
4.20082013377292));
#25194=CARTESIAN_POINT('Ctrl Pts',(-4.85068927007173,-35.6045179709985,
8.40164026752836));
#25195=CARTESIAN_POINT('Ctrl Pts',(1.5129078685785E-11,-35.4295179709985,
8.40164026751963));
#25196=CARTESIAN_POINT('Ctrl Pts',(4.85068927010198,-35.2545179709985,8.4016402675109));
#25197=CARTESIAN_POINT('Ctrl Pts',(7.27603390513785,-35.0795179709985,4.20082013374672));
#25198=CARTESIAN_POINT('Ctrl Pts',(9.70137854017372,-34.9045179709985,-1.74689612655491E-11));
#25199=CARTESIAN_POINT('Ctrl Pts',(7.27603390512273,-34.7295179709985,-4.20082013377291));
#25200=CARTESIAN_POINT('Ctrl Pts',(4.85068927007173,-34.5545179709985,-8.40164026752836));
#25201=CARTESIAN_POINT('Ctrl Pts',(-1.51301075899711E-11,-34.3795179709985,
-8.40164026751963));
#25202=CARTESIAN_POINT('Ctrl Pts',(-4.85068927010199,-34.2045179709985,
-8.4016402675109));
#25203=CARTESIAN_POINT('Ctrl Pts',(-7.27603390513785,-34.0295179709985,
-4.20082013374671));
#25204=CARTESIAN_POINT('Ctrl Pts',(-9.70137854017372,-33.8545179709985,
1.74701493417668E-11));
#25205=CARTESIAN_POINT('Ctrl Pts',(-7.27603390512272,-33.6795179709985,
4.20082013377292));
#25206=CARTESIAN_POINT('Ctrl Pts',(-4.85068927007173,-33.5045179709985,
8.40164026752836));
#25207=CARTESIAN_POINT('Ctrl Pts',(1.5129078685785E-11,-33.3295179709985,
8.40164026751963));
#25208=CARTESIAN_POINT('Ctrl Pts',(4.85068927010198,-33.1545179709985,8.4016402675109));
#25209=CARTESIAN_POINT('Ctrl Pts',(7.27603390513785,-32.9795179709985,4.20082013374672));
#25210=CARTESIAN_POINT('Ctrl Pts',(9.70137854017372,-32.8045179709985,-1.74689612655491E-11));
#25211=CARTESIAN_POINT('Ctrl Pts',(7.27603390512273,-32.6295179709985,-4.20082013377291));
#25212=CARTESIAN_POINT('Ctrl Pts',(4.85068927007173,-32.4545179709985,-8.40164026752836));
#25213=CARTESIAN_POINT('Ctrl Pts',(-1.51301075899711E-11,-32.2795179709985,
-8.40164026751963));
#25214=CARTESIAN_POINT('Ctrl Pts',(-4.85068927010199,-32.1045179709985,
-8.4016402675109));
#25215=CARTESIAN_POINT('Ctrl Pts',(-7.27603390513785,-31.9295179709985,
-4.20082013374671));
#25216=CARTESIAN_POINT('Ctrl Pts',(-9.70137854017372,-31.7545179709985,
1.74701493417668E-11));
#25217=CARTESIAN_POINT('Ctrl Pts',(-7.27603390512272,-31.5795179709985,
4.20082013377292));
#25218=CARTESIAN_POINT('Ctrl Pts',(-4.85068927007173,-31.4045179709985,
8.40164026752836));
#25219=CARTESIAN_POINT('Ctrl Pts',(1.5129078685785E-11,-31.2295179709985,
8.40164026751963));
#25220=CARTESIAN_POINT('Ctrl Pts',(4.85068927010198,-31.0545179709985,8.4016402675109));
#25221=CARTESIAN_POINT('Ctrl Pts',(7.27603390513785,-30.8795179709985,4.20082013374672));
#25222=CARTESIAN_POINT('Ctrl Pts',(9.70137854017372,-30.7045179709985,-1.74689612655491E-11));
#25223=CARTESIAN_POINT('Ctrl Pts',(7.27603390512273,-30.5295179709985,-4.20082013377291));
#25224=CARTESIAN_POINT('Ctrl Pts',(4.85068927007173,-30.3545179709985,-8.40164026752836));
#25225=CARTESIAN_POINT('Ctrl Pts',(-1.51301075899711E-11,-30.1795179709985,
-8.40164026751963));
#25226=CARTESIAN_POINT('Ctrl Pts',(-4.85068927010199,-30.0045179709985,
-8.4016402675109));
#25227=CARTESIAN_POINT('Ctrl Pts',(-7.27603390513785,-29.8295179709985,
-4.20082013374671));
#25228=CARTESIAN_POINT('Ctrl Pts',(-9.70137854017372,-29.6545179709985,
1.74701493417668E-11));
#25229=CARTESIAN_POINT('Ctrl Pts',(-7.27603390512272,-29.4795179709985,
4.20082013377292));
#25230=CARTESIAN_POINT('Ctrl Pts',(-4.85068927007173,-29.3045179709985,
8.40164026752836));
#25231=CARTESIAN_POINT('Ctrl Pts',(1.5129078685785E-11,-29.1295179709985,
8.40164026751963));
#25232=CARTESIAN_POINT('Ctrl Pts',(4.85068927010198,-28.9545179709986,8.4016402675109));
#25233=CARTESIAN_POINT('Ctrl Pts',(7.27603390513785,-28.7795179709985,4.20082013374672));
#25234=CARTESIAN_POINT('Ctrl Pts',(9.70137854017372,-28.6045179709986,-1.74689612655491E-11));
#25235=CARTESIAN_POINT('Ctrl Pts',(7.27603390512273,-28.4295179709985,-4.20082013377291));
#25236=CARTESIAN_POINT('Ctrl Pts',(4.85068927007173,-28.2545179709985,-8.40164026752836));
#25237=CARTESIAN_POINT('Ctrl Pts',(-1.51301075899711E-11,-28.0795179709985,
-8.40164026751963));
#25238=CARTESIAN_POINT('Ctrl Pts',(-4.85068927010199,-27.9045179709985,
-8.4016402675109));
#25239=CARTESIAN_POINT('Ctrl Pts',(-7.27603390513785,-27.7295179709985,
-4.20082013374671));
#25240=CARTESIAN_POINT('Ctrl Pts',(-9.70137854017372,-27.5545179709986,
1.74701493417668E-11));
#25241=CARTESIAN_POINT('Ctrl Pts',(-7.27603390512272,-27.3795179709985,
4.20082013377292));
#25242=CARTESIAN_POINT('Ctrl Pts',(-4.85068927007173,-27.2045179709986,
8.40164026752836));
#25243=CARTESIAN_POINT('Ctrl Pts',(1.5129078685785E-11,-27.0295179709986,
8.40164026751963));
#25244=CARTESIAN_POINT('Ctrl Pts',(4.85068927010198,-26.8545179709985,8.4016402675109));
#25245=CARTESIAN_POINT('Ctrl Pts',(7.27603390513785,-26.6795179709985,4.20082013374672));
#25246=CARTESIAN_POINT('Ctrl Pts',(9.70137854017372,-26.5045179709986,-1.74689612655491E-11));
#25247=CARTESIAN_POINT('Ctrl Pts',(7.27603390512273,-26.3295179709985,-4.20082013377291));
#25248=CARTESIAN_POINT('Ctrl Pts',(4.85068927007173,-26.1545179709986,-8.40164026752836));
#25249=CARTESIAN_POINT('Ctrl Pts',(-1.51301075899711E-11,-25.9795179709985,
-8.40164026751963));
#25250=CARTESIAN_POINT('Ctrl Pts',(-4.85068927010199,-25.8045179709985,
-8.4016402675109));
#25251=CARTESIAN_POINT('Ctrl Pts',(-7.27603390513785,-25.6295179709985,
-4.20082013374671));
#25252=CARTESIAN_POINT('Ctrl Pts',(-9.70137854017372,-25.4545179709985,
1.74701493417668E-11));
#25253=CARTESIAN_POINT('Ctrl Pts',(-7.27603390512272,-25.2795179709985,
4.20082013377292));
#25254=CARTESIAN_POINT('Ctrl Pts',(-4.85068927007173,-25.1045179709986,
8.40164026752836));
#25255=CARTESIAN_POINT('Ctrl Pts',(1.5129078685785E-11,-24.9295179709985,
8.40164026751963));
#25256=CARTESIAN_POINT('Ctrl Pts',(4.85068927010198,-24.7545179709985,8.4016402675109));
#25257=CARTESIAN_POINT('Ctrl Pts',(7.27603390513785,-24.5795179709986,4.20082013374672));
#25258=CARTESIAN_POINT('Ctrl Pts',(9.70137854017372,-24.4045179709986,-1.74689612655491E-11));
#25259=CARTESIAN_POINT('Ctrl Pts',(7.27603390512273,-24.2295179709986,-4.20082013377291));
#25260=CARTESIAN_POINT('Ctrl Pts',(4.85068927007173,-24.0545179709986,-8.40164026752836));
#25261=CARTESIAN_POINT('Ctrl Pts',(-1.51301075899711E-11,-23.8795179709986,
-8.40164026751963));
#25262=CARTESIAN_POINT('Ctrl Pts',(-4.85068927010199,-23.7045179709986,
-8.4016402675109));
#25263=CARTESIAN_POINT('Ctrl Pts',(-7.27603390513785,-23.5295179709985,
-4.20082013374671));
#25264=CARTESIAN_POINT('Ctrl Pts',(-9.70137854017372,-23.3545179709986,
1.74701493417668E-11));
#25265=CARTESIAN_POINT('Ctrl Pts',(-7.27603390512272,-23.1795179709986,
4.20082013377292));
#25266=CARTESIAN_POINT('Ctrl Pts',(-4.85068927007173,-23.0045179709986,
8.40164026752836));
#25267=CARTESIAN_POINT('Ctrl Pts',(1.5129078685785E-11,-22.8295179709986,
8.40164026751963));
#25268=CARTESIAN_POINT('Ctrl Pts',(4.85068927010198,-22.6545179709986,8.4016402675109));
#25269=CARTESIAN_POINT('Ctrl Pts',(7.27603390513785,-22.4795179709986,4.20082013374672));
#25270=CARTESIAN_POINT('Ctrl Pts',(9.70137854017372,-22.3045179709986,-1.74689612655491E-11));
#25271=CARTESIAN_POINT('Ctrl Pts',(7.27603390512273,-22.1295179709986,-4.20082013377291));
#25272=CARTESIAN_POINT('Ctrl Pts',(4.85068927007173,-21.9545179709986,-8.40164026752836));
#25273=CARTESIAN_POINT('Ctrl Pts',(-1.51301075899711E-11,-21.7795179709986,
-8.40164026751963));
#25274=CARTESIAN_POINT('Ctrl Pts',(-4.85068927010199,-21.6045179709986,
-8.4016402675109));
#25275=CARTESIAN_POINT('Ctrl Pts',(-7.27603390513785,-21.4295179709986,
-4.20082013374671));
#25276=CARTESIAN_POINT('Ctrl Pts',(-9.70137854017372,-21.2545179709986,
1.74701493417668E-11));
#25277=CARTESIAN_POINT('Ctrl Pts',(-7.27603390512272,-21.0795179709986,
4.20082013377292));
#25278=CARTESIAN_POINT('Ctrl Pts',(-4.85068927007173,-20.9045179709986,
8.40164026752836));
#25279=CARTESIAN_POINT('Ctrl Pts',(1.5129078685785E-11,-20.7295179709986,
8.40164026751963));
#25280=CARTESIAN_POINT('Ctrl Pts',(4.85068927010198,-20.5545179709986,8.4016402675109));
#25281=CARTESIAN_POINT('Ctrl Pts',(7.27603390513785,-20.3795179709986,4.20082013374672));
#25282=CARTESIAN_POINT('Ctrl Pts',(9.70137854017372,-20.2045179709986,-1.74689612655491E-11));
#25283=CARTESIAN_POINT('Ctrl Pts',(7.27603390512273,-20.0295179709986,-4.20082013377291));
#25284=CARTESIAN_POINT('Ctrl Pts',(4.85068927007173,-19.8545179709986,-8.40164026752836));
#25285=CARTESIAN_POINT('Ctrl Pts',(-1.51301075899711E-11,-19.6795179709986,
-8.40164026751963));
#25286=CARTESIAN_POINT('Ctrl Pts',(-4.85068927010199,-19.5045179709986,
-8.4016402675109));
#25287=CARTESIAN_POINT('Ctrl Pts',(-7.27603390513785,-19.3295179709986,
-4.20082013374671));
#25288=CARTESIAN_POINT('Ctrl Pts',(-9.70137854017372,-19.1545179709986,
1.74701493417668E-11));
#25289=CARTESIAN_POINT('Ctrl Pts',(-7.27603390512272,-18.9795179709986,
4.20082013377292));
#25290=CARTESIAN_POINT('Ctrl Pts',(-4.85068927007173,-18.8045179709986,
8.40164026752836));
#25291=CARTESIAN_POINT('Ctrl Pts',(1.5129078685785E-11,-18.6295179709986,
8.40164026751963));
#25292=CARTESIAN_POINT('Ctrl Pts',(4.85068927010198,-18.4545179709986,8.4016402675109));
#25293=CARTESIAN_POINT('Ctrl Pts',(7.27603390513785,-18.2795179709986,4.20082013374672));
#25294=CARTESIAN_POINT('Ctrl Pts',(9.70137854017372,-18.1045179709986,-1.74689612655491E-11));
#25295=CARTESIAN_POINT('Ctrl Pts',(7.27603390512273,-17.9295179709986,-4.20082013377291));
#25296=CARTESIAN_POINT('Ctrl Pts',(4.85068927007173,-17.7545179709986,-8.40164026752836));
#25297=CARTESIAN_POINT('Ctrl Pts',(-1.51301075899711E-11,-17.5795179709986,
-8.40164026751963));
#25298=CARTESIAN_POINT('Ctrl Pts',(-4.85068927010199,-17.4045179709986,
-8.4016402675109));
#25299=CARTESIAN_POINT('Ctrl Pts',(-7.27603390513785,-17.2295179709986,
-4.20082013374671));
#25300=CARTESIAN_POINT('Ctrl Pts',(-9.70137854017372,-17.0545179709986,
1.74701493417668E-11));
#25301=CARTESIAN_POINT('Ctrl Pts',(-7.27603390512272,-16.8795179709986,
4.20082013377292));
#25302=CARTESIAN_POINT('Ctrl Pts',(-4.85068927007173,-16.7045179709986,
8.40164026752836));
#25303=CARTESIAN_POINT('Ctrl Pts',(1.5129078685785E-11,-16.5295179709986,
8.40164026751963));
#25304=CARTESIAN_POINT('Ctrl Pts',(4.85068927010198,-16.3545179709986,8.4016402675109));
#25305=CARTESIAN_POINT('Ctrl Pts',(7.27603390513785,-16.1795179709986,4.20082013374672));
#25306=CARTESIAN_POINT('Ctrl Pts',(9.70137854017372,-16.0045179709986,-1.74689612655491E-11));
#25307=CARTESIAN_POINT('Ctrl Pts',(7.27603390512273,-15.8295179709986,-4.20082013377291));
#25308=CARTESIAN_POINT('Ctrl Pts',(4.85068927007173,-15.6545179709986,-8.40164026752836));
#25309=CARTESIAN_POINT('Ctrl Pts',(-1.51301075899711E-11,-15.4795179709986,
-8.40164026751963));
#25310=CARTESIAN_POINT('Ctrl Pts',(-4.85068927010199,-15.3045179709986,
-8.4016402675109));
#25311=CARTESIAN_POINT('Ctrl Pts',(-7.27603390513785,-15.1295179709986,
-4.20082013374671));
#25312=CARTESIAN_POINT('Ctrl Pts',(-9.70137854017372,-14.9545179709986,
1.74701493417668E-11));
#25313=CARTESIAN_POINT('Ctrl Pts',(-7.27603390512272,-14.7795179709986,
4.20082013377292));
#25314=CARTESIAN_POINT('Ctrl Pts',(-4.85068927007173,-14.6045179709986,
8.40164026752836));
#25315=CARTESIAN_POINT('Ctrl Pts',(1.5129078685785E-11,-14.4295179709986,
8.40164026751963));
#25316=CARTESIAN_POINT('Ctrl Pts',(4.85068927010198,-14.2545179709986,8.4016402675109));
#25317=CARTESIAN_POINT('Ctrl Pts',(7.27603390513785,-14.0795179709986,4.20082013374672));
#25318=CARTESIAN_POINT('Ctrl Pts',(9.70137854017372,-13.9045179709986,-1.74689612655491E-11));
#25319=CARTESIAN_POINT('Ctrl Pts',(7.27603390512273,-13.7295179709986,-4.20082013377291));
#25320=CARTESIAN_POINT('Ctrl Pts',(4.85068927007173,-13.5545179709986,-8.40164026752836));
#25321=CARTESIAN_POINT('Ctrl Pts',(-1.51301075899711E-11,-13.3795179709986,
-8.40164026751963));
#25322=CARTESIAN_POINT('Ctrl Pts',(-4.85068927010199,-13.2045179709986,
-8.4016402675109));
#25323=CARTESIAN_POINT('Ctrl Pts',(-7.27603390513785,-13.0295179709986,
-4.20082013374671));
#25324=CARTESIAN_POINT('Ctrl Pts',(-9.70137854017372,-12.8545179709986,
1.74701493417668E-11));
#25325=CARTESIAN_POINT('Ctrl Pts',(-7.27603390512272,-12.6795179709986,
4.20082013377292));
#25326=CARTESIAN_POINT('Ctrl Pts',(-4.85068927007173,-12.5045179709986,
8.40164026752836));
#25327=CARTESIAN_POINT('Ctrl Pts',(1.5129078685785E-11,-12.3295179709986,
8.40164026751963));
#25328=CARTESIAN_POINT('Ctrl Pts',(4.85068927010198,-12.1545179709986,8.4016402675109));
#25329=CARTESIAN_POINT('Ctrl Pts',(7.27603390513785,-11.9795179709986,4.20082013374672));
#25330=CARTESIAN_POINT('Ctrl Pts',(9.70137854017372,-11.8045179709986,-1.74689612655491E-11));
#25331=CARTESIAN_POINT('Ctrl Pts',(7.27603390512273,-11.6295179709986,-4.20082013377291));
#25332=CARTESIAN_POINT('Ctrl Pts',(4.85068927007173,-11.4545179709986,-8.40164026752836));
#25333=CARTESIAN_POINT('Ctrl Pts',(-1.51301075899711E-11,-11.2795179709986,
-8.40164026751963));
#25334=CARTESIAN_POINT('Ctrl Pts',(-4.85068927010199,-11.1045179709986,
-8.4016402675109));
#25335=CARTESIAN_POINT('Ctrl Pts',(-7.27603390513785,-10.9295179709986,
-4.20082013374671));
#25336=CARTESIAN_POINT('Ctrl Pts',(-9.70137854017372,-10.7545179709986,
1.74701493417668E-11));
#25337=CARTESIAN_POINT('Ctrl Pts',(-7.27603390512272,-10.5795179709986,
4.20082013377292));
#25338=CARTESIAN_POINT('Ctrl Pts',(-4.85068927007173,-10.4045179709986,
8.40164026752836));
#25339=CARTESIAN_POINT('Ctrl Pts',(1.5129078685785E-11,-10.2295179709986,
8.40164026751963));
#25340=CARTESIAN_POINT('Ctrl Pts',(4.85068927010198,-10.0545179709986,8.4016402675109));
#25341=CARTESIAN_POINT('Ctrl Pts',(7.27603390513785,-9.87951797099859,4.20082013374672));
#25342=CARTESIAN_POINT('Ctrl Pts',(9.70137854017372,-9.70451797099858,-1.74689612655491E-11));
#25343=CARTESIAN_POINT('Ctrl Pts',(7.27603390512273,-9.52951797099857,-4.20082013377291));
#25344=CARTESIAN_POINT('Ctrl Pts',(4.85068927007173,-9.3545179709986,-8.40164026752836));
#25345=CARTESIAN_POINT('Ctrl Pts',(-1.51301075899711E-11,-9.17951797099859,
-8.40164026751963));
#25346=CARTESIAN_POINT('Ctrl Pts',(-4.85068927010199,-9.00451797099858,
-8.4016402675109));
#25347=CARTESIAN_POINT('Ctrl Pts',(-7.27603390513785,-8.8295179709986,-4.20082013374671));
#25348=CARTESIAN_POINT('Ctrl Pts',(-9.70137854017372,-8.65451797099859,
1.74701493417668E-11));
#25349=CARTESIAN_POINT('Ctrl Pts',(-7.27603390512272,-8.47951797099858,
4.20082013377292));
#25350=CARTESIAN_POINT('Ctrl Pts',(-4.85068927007173,-8.3045179709986,8.40164026752836));
#25351=CARTESIAN_POINT('Ctrl Pts',(1.5129078685785E-11,-8.12951797099859,
8.40164026751963));
#25352=CARTESIAN_POINT('Ctrl Pts',(4.85068927010198,-7.95451797099859,8.4016402675109));
#25353=CARTESIAN_POINT('Ctrl Pts',(7.27603390513785,-7.7795179709986,4.20082013374672));
#25354=CARTESIAN_POINT('Ctrl Pts',(9.70137854017372,-7.60451797099859,-1.74689612655491E-11));
#25355=CARTESIAN_POINT('Ctrl Pts',(7.27603390512273,-7.42951797099858,-4.20082013377291));
#25356=CARTESIAN_POINT('Ctrl Pts',(4.85068927007173,-7.25451797099861,-8.40164026752836));
#25357=CARTESIAN_POINT('Ctrl Pts',(-1.51301075899711E-11,-7.07951797099859,
-8.40164026751963));
#25358=CARTESIAN_POINT('Ctrl Pts',(-4.85068927010199,-6.90451797099859,
-8.4016402675109));
#25359=CARTESIAN_POINT('Ctrl Pts',(-7.27603390513785,-6.72951797099858,
-4.20082013374671));
#25360=CARTESIAN_POINT('Ctrl Pts',(-9.70137854017372,-6.5545179709986,1.74701493417668E-11));
#25361=CARTESIAN_POINT('Ctrl Pts',(-7.27603390512272,-6.37951797099859,
4.20082013377292));
#25362=CARTESIAN_POINT('Ctrl Pts',(-4.85068927007173,-6.20451797099858,
8.40164026752836));
#25363=CARTESIAN_POINT('Ctrl Pts',(1.5129078685785E-11,-6.0295179709986,
8.40164026751963));
#25364=CARTESIAN_POINT('Ctrl Pts',(4.85068927010198,-5.8545179709986,8.4016402675109));
#25365=CARTESIAN_POINT('Ctrl Pts',(7.27603390513785,-5.67951797099858,4.20082013374672));
#25366=CARTESIAN_POINT('Ctrl Pts',(9.70137854017372,-5.5045179709986,-1.74689612655491E-11));
#25367=CARTESIAN_POINT('Ctrl Pts',(7.27603390512273,-5.32951797099859,-4.20082013377291));
#25368=CARTESIAN_POINT('Ctrl Pts',(4.85068927007173,-5.15451797099859,-8.40164026752836));
#25369=CARTESIAN_POINT('Ctrl Pts',(-1.51301075899711E-11,-4.9795179709986,
-8.40164026751963));
#25370=CARTESIAN_POINT('Ctrl Pts',(-4.85068927010199,-4.8045179709986,-8.4016402675109));
#25371=CARTESIAN_POINT('Ctrl Pts',(-7.27603390513785,-4.62951797099859,
-4.20082013374671));
#25372=CARTESIAN_POINT('Ctrl Pts',(-9.70137854017372,-4.45451797099861,
1.74701493417668E-11));
#25373=CARTESIAN_POINT('Ctrl Pts',(-7.27603390512272,-4.2795179709986,4.20082013377292));
#25374=CARTESIAN_POINT('Ctrl Pts',(-4.85068927007173,-4.10451797099859,
8.40164026752836));
#25375=CARTESIAN_POINT('Ctrl Pts',(1.5129078685785E-11,-3.92951797099861,
8.40164026751963));
#25376=CARTESIAN_POINT('Ctrl Pts',(4.85068927010198,-3.75451797099861,8.4016402675109));
#25377=CARTESIAN_POINT('Ctrl Pts',(7.27603390513785,-3.57951797099859,4.20082013374672));
#25378=CARTESIAN_POINT('Ctrl Pts',(9.70137854017372,-3.40451797099861,-1.74689612655491E-11));
#25379=CARTESIAN_POINT('Ctrl Pts',(7.27603390512273,-3.2295179709986,-4.20082013377291));
#25380=CARTESIAN_POINT('Ctrl Pts',(4.85068927007173,-3.0545179709986,-8.40164026752836));
#25381=CARTESIAN_POINT('Ctrl Pts',(-1.51301075899711E-11,-2.87951797099861,
-8.40164026751963));
#25382=CARTESIAN_POINT('Ctrl Pts',(-4.85068927010199,-2.70451797099861,
-8.4016402675109));
#25383=CARTESIAN_POINT('Ctrl Pts',(-7.27603390513785,-2.5295179709986,-4.20082013374671));
#25384=CARTESIAN_POINT('Ctrl Pts',(-9.70137854017372,-2.3545179709986,1.74701493417668E-11));
#25385=CARTESIAN_POINT('Ctrl Pts',(-7.27603390512272,-2.17951797099861,
4.20082013377292));
#25386=CARTESIAN_POINT('Ctrl Pts',(-4.85068927007173,-2.0045179709986,8.40164026752836));
#25387=CARTESIAN_POINT('Ctrl Pts',(1.5129078685785E-11,-1.82951797099859,
8.40164026751963));
#25388=CARTESIAN_POINT('Ctrl Pts',(4.85068927010198,-1.65451797099861,8.4016402675109));
#25389=CARTESIAN_POINT('Ctrl Pts',(7.27603390513785,-1.4795179709986,4.20082013374672));
#25390=CARTESIAN_POINT('Ctrl Pts',(9.70137854017372,-1.3045179709986,-1.74689612655491E-11));
#25391=CARTESIAN_POINT('Ctrl Pts',(7.27603390512273,-1.12951797099861,-4.20082013377291));
#25392=CARTESIAN_POINT('Ctrl Pts',(4.85068927007173,-0.954517970998605,
-8.40164026752836));
#25393=CARTESIAN_POINT('Ctrl Pts',(-1.51301075899711E-11,-0.779517970998594,
-8.40164026751963));
#25394=CARTESIAN_POINT('Ctrl Pts',(-4.85068927010199,-0.604517970998614,
-8.4016402675109));
#25395=CARTESIAN_POINT('Ctrl Pts',(-7.27603390513785,-0.429517970998605,
-4.20082013374671));
#25396=CARTESIAN_POINT('Ctrl Pts',(-9.70137854017372,-0.2545179709986,1.74701493417668E-11));
#25397=CARTESIAN_POINT('Ctrl Pts',(-7.27603390512272,-0.079517970998616,
4.20082013377292));
#25398=CARTESIAN_POINT('Ctrl Pts',(-4.85068927007173,0.0954820290013905,
8.40164026752836));
#25399=CARTESIAN_POINT('Ctrl Pts',(1.5129078685785E-11,0.270482029001401,
8.40164026751963));
#25400=CARTESIAN_POINT('Ctrl Pts',(4.85068927010198,0.445482029001381,8.4016402675109));
#25401=CARTESIAN_POINT('Ctrl Pts',(7.27603390513785,0.62048202900139,4.20082013374672));
#25402=CARTESIAN_POINT('Ctrl Pts',(9.70137854017372,0.795482029001395,-1.74689612655491E-11));
#25403=CARTESIAN_POINT('Ctrl Pts',(7.27603390512273,0.970482029001379,-4.20082013377291));
#25404=CARTESIAN_POINT('Ctrl Pts',(4.85068927007173,1.14548202900139,-8.40164026752836));
#25405=CARTESIAN_POINT('Ctrl Pts',(-1.51301075899711E-11,1.3204820290014,
-8.40164026751963));
#25406=CARTESIAN_POINT('Ctrl Pts',(-4.85068927010199,1.49548202900138,-8.4016402675109));
#25407=CARTESIAN_POINT('Ctrl Pts',(-7.27603390513785,1.67048202900139,-4.20082013374671));
#25408=CARTESIAN_POINT('Ctrl Pts',(-9.70137854017372,1.84548202900139,1.74701493417668E-11));
#25409=CARTESIAN_POINT('Ctrl Pts',(-7.27603390512272,2.0204820290014,4.20082013377292));
#25410=CARTESIAN_POINT('Ctrl Pts',(-4.85068927007173,2.19548202900138,8.40164026752836));
#25411=CARTESIAN_POINT('Ctrl Pts',(1.5129078685785E-11,2.37048202900139,
8.40164026751963));
#25412=CARTESIAN_POINT('Ctrl Pts',(4.85068927010198,2.5454820290014,8.4016402675109));
#25413=CARTESIAN_POINT('Ctrl Pts',(7.27603390513785,2.72048202900138,4.20082013374672));
#25414=CARTESIAN_POINT('Ctrl Pts',(9.70137854017372,2.89548202900139,-1.74689612655491E-11));
#25415=CARTESIAN_POINT('Ctrl Pts',(7.27603390512273,3.0704820290014,-4.20082013377291));
#25416=CARTESIAN_POINT('Ctrl Pts',(4.85068927007173,3.24548202900138,-8.40164026752836));
#25417=CARTESIAN_POINT('Ctrl Pts',(-1.51301075899711E-11,3.42048202900139,
-8.40164026751963));
#25418=CARTESIAN_POINT('Ctrl Pts',(-4.85068927010199,3.59548202900139,-8.4016402675109));
#25419=CARTESIAN_POINT('Ctrl Pts',(-7.27603390513785,3.77048202900138,-4.20082013374671));
#25420=CARTESIAN_POINT('Ctrl Pts',(-9.70137854017372,3.94548202900138,1.74701493417668E-11));
#25421=CARTESIAN_POINT('Ctrl Pts',(-7.27603390512272,4.12048202900139,4.20082013377292));
#25422=CARTESIAN_POINT('Ctrl Pts',(-4.85068927007173,4.29548202900137,8.40164026752836));
#25423=CARTESIAN_POINT('Ctrl Pts',(1.5129078685785E-11,4.47048202900138,
8.40164026751963));
#25424=CARTESIAN_POINT('Ctrl Pts',(4.85068927010198,4.64548202900139,8.4016402675109));
#25425=CARTESIAN_POINT('Ctrl Pts',(7.27603390513785,4.82048202900137,4.20082013374672));
#25426=CARTESIAN_POINT('Ctrl Pts',(9.70137854017372,4.99548202900138,-1.74689612655491E-11));
#25427=CARTESIAN_POINT('Ctrl Pts',(7.27603390512273,5.17048202900139,-4.20082013377291));
#25428=CARTESIAN_POINT('Ctrl Pts',(4.85068927007173,5.34548202900137,-8.40164026752836));
#25429=CARTESIAN_POINT('Ctrl Pts',(-1.51301075899711E-11,5.52048202900138,
-8.40164026751963));
#25430=CARTESIAN_POINT('Ctrl Pts',(-4.85068927010199,5.69548202900138,-8.4016402675109));
#25431=CARTESIAN_POINT('Ctrl Pts',(-7.27603390513785,5.87048202900137,-4.20082013374671));
#25432=CARTESIAN_POINT('Ctrl Pts',(-9.70137854017372,6.04548202900137,1.74701493417668E-11));
#25433=CARTESIAN_POINT('Ctrl Pts',(-7.27603390512272,6.22048202900138,4.20082013377292));
#25434=CARTESIAN_POINT('Ctrl Pts',(-4.85068927007173,6.39548202900136,8.40164026752836));
#25435=CARTESIAN_POINT('Ctrl Pts',(1.5129078685785E-11,6.57048202900137,
8.40164026751963));
#25436=CARTESIAN_POINT('Ctrl Pts',(4.85068927010198,6.74548202900138,8.4016402675109));
#25437=CARTESIAN_POINT('Ctrl Pts',(7.27603390513785,6.92048202900139,4.20082013374672));
#25438=CARTESIAN_POINT('Ctrl Pts',(9.70137854017372,7.09548202900137,-1.74689612655491E-11));
#25439=CARTESIAN_POINT('Ctrl Pts',(7.27603390512273,7.27048202900138,-4.20082013377291));
#25440=CARTESIAN_POINT('Ctrl Pts',(4.85068927007173,7.44548202900138,-8.40164026752836));
#25441=CARTESIAN_POINT('Ctrl Pts',(-1.51301075899711E-11,7.62048202900137,
-8.40164026751963));
#25442=CARTESIAN_POINT('Ctrl Pts',(-4.85068927010199,7.79548202900137,-8.4016402675109));
#25443=CARTESIAN_POINT('Ctrl Pts',(-7.27603390513785,7.97048202900139,-4.20082013374671));
#25444=CARTESIAN_POINT('Ctrl Pts',(-9.70137854017372,8.14548202900136,1.74701493417668E-11));
#25445=CARTESIAN_POINT('Ctrl Pts',(-7.27603390512272,8.32048202900138,4.20082013377292));
#25446=CARTESIAN_POINT('Ctrl Pts',(-4.85068927007173,8.49548202900138,8.40164026752836));
#25447=CARTESIAN_POINT('Ctrl Pts',(1.5129078685785E-11,8.67048202900136,
8.40164026751963));
#25448=CARTESIAN_POINT('Ctrl Pts',(4.85068927010198,8.84548202900137,8.4016402675109));
#25449=CARTESIAN_POINT('Ctrl Pts',(7.27603390513785,9.02048202900138,4.20082013374672));
#25450=CARTESIAN_POINT('Ctrl Pts',(9.70137854017372,9.19548202900136,-1.74689612655491E-11));
#25451=CARTESIAN_POINT('Ctrl Pts',(7.27603390512273,9.37048202900137,-4.20082013377291));
#25452=CARTESIAN_POINT('Ctrl Pts',(4.85068927007173,9.54548202900137,-8.40164026752836));
#25453=CARTESIAN_POINT('Ctrl Pts',(-1.51301075899711E-11,9.72048202900136,
-8.40164026751963));
#25454=CARTESIAN_POINT('Ctrl Pts',(-4.85068927010199,9.89548202900136,-8.4016402675109));
#25455=CARTESIAN_POINT('Ctrl Pts',(-7.27603390513785,10.0704820290014,-4.20082013374671));
#25456=CARTESIAN_POINT('Ctrl Pts',(-9.70137854017372,10.2454820290014,1.74701493417668E-11));
#25457=CARTESIAN_POINT('Ctrl Pts',(-7.27603390512272,10.4204820290014,4.20082013377292));
#25458=CARTESIAN_POINT('Ctrl Pts',(-4.85068927007173,10.5954820290014,8.40164026752836));
#25459=CARTESIAN_POINT('Ctrl Pts',(1.5129078685785E-11,10.7704820290014,
8.40164026751963));
#25460=CARTESIAN_POINT('Ctrl Pts',(4.85068927010198,10.9454820290014,8.4016402675109));
#25461=CARTESIAN_POINT('Ctrl Pts',(7.27603390513785,11.1204820290014,4.20082013374672));
#25462=CARTESIAN_POINT('Ctrl Pts',(9.70137854017372,11.2954820290014,-1.74689612655491E-11));
#25463=CARTESIAN_POINT('Ctrl Pts',(7.27603390512273,11.4704820290014,-4.20082013377291));
#25464=CARTESIAN_POINT('Ctrl Pts',(4.85068927007173,11.6454820290014,-8.40164026752836));
#25465=CARTESIAN_POINT('Ctrl Pts',(-1.51301075899711E-11,11.8204820290014,
-8.40164026751963));
#25466=CARTESIAN_POINT('Ctrl Pts',(-4.85068927010199,11.9954820290014,-8.4016402675109));
#25467=CARTESIAN_POINT('Ctrl Pts',(-7.27603390513785,12.1704820290014,-4.20082013374671));
#25468=CARTESIAN_POINT('Ctrl Pts',(-9.70137854017372,12.3454820290014,1.74701493417668E-11));
#25469=CARTESIAN_POINT('Ctrl Pts',(-7.27603390512272,12.5204820290014,4.20082013377292));
#25470=CARTESIAN_POINT('Ctrl Pts',(-4.85068927007173,12.6954820290014,8.40164026752836));
#25471=CARTESIAN_POINT('Ctrl Pts',(1.5129078685785E-11,12.8704820290014,
8.40164026751963));
#25472=CARTESIAN_POINT('Ctrl Pts',(4.85068927010198,13.0454820290013,8.4016402675109));
#25473=CARTESIAN_POINT('Ctrl Pts',(7.27603390513785,13.2204820290014,4.20082013374672));
#25474=CARTESIAN_POINT('Ctrl Pts',(9.70137854017372,13.3954820290014,-1.74689612655491E-11));
#25475=CARTESIAN_POINT('Ctrl Pts',(7.27603390512273,13.5704820290014,-4.20082013377291));
#25476=CARTESIAN_POINT('Ctrl Pts',(4.85068927007173,13.7454820290014,-8.40164026752836));
#25477=CARTESIAN_POINT('Ctrl Pts',(-1.51301075899711E-11,13.9204820290014,
-8.40164026751963));
#25478=CARTESIAN_POINT('Ctrl Pts',(-4.85068927010199,14.0954820290013,-8.4016402675109));
#25479=CARTESIAN_POINT('Ctrl Pts',(-7.27603390513785,14.2704820290014,-4.20082013374671));
#25480=CARTESIAN_POINT('Ctrl Pts',(-9.70137854017372,14.4454820290014,1.74701493417668E-11));
#25481=CARTESIAN_POINT('Ctrl Pts',(-7.27603390512272,14.6204820290013,4.20082013377292));
#25482=CARTESIAN_POINT('Ctrl Pts',(-4.85068927007173,14.7954820290014,8.40164026752836));
#25483=CARTESIAN_POINT('Ctrl Pts',(1.5129078685785E-11,14.9704820290014,
8.40164026751963));
#25484=CARTESIAN_POINT('Ctrl Pts',(4.85068927010198,15.1454820290013,8.4016402675109));
#25485=CARTESIAN_POINT('Ctrl Pts',(7.27603390513785,15.3204820290014,4.20082013374672));
#25486=CARTESIAN_POINT('Ctrl Pts',(9.70137854017372,15.4954820290014,-1.74689612655491E-11));
#25487=CARTESIAN_POINT('Ctrl Pts',(7.27603390512273,15.6704820290014,-4.20082013377291));
#25488=CARTESIAN_POINT('Ctrl Pts',(4.85068927007173,15.8454820290013,-8.40164026752836));
#25489=CARTESIAN_POINT('Ctrl Pts',(-1.51301075899711E-11,16.0204820290014,
-8.40164026751963));
#25490=CARTESIAN_POINT('Ctrl Pts',(-4.85068927010199,16.1954820290014,-8.4016402675109));
#25491=CARTESIAN_POINT('Ctrl Pts',(-7.27603390513785,16.3704820290014,-4.20082013374671));
#25492=CARTESIAN_POINT('Ctrl Pts',(-9.70137854017372,16.5454820290013,1.74701493417668E-11));
#25493=CARTESIAN_POINT('Ctrl Pts',(-7.27603390512272,16.7204820290014,4.20082013377292));
#25494=CARTESIAN_POINT('Ctrl Pts',(-4.85068927007173,16.8954820290013,8.40164026752836));
#25495=CARTESIAN_POINT('Ctrl Pts',(1.5129078685785E-11,17.0704820290014,
8.40164026751963));
#25496=CARTESIAN_POINT('Ctrl Pts',(4.85068927010198,17.2454820290014,8.4016402675109));
#25497=CARTESIAN_POINT('Ctrl Pts',(7.27603390513785,17.4204820290013,4.20082013374672));
#25498=CARTESIAN_POINT('Ctrl Pts',(9.70137854017372,17.5954820290013,-1.74689612655491E-11));
#25499=CARTESIAN_POINT('Ctrl Pts',(7.27603390512273,17.7704820290014,-4.20082013377291));
#25500=CARTESIAN_POINT('Ctrl Pts',(4.85068927007173,17.9454820290013,-8.40164026752836));
#25501=CARTESIAN_POINT('Ctrl Pts',(-1.51301075899711E-11,18.1204820290014,
-8.40164026751963));
#25502=CARTESIAN_POINT('Ctrl Pts',(-4.85068927010199,18.2954820290014,-8.4016402675109));
#25503=CARTESIAN_POINT('Ctrl Pts',(-7.27603390513785,18.4704820290013,-4.20082013374671));
#25504=CARTESIAN_POINT('Ctrl Pts',(-9.70137854017372,18.6454820290013,1.74701493417668E-11));
#25505=CARTESIAN_POINT('Ctrl Pts',(-7.27603390512272,18.8204820290014,4.20082013377292));
#25506=CARTESIAN_POINT('Ctrl Pts',(-4.85068927007173,18.9954820290013,8.40164026752836));
#25507=CARTESIAN_POINT('Ctrl Pts',(1.5129078685785E-11,19.1704820290013,
8.40164026751963));
#25508=CARTESIAN_POINT('Ctrl Pts',(4.85068927010198,19.3454820290014,8.4016402675109));
#25509=CARTESIAN_POINT('Ctrl Pts',(7.27603390513785,19.5204820290013,4.20082013374672));
#25510=CARTESIAN_POINT('Ctrl Pts',(9.70137854017372,19.6954820290013,-1.74689612655491E-11));
#25511=CARTESIAN_POINT('Ctrl Pts',(7.27603390512273,19.8704820290014,-4.20082013377291));
#25512=CARTESIAN_POINT('Ctrl Pts',(4.85068927007173,20.0454820290014,-8.40164026752836));
#25513=CARTESIAN_POINT('Ctrl Pts',(-1.51301075899711E-11,20.2204820290013,
-8.40164026751963));
#25514=CARTESIAN_POINT('Ctrl Pts',(-4.85068927010199,20.3954820290014,-8.4016402675109));
#25515=CARTESIAN_POINT('Ctrl Pts',(-7.27603390513785,20.5704820290014,-4.20082013374671));
#25516=CARTESIAN_POINT('Ctrl Pts',(-9.70137854017372,20.7454820290013,1.74701493417668E-11));
#25517=CARTESIAN_POINT('Ctrl Pts',(-7.27603390512272,20.9204820290013,4.20082013377292));
#25518=CARTESIAN_POINT('Ctrl Pts',(-4.85068927007173,21.0954820290014,8.40164026752836));
#25519=CARTESIAN_POINT('Ctrl Pts',(1.5129078685785E-11,21.2704820290013,
8.40164026751963));
#25520=CARTESIAN_POINT('Ctrl Pts',(4.85068927010198,21.4454820290013,8.4016402675109));
#25521=CARTESIAN_POINT('Ctrl Pts',(7.27603390513785,21.6204820290014,4.20082013374672));
#25522=CARTESIAN_POINT('Ctrl Pts',(9.70137854017372,21.7954820290013,-1.74689612655491E-11));
#25523=CARTESIAN_POINT('Ctrl Pts',(7.27603390512273,21.9704820290013,-4.20082013377291));
#25524=CARTESIAN_POINT('Ctrl Pts',(4.85068927007173,22.1454820290013,-8.40164026752836));
#25525=CARTESIAN_POINT('Ctrl Pts',(-1.51301075899711E-11,22.3204820290013,
-8.40164026751963));
#25526=CARTESIAN_POINT('Ctrl Pts',(-4.85068927010199,22.4954820290013,-8.4016402675109));
#25527=CARTESIAN_POINT('Ctrl Pts',(-7.27603390513785,22.6704820290013,-4.20082013374671));
#25528=CARTESIAN_POINT('Ctrl Pts',(-9.70137854017372,22.8454820290013,1.74701493417668E-11));
#25529=CARTESIAN_POINT('Ctrl Pts',(-7.27603390512272,23.0204820290013,4.20082013377292));
#25530=CARTESIAN_POINT('Ctrl Pts',(-4.85068927007173,23.1954820290013,8.40164026752836));
#25531=CARTESIAN_POINT('Ctrl Pts',(1.5129078685785E-11,23.3704820290013,
8.40164026751963));
#25532=CARTESIAN_POINT('Ctrl Pts',(4.85068927010198,23.5454820290013,8.4016402675109));
#25533=CARTESIAN_POINT('Ctrl Pts',(7.27603390513785,23.7204820290013,4.20082013374672));
#25534=CARTESIAN_POINT('Ctrl Pts',(9.70137854017372,23.8954820290013,-1.74689612655491E-11));
#25535=CARTESIAN_POINT('Ctrl Pts',(7.27603390512273,24.0704820290013,-4.20082013377291));
#25536=CARTESIAN_POINT('Ctrl Pts',(4.85068927007173,24.2454820290013,-8.40164026752836));
#25537=CARTESIAN_POINT('Ctrl Pts',(-1.51301075899711E-11,24.4204820290013,
-8.40164026751963));
#25538=CARTESIAN_POINT('Ctrl Pts',(-4.85068927010199,24.5954820290013,-8.4016402675109));
#25539=CARTESIAN_POINT('Ctrl Pts',(-7.27603390513785,24.7704820290013,-4.20082013374671));
#25540=CARTESIAN_POINT('Ctrl Pts',(-9.70137854017372,24.9454820290013,1.74701493417668E-11));
#25541=CARTESIAN_POINT('Ctrl Pts',(-7.27603390512272,25.1204820290013,4.20082013377292));
#25542=CARTESIAN_POINT('Ctrl Pts',(-4.85068927007173,25.2954820290013,8.40164026752836));
#25543=CARTESIAN_POINT('Ctrl Pts',(1.5129078685785E-11,25.4704820290013,
8.40164026751963));
#25544=CARTESIAN_POINT('Ctrl Pts',(4.85068927010198,25.6454820290013,8.4016402675109));
#25545=CARTESIAN_POINT('Ctrl Pts',(7.27603390513785,25.8204820290013,4.20082013374672));
#25546=CARTESIAN_POINT('Ctrl Pts',(9.70137854017372,25.9954820290013,-1.74689612655491E-11));
#25547=CARTESIAN_POINT('Ctrl Pts',(7.27603390512273,26.1704820290013,-4.20082013377291));
#25548=CARTESIAN_POINT('Ctrl Pts',(4.85068927007173,26.3454820290013,-8.40164026752836));
#25549=CARTESIAN_POINT('Ctrl Pts',(-1.51301075899711E-11,26.5204820290013,
-8.40164026751963));
#25550=CARTESIAN_POINT('Origin',(0.,15.4,0.));
#25551=CARTESIAN_POINT('',(-12.9886751345948,15.4,-1.5));
#25552=CARTESIAN_POINT('',(-7.79337567297407,15.4,-10.4985226280624));
#25553=CARTESIAN_POINT('',(-7.79337567297407,15.4,-10.4985226280624));
#25554=CARTESIAN_POINT('',(-5.19529946162075,15.4,-11.9985226280624));
#25555=CARTESIAN_POINT('Origin',(-5.19529946162075,15.4,-8.99852262806237));
#25556=CARTESIAN_POINT('',(5.19529946162075,15.4,-11.9985226280624));
#25557=CARTESIAN_POINT('',(5.19529946162075,15.4,-11.9985226280624));
#25558=CARTESIAN_POINT('',(7.79337567297407,15.4,-10.4985226280624));
#25559=CARTESIAN_POINT('Origin',(5.19529946162075,15.4,-8.99852262806237));
#25560=CARTESIAN_POINT('',(12.9886751345948,15.4,-1.5));
#25561=CARTESIAN_POINT('',(12.9886751345948,15.4,-1.50000000000001));
#25562=CARTESIAN_POINT('',(12.9886751345948,15.4,1.5));
#25563=CARTESIAN_POINT('Origin',(10.3905989232415,15.4,-5.20417042793042E-15));
#25564=CARTESIAN_POINT('',(7.79337567297406,15.4,10.4985226280624));
#25565=CARTESIAN_POINT('',(7.79337567297406,15.4,10.4985226280624));
#25566=CARTESIAN_POINT('',(5.19529946162075,15.4,11.9985226280624));
#25567=CARTESIAN_POINT('Origin',(5.19529946162075,15.4,8.99852262806237));
#25568=CARTESIAN_POINT('',(-5.19529946162075,15.4,11.9985226280624));
#25569=CARTESIAN_POINT('',(-5.19529946162075,15.4,11.9985226280624));
#25570=CARTESIAN_POINT('',(-7.79337567297407,15.4,10.4985226280624));
#25571=CARTESIAN_POINT('Origin',(-5.19529946162075,15.4,8.99852262806237));
#25572=CARTESIAN_POINT('',(-12.9886751345948,15.4,1.5));
#25573=CARTESIAN_POINT('',(-12.9886751345948,15.4,1.5));
#25574=CARTESIAN_POINT('Origin',(-10.3905989232415,15.4,-1.73472347597681E-15));
#25575=CARTESIAN_POINT('Origin',(0.,25.4,0.));
#25576=CARTESIAN_POINT('Ctrl Pts',(5.19529946162075,24.727212412536,10.9985226280624));
#25577=CARTESIAN_POINT('Ctrl Pts',(5.24518280334989,24.7149115564442,10.9985226280624));
#25578=CARTESIAN_POINT('Ctrl Pts',(5.2952655533899,24.7033920689907,10.9966536241576));
#25579=CARTESIAN_POINT('Ctrl Pts',(5.64376907527105,24.629016743781,10.970436558046));
#25580=CARTESIAN_POINT('Ctrl Pts',(5.94190593321436,24.5962843762458,10.8768702574676));
#25581=CARTESIAN_POINT('Ctrl Pts',(6.44869299002713,24.5962843762458,10.5842766137949));
#25582=CARTESIAN_POINT('Ctrl Pts',(6.67879221223778,24.629016743781,10.3728656713007));
#25583=CARTESIAN_POINT('Ctrl Pts',(6.8757486184437,24.7033920689907,10.0841613010991));
#25584=CARTESIAN_POINT('Ctrl Pts',(6.90240859832505,24.7149115564442,10.0417228692255));
#25585=CARTESIAN_POINT('Ctrl Pts',(6.92735026918962,24.727212412536,9.99852262806237));
#25586=CARTESIAN_POINT('Origin',(0.,25.4,0.));
#25587=CARTESIAN_POINT('Ctrl Pts',(12.1226497308104,24.727212412536,0.999999999999993));
#25588=CARTESIAN_POINT('Ctrl Pts',(12.1475914016749,24.7149115564442,0.956799758836891));
#25589=CARTESIAN_POINT('Ctrl Pts',(12.1710141718336,24.7033920689907,0.912492323058454));
#25590=CARTESIAN_POINT('Ctrl Pts',(12.3225612875088,24.629016743781,0.597570886745228));
#25591=CARTESIAN_POINT('Ctrl Pts',(12.3905989232415,24.5962843762458,0.292593643672666));
#25592=CARTESIAN_POINT('Ctrl Pts',(12.3905989232415,24.5962843762458,-0.292593643672677));
#25593=CARTESIAN_POINT('Ctrl Pts',(12.3225612875088,24.629016743781,-0.597570886745239));
#25594=CARTESIAN_POINT('Ctrl Pts',(12.1710141718336,24.7033920689907,-0.912492323058464));
#25595=CARTESIAN_POINT('Ctrl Pts',(12.1475914016749,24.7149115564442,-0.9567997588369));
#25596=CARTESIAN_POINT('Ctrl Pts',(12.1226497308104,24.727212412536,-1.));
#25597=CARTESIAN_POINT('Origin',(0.,25.4,0.));
#25598=CARTESIAN_POINT('Ctrl Pts',(6.92735026918963,24.727212412536,-9.99852262806237));
#25599=CARTESIAN_POINT('Ctrl Pts',(6.90240859832505,24.7149115564442,-10.0417228692255));
#25600=CARTESIAN_POINT('Ctrl Pts',(6.87574861844371,24.7033920689907,-10.0841613010991));
#25601=CARTESIAN_POINT('Ctrl Pts',(6.67879221223779,24.629016743781,-10.3728656713007));
#25602=CARTESIAN_POINT('Ctrl Pts',(6.44869299002713,24.5962843762458,-10.5842766137949));
#25603=CARTESIAN_POINT('Ctrl Pts',(5.94190593321436,24.5962843762458,-10.8768702574676));
#25604=CARTESIAN_POINT('Ctrl Pts',(5.64376907527106,24.629016743781,-10.970436558046));
#25605=CARTESIAN_POINT('Ctrl Pts',(5.29526555338991,24.7033920689907,-10.9966536241576));
#25606=CARTESIAN_POINT('Ctrl Pts',(5.2451828033499,24.7149115564442,-10.9985226280624));
#25607=CARTESIAN_POINT('Ctrl Pts',(5.19529946162075,24.727212412536,-10.9985226280624));
#25608=CARTESIAN_POINT('Origin',(0.,25.4,0.));
#25609=CARTESIAN_POINT('Ctrl Pts',(-5.19529946162075,24.727212412536,-10.9985226280624));
#25610=CARTESIAN_POINT('Ctrl Pts',(-5.2451828033499,24.7149115564442,-10.9985226280624));
#25611=CARTESIAN_POINT('Ctrl Pts',(-5.2952655533899,24.7033920689907,-10.9966536241576));
#25612=CARTESIAN_POINT('Ctrl Pts',(-5.64376907527106,24.629016743781,-10.970436558046));
#25613=CARTESIAN_POINT('Ctrl Pts',(-5.94190593321436,24.5962843762458,-10.8768702574676));
#25614=CARTESIAN_POINT('Ctrl Pts',(-6.44869299002714,24.5962843762458,-10.5842766137949));
#25615=CARTESIAN_POINT('Ctrl Pts',(-6.67879221223779,24.629016743781,-10.3728656713007));
#25616=CARTESIAN_POINT('Ctrl Pts',(-6.87574861844371,24.7033920689907,-10.0841613010991));
#25617=CARTESIAN_POINT('Ctrl Pts',(-6.90240859832505,24.7149115564442,-10.0417228692255));
#25618=CARTESIAN_POINT('Ctrl Pts',(-6.92735026918963,24.727212412536,-9.99852262806237));
#25619=CARTESIAN_POINT('Origin',(0.,25.4,0.));
#25620=CARTESIAN_POINT('Ctrl Pts',(-12.1226497308104,24.727212412536,-1.));
#25621=CARTESIAN_POINT('Ctrl Pts',(-12.1475914016749,24.7149115564442,-0.956799758836898));
#25622=CARTESIAN_POINT('Ctrl Pts',(-12.1710141718336,24.7033920689907,-0.912492323058462));
#25623=CARTESIAN_POINT('Ctrl Pts',(-12.3225612875088,24.629016743781,-0.597570886745235));
#25624=CARTESIAN_POINT('Ctrl Pts',(-12.3905989232415,24.5962843762458,-0.292593643672673));
#25625=CARTESIAN_POINT('Ctrl Pts',(-12.3905989232415,24.5962843762458,0.29259364367267));
#25626=CARTESIAN_POINT('Ctrl Pts',(-12.3225612875088,24.629016743781,0.597570886745232));
#25627=CARTESIAN_POINT('Ctrl Pts',(-12.1710141718336,24.7033920689907,0.912492323058458));
#25628=CARTESIAN_POINT('Ctrl Pts',(-12.147591401675,24.7149115564442,0.956799758836896));
#25629=CARTESIAN_POINT('Ctrl Pts',(-12.1226497308104,24.727212412536,0.999999999999997));
#25630=CARTESIAN_POINT('Origin',(0.,25.4,0.));
#25631=CARTESIAN_POINT('Ctrl Pts',(-6.92735026918963,24.727212412536,9.99852262806237));
#25632=CARTESIAN_POINT('Ctrl Pts',(-6.90240859832505,24.7149115564442,10.0417228692255));
#25633=CARTESIAN_POINT('Ctrl Pts',(-6.87574861844371,24.7033920689907,10.0841613010991));
#25634=CARTESIAN_POINT('Ctrl Pts',(-6.67879221223779,24.629016743781,10.3728656713007));
#25635=CARTESIAN_POINT('Ctrl Pts',(-6.44869299002713,24.5962843762458,10.5842766137949));
#25636=CARTESIAN_POINT('Ctrl Pts',(-5.94190593321436,24.5962843762458,10.8768702574676));
#25637=CARTESIAN_POINT('Ctrl Pts',(-5.64376907527106,24.629016743781,10.970436558046));
#25638=CARTESIAN_POINT('Ctrl Pts',(-5.2952655533899,24.7033920689907,10.9966536241576));
#25639=CARTESIAN_POINT('Ctrl Pts',(-5.2451828033499,24.7149115564442,10.9985226280624));
#25640=CARTESIAN_POINT('Ctrl Pts',(-5.19529946162075,24.727212412536,10.9985226280624));
#25641=CARTESIAN_POINT('Origin',(-10.3905989232415,15.4,-1.73472347597681E-15));
#25642=CARTESIAN_POINT('Origin',(-10.3905989232415,16.4,-1.73472347597681E-15));
#25643=CARTESIAN_POINT('Origin',(-5.19529946162075,15.4,-8.99852262806237));
#25644=CARTESIAN_POINT('Origin',(-5.19529946162075,16.4,-8.99852262806237));
#25645=CARTESIAN_POINT('Origin',(5.19529946162075,15.4,-8.99852262806237));
#25646=CARTESIAN_POINT('Origin',(5.19529946162075,16.4,-8.99852262806237));
#25647=CARTESIAN_POINT('Origin',(10.3905989232415,15.4,-5.20417042793042E-15));
#25648=CARTESIAN_POINT('Origin',(10.3905989232415,16.4,-5.20417042793042E-15));
#25649=CARTESIAN_POINT('Origin',(5.19529946162075,15.4,8.99852262806237));
#25650=CARTESIAN_POINT('Origin',(5.19529946162075,16.4,8.99852262806237));
#25651=CARTESIAN_POINT('Origin',(-5.19529946162075,15.4,8.99852262806237));
#25652=CARTESIAN_POINT('Origin',(-5.19529946162075,16.4,8.99852262806237));
#25653=CARTESIAN_POINT('Origin',(5.19529946162075,16.4,8.99852262806237));
#25654=CARTESIAN_POINT('Origin',(7.79337567297406,16.4,10.4985226280624));
#25655=CARTESIAN_POINT('Origin',(5.19529946162075,16.4,11.9985226280624));
#25656=CARTESIAN_POINT('Origin',(-6.35,16.4,11.9985226280624));
#25657=CARTESIAN_POINT('Origin',(-5.19529946162075,16.4,11.9985226280624));
#25658=CARTESIAN_POINT('Origin',(7.21602540378444,16.4,11.4985226280624));
#25659=CARTESIAN_POINT('Origin',(12.9886751345948,16.4,1.5));
#25660=CARTESIAN_POINT('Origin',(-5.19529946162075,16.4,8.99852262806237));
#25661=CARTESIAN_POINT('Origin',(-7.79337567297407,16.4,10.4985226280624));
#25662=CARTESIAN_POINT('Origin',(10.3905989232415,16.4,-5.20417042793042E-15));
#25663=CARTESIAN_POINT('Origin',(12.9886751345948,16.4,-1.5));
#25664=CARTESIAN_POINT('Origin',(-13.5660254037844,16.4,0.5));
#25665=CARTESIAN_POINT('Origin',(-12.9886751345948,16.4,1.5));
#25666=CARTESIAN_POINT('Origin',(13.5660254037844,16.4,-0.500000000000007));
#25667=CARTESIAN_POINT('Origin',(7.79337567297406,16.4,-10.4985226280624));
#25668=CARTESIAN_POINT('Origin',(-10.3905989232415,16.4,-1.73472347597681E-15));
#25669=CARTESIAN_POINT('Origin',(-12.9886751345948,16.4,-1.5));
#25670=CARTESIAN_POINT('Origin',(5.19529946162075,16.4,-8.99852262806237));
#25671=CARTESIAN_POINT('Origin',(5.19529946162075,16.4,-11.9985226280624));
#25672=CARTESIAN_POINT('Origin',(-7.21602540378444,16.4,-11.4985226280624));
#25673=CARTESIAN_POINT('Origin',(-7.79337567297407,16.4,-10.4985226280624));
#25674=CARTESIAN_POINT('Origin',(6.35,16.4,-11.9985226280624));
#25675=CARTESIAN_POINT('Origin',(-5.19529946162075,16.4,-11.9985226280624));
#25676=CARTESIAN_POINT('Origin',(-5.19529946162075,16.4,-8.99852262806237));
#25677=CARTESIAN_POINT('Origin',(-48.,-7.90000000000001,7.7));
#25678=CARTESIAN_POINT('Origin',(-48.,-21.9,7.7));
#25679=CARTESIAN_POINT('Origin',(-48.,-7.90000000000001,7.7));
#25680=CARTESIAN_POINT('Origin',(-48.,-7.90000000000001,7.7));
#25681=CARTESIAN_POINT('Origin',(-48.,-7.90000000000001,7.7));
#25682=CARTESIAN_POINT('Origin',(-48.,-7.90000000000001,7.7));
#25683=CARTESIAN_POINT('Ctrl Pts',(-37.2370215606994,11.6489333498058,7.7));
#25684=CARTESIAN_POINT('Ctrl Pts',(-37.2370215606994,11.6489333498058,7.8077479627862));
#25685=CARTESIAN_POINT('Ctrl Pts',(-37.2348311473986,11.6461366519307,7.91713462674333));
#25686=CARTESIAN_POINT('Ctrl Pts',(-37.2302752431834,11.6403197188282,8.02776680121651));
#25687=CARTESIAN_POINT('Ctrl Pts',(-37.2256774210564,11.6344492653536,8.13941687894383));
#25688=CARTESIAN_POINT('Ctrl Pts',(-37.2186702459623,11.6255025740195,8.25233526639646));
#25689=CARTESIAN_POINT('Ctrl Pts',(-37.2090968020071,11.6132792961762,8.36607958557781));
#25690=CARTESIAN_POINT('Ctrl Pts',(-37.2004639399102,11.6022569438768,8.46864863245277));
#25691=CARTESIAN_POINT('Ctrl Pts',(-37.1897445552481,11.5885705403581,8.57188861673383));
#25692=CARTESIAN_POINT('Ctrl Pts',(-37.1768406531966,11.572094966805,8.67545161008087));
#25693=CARTESIAN_POINT('Ctrl Pts',(-37.1626489093056,11.5539750896244,8.78935045031606));
#25694=CARTESIAN_POINT('Ctrl Pts',(-37.1458143533317,11.5324808963114,8.9036374875757));
#25695=CARTESIAN_POINT('Ctrl Pts',(-37.1262661819627,11.5075219859026,9.01783447063753));
#25696=CARTESIAN_POINT('Ctrl Pts',(-37.1064327010615,11.4821987951262,9.13369818186538));
#25697=CARTESIAN_POINT('Ctrl Pts',(-37.083805740066,11.4533089168019,9.24946879412115));
#25698=CARTESIAN_POINT('Ctrl Pts',(-37.0583419637689,11.420797020969,9.36462556197383));
#25699=CARTESIAN_POINT('Ctrl Pts',(-37.0399180815693,11.3972735917682,9.44794528253116));
#25700=CARTESIAN_POINT('Ctrl Pts',(-37.0200097712987,11.3718548595984,9.53094317961308));
#25701=CARTESIAN_POINT('Ctrl Pts',(-36.9986106492179,11.3445326737651,9.61341716182606));
#25702=CARTESIAN_POINT('Ctrl Pts',(-36.9694052390191,11.3072434970515,9.72597722256865));
#25703=CARTESIAN_POINT('Ctrl Pts',(-36.9373995710248,11.2663789790887,9.83753573161566));
#25704=CARTESIAN_POINT('Ctrl Pts',(-36.902657311863,11.2220204087928,9.94761455701875));
#25705=CARTESIAN_POINT('Ctrl Pts',(-36.8657225277775,11.1748624445227,10.0646402699898));
#25706=CARTESIAN_POINT('Ctrl Pts',(-36.8256946326858,11.1237552269421,10.1799930477234));
#25707=CARTESIAN_POINT('Ctrl Pts',(-36.7826890673221,11.0688461496304,10.2931010720517));
#25708=CARTESIAN_POINT('Ctrl Pts',(-36.7410984721777,11.0157436921946,10.4024876132504));
#25709=CARTESIAN_POINT('Ctrl Pts',(-36.69672330252,10.9590859177681,10.5097741691194));
#25710=CARTESIAN_POINT('Ctrl Pts',(-36.6497011112435,10.8990484525159,10.6144542442965));
#25711=CARTESIAN_POINT('Ctrl Pts',(-36.6002792788918,10.835947149451,10.7244763633326));
#25712=CARTESIAN_POINT('Ctrl Pts',(-36.5479333176005,10.7691123476947,10.8316183371238));
#25713=CARTESIAN_POINT('Ctrl Pts',(-36.4928582485832,10.6987930483889,10.9353147905031));
#25714=CARTESIAN_POINT('Ctrl Pts',(-36.4377831795658,10.6284737490832,11.0390112438824));
#25715=CARTESIAN_POINT('Ctrl Pts',(-36.3799792804388,10.5546703066858,11.1392614617744));
#25716=CARTESIAN_POINT('Ctrl Pts',(-36.3196738148537,10.4776728891628,11.2355339059335));
#25717=CARTESIAN_POINT('Ctrl Pts',(-36.2619915983051,10.4040248098692,11.3276185605792));
#25718=CARTESIAN_POINT('Ctrl Pts',(-36.2020302432153,10.3274667491973,11.4160493299939));
#25719=CARTESIAN_POINT('Ctrl Pts',(-36.1400807365056,10.2483702363487,11.5005079328353));
#25720=CARTESIAN_POINT('Ctrl Pts',(-36.0768630623417,10.1676545399319,11.5866954865115));
#25721=CARTESIAN_POINT('Ctrl Pts',(-36.011575325106,10.0842958076127,11.6687460449283));
#25722=CARTESIAN_POINT('Ctrl Pts',(-35.944546007913,9.99871344335855,11.7463674222083));
#25723=CARTESIAN_POINT('Ctrl Pts',(-35.8792875513239,9.91539209627714,11.8219381051833));
#25724=CARTESIAN_POINT('Ctrl Pts',(-35.8123787392189,9.82996359171854,11.893310428993));
#25725=CARTESIAN_POINT('Ctrl Pts',(-35.7441350624009,9.74283074519608,11.9602622260613));
#25726=CARTESIAN_POINT('Ctrl Pts',(-35.6731135837839,9.65215122901703,12.0299392400438));
#25727=CARTESIAN_POINT('Ctrl Pts',(-35.6006467011536,9.55962623539705,12.0948278197615));
#25728=CARTESIAN_POINT('Ctrl Pts',(-35.5270979720375,9.46571995096445,12.1547367464213));
#25729=CARTESIAN_POINT('Ctrl Pts',(-35.4581365562657,9.37767070249793,12.2109090888871));
#25730=CARTESIAN_POINT('Ctrl Pts',(-35.3882243786871,9.28840753083064,12.2627039132039));
#25731=CARTESIAN_POINT('Ctrl Pts',(-35.3176628312434,9.19831525019048,12.3100156165359));
#25732=CARTESIAN_POINT('Ctrl Pts',(-35.312969077141,9.19232231172517,12.313162791019));
#25733=CARTESIAN_POINT('Ctrl Pts',(-35.3082724492566,9.18632570404355,12.3162901472982));
#25734=CARTESIAN_POINT('Ctrl Pts',(-35.3035730360603,9.18032554010357,12.3193976625566));
#25735=CARTESIAN_POINT('Ctrl Pts',(-35.2309234491108,9.08756727142935,12.367437639153));
#25736=CARTESIAN_POINT('Ctrl Pts',(-35.157622566231,8.99397743460166,12.4107244434961));
#25737=CARTESIAN_POINT('Ctrl Pts',(-35.0840243715693,8.90000799305338,12.4493287586889));
#25738=CARTESIAN_POINT('Ctrl Pts',(-35.011193186692,8.8070178619548,12.4875307557594));
#25739=CARTESIAN_POINT('Ctrl Pts',(-34.9380711627225,8.71365639040143,12.521147462252));
#25740=CARTESIAN_POINT('Ctrl Pts',(-34.864990431616,8.62034764116423,12.5502951735018));
#25741=CARTESIAN_POINT('Ctrl Pts',(-34.793030700632,8.52847017371273,12.5789957821106));
#25742=CARTESIAN_POINT('Ctrl Pts',(-34.721111242736,8.43664412653876,12.603363613898));
#25743=CARTESIAN_POINT('Ctrl Pts',(-34.6495345151887,8.34525567405873,12.6235541698602));
#25744=CARTESIAN_POINT('Ctrl Pts',(-34.5785107837497,8.25457328149928,12.6435887351917));
#25745=CARTESIAN_POINT('Ctrl Pts',(-34.5078247134336,8.16432201129683,12.6595104555204));
#25746=CARTESIAN_POINT('Ctrl Pts',(-34.4377539870199,8.07485640605711,12.6715132355078));
#25747=CARTESIAN_POINT('Ctrl Pts',(-34.368285509019,7.98615974558962,12.6834128532252));
#25748=CARTESIAN_POINT('Ctrl Pts',(-34.2994219988082,7.898235501968,12.6914607677224));
#25749=CARTESIAN_POINT('Ctrl Pts',(-34.2314137778158,7.81140328309775,12.6958851496815));
#25750=CARTESIAN_POINT('Ctrl Pts',(-34.1889236830279,7.75715235348064,12.6986494097382));
#25751=CARTESIAN_POINT('Ctrl Pts',(-34.1467670361917,7.70332716688543,12.7));
#25752=CARTESIAN_POINT('Ctrl Pts',(-34.1050004454305,7.65,12.7));
#25753=CARTESIAN_POINT('Ctrl Pts',(-34.1050004454305,7.65,12.7));
#25754=CARTESIAN_POINT('Ctrl Pts',(-34.1050004454305,7.65,12.7));
#25755=CARTESIAN_POINT('Ctrl Pts',(-34.1050004454305,7.65,12.7));
#25756=CARTESIAN_POINT('Ctrl Pts',(-34.2221767330303,8.30461645762901,12.7));
#25757=CARTESIAN_POINT('Ctrl Pts',(-34.3684200110126,8.23864736688717,12.7));
#25758=CARTESIAN_POINT('Ctrl Pts',(-34.5150549589694,8.17355351674842,12.7));
#25759=CARTESIAN_POINT('Ctrl Pts',(-34.3392646891937,8.95873944331344,12.5698633744289));
#25760=CARTESIAN_POINT('Ctrl Pts',(-34.6344129874181,8.833045375353,12.5964281310995));
#25761=CARTESIAN_POINT('Ctrl Pts',(-34.9248003596003,8.69671236121519,12.5698633744284));
#25762=CARTESIAN_POINT('Ctrl Pts',(-34.5557392046831,10.1680948803375,12.0689319506839));
#25763=CARTESIAN_POINT('Ctrl Pts',(-35.1421214426245,9.96758997397988,12.1778901074191));
#25764=CARTESIAN_POINT('Ctrl Pts',(-35.6823457125228,9.66393871899066,12.0689319506845));
#25765=CARTESIAN_POINT('Ctrl Pts',(-34.6550194892076,10.7227336174031,11.6983341944624));
#25766=CARTESIAN_POINT('Ctrl Pts',(-35.3869447814668,10.5146815062463,11.8564353766687));
#25767=CARTESIAN_POINT('Ctrl Pts',(-36.0297737596904,10.1075313875409,11.6983341944627));
#25768=CARTESIAN_POINT('Ctrl Pts',(-34.8207019100435,11.6483341944624,10.7727336174031));
#25769=CARTESIAN_POINT('Ctrl Pts',(-35.8197142077533,11.48176450439,10.9904588000058));
#25770=CARTESIAN_POINT('Ctrl Pts',(-36.6095738700229,10.8478143907806,10.7727336174027));
#25771=CARTESIAN_POINT('Ctrl Pts',(-34.8870388756109,12.0189319519099,10.2180948773777));
#25772=CARTESIAN_POINT('Ctrl Pts',(-36.0061527172947,11.8983870794296,10.439161626936));
#25773=CARTESIAN_POINT('Ctrl Pts',(-36.8417178703412,11.144213537105,10.2180948773781));
#25774=CARTESIAN_POINT('Ctrl Pts',(-34.9542888854506,12.3946305178797,9.31107830404935));
#25775=CARTESIAN_POINT('Ctrl Pts',(-36.2030730684665,12.338432775914,9.4822033404738));
#25776=CARTESIAN_POINT('Ctrl Pts',(-37.0770570386603,11.4446922420911,9.31107830404915));
#25777=CARTESIAN_POINT('Ctrl Pts',(-34.9713749152927,12.4900832460695,8.99641282927341));
#25778=CARTESIAN_POINT('Ctrl Pts',(-36.2546886211118,12.4537748504033,9.14076955834494));
#25779=CARTESIAN_POINT('Ctrl Pts',(-37.1368490306999,11.5210340617091,8.99641282927351));
#25780=CARTESIAN_POINT('Ctrl Pts',(-34.9942307537467,12.6177695579628,8.35449039088788));
#25781=CARTESIAN_POINT('Ctrl Pts',(-36.3245787042152,12.6099538847863,8.43215085130189));
#25782=CARTESIAN_POINT('Ctrl Pts',(-37.2168322756968,11.6231558718972,8.35449039088778));
#25783=CARTESIAN_POINT('Ctrl Pts',(-34.9999999999986,12.65,8.02725293702972));
#25784=CARTESIAN_POINT('Ctrl Pts',(-36.3424993318352,12.6499999999596,8.06661933627904));
#25785=CARTESIAN_POINT('Ctrl Pts',(-37.2370215607001,11.648933349805,8.02725293702981));
#25786=CARTESIAN_POINT('Ctrl Pts',(-35.,12.65,7.7));
#25787=CARTESIAN_POINT('Ctrl Pts',(-36.3424993318543,12.65,7.69999999999999));
#25788=CARTESIAN_POINT('Ctrl Pts',(-37.2370215606994,11.6489333498058,7.7));
#25789=CARTESIAN_POINT('Ctrl Pts',(-35.,12.65,7.7));
#25790=CARTESIAN_POINT('Ctrl Pts',(-35.,12.65,7.80774796278557));
#25791=CARTESIAN_POINT('Ctrl Pts',(-34.9993740722507,12.6465031951891,7.91713462674209));
#25792=CARTESIAN_POINT('Ctrl Pts',(-34.9980721869531,12.6392300893458,8.02776680121466));
#25793=CARTESIAN_POINT('Ctrl Pts',(-34.9967583232841,12.6318900651929,8.13941687894151));
#25794=CARTESIAN_POINT('Ctrl Pts',(-34.9947559681418,12.6207037180452,8.25233526639368));
#25795=CARTESIAN_POINT('Ctrl Pts',(-34.9920202815809,12.6054205452911,8.36607958557456));
#25796=CARTESIAN_POINT('Ctrl Pts',(-34.9895533736499,12.5916389298757,8.46864863245064));
#25797=CARTESIAN_POINT('Ctrl Pts',(-34.9864902255602,12.5745263621959,8.57188861673282));
#25798=CARTESIAN_POINT('Ctrl Pts',(-34.9828028345235,12.5539264020161,8.67545161008097));
#25799=CARTESIAN_POINT('Ctrl Pts',(-34.9787474325986,12.5312705140633,8.78935045031526));
#25800=CARTESIAN_POINT('Ctrl Pts',(-34.9739368264302,12.5043956058905,8.90363748757406));
#25801=CARTESIAN_POINT('Ctrl Pts',(-34.9683507834176,12.4731886461523,9.01783447063506));
#25802=CARTESIAN_POINT('Ctrl Pts',(-34.9626832109724,12.4415262144972,9.1336981818622));
#25803=CARTESIAN_POINT('Ctrl Pts',(-34.9562173797198,12.4054042342126,9.24946879411729));
#25804=CARTESIAN_POINT('Ctrl Pts',(-34.9489409062851,12.3647535244,9.36462556196926));
#25805=CARTESIAN_POINT('Ctrl Pts',(-34.9436761377044,12.335341394785,9.44794528252829));
#25806=CARTESIAN_POINT('Ctrl Pts',(-34.9379871821807,12.3035595045322,9.53094317961187));
#25807=CARTESIAN_POINT('Ctrl Pts',(-34.9318722155105,12.269397662556,9.61341716182647));
#25808=CARTESIAN_POINT('Ctrl Pts',(-34.9235265408946,12.2227737588152,9.72597722256831));
#25809=CARTESIAN_POINT('Ctrl Pts',(-34.9143806706902,12.1716794864331,9.83753573161463));
#25810=CARTESIAN_POINT('Ctrl Pts',(-34.9044527981345,12.1162164836579,9.94761455701708));
#25811=CARTESIAN_POINT('Ctrl Pts',(-34.8938983944165,12.0572533050486,10.0646402699884));
#25812=CARTESIAN_POINT('Ctrl Pts',(-34.8824601100121,11.9933522430528,10.1799930477223));
#25813=CARTESIAN_POINT('Ctrl Pts',(-34.870170933015,11.924697588788,10.2931010720508));
#25814=CARTESIAN_POINT('Ctrl Pts',(-34.8582860948361,11.8583018117264,10.4024876132491));
#25815=CARTESIAN_POINT('Ctrl Pts',(-34.8456055426893,11.7874607030231,10.5097741691177));
#25816=CARTESIAN_POINT('Ctrl Pts',(-34.8321685833911,11.712393853941,10.6144542442945));
#25817=CARTESIAN_POINT('Ctrl Pts',(-34.8180459078685,11.6334961860564,10.7244763633312));
#25818=CARTESIAN_POINT('Ctrl Pts',(-34.8030876396081,11.5499303999952,10.831618337123));
#25819=CARTESIAN_POINT('Ctrl Pts',(-34.7873495074485,11.4620078302062,10.9353147905027));
#25820=CARTESIAN_POINT('Ctrl Pts',(-34.7716113752889,11.3740852604171,11.0390112438825));
#25821=CARTESIAN_POINT('Ctrl Pts',(-34.7550934585612,11.2818063500906,11.139261461775));
#25822=CARTESIAN_POINT('Ctrl Pts',(-34.737860699633,11.1855339059311,11.2355339059344));
#25823=CARTESIAN_POINT('Ctrl Pts',(-34.7213775546548,11.0934492512856,11.3276185605798));
#25824=CARTESIAN_POINT('Ctrl Pts',(-34.7042431279947,10.99772614968,11.4160493299941));
#25825=CARTESIAN_POINT('Ctrl Pts',(-34.6865405714439,10.8988291364902,11.5005079328351));
#25826=CARTESIAN_POINT('Ctrl Pts',(-34.6684756261143,10.7979076039761,11.5866954865114));
#25827=CARTESIAN_POINT('Ctrl Pts',(-34.6498191440552,10.6936813953507,11.6687460449281));
#25828=CARTESIAN_POINT('Ctrl Pts',(-34.6306649918883,10.5866749054099,11.7463674222083));
#25829=CARTESIAN_POINT('Ctrl Pts',(-34.6120168770032,10.482495440797,11.821938105183));
#25830=CARTESIAN_POINT('Ctrl Pts',(-34.5928971601087,10.3756813267753,11.8933104289926));
#25831=CARTESIAN_POINT('Ctrl Pts',(-34.5733959951717,10.266736217042,11.9602622260608));
#25832=CARTESIAN_POINT('Ctrl Pts',(-34.5531010516228,10.1533565877173,12.0299392400434));
#25833=CARTESIAN_POINT('Ctrl Pts',(-34.5323930725609,10.0376694962776,12.0948278197612));
#25834=CARTESIAN_POINT('Ctrl Pts',(-34.5113759473958,9.9202553307762,12.1547367464212));
#25835=CARTESIAN_POINT('Ctrl Pts',(-34.4916696829333,9.81016441306816,12.2109090888872));
#25836=CARTESIAN_POINT('Ctrl Pts',(-34.471691730841,9.69855568661636,12.2627039132042));
#25837=CARTESIAN_POINT('Ctrl Pts',(-34.4515282162257,9.5859102975093,12.3100156165363));
#25838=CARTESIAN_POINT('Ctrl Pts',(-34.4501869392431,9.57841712627964,12.3131627910194));
#25839=CARTESIAN_POINT('Ctrl Pts',(-34.4488448410548,9.57091936730622,12.3162901472986));
#25840=CARTESIAN_POINT('Ctrl Pts',(-34.4475019469419,9.56341716182413,12.319397662557));
#25841=CARTESIAN_POINT('Ctrl Pts',(-34.4267417586902,9.44743839878783,12.3674376391538));
#25842=CARTESIAN_POINT('Ctrl Pts',(-34.4057954575275,9.33041989830073,12.4107244434972));
#25843=CARTESIAN_POINT('Ctrl Pts',(-34.3847641971955,9.21292676534625,12.4493287586903));
#25844=CARTESIAN_POINT('Ctrl Pts',(-34.3639521159143,9.09665809697244,12.4875307557612));
#25845=CARTESIAN_POINT('Ctrl Pts',(-34.3430569250855,8.97992512921895,12.521147462254));
#25846=CARTESIAN_POINT('Ctrl Pts',(-34.3221735340156,8.86325808193921,12.5502951735039));
#25847=CARTESIAN_POINT('Ctrl Pts',(-34.301610477507,8.74838061410455,12.578995782113));
#25848=CARTESIAN_POINT('Ctrl Pts',(-34.2810589293485,8.63356743876123,12.6033636139005));
#25849=CARTESIAN_POINT('Ctrl Pts',(-34.2606053190705,8.51930140268692,12.6235541698628));
#25850=CARTESIAN_POINT('Ctrl Pts',(-34.2403097317599,8.40591817692525,12.6435887351944));
#25851=CARTESIAN_POINT('Ctrl Pts',(-34.2201106337586,8.29307399785344,12.659510455523));
#25852=CARTESIAN_POINT('Ctrl Pts',(-34.2000873750951,8.18121216193919,12.6715132355102));
#25853=CARTESIAN_POINT('Ctrl Pts',(-34.1802362136306,8.07031176336932,12.6834128532274));
#25854=CARTESIAN_POINT('Ctrl Pts',(-34.1605579264484,7.9603771433938,12.6914607677241));
#25855=CARTESIAN_POINT('Ctrl Pts',(-34.1411240448565,7.85180791845727,12.6958851496827));
#25856=CARTESIAN_POINT('Ctrl Pts',(-34.1289821676136,7.78397616825827,12.6986494097386));
#25857=CARTESIAN_POINT('Ctrl Pts',(-34.1169355757335,7.71667673878648,12.7));
#25858=CARTESIAN_POINT('Ctrl Pts',(-34.1050004454305,7.65,12.7));
#25859=CARTESIAN_POINT('Origin',(-48.,7.65,7.7));
#25860=CARTESIAN_POINT('Origin',(-17.9697662756086,7.65,7.7));
#25861=CARTESIAN_POINT('Ctrl Pts',(-17.9697662756086,7.65,12.7));
#25862=CARTESIAN_POINT('Ctrl Pts',(-17.9697662756086,12.65,12.7));
#25863=CARTESIAN_POINT('Ctrl Pts',(-17.9697662756086,12.65,7.7));
#25864=CARTESIAN_POINT('Ctrl Pts',(-17.5769226509334,7.65000000135137,12.7));
#25865=CARTESIAN_POINT('Ctrl Pts',(-17.8797974234722,12.5223340542636,12.7));
#25866=CARTESIAN_POINT('Ctrl Pts',(-17.8786433834304,12.65,7.82930352963304));
#25867=CARTESIAN_POINT('Ctrl Pts',(-17.1871178707086,7.68525114336172,12.7));
#25868=CARTESIAN_POINT('Ctrl Pts',(-17.7621458420668,12.4006679911033,12.699999999999));
#25869=CARTESIAN_POINT('Ctrl Pts',(-17.7836615820008,12.6532040193815,7.96407165192601));
#25870=CARTESIAN_POINT('Ctrl Pts',(-16.8005208252602,7.75488674445212,12.7));
#25871=CARTESIAN_POINT('Ctrl Pts',(-17.617785931914,12.2921100651331,12.7));
#25872=CARTESIAN_POINT('Ctrl Pts',(-17.6839681951541,12.6595351585866,8.1049008253337));
#25873=CARTESIAN_POINT('Origin',(-16.8005208252601,7.75488674445212,7.7));
#25874=CARTESIAN_POINT('Ctrl Pts',(-16.8005208252602,7.75488674445212,12.7));
#25875=CARTESIAN_POINT('Ctrl Pts',(-17.617785931914,12.2921100651331,12.7));
#25876=CARTESIAN_POINT('Ctrl Pts',(-17.6839681951541,12.6595351585866,8.10490082533369));
#25877=CARTESIAN_POINT('Ctrl Pts',(-16.57400807036,7.82781362133464,12.7));
#25878=CARTESIAN_POINT('Ctrl Pts',(-17.6286821698629,12.155095870898,12.671192031208));
#25879=CARTESIAN_POINT('Ctrl Pts',(-17.5797557624158,12.6661532847416,8.25211370792749));
#25880=CARTESIAN_POINT('Ctrl Pts',(-16.3460043190073,7.93905335192941,12.712469440238));
#25881=CARTESIAN_POINT('Ctrl Pts',(-17.5788419030212,12.0132242375904,12.6289721703847));
#25882=CARTESIAN_POINT('Ctrl Pts',(-17.4601309122998,12.6762775771018,8.42880065885016));
#25883=CARTESIAN_POINT('Ctrl Pts',(-15.9085797765213,8.21703647488218,12.7591081700646));
#25884=CARTESIAN_POINT('Ctrl Pts',(-17.3634553041143,11.7807433434256,12.5578936033112));
#25885=CARTESIAN_POINT('Ctrl Pts',(-17.1967503219572,12.7015487707901,8.82270036173133));
#25886=CARTESIAN_POINT('Ctrl Pts',(-15.6990852529236,8.3825852909746,12.7928422221643));
#25887=CARTESIAN_POINT('Ctrl Pts',(-17.2053550226203,11.6893488147424,12.5292392590373));
#25888=CARTESIAN_POINT('Ctrl Pts',(-17.053307387847,12.7165986624452,9.03920832840638));
#25889=CARTESIAN_POINT('Ctrl Pts',(-15.2946854951174,8.75509815651616,12.8776711254801));
#25890=CARTESIAN_POINT('Ctrl Pts',(-16.8188792119444,11.5743897252593,12.5075888732474));
#25891=CARTESIAN_POINT('Ctrl Pts',(-16.7385788933035,12.7504634691449,9.50671774903932));
#25892=CARTESIAN_POINT('Ctrl Pts',(-15.0994609327293,8.96258837046799,12.9289025745581));
#25893=CARTESIAN_POINT('Ctrl Pts',(-16.5928074468314,11.5481648613874,12.5132247397972));
#25894=CARTESIAN_POINT('Ctrl Pts',(-16.5669250005632,12.7693262151711,9.75824593848983));
#25895=CARTESIAN_POINT('Ctrl Pts',(-14.7226800076233,9.40977222762574,13.0463331216422));
#25896=CARTESIAN_POINT('Ctrl Pts',(-16.1048897677201,11.5609929861839,12.5675172427461));
#25897=CARTESIAN_POINT('Ctrl Pts',(-16.1929560790172,12.8099792937465,10.2884101870157));
#25898=CARTESIAN_POINT('Ctrl Pts',(-14.5437893111222,9.64614677008646,13.1116414598527));
#25899=CARTESIAN_POINT('Ctrl Pts',(-15.8472046102766,11.5974627760302,12.6142743787051));
#25900=CARTESIAN_POINT('Ctrl Pts',(-15.993385566602,12.8314678879228,10.5631032975644));
#25901=CARTESIAN_POINT('Ctrl Pts',(-14.0293669548612,10.3837101835141,13.3245337884544));
#25902=CARTESIAN_POINT('Ctrl Pts',(-15.0766777630351,11.7789057456683,12.8105573724733));
#25903=CARTESIAN_POINT('Ctrl Pts',(-15.354300460823,12.898519108126,11.4060563768849));
#25904=CARTESIAN_POINT('Ctrl Pts',(-13.7157820791968,10.9130303131153,13.4887739635291));
#25905=CARTESIAN_POINT('Ctrl Pts',(-14.5379048034935,11.9964940699689,13.0187576709113));
#25906=CARTESIAN_POINT('Ctrl Pts',(-14.8736435223247,12.9466391191654,11.993249292684));
#25907=CARTESIAN_POINT('Ctrl Pts',(-13.1283088804427,12.0122001031246,13.8579187609855));
#25908=CARTESIAN_POINT('Ctrl Pts',(-13.525404177229,12.5253529301391,13.5631951324379));
#25909=CARTESIAN_POINT('Ctrl Pts',(-13.8052132993074,13.0465636459474,13.1624707293919));
#25910=CARTESIAN_POINT('Ctrl Pts',(-12.8547128646902,12.5827074287807,14.063208861629));
#25911=CARTESIAN_POINT('Ctrl Pts',(-13.0355631159118,12.8406828545529,13.9037139318704));
#25912=CARTESIAN_POINT('Ctrl Pts',(-13.2169060869103,13.0984138348476,13.7437844641131));
#25913=CARTESIAN_POINT('Ctrl Pts',(-12.6003906189451,13.15,14.2875));
#25914=CARTESIAN_POINT('Ctrl Pts',(-12.6003906189451,13.15,14.2875));
#25915=CARTESIAN_POINT('Ctrl Pts',(-12.6003906189451,13.15,14.2875));
#25916=CARTESIAN_POINT('Origin',(-48.,-22.9,-7.7));
#25917=CARTESIAN_POINT('Origin',(-48.,-21.9,-7.7));
#25918=CARTESIAN_POINT('Origin',(-48.,-7.90000000000001,-7.7));
#25919=CARTESIAN_POINT('Origin',(-48.,-7.90000000000001,-7.7));
#25920=CARTESIAN_POINT('Origin',(-48.,-7.90000000000001,-7.7));
#25921=CARTESIAN_POINT('Origin',(-48.,-7.90000000000001,-7.7));
#25922=CARTESIAN_POINT('Ctrl Pts',(-34.1050004454305,7.65,-12.7));
#25923=CARTESIAN_POINT('Ctrl Pts',(-34.1718099032197,7.73530164995786,-12.7));
#25924=CARTESIAN_POINT('Ctrl Pts',(-34.2396185565292,7.82187906279926,-12.6965423806533));
#25925=CARTESIAN_POINT('Ctrl Pts',(-34.3081904207592,7.90943093573856,-12.6893758899384));
#25926=CARTESIAN_POINT('Ctrl Pts',(-34.3771672099234,7.99749981279899,-12.6821670802517));
#25927=CARTESIAN_POINT('Ctrl Pts',(-34.4469161091026,8.0865545122324,-12.6712053060908));
#25928=CARTESIAN_POINT('Ctrl Pts',(-34.5171747421384,8.17626003477469,-12.6562735357966));
#25929=CARTESIAN_POINT('Ctrl Pts',(-34.5883719103702,8.2671638697028,-12.6411423025843));
#25930=CARTESIAN_POINT('Ctrl Pts',(-34.66009235558,8.35873581946203,-12.6219341077298));
#25931=CARTESIAN_POINT('Ctrl Pts',(-34.7320426204516,8.45060120067544,-12.598465486817));
#25932=CARTESIAN_POINT('Ctrl Pts',(-34.804616020137,8.5432621942096,-12.5747936127996));
#25933=CARTESIAN_POINT('Ctrl Pts',(-34.8774230033899,8.63622142491524,-12.5467870597146));
#25934=CARTESIAN_POINT('Ctrl Pts',(-34.9501448392507,8.72907194027922,-12.5143028492619));
#25935=CARTESIAN_POINT('Ctrl Pts',(-35.0238838277916,8.82322114604926,-12.4813642855694));
#25936=CARTESIAN_POINT('Ctrl Pts',(-35.0975349916622,8.91725821815552,-12.4438217748955));
#25937=CARTESIAN_POINT('Ctrl Pts',(-35.1707519133804,9.01074085420895,-12.4015749261073));
#25938=CARTESIAN_POINT('Ctrl Pts',(-35.2152124509763,9.06750762556827,-12.3759207799786));
#25939=CARTESIAN_POINT('Ctrl Pts',(-35.2595126064814,9.12406962267239,-12.3485328867842));
#25940=CARTESIAN_POINT('Ctrl Pts',(-35.3035730360607,9.18032554010333,-12.3193976625566));
#25941=CARTESIAN_POINT('Ctrl Pts',(-35.3743528484633,9.270696499268,-12.2725940856323));
#25942=CARTESIAN_POINT('Ctrl Pts',(-35.4445009330806,9.36026087469156,-12.2212852588861));
#25943=CARTESIAN_POINT('Ctrl Pts',(-35.5137142400593,9.44863173534098,-12.165573946384));
#25944=CARTESIAN_POINT('Ctrl Pts',(-35.5869435953334,9.54213024643472,-12.1066300283126));
#25945=CARTESIAN_POINT('Ctrl Pts',(-35.6591261721559,9.6342922412322,-12.042757601111));
#25946=CARTESIAN_POINT('Ctrl Pts',(-35.7299047145333,9.7246615788413,-11.9741404696194));
#25947=CARTESIAN_POINT('Ctrl Pts',(-35.7986260588343,9.81240430644607,-11.9075177141939));
#25948=CARTESIAN_POINT('Ctrl Pts',(-35.866023469218,9.89845664841804,-11.836422628961));
#25949=CARTESIAN_POINT('Ctrl Pts',(-35.931776733129,9.98240976055746,-11.761076892045));
#25950=CARTESIAN_POINT('Ctrl Pts',(-36.0004825183291,10.0701326224572,-11.682347902663));
#25951=CARTESIAN_POINT('Ctrl Pts',(-36.0673926725241,10.1555628405829,-11.5989779345116));
#25952=CARTESIAN_POINT('Ctrl Pts',(-36.1321559838961,10.2382519911851,-11.5112757977197));
#25953=CARTESIAN_POINT('Ctrl Pts',(-36.1969192952681,10.3209411417873,-11.4235736609278));
#25954=CARTESIAN_POINT('Ctrl Pts',(-36.2595353220431,10.4008886608136,-11.331539792544));
#25955=CARTESIAN_POINT('Ctrl Pts',(-36.319673814854,10.4776728891626,-11.2355339059334));
#25956=CARTESIAN_POINT('Ctrl Pts',(-36.3772994165222,10.5512486831415,-11.1435396320325));
#25957=CARTESIAN_POINT('Ctrl Pts',(-36.4326410435374,10.6219083210428,-11.047913512207));
#25958=CARTESIAN_POINT('Ctrl Pts',(-36.4854998118621,10.6893978697096,-10.9491185834245));
#25959=CARTESIAN_POINT('Ctrl Pts',(-36.5395045498368,10.758350581006,-10.8481817963743));
#25960=CARTESIAN_POINT('Ctrl Pts',(-36.5909172651151,10.8239938235529,-10.7439378175919));
#25961=CARTESIAN_POINT('Ctrl Pts',(-36.6395546932315,10.8860936071067,-10.6369112386827));
#25962=CARTESIAN_POINT('Ctrl Pts',(-36.6867359586466,10.9463341766341,-10.5330889433528));
#25963=CARTESIAN_POINT('Ctrl Pts',(-36.7313055740367,11.0032402174342,-10.4266488425142));
#25964=CARTESIAN_POINT('Ctrl Pts',(-36.7731256175259,11.0566356322302,-10.3180893465301));
#25965=CARTESIAN_POINT('Ctrl Pts',(-36.8145521714388,11.1095286434562,-10.2105512992704));
#25966=CARTESIAN_POINT('Ctrl Pts',(-36.8532805293795,11.1589766249522,-10.1009340887698));
#25967=CARTESIAN_POINT('Ctrl Pts',(-36.8892073412382,11.2048476203274,-9.98973289375452));
#25968=CARTESIAN_POINT('Ctrl Pts',(-36.9245963841465,11.2500319976657,-9.88019620908197));
#25969=CARTESIAN_POINT('Ctrl Pts',(-36.9572670623662,11.2917455940576,-9.76912308215516));
#25970=CARTESIAN_POINT('Ctrl Pts',(-36.9871518459034,11.3299021878797,-9.65698972956914));
#25971=CARTESIAN_POINT('Ctrl Pts',(-36.9910180653701,11.3348385383683,-9.64248294386366));
#25972=CARTESIAN_POINT('Ctrl Pts',(-36.994837701986,11.3397154123373,-9.62795841177471));
#25973=CARTESIAN_POINT('Ctrl Pts',(-36.9986106492175,11.3445326737655,-9.61341716182616));
#25974=CARTESIAN_POINT('Ctrl Pts',(-37.0282507404559,11.3823768468988,-9.49918180449011));
#25975=CARTESIAN_POINT('Ctrl Pts',(-37.0550294404338,11.4165676241844,-9.38394181607375));
#25976=CARTESIAN_POINT('Ctrl Pts',(-37.0789680109407,11.4471321524627,-9.26823244742671));
#25977=CARTESIAN_POINT('Ctrl Pts',(-37.1025632992548,11.4772583814581,-9.15418236606997));
#25978=CARTESIAN_POINT('Ctrl Pts',(-37.1233993879242,11.5038616918423,-9.03967670402529));
#25979=CARTESIAN_POINT('Ctrl Pts',(-37.141526145474,11.5270057552509,-8.9252124146849));
#25980=CARTESIAN_POINT('Ctrl Pts',(-37.1547234940072,11.5438559983481,-8.84187566144162));
#25981=CARTESIAN_POINT('Ctrl Pts',(-37.1664853189077,11.5588733791759,-8.75856053416828));
#25982=CARTESIAN_POINT('Ctrl Pts',(-37.1768406531962,11.5720949668055,-8.67545161008092));
#25983=CARTESIAN_POINT('Ctrl Pts',(-37.1911777621346,11.5904004446303,-8.56038611193216));
#25984=CARTESIAN_POINT('Ctrl Pts',(-37.2028177491878,11.6052622641081,-8.4457198673854));
#25985=CARTESIAN_POINT('Ctrl Pts',(-37.2118962775322,11.6168536386311,-8.33192848403724));
#25986=CARTESIAN_POINT('Ctrl Pts',(-37.2208885087921,11.6283348298965,-8.21921875888853));
#25987=CARTESIAN_POINT('Ctrl Pts',(-37.2273678674517,11.6366076104664,-8.10736762720217));
#25988=CARTESIAN_POINT('Ctrl Pts',(-37.2314899522891,11.6418706473102,-7.99680400773177));
#25989=CARTESIAN_POINT('Ctrl Pts',(-37.2352214310094,11.646634962156,-7.89671732597749));
#25990=CARTESIAN_POINT('Ctrl Pts',(-37.2370215606994,11.6489333498058,-7.79768544011085));
#25991=CARTESIAN_POINT('Ctrl Pts',(-37.2370215606994,11.6489333498058,-7.7));
#25992=CARTESIAN_POINT('Ctrl Pts',(-34.1050004454305,7.65,-12.7));
#25993=CARTESIAN_POINT('Ctrl Pts',(-34.1050004454305,7.65,-12.7));
#25994=CARTESIAN_POINT('Ctrl Pts',(-34.1050004454305,7.65,-12.7));
#25995=CARTESIAN_POINT('Ctrl Pts',(-34.51505495897,8.17355351674855,-12.7));
#25996=CARTESIAN_POINT('Ctrl Pts',(-34.3684200110127,8.23864736688751,-12.7));
#25997=CARTESIAN_POINT('Ctrl Pts',(-34.2221767330303,8.30461645762911,-12.7));
#25998=CARTESIAN_POINT('Ctrl Pts',(-34.9248003596002,8.69671236121437,-12.5698633744286));
#25999=CARTESIAN_POINT('Ctrl Pts',(-34.6344129874201,8.83304537535153,-12.5964281310995));
#26000=CARTESIAN_POINT('Ctrl Pts',(-34.3392646891937,8.95873944331332,-12.569863374429));
#26001=CARTESIAN_POINT('Ctrl Pts',(-35.6823457125229,9.66393871899146,-12.0689319506843));
#26002=CARTESIAN_POINT('Ctrl Pts',(-35.1421214426225,9.96758997398136,-12.1778901074191));
#26003=CARTESIAN_POINT('Ctrl Pts',(-34.5557392046831,10.1680948803376,-12.0689319506839));
#26004=CARTESIAN_POINT('Ctrl Pts',(-36.0297737596905,10.1075313875401,-11.6983341944632));
#26005=CARTESIAN_POINT('Ctrl Pts',(-35.3869447814668,10.5146815062458,-11.8564353766689));
#26006=CARTESIAN_POINT('Ctrl Pts',(-34.6550194892076,10.7227336174029,-11.6983341944626));
#26007=CARTESIAN_POINT('Ctrl Pts',(-36.6095738700227,10.8478143907814,-10.7727336174023));
#26008=CARTESIAN_POINT('Ctrl Pts',(-35.8197142077533,11.4817645043905,-10.9904588000056));
#26009=CARTESIAN_POINT('Ctrl Pts',(-34.8207019100435,11.6483341944626,-10.7727336174029));
#26010=CARTESIAN_POINT('Ctrl Pts',(-36.8417178703408,11.1442135371056,-10.2180948773779));
#26011=CARTESIAN_POINT('Ctrl Pts',(-36.0061527172947,11.8983870794298,-10.439161626936));
#26012=CARTESIAN_POINT('Ctrl Pts',(-34.8870388756109,12.01893195191,-10.2180948773776));
#26013=CARTESIAN_POINT('Ctrl Pts',(-37.0770570386605,11.4446922420908,-9.31107830404926));
#26014=CARTESIAN_POINT('Ctrl Pts',(-36.2030730684665,12.3384327759139,-9.4822033404738));
#26015=CARTESIAN_POINT('Ctrl Pts',(-34.9542888854505,12.3946305178797,-9.31107830404939));
#26016=CARTESIAN_POINT('Ctrl Pts',(-37.1368490307002,11.5210340617088,-8.99641282927347));
#26017=CARTESIAN_POINT('Ctrl Pts',(-36.2546886211114,12.4537748504034,-9.14076955834483));
#26018=CARTESIAN_POINT('Ctrl Pts',(-34.9713749152927,12.4900832460695,-8.99641282927339));
#26019=CARTESIAN_POINT('Ctrl Pts',(-37.2168322756965,11.6231558718975,-8.35449039088781));
#26020=CARTESIAN_POINT('Ctrl Pts',(-36.3245787042157,12.6099538847862,-8.43215085130202));
#26021=CARTESIAN_POINT('Ctrl Pts',(-34.9942307537467,12.6177695579628,-8.3544903908879));
#26022=CARTESIAN_POINT('Ctrl Pts',(-37.2370215607004,11.6489333498047,-8.02725293702977));
#26023=CARTESIAN_POINT('Ctrl Pts',(-36.3424993318365,12.6499999999592,-8.06661933627898));
#26024=CARTESIAN_POINT('Ctrl Pts',(-34.9999999999986,12.65,-8.02725293702971));
#26025=CARTESIAN_POINT('Ctrl Pts',(-37.2370215606994,11.6489333498058,-7.69999999999999));
#26026=CARTESIAN_POINT('Ctrl Pts',(-36.3424993318542,12.65,-7.69999999999999));
#26027=CARTESIAN_POINT('Ctrl Pts',(-35.,12.65,-7.69999999999999));
#26028=CARTESIAN_POINT('Ctrl Pts',(-34.1050004454305,7.65,-12.7));
#26029=CARTESIAN_POINT('Ctrl Pts',(-34.1240917710517,7.75665550347773,-12.7));
#26030=CARTESIAN_POINT('Ctrl Pts',(-34.1434686246157,7.86490613592107,-12.6965423806532));
#26031=CARTESIAN_POINT('Ctrl Pts',(-34.1630635716754,7.97437516838843,-12.689375889938));
#26032=CARTESIAN_POINT('Ctrl Pts',(-34.1827742292053,8.08449062838514,-12.6821670802511));
#26033=CARTESIAN_POINT('Ctrl Pts',(-34.2027055232168,8.19583869503812,-12.6712053060899));
#26034=CARTESIAN_POINT('Ctrl Pts',(-34.2227824776687,8.30800050757273,-12.6562735357951));
#26035=CARTESIAN_POINT('Ctrl Pts',(-34.2431276259006,8.42166061012692,-12.6411423025824));
#26036=CARTESIAN_POINT('Ctrl Pts',(-34.2636223046257,8.53615607898092,-12.6219341077272));
#26037=CARTESIAN_POINT('Ctrl Pts',(-34.2841826561185,8.65101843498767,-12.5984654868138));
#26038=CARTESIAN_POINT('Ctrl Pts',(-34.3049210732628,8.76687557166583,-12.5747936127957));
#26039=CARTESIAN_POINT('Ctrl Pts',(-34.3257262387403,8.88310560424568,-12.5467870597101));
#26040=CARTESIAN_POINT('Ctrl Pts',(-34.3465070726839,8.99919970640085,-12.5143028492565));
#26041=CARTESIAN_POINT('Ctrl Pts',(-34.3675785659692,9.11691760456874,-12.4813642855633));
#26042=CARTESIAN_POINT('Ctrl Pts',(-34.3886249626673,9.23449529826958,-12.4438217748886));
#26043=CARTESIAN_POINT('Ctrl Pts',(-34.4095472712707,9.35137976204587,-12.4015749260995));
#26044=CARTESIAN_POINT('Ctrl Pts',(-34.4222522179732,9.42235715324929,-12.3759207799732));
#26045=CARTESIAN_POINT('Ctrl Pts',(-34.4349113342375,9.49307850835849,-12.3485328867815));
#26046=CARTESIAN_POINT('Ctrl Pts',(-34.4475019469418,9.56341716182414,-12.319397662557));
#26047=CARTESIAN_POINT('Ctrl Pts',(-34.4677278324778,9.67641099200239,-12.2725940856327));
#26048=CARTESIAN_POINT('Ctrl Pts',(-34.4877731968533,9.78839632357546,-12.2212852588866));
#26049=CARTESIAN_POINT('Ctrl Pts',(-34.5075514412001,9.89888936374264,-12.1655739463846));
#26050=CARTESIAN_POINT('Ctrl Pts',(-34.5284773027894,10.0157936766117,-12.1066300283132));
#26051=CARTESIAN_POINT('Ctrl Pts',(-34.5491040392408,10.1310268984931,-12.0427576011116));
#26052=CARTESIAN_POINT('Ctrl Pts',(-34.5693295618572,10.2440187011864,-11.97414046962));
#26053=CARTESIAN_POINT('Ctrl Pts',(-34.5889672240172,10.3537263656172,-11.9075177141948));
#26054=CARTESIAN_POINT('Ctrl Pts',(-34.6082265616951,10.4613204844035,-11.8364226289622));
#26055=CARTESIAN_POINT('Ctrl Pts',(-34.6270160716463,10.5662898659801,-11.7610768920466));
#26056=CARTESIAN_POINT('Ctrl Pts',(-34.6466492876715,10.6759726916567,-11.6823479026645));
#26057=CARTESIAN_POINT('Ctrl Pts',(-34.6657693880788,10.7827889482092,-11.598977934513));
#26058=CARTESIAN_POINT('Ctrl Pts',(-34.6842760113416,10.8861779564385,-11.511275797721));
#26059=CARTESIAN_POINT('Ctrl Pts',(-34.7027826346044,10.9895669646678,-11.423573660929));
#26060=CARTESIAN_POINT('Ctrl Pts',(-34.7206756544822,11.0895280193203,-11.3315397925451));
#26061=CARTESIAN_POINT('Ctrl Pts',(-34.7378606996329,11.1855339059311,-11.2355339059344));
#26062=CARTESIAN_POINT('Ctrl Pts',(-34.7543276664658,11.2775281798313,-11.1435396320343));
#26063=CARTESIAN_POINT('Ctrl Pts',(-34.7701419696601,11.3658762863383,-11.0479135122097));
#26064=CARTESIAN_POINT('Ctrl Pts',(-34.785246776545,11.4502607243403,-10.949118583428));
#26065=CARTESIAN_POINT('Ctrl Pts',(-34.8006790532294,11.5364746034736,-10.8481817963777));
#26066=CARTESIAN_POINT('Ctrl Pts',(-34.8153706391351,11.6185505432366,-10.743937817595));
#26067=CARTESIAN_POINT('Ctrl Pts',(-34.8292691650063,11.6961959778085,-10.6369112386856));
#26068=CARTESIAN_POINT('Ctrl Pts',(-34.8427515809851,11.7715167749529,-10.5330889433564));
#26069=CARTESIAN_POINT('Ctrl Pts',(-34.8554876975223,11.8426682993994,-10.4266488425185));
#26070=CARTESIAN_POINT('Ctrl Pts',(-34.8674381023621,11.9094303708381,-10.3180893465352));
#26071=CARTESIAN_POINT('Ctrl Pts',(-34.8792760644748,11.9755642703044,-10.2105512992764));
#26072=CARTESIAN_POINT('Ctrl Pts',(-34.8903429959641,12.0373907339765,-10.1009340887766));
#26073=CARTESIAN_POINT('Ctrl Pts',(-34.9006093637268,12.0947447723694,-9.98973289376224));
#26074=CARTESIAN_POINT('Ctrl Pts',(-34.9107220598017,12.1512403092858,-9.88019620909055));
#26075=CARTESIAN_POINT('Ctrl Pts',(-34.9200579618845,12.2033962128018,-9.76912308216464));
#26076=CARTESIAN_POINT('Ctrl Pts',(-34.9285977727507,12.2511046771403,-9.65698972957955));
#26077=CARTESIAN_POINT('Ctrl Pts',(-34.9297025752325,12.2572767611162,-9.64248294387071));
#26078=CARTESIAN_POINT('Ctrl Pts',(-34.9307940663001,12.2633744796121,-9.6279584117784));
#26079=CARTESIAN_POINT('Ctrl Pts',(-34.9318722155104,12.269397662556,-9.61341716182647));
#26080=CARTESIAN_POINT('Ctrl Pts',(-34.9403421036365,12.316715496867,-9.49918180449091));
#26081=CARTESIAN_POINT('Ctrl Pts',(-34.9479943268078,12.3594653682635,-9.383941816075));
#26082=CARTESIAN_POINT('Ctrl Pts',(-34.954834960747,12.3976812193477,-9.26823244742841));
#26083=CARTESIAN_POINT('Ctrl Pts',(-34.9615774991121,12.4353490501917,-9.15418236607224));
#26084=CARTESIAN_POINT('Ctrl Pts',(-34.9675315745766,12.4686120581704,-9.03967670402811));
#26085=CARTESIAN_POINT('Ctrl Pts',(-34.9727114374621,12.4975498540576,-8.92521241468831));
#26086=CARTESIAN_POINT('Ctrl Pts',(-34.9764826831285,12.5186182760887,-8.84187566144388));
#26087=CARTESIAN_POINT('Ctrl Pts',(-34.9798437166779,12.5373950091753,-8.75856053416942));
#26088=CARTESIAN_POINT('Ctrl Pts',(-34.9828028345235,12.5539264020161,-8.67545161008097));
#26089=CARTESIAN_POINT('Ctrl Pts',(-34.9868997756487,12.5768143526564,-8.56038611193321));
#26090=CARTESIAN_POINT('Ctrl Pts',(-34.990225993079,12.5953965821887,-8.44571986738742));
#26091=CARTESIAN_POINT('Ctrl Pts',(-34.9928202536293,12.6098896651052,-8.3319284840402));
#26092=CARTESIAN_POINT('Ctrl Pts',(-34.9953898541122,12.6242449822129,-8.21921875889255));
#26093=CARTESIAN_POINT('Ctrl Pts',(-34.997241381576,12.6345887162122,-8.10736762720722));
#26094=CARTESIAN_POINT('Ctrl Pts',(-34.99841929959,12.6411692670538,-7.99680400773782));
#26095=CARTESIAN_POINT('Ctrl Pts',(-34.999485598848,12.6471262491157,-7.89671732598147));
#26096=CARTESIAN_POINT('Ctrl Pts',(-35.,12.65,-7.79768544011281));
#26097=CARTESIAN_POINT('Ctrl Pts',(-35.,12.65,-7.7));
#26098=CARTESIAN_POINT('Origin',(-35.,7.65,-7.7));
#26099=CARTESIAN_POINT('Origin',(-17.9697662756086,7.65,-7.7));
#26100=CARTESIAN_POINT('Ctrl Pts',(-17.9697662756086,12.65,-7.7));
#26101=CARTESIAN_POINT('Ctrl Pts',(-17.9697662756086,12.65,-12.7));
#26102=CARTESIAN_POINT('Ctrl Pts',(-17.9697662756086,7.65,-12.7));
#26103=CARTESIAN_POINT('Ctrl Pts',(-17.8786433834317,12.65,-7.82930352963403));
#26104=CARTESIAN_POINT('Ctrl Pts',(-17.8797974234738,12.5223340542632,-12.7));
#26105=CARTESIAN_POINT('Ctrl Pts',(-17.5769226509335,7.65000000135137,-12.7));
#26106=CARTESIAN_POINT('Ctrl Pts',(-17.7836615819991,12.6532040193819,-7.96407165192472));
#26107=CARTESIAN_POINT('Ctrl Pts',(-17.7621458420662,12.4006679911028,-12.7));
#26108=CARTESIAN_POINT('Ctrl Pts',(-17.1871178707085,7.68525114336134,-12.7));
#26109=CARTESIAN_POINT('Ctrl Pts',(-17.6839681951541,12.6595351585866,-8.1049008253337));
#26110=CARTESIAN_POINT('Ctrl Pts',(-17.617785931914,12.2921100651331,-12.7));
#26111=CARTESIAN_POINT('Ctrl Pts',(-16.8005208252602,7.75488674445212,-12.7));
#26112=CARTESIAN_POINT('Origin',(-16.8005208252602,7.75488674445212,-7.7));
#26113=CARTESIAN_POINT('Ctrl Pts',(-17.6839681951541,12.6595351585866,-8.1049008253337));
#26114=CARTESIAN_POINT('Ctrl Pts',(-17.617785931914,12.2921100651331,-12.7));
#26115=CARTESIAN_POINT('Ctrl Pts',(-16.8005208252602,7.75488674445212,-12.7));
#26116=CARTESIAN_POINT('Ctrl Pts',(-17.5771561971189,12.6663183729863,-8.25578591414162));
#26117=CARTESIAN_POINT('Ctrl Pts',(-17.6289209271536,12.15209358202,-12.6705607830935));
#26118=CARTESIAN_POINT('Ctrl Pts',(-16.5687698658206,7.82950008896473,-12.7));
#26119=CARTESIAN_POINT('Ctrl Pts',(-17.4598936459479,12.6763099143986,-8.4291699077561));
#26120=CARTESIAN_POINT('Ctrl Pts',(-17.5782752445044,12.013218333086,-12.6289627825015));
#26121=CARTESIAN_POINT('Ctrl Pts',(-16.3458206877549,7.93940906195254,-12.7125729192313));
#26122=CARTESIAN_POINT('Ctrl Pts',(-17.1998888841757,12.7012381622111,-8.81799222980845));
#26123=CARTESIAN_POINT('Ctrl Pts',(-17.3662719339354,11.7832074074828,-12.5586541771898));
#26124=CARTESIAN_POINT('Ctrl Pts',(-15.9135842369118,8.21361978075451,-12.7584916190665));
#26125=CARTESIAN_POINT('Ctrl Pts',(-17.0571441869795,12.7161912440269,-9.03346319244822));
#26126=CARTESIAN_POINT('Ctrl Pts',(-17.2098830150751,11.6912659624442,-12.5297453843541));
#26127=CARTESIAN_POINT('Ctrl Pts',(-15.7043519652416,8.37810368845214,-12.7918748657651));
#26128=CARTESIAN_POINT('Ctrl Pts',(-16.7409348394768,12.7502046526729,-9.50326306101304));
#26129=CARTESIAN_POINT('Ctrl Pts',(-16.8220227865866,11.5747870675349,-12.5075269194728));
#26130=CARTESIAN_POINT('Ctrl Pts',(-15.2973824695118,8.75225117524501,-12.8769706424726));
#26131=CARTESIAN_POINT('Ctrl Pts',(-16.5677687617376,12.7692327202595,-9.75697351939234));
#26132=CARTESIAN_POINT('Ctrl Pts',(-16.5938533615665,11.5484270002405,-12.5132837475877));
#26133=CARTESIAN_POINT('Ctrl Pts',(-15.1005185854711,8.96155992656123,-12.9286629823072));
#26134=CARTESIAN_POINT('Ctrl Pts',(-16.1973605868977,12.8095022395595,-10.2822412234627));
#26135=CARTESIAN_POINT('Ctrl Pts',(-16.1105390364457,11.5605687167964,-12.5667216513117));
#26136=CARTESIAN_POINT('Ctrl Pts',(-14.7269130064669,9.40452463144808,-13.0449250534816));
#26137=CARTESIAN_POINT('Ctrl Pts',(-15.998896046405,12.8308799157883,-10.5556257828799));
#26138=CARTESIAN_POINT('Ctrl Pts',(-15.8541814468065,11.5962530038123,-12.6128339202831));
#26139=CARTESIAN_POINT('Ctrl Pts',(-14.5485608660789,9.63967907679423,-13.1098286335377));
#26140=CARTESIAN_POINT('Ctrl Pts',(-15.573397634044,12.87554153991,-11.1172708424565));
#26141=CARTESIAN_POINT('Ctrl Pts',(-15.3333943403924,11.7180448914412,-12.7448433212756));
#26142=CARTESIAN_POINT('Ctrl Pts',(-14.2053991112487,10.1309569358866,-13.2515258205145));
#26143=CARTESIAN_POINT('Ctrl Pts',(-15.3463523739799,12.8988286442761,-11.4055303863304));
#26144=CARTESIAN_POINT('Ctrl Pts',(-15.0678470816742,11.8029800287259,-12.829901640401));
#26145=CARTESIAN_POINT('Ctrl Pts',(-14.0406084083384,10.3871150892957,-13.3283300196113));
#26146=CARTESIAN_POINT('Ctrl Pts',(-14.8628607081636,12.9468769497922,-11.9898209804218));
#26147=CARTESIAN_POINT('Ctrl Pts',(-14.5414297968434,12.0098985669587,-13.0365151718341));
#26148=CARTESIAN_POINT('Ctrl Pts',(-13.722266387327,10.9156464454547,-13.4931147637453));
#26149=CARTESIAN_POINT('Ctrl Pts',(-14.6063601361617,12.9716383743557,-12.2857804525791));
#26150=CARTESIAN_POINT('Ctrl Pts',(-14.2788785559446,12.1317581217325,-13.1579975413437));
#26151=CARTESIAN_POINT('Ctrl Pts',(-13.568789765243,11.1880221188636,-13.5811194448631));
#26152=CARTESIAN_POINT('Ctrl Pts',(-13.8028973740084,13.0467768755486,-13.1649381963916));
#26153=CARTESIAN_POINT('Ctrl Pts',(-13.5233243480122,12.5265039443217,-13.5643970241019));
#26154=CARTESIAN_POINT('Ctrl Pts',(-13.1270902810059,12.0145456291354,-13.8587218607487));
#26155=CARTESIAN_POINT('Ctrl Pts',(-13.2185390460369,13.0982771986992,-13.7423443295298));
#26156=CARTESIAN_POINT('Ctrl Pts',(-13.0367148554586,12.8398642053082,-13.902698193065));
#26157=CARTESIAN_POINT('Ctrl Pts',(-12.8553998351504,12.5811750652043,-14.0626030106305));
#26158=CARTESIAN_POINT('Ctrl Pts',(-12.6003906189451,13.15,-14.2875));
#26159=CARTESIAN_POINT('Ctrl Pts',(-12.6003906189451,13.15,-14.2875));
#26160=CARTESIAN_POINT('Ctrl Pts',(-12.6003906189451,13.15,-14.2875));
#26161=CARTESIAN_POINT('Origin',(30.6683956091404,-22.9,-37.7192193816529));
#26162=CARTESIAN_POINT('Origin',(30.6683956091404,-21.9,-37.7192193816529));
#26163=CARTESIAN_POINT('Origin',(30.6683956091404,-7.90000000000001,-37.7192193816529));
#26164=CARTESIAN_POINT('Origin',(30.6683956091404,-7.90000000000001,-37.7192193816529));
#26165=CARTESIAN_POINT('Origin',(30.6683956091404,-7.90000000000001,-37.7192193816529));
#26166=CARTESIAN_POINT('Origin',(30.6683956091404,-7.90000000000001,-37.7192193816529));
#26167=CARTESIAN_POINT('Ctrl Pts',(28.0510228507777,7.65,-23.1857967818223));
#26168=CARTESIAN_POINT('Ctrl Pts',(28.0844275796734,7.7353016499602,-23.2436554694827));
#26169=CARTESIAN_POINT('Ctrl Pts',(28.1153375201382,7.82187906280401,-23.3041082955204));
#26170=CARTESIAN_POINT('Ctrl Pts',(28.1434170892388,7.90943093574576,-23.3670765172878));
#26171=CARTESIAN_POINT('Ctrl Pts',(28.1716624715019,7.99749981280845,-23.4304165738206));
#26172=CARTESIAN_POINT('Ctrl Pts',(28.197043746198,8.08655451224417,-23.4963017794781));
#26173=CARTESIAN_POINT('Ctrl Pts',(28.2192417703178,8.17626003478879,-23.5646134256713));
#26174=CARTESIAN_POINT('Ctrl Pts',(28.2417363220814,8.26716386971868,-23.6338375986452));
#26175=CARTESIAN_POINT('Ctrl Pts',(28.2609617599813,8.35873581947972,-23.7055534235965));
#26176=CARTESIAN_POINT('Ctrl Pts',(28.2766124705147,8.45060120069494,-23.7795984912424));
#26177=CARTESIAN_POINT('Ctrl Pts',(28.2923987261027,8.5432621942306,-23.854284836019));
#26178=CARTESIAN_POINT('Ctrl Pts',(28.3045478312848,8.63622142493773,-23.9313408096329));
#26179=CARTESIAN_POINT('Ctrl Pts',(28.3127765977406,8.72907194030321,-24.0105618721263));
#26180=CARTESIAN_POINT('Ctrl Pts',(28.3211204590885,8.82322114607408,-24.0908909912993));
#26181=CARTESIAN_POINT('Ctrl Pts',(28.3254332730576,8.91725821818117,-24.1734460255676));
#26182=CARTESIAN_POINT('Ctrl Pts',(28.3254548896355,9.01074085423544,-24.2579771641579));
#26183=CARTESIAN_POINT('Ctrl Pts',(28.3254680161731,9.06750762558578,-24.3093081922384));
#26184=CARTESIAN_POINT('Ctrl Pts',(28.3238994826631,9.12406962268099,-24.3613671988867));
#26185=CARTESIAN_POINT('Ctrl Pts',(28.3206978531272,9.18032554010316,-24.4140922623098));
#26186=CARTESIAN_POINT('Ctrl Pts',(28.3155546727241,9.27069649926788,-24.4987911663879));
#26187=CARTESIAN_POINT('Ctrl Pts',(28.3061939676322,9.36026087469145,-24.5851956030667));
#26188=CARTESIAN_POINT('Ctrl Pts',(28.2925532092166,9.44863173534083,-24.6729917414413));
#26189=CARTESIAN_POINT('Ctrl Pts',(28.2781209564053,9.54213024643462,-24.7658821824474));
#26190=CARTESIAN_POINT('Ctrl Pts',(28.2588971002586,9.63429224123211,-24.8603303412872));
#26191=CARTESIAN_POINT('Ctrl Pts',(28.2348621924407,9.72466157884118,-24.9559349227747));
#26192=CARTESIAN_POINT('Ctrl Pts',(28.2115258659228,9.81240430644562,-25.048760730434));
#26193=CARTESIAN_POINT('Ctrl Pts',(28.1836544212187,9.89845664841724,-25.1426761425918));
#26194=CARTESIAN_POINT('Ctrl Pts',(28.1512797309383,9.98240976055632,-25.2372930079781));
#26195=CARTESIAN_POINT('Ctrl Pts',(28.1174513187192,10.0701326224562,-25.3361584580394));
#26196=CARTESIAN_POINT('Ctrl Pts',(28.0787058854849,10.1555628405819,-25.4357893354192));
#26197=CARTESIAN_POINT('Ctrl Pts',(28.0351352627429,10.2382519911843,-25.5357270766966));
#26198=CARTESIAN_POINT('Ctrl Pts',(27.9915646400008,10.3209411417866,-25.6356648179739));
#26199=CARTESIAN_POINT('Ctrl Pts',(27.9431689853593,10.4008886608129,-25.735908822037));
#26200=CARTESIAN_POINT('Ctrl Pts',(27.8900946950471,10.4776728891621,-25.8359932278618));
#26201=CARTESIAN_POINT('Ctrl Pts',(27.8392381176804,10.5512486831409,-25.9318955997651));
#26202=CARTESIAN_POINT('Ctrl Pts',(27.7840942821539,10.621908321042,-26.0276359145594));
#26203=CARTESIAN_POINT('Ctrl Pts',(27.7249647482256,10.6893978697086,-26.1228104151325));
#26204=CARTESIAN_POINT('Ctrl Pts',(27.6645532954511,10.758350581005,-26.2200482836684));
#26205=CARTESIAN_POINT('Ctrl Pts',(27.599981719273,10.8239938235519,-26.3166949905683));
#26206=CARTESIAN_POINT('Ctrl Pts',(27.5316126971157,10.8860936071058,-26.4123295283466));
#26207=CARTESIAN_POINT('Ctrl Pts',(27.4652905845885,10.9463341766329,-26.5051008504436));
#26208=CARTESIAN_POINT('Ctrl Pts',(27.3953955609761,11.0032402174329,-26.5969193200274));
#26209=CARTESIAN_POINT('Ctrl Pts',(27.3222903013767,11.0566356322287,-26.6874162880683));
#26210=CARTESIAN_POINT('Ctrl Pts',(27.2498728975334,11.1095286434545,-26.7770617597774));
#26211=CARTESIAN_POINT('Ctrl Pts',(27.1743057875187,11.1589766249502,-26.8654101068509));
#26212=CARTESIAN_POINT('Ctrl Pts',(27.0959661336342,11.2048476203253,-26.9521242361045));
#26213=CARTESIAN_POINT('Ctrl Pts',(27.0187991035163,11.2500319976632,-27.0375403886143));
#26214=CARTESIAN_POINT('Ctrl Pts',(26.9389422930305,11.291745594055,-27.1213705893742));
#26215=CARTESIAN_POINT('Ctrl Pts',(26.8567743528488,11.329902187877,-27.2033182473963));
#26216=CARTESIAN_POINT('Ctrl Pts',(26.8461442176325,11.3348385383663,-27.2139198845252));
#26217=CARTESIAN_POINT('Ctrl Pts',(26.8354754221718,11.3397154123361,-27.2244900529138));
#26218=CARTESIAN_POINT('Ctrl Pts',(26.8247688039278,11.3445326737649,-27.2350281460392));
#26219=CARTESIAN_POINT('Ctrl Pts',(26.7406581280853,11.3823768468976,-27.3178148966883));
#26220=CARTESIAN_POINT('Ctrl Pts',(26.6542467205756,11.4165676241826,-27.3986259253561));
#26221=CARTESIAN_POINT('Ctrl Pts',(26.5660087531266,11.4471321524605,-27.4772120198674));
#26222=CARTESIAN_POINT('Ctrl Pts',(26.4790361295275,11.4772583814553,-27.5546711796333));
#26223=CARTESIAN_POINT('Ctrl Pts',(26.3902893616569,11.503861691839,-27.6299685927569));
#26224=CARTESIAN_POINT('Ctrl Pts',(26.3002237580396,11.5270057552473,-27.7028989699517));
#26225=CARTESIAN_POINT('Ctrl Pts',(26.2346506869243,11.5438559983458,-27.7559965856693));
#26226=CARTESIAN_POINT('Ctrl Pts',(26.168378582632,11.5588733791746,-27.8078401884682));
#26227=CARTESIAN_POINT('Ctrl Pts',(26.101581810231,11.5720949668051,-27.8583626330737));
#26228=CARTESIAN_POINT('Ctrl Pts',(26.0091007202041,11.59040044463,-27.9283116827057));
#26229=CARTESIAN_POINT('Ctrl Pts',(25.9156168329965,11.6052622641078,-27.995725329467));
#26230=CARTESIAN_POINT('Ctrl Pts',(25.8216098684572,11.6168536386309,-28.0604832573163));
#26231=CARTESIAN_POINT('Ctrl Pts',(25.7284964988546,11.6283348298964,-28.1246256205985));
#26232=CARTESIAN_POINT('Ctrl Pts',(25.6348702567017,11.6366076104663,-28.1861624756413));
#26233=CARTESIAN_POINT('Ctrl Pts',(25.5411803959244,11.6418706473102,-28.2450141155623));
#26234=CARTESIAN_POINT('Ctrl Pts',(25.4563685263053,11.646634962156,-28.2982890118046));
#26235=CARTESIAN_POINT('Ctrl Pts',(25.3715044622055,11.6489333498058,-28.3493639127792));
#26236=CARTESIAN_POINT('Ctrl Pts',(25.28690638949,11.6489333498058,-28.3982066328344));
#26237=CARTESIAN_POINT('Ctrl Pts',(28.0510228507777,7.65,-23.1857967818223));
#26238=CARTESIAN_POINT('Ctrl Pts',(28.0510228507777,7.65,-23.1857967818223));
#26239=CARTESIAN_POINT('Ctrl Pts',(28.0510228507777,7.65,-23.1857967818223));
#26240=CARTESIAN_POINT('Ctrl Pts',(28.2560501075485,8.17355351674861,-23.5409144074858));
#26241=CARTESIAN_POINT('Ctrl Pts',(28.1827326335689,8.23864736688846,-23.4139248174704));
#26242=CARTESIAN_POINT('Ctrl Pts',(28.1096109945771,8.30461645762955,-23.2872744236039));
#26243=CARTESIAN_POINT('Ctrl Pts',(28.3482211841548,8.69671236121348,-23.9608326462974));
#26244=CARTESIAN_POINT('Ctrl Pts',(28.226033252186,8.83304537535178,-23.6960674267144));
#26245=CARTESIAN_POINT('Ctrl Pts',(28.0554533489517,8.95873944331314,-23.4537438809043));
#26246=CARTESIAN_POINT('Ctrl Pts',(28.2931745221,9.66393871899236,-24.8673518783231));
#26247=CARTESIAN_POINT('Ctrl Pts',(28.1174229188328,9.96758997398111,-24.3450248584826));
#26248=CARTESIAN_POINT('Ctrl Pts',(27.72987126818,10.1680948803378,-23.8916820224642));
#26249=CARTESIAN_POINT('Ctrl Pts',(28.1459414742105,10.1075313875402,-25.3535322712673));
#26250=CARTESIAN_POINT('Ctrl Pts',(27.9614466252583,10.5146815062458,-24.7177754547341));
#26251=CARTESIAN_POINT('Ctrl Pts',(27.4585643389691,10.7227336174028,-24.1629601490677));
#26252=CARTESIAN_POINT('Ctrl Pts',(27.6342479158847,10.8478143907813,-26.3184541844604));
#26253=CARTESIAN_POINT('Ctrl Pts',(27.4278736239269,11.4817645043905,-25.5255530602085));
#26254=CARTESIAN_POINT('Ctrl Pts',(26.739811935895,11.6483341944627,-24.7692456230009));
#26255=CARTESIAN_POINT('Ctrl Pts',(27.2699886772589,11.1442135371053,-26.7968161560865));
#26256=CARTESIAN_POINT('Ctrl Pts',(27.0436555217853,11.8983870794305,-25.9626621322513));
#26257=CARTESIAN_POINT('Ctrl Pts',(26.2926491798934,12.0189319519104,-25.1040144904059));
#26258=CARTESIAN_POINT('Ctrl Pts',(26.6021588672634,11.4446922420909,-27.4541341410193));
#26259=CARTESIAN_POINT('Ctrl Pts',(26.3133655109336,12.3384327759135,-26.6116793021192));
#26260=CARTESIAN_POINT('Ctrl Pts',(25.5407747906587,12.3946305178795,-25.6157629939952));
#26261=CARTESIAN_POINT('Ctrl Pts',(26.3595465684333,11.5210340617089,-27.6632482624569));
#26262=CARTESIAN_POINT('Ctrl Pts',(26.0434829582226,12.4537748504032,-26.8270965730051));
#26263=CARTESIAN_POINT('Ctrl Pts',(25.2768095107295,12.4900832460694,-25.7878926672764));
#26264=CARTESIAN_POINT('Ctrl Pts',(25.8436170520302,11.6231558718974,-28.0534770036939));
#26265=CARTESIAN_POINT('Ctrl Pts',(25.4647461978775,12.6099538847864,-27.2419325139664));
#26266=CARTESIAN_POINT('Ctrl Pts',(24.7323162910554,12.6177695579629,-26.1286476231954));
#26267=CARTESIAN_POINT('Ctrl Pts',(25.5703157464213,11.6489333498049,-28.2345801643203));
#26268=CARTESIAN_POINT('Ctrl Pts',(25.1571469337947,12.6499999999603,-27.4402179902493));
#26269=CARTESIAN_POINT('Ctrl Pts',(24.4518049660702,12.65,-26.2972626639387));
#26270=CARTESIAN_POINT('Ctrl Pts',(25.28690638949,11.6489333498058,-28.3982066328345));
#26271=CARTESIAN_POINT('Ctrl Pts',(24.8396452750674,12.65,-27.6235276584047));
#26272=CARTESIAN_POINT('Ctrl Pts',(24.1683956091403,12.65,-26.4608891324552));
#26273=CARTESIAN_POINT('Ctrl Pts',(28.0510228507777,7.65,-23.1857967818223));
#26274=CARTESIAN_POINT('Ctrl Pts',(28.0605685135883,7.75665550347771,-23.202330354802));
#26275=CARTESIAN_POINT('Ctrl Pts',(28.0672625541792,7.86490613592101,-23.2208400119071));
#26276=CARTESIAN_POINT('Ctrl Pts',(28.0708536646936,7.97437516838833,-23.241392979204));
#26277=CARTESIAN_POINT('Ctrl Pts',(28.0744659811386,8.084490628385,-23.2620673141935));
#26278=CARTESIAN_POINT('Ctrl Pts',(28.0749384532501,8.19583869503793,-23.2848092082182));
#26279=CARTESIAN_POINT('Ctrl Pts',(28.0720456380772,8.30800050757249,-23.3096622459514));
#26280=CARTESIAN_POINT('Ctrl Pts',(28.0691141798403,8.42166061012672,-23.3348472777702));
#26281=CARTESIAN_POINT('Ctrl Pts',(28.0627267344974,8.53615607898074,-23.362200287616));
#26282=CARTESIAN_POINT('Ctrl Pts',(28.0526824883409,8.65101843498752,-23.3917403847761));
#26283=CARTESIAN_POINT('Ctrl Pts',(28.0425512526582,8.76687557166562,-23.4215363178663));
#26284=CARTESIAN_POINT('Ctrl Pts',(28.0286994489523,8.8831056042454,-23.4535573962425));
#26285=CARTESIAN_POINT('Ctrl Pts',(28.0109577144494,8.99919970640052,-23.4877962315763));
#26286=CARTESIAN_POINT('Ctrl Pts',(27.9929678281695,9.11691760456845,-23.5225139619035));
#26287=CARTESIAN_POINT('Ctrl Pts',(27.9709782585524,9.23449529826935,-23.5595119314396));
#26288=CARTESIAN_POINT('Ctrl Pts',(27.9448525685729,9.35137976204572,-23.5987546065905));
#26289=CARTESIAN_POINT('Ctrl Pts',(27.9289878996663,9.42235715324939,-23.6225844862518));
#26290=CARTESIAN_POINT('Ctrl Pts',(27.9115988465383,9.49307850835886,-23.6472415491221));
#26291=CARTESIAN_POINT('Ctrl Pts',(27.892662308567,9.56341716182476,-23.6727129516856));
#26292=CARTESIAN_POINT('Ctrl Pts',(27.8622421647305,9.67641099200318,-23.713630870836));
#26293=CARTESIAN_POINT('Ctrl Pts',(27.8278300995177,9.7883963235764,-23.7566450789865));
#26294=CARTESIAN_POINT('Ctrl Pts',(27.7894718097861,9.8988893637437,-23.8016291972841));
#26295=CARTESIAN_POINT('Ctrl Pts',(27.7488878101323,10.0157936766128,-23.8492234840522));
#26296=CARTESIAN_POINT('Ctrl Pts',(27.7038860338,10.1310268984941,-23.8990229754171));
#26297=CARTESIAN_POINT('Ctrl Pts',(27.6545746161017,10.2440187011874,-23.9508473575535));
#26298=CARTESIAN_POINT('Ctrl Pts',(27.6066964485132,10.3537263656184,-24.0011654495676));
#26299=CARTESIAN_POINT('Ctrl Pts',(27.5547559674564,10.4613204844049,-24.0533920678732));
#26300=CARTESIAN_POINT('Ctrl Pts',(27.4988994001961,10.5662898659816,-24.1073371292734));
#26301=CARTESIAN_POINT('Ctrl Pts',(27.4405347033895,10.675972691658,-24.1637044878002));
#26302=CARTESIAN_POINT('Ctrl Pts',(27.3778942432613,10.7827889482103,-24.2219479645514));
#26303=CARTESIAN_POINT('Ctrl Pts',(27.3111952764647,10.8861779564394,-24.2818262388311));
#26304=CARTESIAN_POINT('Ctrl Pts',(27.244496309668,10.9895669646686,-24.3417045131109));
#26305=CARTESIAN_POINT('Ctrl Pts',(27.173739151578,11.0895280193209,-24.4032172570673));
#26306=CARTESIAN_POINT('Ctrl Pts',(27.0991881374357,11.1855339059316,-24.4661028860382));
#26307=CARTESIAN_POINT('Ctrl Pts',(27.0277522426516,11.2775281798321,-24.526360834589));
#26308=CARTESIAN_POINT('Ctrl Pts',(26.952844745215,11.3658762863394,-24.587869482811));
#26309=CARTESIAN_POINT('Ctrl Pts',(26.8748382305671,11.4502607243417,-24.6503480936837));
#26310=CARTESIAN_POINT('Ctrl Pts',(26.7951405471474,11.5364746034749,-24.7141812308558));
#26311=CARTESIAN_POINT('Ctrl Pts',(26.712208406283,11.6185505432378,-24.7790265068635));
#26312=CARTESIAN_POINT('Ctrl Pts',(26.626469933003,11.6961959778096,-24.8445762727979));
#26313=CARTESIAN_POINT('Ctrl Pts',(26.543298395758,11.771516774954,-24.9081635352047));
#26314=CARTESIAN_POINT('Ctrl Pts',(26.4574866227195,11.8426682994006,-24.9724133860907));
#26315=CARTESIAN_POINT('Ctrl Pts',(26.3694465437957,11.9094303708394,-25.0370424882595));
#26316=CARTESIAN_POINT('Ctrl Pts',(26.2822348440526,11.9755642703057,-25.1010634878077));
#26317=CARTESIAN_POINT('Ctrl Pts',(26.1928370208126,12.0373907339777,-25.1654563368694));
#26318=CARTESIAN_POINT('Ctrl Pts',(26.1016671448805,12.0947447723705,-25.2299478696638));
#26319=CARTESIAN_POINT('Ctrl Pts',(26.0118619413461,12.1512403092868,-25.2934740637013));
#26320=CARTESIAN_POINT('Ctrl Pts',(25.9203377427922,12.2033962128026,-25.3570957555352));
#26321=CARTESIAN_POINT('Ctrl Pts',(25.8274973162754,12.2511046771409,-25.4205581249814));
#26322=CARTESIAN_POINT('Ctrl Pts',(25.8154864725656,12.2572767611166,-25.428768304851));
#26323=CARTESIAN_POINT('Ctrl Pts',(25.8034536043298,12.2633744796123,-25.4369758298894));
#26324=CARTESIAN_POINT('Ctrl Pts',(25.7913995870742,12.269397662556,-25.4451801594703));
#26325=CARTESIAN_POINT('Ctrl Pts',(25.6967038096758,12.3167154968663,-25.5096329764217));
#26326=CARTESIAN_POINT('Ctrl Pts',(25.6007291637629,12.3594653682623,-25.5738799902906));
#26327=CARTESIAN_POINT('Ctrl Pts',(25.50394222803,12.397681219346,-25.6376588373824));
#26328=CARTESIAN_POINT('Ctrl Pts',(25.4085432294565,12.4353490501894,-25.7005230875694));
#26329=CARTESIAN_POINT('Ctrl Pts',(25.3123554549835,12.4686120581676,-25.7629322991986));
#26330=CARTESIAN_POINT('Ctrl Pts',(25.2158164040339,12.4975498540546,-25.8246503367143));
#26331=CARTESIAN_POINT('Ctrl Pts',(25.1455302814851,12.5186182760868,-25.8695847078898));
#26332=CARTESIAN_POINT('Ctrl Pts',(25.0750577815173,12.5373950091745,-25.914153011966));
#26333=CARTESIAN_POINT('Ctrl Pts',(25.0045629008949,12.5539264020161,-25.9582701452394));
#26334=CARTESIAN_POINT('Ctrl Pts',(24.906961726961,12.5768143526567,-26.0193509494066));
#26335=CARTESIAN_POINT('Ctrl Pts',(24.8093209549414,12.5953965821892,-26.0795646604735));
#26336=CARTESIAN_POINT('Ctrl Pts',(24.7120718565046,12.6098896651059,-26.1387070476885));
#26337=CARTESIAN_POINT('Ctrl Pts',(24.6157471715131,12.6242449822136,-26.1972872495588));
#26338=CARTESIAN_POINT('Ctrl Pts',(24.519807013762,12.6345887162129,-26.2548162852217));
#26339=CARTESIAN_POINT('Ctrl Pts',(24.4246450695727,12.6411692670544,-26.3111182018807));
#26340=CARTESIAN_POINT('Ctrl Pts',(24.3385006102231,12.6471262491159,-26.3620849850025));
#26341=CARTESIAN_POINT('Ctrl Pts',(24.252993681855,12.65,-26.4120464124005));
#26342=CARTESIAN_POINT('Ctrl Pts',(24.1683956091403,12.65,-26.4608891324552));
#26343=CARTESIAN_POINT('Origin',(24.1683956091403,7.65,-26.4608891324553));
#26344=CARTESIAN_POINT('Origin',(15.6532787469445,7.65,-11.7122740947458));
#26345=CARTESIAN_POINT('Ctrl Pts',(15.6532787469445,12.65,-11.7122740947458));
#26346=CARTESIAN_POINT('Ctrl Pts',(19.9834057658667,12.65,-9.21227409474583));
#26347=CARTESIAN_POINT('Ctrl Pts',(19.9834057658667,7.65,-9.21227409474583));
#26348=CARTESIAN_POINT('Ctrl Pts',(15.7196974423161,12.65,-11.5687075904364));
#26349=CARTESIAN_POINT('Ctrl Pts',(19.9384213397983,12.5223340542639,-9.13435878324517));
#26350=CARTESIAN_POINT('Ctrl Pts',(19.7869839535292,7.65000000135137,-8.8720615360625));
#26351=CARTESIAN_POINT('Ctrl Pts',(15.7889191591276,12.6532040193816,-11.4190668763549));
#26352=CARTESIAN_POINT('Ctrl Pts',(19.8795955490932,12.4006679911038,-9.03246952495588));
#26353=CARTESIAN_POINT('Ctrl Pts',(19.5920815634166,7.68525114336099,-8.53448069387081));
#26354=CARTESIAN_POINT('Ctrl Pts',(15.8610341074696,12.6595351585866,-11.2623152840526));
#26355=CARTESIAN_POINT('Ctrl Pts',(19.8074155940194,12.2921100651331,-8.90745017547355));
#26356=CARTESIAN_POINT('Ctrl Pts',(19.3987830406925,7.75488674445212,-8.19967783148469));
#26357=CARTESIAN_POINT('Origin',(15.0686560217703,7.75488674445212,-10.6996778314847));
#26358=CARTESIAN_POINT('Ctrl Pts',(15.8610341074696,12.6595351585866,-11.2623152840526));
#26359=CARTESIAN_POINT('Ctrl Pts',(19.8074155940194,12.2921100651332,-8.90745017547354));
#26360=CARTESIAN_POINT('Ctrl Pts',(19.3987830406925,7.75488674445212,-8.19967783148469));
#26361=CARTESIAN_POINT('Ctrl Pts',(15.9382984284129,12.6663183729861,-11.0943708359216));
#26362=CARTESIAN_POINT('Ctrl Pts',(19.7874879819338,12.1520935820195,-8.93181297267561));
#26363=CARTESIAN_POINT('Ctrl Pts',(19.2829075609725,7.82950008896404,-7.99897561325821));
#26364=CARTESIAN_POINT('Ctrl Pts',(16.0298220959059,12.6763099143987,-10.9061264908871));
#26365=CARTESIAN_POINT('Ctrl Pts',(19.7261402153455,12.0132183330864,-8.90875152520499));
#26366=CARTESIAN_POINT('Ctrl Pts',(19.1823214393941,7.93940906195289,-7.79960950168563));
#26367=CARTESIAN_POINT('Ctrl Pts',(16.236549723476,12.701238162211,-10.4865446010616));
#26368=CARTESIAN_POINT('Ctrl Pts',(19.5592495217588,11.7832074074825,-8.76030557522187));
#26369=CARTESIAN_POINT('Ctrl Pts',(19.0059699745382,8.21361978075416,-7.40232240489545));
#26370=CARTESIAN_POINT('Ctrl Pts',(16.3517807023014,12.7161912440271,-10.2551885857138));
#26371=CARTESIAN_POINT('Ctrl Pts',(19.4560193133398,11.6912659624446,-8.63932319503599));
#26372=CARTESIAN_POINT('Ctrl Pts',(18.9302645784051,8.37810368845214,-7.2044303189888));
#26373=CARTESIAN_POINT('Ctrl Pts',(16.6005346494223,12.7502046526726,-9.74644332358053));
#26374=CARTESIAN_POINT('Ctrl Pts',(19.2428474440738,11.5747870675345,-8.3145356164884));
#26375=CARTESIAN_POINT('Ctrl Pts',(18.8004749349236,8.752251175245,-6.80943650876738));
#26376=CARTESIAN_POINT('Ctrl Pts',(16.7336713127152,12.7692327202591,-9.46962187199463));
#26377=CARTESIAN_POINT('Ctrl Pts',(19.1337482909567,11.5484270002398,-8.11405668399569));
#26378=CARTESIAN_POINT('Ctrl Pts',(18.7468098723811,8.96155992656123,-6.61310121418329));
#26379=CARTESIAN_POINT('Ctrl Pts',(17.0033624008067,12.8095022395598,-8.8862051307789));
#26380=CARTESIAN_POINT('Ctrl Pts',(18.9383697105472,11.5605687167971,-7.66877524856764));
#26381=CARTESIAN_POINT('Ctrl Pts',(18.6606929900126,9.40452463144807,-6.23141825618296));
#26382=CARTESIAN_POINT('Ctrl Pts',(17.1408881040185,12.8308799157881,-8.57763751725331));
#26383=CARTESIAN_POINT('Ctrl Pts',(18.8501253120837,11.5962530038116,-7.42370692900014));
#26384=CARTESIAN_POINT('Ctrl Pts',(18.6277250689438,9.63967907679459,-6.04450898175927));
#26385=CARTESIAN_POINT('Ctrl Pts',(17.4145377873414,12.8755415399101,-7.92832255308998));
#26386=CARTESIAN_POINT('Ctrl Pts',(18.7040552536722,11.7180448914419,-6.90668736438696));
#26387=CARTESIAN_POINT('Ctrl Pts',(18.5788575550954,10.1309569358863,-5.67647359098107));
#26388=CARTESIAN_POINT('Ctrl Pts',(17.5506552451877,12.8988286442756,-7.58756581812893));
#26389=CARTESIAN_POINT('Ctrl Pts',(18.6449442894794,11.8029800287248,-6.63418753286814));
#26390=CARTESIAN_POINT('Ctrl Pts',(18.5629765911754,10.3871150892957,-5.49535855640502));
#26391=CARTESIAN_POINT('Ctrl Pts',(17.8149199099546,12.9468769497926,-6.87670445596825));
#26392=CARTESIAN_POINT('Ctrl Pts',(18.560668214052,12.0098985669597,-6.07499002549749));
#26393=CARTESIAN_POINT('Ctrl Pts',(18.5465133552458,10.9156464454547,-5.13727390704943));
#26394=CARTESIAN_POINT('Ctrl Pts',(17.9429780453325,12.9716383743554,-6.50658870845175));
#26395=CARTESIAN_POINT('Ctrl Pts',(18.5345994117103,12.1317581217343,-5.78687279633148));
#26396=CARTESIAN_POINT('Ctrl Pts',(18.5459893337037,11.1880221188647,-4.96035691287977));
#26397=CARTESIAN_POINT('Ctrl Pts',(18.3026196043319,13.0467768755492,-5.37119067352287));
#26398=CARTESIAN_POINT('Ctrl Pts',(18.5087745838942,12.5265039443181,-4.92934391693923));
#26399=CARTESIAN_POINT('Ctrl Pts',(18.5655503358942,12.0145456291332,-4.43903273074705));
#26400=CARTESIAN_POINT('Ctrl Pts',(18.5104888199441,13.0982771986907,-4.57641845002038));
#26401=CARTESIAN_POINT('Ctrl Pts',(18.5584472440761,12.8398642052624,-4.33877715016644));
#26402=CARTESIAN_POINT('Ctrl Pts',(18.6062713681263,12.5811750651764,-4.10180132768386));
#26403=CARTESIAN_POINT('Ctrl Pts',(18.6735332660427,13.15,-3.76850837361349));
#26404=CARTESIAN_POINT('Ctrl Pts',(18.6735332660427,13.15,-3.76850837361349));
#26405=CARTESIAN_POINT('Ctrl Pts',(18.6735332660427,13.15,-3.76850837361349));
#26406=CARTESIAN_POINT('Ctrl Pts',(-2.59826221543221,7.75488674445212,-20.8996778314848));
#26407=CARTESIAN_POINT('Ctrl Pts',(-2.18962966210527,12.2921100651332,-21.6074501754737));
#26408=CARTESIAN_POINT('Ctrl Pts',(1.82293408768471,12.6595351585866,-19.3672161093864));
#26409=CARTESIAN_POINT('Ctrl Pts',(-2.71151859288215,7.82781362133594,-20.7035120314603));
#26410=CARTESIAN_POINT('Ctrl Pts',(-2.15923311032346,12.1550958708992,-21.6024826099445));
#26411=CARTESIAN_POINT('Ctrl Pts',(1.6433377752248,12.6661532847417,-19.3505719365413));
#26412=CARTESIAN_POINT('Ctrl Pts',(-2.83631932057571,7.93905335192905,-20.5122897107496));
#26413=CARTESIAN_POINT('Ctrl Pts',(-2.14758977172822,12.0132242375897,-21.5382097423197));
#26414=CARTESIAN_POINT('Ctrl Pts',(1.43050996215087,12.6762775771012,-19.3353172528801));
#26415=CARTESIAN_POINT('Ctrl Pts',(-3.09542191664885,8.21703647488254,-20.1567883096311));
#26416=CARTESIAN_POINT('Ctrl Pts',(-2.19372722643324,11.7807433434263,-21.3161401924937));
#26417=CARTESIAN_POINT('Ctrl Pts',(0.957692517741071,12.7015487707907,-19.3041728222174));
#26418=CARTESIAN_POINT('Ctrl Pts',(-3.22938372453809,8.38258529097424,-19.9922277562922));
#26419=CARTESIAN_POINT('Ctrl Pts',(-2.24796197710858,11.6893488147428,-21.1648941602397));
#26420=CARTESIAN_POINT('Ctrl Pts',(0.698469651424131,12.7165986624447,-19.2882015806242));
#26421=CARTESIAN_POINT('Ctrl Pts',(-3.50504758868887,8.75509815651651,-19.6844217444045));
#26422=CARTESIAN_POINT('Ctrl Pts',(-2.4224500983523,11.5743897252589,-20.8193710973479));
#26423=CARTESIAN_POINT('Ctrl Pts',(0.136230369374985,12.7504634691454,-19.2493934193698));
#26424=CARTESIAN_POINT('Ctrl Pts',(-3.64702760625654,8.96258837046762,-19.5409680384734));
#26425=CARTESIAN_POINT('Ctrl Pts',(-2.54036678451312,11.548164861387,-20.626405138958));
#26426=CARTESIAN_POINT('Ctrl Pts',(-0.167426378826852,12.7693262151714,
-19.2265008823239));
#26427=CARTESIAN_POINT('Ctrl Pts',(-3.93711590576484,9.4097722276261,-19.2733814592121));
#26428=CARTESIAN_POINT('Ctrl Pts',(-2.8313443108564,11.5609929861842,-20.231002285367));
#26429=CARTESIAN_POINT('Ctrl Pts',(-0.813546547001557,12.8099792937463,
-19.1677164203027));
#26430=CARTESIAN_POINT('Ctrl Pts',(-4.08311993398416,9.64614677008682,-19.151111740647));
#26431=CARTESIAN_POINT('Ctrl Pts',(-3.00067975712713,11.5974627760305,-20.0312189608217));
#26432=CARTESIAN_POINT('Ctrl Pts',(-1.15122301518874,12.8314678879227,-19.132229841979));
#26433=CARTESIAN_POINT('Ctrl Pts',(-4.52470127695561,10.3837101835134,-18.8120550761505));
#26434=CARTESIAN_POINT('Ctrl Pts',(-3.55592923968279,11.7789057456676,-19.4620646336976));
#26435=CARTESIAN_POINT('Ctrl Pts',(-2.20078434896851,12.8985191081262,-19.0002424448541));
#26436=CARTESIAN_POINT('Ctrl Pts',(-4.82372987872531,10.9130303131124,-18.6226026951196));
#26437=CARTESIAN_POINT('Ctrl Pts',(-4.00562246697594,11.9964940699711,-19.0995737130823));
#26438=CARTESIAN_POINT('Ctrl Pts',(-2.94963680022586,12.9466391191654,-18.8775777835082));
#26439=CARTESIAN_POINT('Ctrl Pts',(-5.43715525037156,12.0122001031275,-18.2984083796858));
#26440=CARTESIAN_POINT('Ctrl Pts',(-4.98336945256202,12.525352930137,-18.4949411801501));
#26441=CARTESIAN_POINT('Ctrl Pts',(-4.49642737856456,13.0465636459473,-18.5369007865598));
#26442=CARTESIAN_POINT('Ctrl Pts',(-5.75173970056742,12.5827074287695,-18.1641123299857));
#26443=CARTESIAN_POINT('Ctrl Pts',(-5.52318791400461,12.8406828545358,-18.2409857769472));
#26444=CARTESIAN_POINT('Ctrl Pts',(-5.29401344660782,13.098413834845,-18.318068662753));
#26445=CARTESIAN_POINT('Ctrl Pts',(-6.07314264709754,13.15,-18.0560083736136));
#26446=CARTESIAN_POINT('Ctrl Pts',(-6.07314264709754,13.15,-18.0560083736136));
#26447=CARTESIAN_POINT('Ctrl Pts',(-6.07314264709754,13.15,-18.0560083736136));
#26448=CARTESIAN_POINT('Origin',(1.73186480348997,7.75488674445212,-18.3996778314848));
#26449=CARTESIAN_POINT('Ctrl Pts',(-2.01363949025797,7.65,-21.9122740947459));
#26450=CARTESIAN_POINT('Ctrl Pts',(-2.01363949025797,12.65,-21.9122740947459));
#26451=CARTESIAN_POINT('Ctrl Pts',(2.31648752866421,12.65,-19.4122740947459));
#26452=CARTESIAN_POINT('Ctrl Pts',(-2.21006130259559,7.65000000135137,-21.5720615360624));
#26453=CARTESIAN_POINT('Ctrl Pts',(-2.05862391632681,12.5223340542645,-21.8343587832484));
#26454=CARTESIAN_POINT('Ctrl Pts',(2.15894594111395,12.65,-19.3980111200692));
#26455=CARTESIAN_POINT('Ctrl Pts',(-2.40496369270797,7.68525114336172,-21.2344806938712));
#26456=CARTESIAN_POINT('Ctrl Pts',(-2.11744970702864,12.4006679911003,-21.7324695249547));
#26457=CARTESIAN_POINT('Ctrl Pts',(1.99474242287307,12.6532040193815,-19.3831385282814));
#26458=CARTESIAN_POINT('Ctrl Pts',(-2.5982622154322,7.75488674445212,-20.8996778314848));
#26459=CARTESIAN_POINT('Ctrl Pts',(-2.18962966210525,12.2921100651332,-21.6074501754737));
#26460=CARTESIAN_POINT('Ctrl Pts',(1.82293408768472,12.6595351585866,-19.3672161093864));
#26461=CARTESIAN_POINT('Origin',(2.31648752866421,7.65,-19.4122740947459));
#26462=CARTESIAN_POINT('Origin',(17.33160439086,7.65,-45.419219381653));
#26463=CARTESIAN_POINT('Ctrl Pts',(6.05397759465306,7.65,-35.8857967818224));
#26464=CARTESIAN_POINT('Ctrl Pts',(6.06352325746355,7.75665550347739,-35.9023303548021));
#26465=CARTESIAN_POINT('Ctrl Pts',(6.07620607043637,7.86490613592037,-35.9173823925603));
#26466=CARTESIAN_POINT('Ctrl Pts',(6.09220990698139,7.97437516838736,-35.930768869142));
#26467=CARTESIAN_POINT('Ctrl Pts',(6.10830824806606,8.08449062838374,-35.9442343944446));
#26468=CARTESIAN_POINT('Ctrl Pts',(6.12776706996586,8.19583869503638,-35.9560145143081));
#26469=CARTESIAN_POINT('Ctrl Pts',(6.15073683959036,8.30800050757065,-35.9659357817465));
#26470=CARTESIAN_POINT('Ctrl Pts',(6.17401344605895,8.4216606101247,-35.9759895803526));
#26471=CARTESIAN_POINT('Ctrl Pts',(6.20089557012674,8.53615607897855,-35.9841343953433));
#26472=CARTESIAN_POINT('Ctrl Pts',(6.23150016777579,8.65101843498515,-35.99020587159));
#26473=CARTESIAN_POINT('Ctrl Pts',(6.2623698206027,8.76687557166323,-35.9963299306622));
#26474=CARTESIAN_POINT('Ctrl Pts',(6.29702678978594,8.88310560424299,-36.0003444559528));
#26475=CARTESIAN_POINT('Ctrl Pts',(6.33554935823233,8.99919970639809,-36.002099080833));
#26476=CARTESIAN_POINT('Ctrl Pts',(6.37461073779734,9.11691760456602,-36.003878247467));
#26477=CARTESIAN_POINT('Ctrl Pts',(6.4176467041125,9.2344952982669,-36.0033337063284));
#26478=CARTESIAN_POINT('Ctrl Pts',(6.46469470269531,9.35137976204325,-36.0003295326902));
#26479=CARTESIAN_POINT('Ctrl Pts',(6.49326431830472,9.42235715324775,-35.9985052662251));
#26480=CARTESIAN_POINT('Ctrl Pts',(6.5233124876975,9.49307850835805,-35.9957744359036));
#26481=CARTESIAN_POINT('Ctrl Pts',(6.55483963837352,9.56341716182477,-35.9921106142424));
#26482=CARTESIAN_POINT('Ctrl Pts',(6.60548566774611,9.67641099200345,-35.9862249564685));
#26483=CARTESIAN_POINT('Ctrl Pts',(6.65994309733461,9.78839632357693,-35.9779303378726));
#26484=CARTESIAN_POINT('Ctrl Pts',(6.71807963141314,9.8988893637445,-35.9672031436682));
#26485=CARTESIAN_POINT('Ctrl Pts',(6.77958949265622,10.0157936766134,-35.9558535123649));
#26486=CARTESIAN_POINT('Ctrl Pts',(6.84521800543985,10.1310268984947,-35.9417805765281));
#26487=CARTESIAN_POINT('Ctrl Pts',(6.91475494575457,10.2440187011879,-35.924987827173));
#26488=CARTESIAN_POINT('Ctrl Pts',(6.98227077550315,10.3537263656191,-35.9086831637618));
#26489=CARTESIAN_POINT('Ctrl Pts',(7.05347059423811,10.4613204844058,-35.8898146968345));
#26490=CARTESIAN_POINT('Ctrl Pts',(7.12811667144977,10.5662898659827,-35.868414021319));
#26491=CARTESIAN_POINT('Ctrl Pts',(7.20611458428136,10.675972691659,-35.8460523904638));
#26492=CARTESIAN_POINT('Ctrl Pts',(7.28787514481669,10.782788948211,-35.8209258990637));
#26493=CARTESIAN_POINT('Ctrl Pts',(7.37308073487587,10.8861779564399,-35.7931020365515));
#26494=CARTESIAN_POINT('Ctrl Pts',(7.45828632493505,10.9895669646689,-35.7652781740394));
#26495=CARTESIAN_POINT('Ctrl Pts',(7.54693650290271,11.089528019321,-35.7347570496121));
#26496=CARTESIAN_POINT('Ctrl Pts',(7.63867256219547,11.1855339059315,-35.7016367919725));
#26497=CARTESIAN_POINT('Ctrl Pts',(7.72657542381271,11.2775281798324,-35.6699004666227));
#26498=CARTESIAN_POINT('Ctrl Pts',(7.81729722444394,11.36587628634,-35.6357829950195));
#26499=CARTESIAN_POINT('Ctrl Pts',(7.91040854597715,11.4502607243425,-35.59946667711));
#26500=CARTESIAN_POINT('Ctrl Pts',(8.00553850608124,11.5364746034756,-35.5623630272319));
#26501=CARTESIAN_POINT('Ctrl Pts',(8.10316223285138,11.6185505432383,-35.5229643244569));
#26502=CARTESIAN_POINT('Ctrl Pts',(8.20279923200259,11.6961959778101,-35.481487511482));
#26503=CARTESIAN_POINT('Ctrl Pts',(8.29945318522683,11.7715167749547,-35.4412524785593));
#26504=CARTESIAN_POINT('Ctrl Pts',(8.39800107480301,11.8426682994014,-35.3990622286071));
#26505=CARTESIAN_POINT('Ctrl Pts',(8.49799155856711,11.9094303708404,-35.3551318347922));
#26506=CARTESIAN_POINT('Ctrl Pts',(8.59704122042354,11.9755642703069,-35.3116147870814));
#26507=CARTESIAN_POINT('Ctrl Pts',(8.6975059751535,12.0373907339791,-35.2663904256432));
#26508=CARTESIAN_POINT('Ctrl Pts',(8.79894221884899,12.094744772372,-35.219680763423));
#26509=CARTESIAN_POINT('Ctrl Pts',(8.89886011845857,12.1512403092884,-35.173670272789));
#26510=CARTESIAN_POINT('Ctrl Pts',(8.99972021909567,12.2033962128042,-35.1262188376971));
#26511=CARTESIAN_POINT('Ctrl Pts',(9.10110045647905,12.2511046771425,-35.0775478545584));
#26512=CARTESIAN_POINT('Ctrl Pts',(9.11421610266949,12.2572767611176,-35.0712512487201));
#26513=CARTESIAN_POINT('Ctrl Pts',(9.12734046197172,12.2633744796128,-35.0649342416672));
#26514=CARTESIAN_POINT('Ctrl Pts',(9.14047262843647,12.269397662556,-35.0585973212973));
#26515=CARTESIAN_POINT('Ctrl Pts',(9.24363829396122,12.3167154968663,-35.0088147809147));
#26516=CARTESIAN_POINT('Ctrl Pts',(9.34726516304563,12.3594653682624,-34.9578218063693));
#26517=CARTESIAN_POINT('Ctrl Pts',(9.45089273271786,12.3976812193462,-34.9058912848161));
#26518=CARTESIAN_POINT('Ctrl Pts',(9.55303426965624,12.4353490501894,-34.8547054536494));
#26519=CARTESIAN_POINT('Ctrl Pts',(9.65517611959362,12.4686120581676,-34.8026090032369));
#26520=CARTESIAN_POINT('Ctrl Pts',(9.75689503342851,12.4975498540545,-34.7498627514153));
#26521=CARTESIAN_POINT('Ctrl Pts',(9.83095240164393,12.5186182760868,-34.7114603693422));
#26522=CARTESIAN_POINT('Ctrl Pts',(9.9047859351615,12.5373950091745,-34.67271354614));
#26523=CARTESIAN_POINT('Ctrl Pts',(9.97823993362958,12.5539264020161,-34.6337217553209));
#26524=CARTESIAN_POINT('Ctrl Pts',(10.0799380486854,12.576814352656,-34.5797370613403));
#26525=CARTESIAN_POINT('Ctrl Pts',(10.180905038132,12.595396582188,-34.5252845278614));
#26526=CARTESIAN_POINT('Ctrl Pts',(10.2807483971159,12.6098896651044,-34.4706355317292));
#26527=CARTESIAN_POINT('Ctrl Pts',(10.3796426825862,12.6242449822119,-34.4165060084523));
#26528=CARTESIAN_POINT('Ctrl Pts',(10.4774343677972,12.6345887162111,-34.3621839124303));
#26529=CARTESIAN_POINT('Ctrl Pts',(10.5737742299967,12.641169267053,-34.3079222096205));
#26530=CARTESIAN_POINT('Ctrl Pts',(10.6609849886114,12.6471262491154,-34.2588023109854));
#26531=CARTESIAN_POINT('Ctrl Pts',(10.7470063181385,12.65,-34.209731852514));
#26532=CARTESIAN_POINT('Ctrl Pts',(10.83160439086,12.65,-34.1608891324553));
#26533=CARTESIAN_POINT('Ctrl Pts',(6.05397759465306,7.65,-35.8857967818224));
#26534=CARTESIAN_POINT('Ctrl Pts',(6.05397759465306,7.65,-35.8857967818224));
#26535=CARTESIAN_POINT('Ctrl Pts',(6.05397759465306,7.65,-35.8857967818224));
#26536=CARTESIAN_POINT('Ctrl Pts',(6.11256573845244,8.30461645762939,-35.9872744236041));
#26537=CARTESIAN_POINT('Ctrl Pts',(6.18568737744441,8.23864736688774,-36.1139248174709));
#26538=CARTESIAN_POINT('Ctrl Pts',(6.25900485142217,8.17355351675001,-36.240914407483));
#26539=CARTESIAN_POINT('Ctrl Pts',(6.2838113402416,8.9587394433133,-36.0236072553336));
#26540=CARTESIAN_POINT('Ctrl Pts',(6.4083797352317,8.83304537535228,-36.2924955578147));
#26541=CARTESIAN_POINT('Ctrl Pts',(6.57657917544434,8.69671236121524,-36.5306960207266));
#26542=CARTESIAN_POINT('Ctrl Pts',(6.82586793650413,10.1680948803376,-35.9606139731479));
#26543=CARTESIAN_POINT('Ctrl Pts',(7.02469852379275,9.96758997398064,-36.522914965901));
#26544=CARTESIAN_POINT('Ctrl Pts',(7.38917119042457,9.6639387189906,-36.9362838290071));
#26545=CARTESIAN_POINT('Ctrl Pts',(7.19645515023948,10.7227336174027,-35.8612943435307));
#26546=CARTESIAN_POINT('Ctrl Pts',(7.42549815621051,10.5146815062461,-36.5742108314027));
#26547=CARTESIAN_POINT('Ctrl Pts',(7.88383228548133,10.1075313875409,-37.0518664657295));
#26548=CARTESIAN_POINT('Ctrl Pts',(8.08088997414811,11.6483341944628,-35.5419792404035));
#26549=CARTESIAN_POINT('Ctrl Pts',(8.39184058382502,11.4817645043902,-36.5160118602147));
#26550=CARTESIAN_POINT('Ctrl Pts',(8.97532595413734,10.8478143907806,-37.0911878018637));
#26551=CARTESIAN_POINT('Ctrl Pts',(8.59438969571741,12.0189319519102,-35.3221093677828));
#26552=CARTESIAN_POINT('Ctrl Pts',(8.96249719550974,11.89838707943,-36.4018237591869));
#26553=CARTESIAN_POINT('Ctrl Pts',(9.57172919308274,11.1442135371052,-37.0149110334635));
#26554=CARTESIAN_POINT('Ctrl Pts',(9.41351409479233,12.3946305178796,-34.926841298045));
#26555=CARTESIAN_POINT('Ctrl Pts',(9.88970755753321,12.3384327759138,-36.0938826425933));
#26556=CARTESIAN_POINT('Ctrl Pts',(10.4748981713972,11.444692242091,-36.7652124450691));
#26557=CARTESIAN_POINT('Ctrl Pts',(9.69456540456372,12.4900832460695,-34.7843054965499));
#26558=CARTESIAN_POINT('Ctrl Pts',(10.2112056628904,12.4537748504033,-35.96786613135));
#26559=CARTESIAN_POINT('Ctrl Pts',(10.7773024622675,11.5210340617089,-36.6596610917303));
#26560=CARTESIAN_POINT('Ctrl Pts',(10.2619144626914,12.6177695579628,-34.4831380140834));
#26561=CARTESIAN_POINT('Ctrl Pts',(10.8598325063373,12.6099538847863,-35.6740833652685));
#26562=CARTESIAN_POINT('Ctrl Pts',(11.3732152236663,11.6231558718973,-36.4079673945819));
#26563=CARTESIAN_POINT('Ctrl Pts',(10.5481950339283,12.65,-34.3245156009683));
#26564=CARTESIAN_POINT('Ctrl Pts',(11.1853523980411,12.6499999999596,-35.5068373265266));
#26565=CARTESIAN_POINT('Ctrl Pts',(11.6667058142795,11.6489333498051,-36.2618331013498));
#26566=CARTESIAN_POINT('Ctrl Pts',(10.83160439086,12.65,-34.1608891324553));
#26567=CARTESIAN_POINT('Ctrl Pts',(11.5028540567871,12.65,-35.3235276584047));
#26568=CARTESIAN_POINT('Ctrl Pts',(11.9501151712097,11.6489333498058,-36.0982066328345));
#26569=CARTESIAN_POINT('Origin',(17.33160439086,-7.90000000000001,-45.419219381653));
#26570=CARTESIAN_POINT('Origin',(17.3316043908594,-7.90000000000001,45.4192193816532));
#26571=CARTESIAN_POINT('Ctrl Pts',(6.05397759465256,7.65,35.8857967818225));
#26572=CARTESIAN_POINT('Ctrl Pts',(6.05397759465256,7.65,35.8857967818225));
#26573=CARTESIAN_POINT('Ctrl Pts',(6.05397759465256,7.65,35.8857967818225));
#26574=CARTESIAN_POINT('Ctrl Pts',(6.25900485142175,8.17355351675083,36.2409144074832));
#26575=CARTESIAN_POINT('Ctrl Pts',(6.18568737744254,8.23864736688944,36.1139248174686));
#26576=CARTESIAN_POINT('Ctrl Pts',(6.11256573845197,8.30461645762935,35.9872744236042));
#26577=CARTESIAN_POINT('Ctrl Pts',(6.57657917544341,8.69671236121402,36.5306960207267));
#26578=CARTESIAN_POINT('Ctrl Pts',(6.40837973523168,8.83304537535155,36.2924955578148));
#26579=CARTESIAN_POINT('Ctrl Pts',(6.28381134024114,8.95873944331333,36.0236072553337));
#26580=CARTESIAN_POINT('Ctrl Pts',(7.38917119042446,9.66393871899181,36.9362838290071));
#26581=CARTESIAN_POINT('Ctrl Pts',(7.02469852379175,9.96758997398138,36.5229149659011));
#26582=CARTESIAN_POINT('Ctrl Pts',(6.82586793650358,10.1680948803376,35.9606139731479));
#26583=CARTESIAN_POINT('Ctrl Pts',(7.88383228548062,10.10753138754,37.0518664657301));
#26584=CARTESIAN_POINT('Ctrl Pts',(7.42549815620927,10.5146815062463,36.5742108314018));
#26585=CARTESIAN_POINT('Ctrl Pts',(7.19645515023883,10.7227336174031,35.8612943435298));
#26586=CARTESIAN_POINT('Ctrl Pts',(8.97532595413702,10.8478143907815,37.0911878018634));
#26587=CARTESIAN_POINT('Ctrl Pts',(8.3918405838252,11.48176450439,36.5160118602157));
#26588=CARTESIAN_POINT('Ctrl Pts',(8.08088997414776,11.6483341944624,35.5419792404046));
#26589=CARTESIAN_POINT('Ctrl Pts',(9.571729193082,11.1442135371058,37.0149110334632));
#26590=CARTESIAN_POINT('Ctrl Pts',(8.96249719550926,11.89838707943,36.4018237591861));
#26591=CARTESIAN_POINT('Ctrl Pts',(8.59438969571705,12.0189319519102,35.3221093677829));
#26592=CARTESIAN_POINT('Ctrl Pts',(10.4748981713968,11.4446922420907,36.7652124450694));
#26593=CARTESIAN_POINT('Ctrl Pts',(9.88970755753271,12.3384327759138,36.0938826425938));
#26594=CARTESIAN_POINT('Ctrl Pts',(9.41351409479177,12.3946305178795,34.9268412980451));
#26595=CARTESIAN_POINT('Ctrl Pts',(10.7773024622668,11.5210340617088,36.6596610917307));
#26596=CARTESIAN_POINT('Ctrl Pts',(10.2112056628899,12.4537748504033,35.9678661313506));
#26597=CARTESIAN_POINT('Ctrl Pts',(9.69456540456328,12.4900832460695,34.78430549655));
#26598=CARTESIAN_POINT('Ctrl Pts',(11.373215223666,11.6231558718975,36.4079673945819));
#26599=CARTESIAN_POINT('Ctrl Pts',(10.8598325063368,12.6099538847863,35.6740833652681));
#26600=CARTESIAN_POINT('Ctrl Pts',(10.2619144626909,12.6177695579628,34.4831380140835));
#26601=CARTESIAN_POINT('Ctrl Pts',(11.6667058142791,11.6489333498044,36.2618331013506));
#26602=CARTESIAN_POINT('Ctrl Pts',(11.1853523980417,12.6499999999595,35.5068373265291));
#26603=CARTESIAN_POINT('Ctrl Pts',(10.5481950339276,12.65,34.3245156009679));
#26604=CARTESIAN_POINT('Ctrl Pts',(11.9501151712092,11.6489333498058,36.0982066328347));
#26605=CARTESIAN_POINT('Ctrl Pts',(11.5028540567866,12.65,35.3235276584049));
#26606=CARTESIAN_POINT('Ctrl Pts',(10.8316043908595,12.65,34.1608891324555));
#26607=CARTESIAN_POINT('Ctrl Pts',(6.05397759465256,7.65,35.8857967818225));
#26608=CARTESIAN_POINT('Ctrl Pts',(6.06352325746305,7.75665550347733,35.9023303548022));
#26609=CARTESIAN_POINT('Ctrl Pts',(6.07620607043586,7.86490613592026,35.9173823925604));
#26610=CARTESIAN_POINT('Ctrl Pts',(6.09220990698088,7.9743751683872,35.9307688691421));
#26611=CARTESIAN_POINT('Ctrl Pts',(6.10830824806559,8.08449062838383,35.9442343944447));
#26612=CARTESIAN_POINT('Ctrl Pts',(6.12776706996545,8.19583869503674,35.9560145143083));
#26613=CARTESIAN_POINT('Ctrl Pts',(6.15073683959002,8.30800050757127,35.9659357817467));
#26614=CARTESIAN_POINT('Ctrl Pts',(6.17401344605865,8.42166061012539,35.9759895803528));
#26615=CARTESIAN_POINT('Ctrl Pts',(6.20089557012648,8.53615607897931,35.9841343953435));
#26616=CARTESIAN_POINT('Ctrl Pts',(6.23150016777558,8.65101843498598,35.9902058715903));
#26617=CARTESIAN_POINT('Ctrl Pts',(6.26236982060258,8.7668755716643,35.9963299306624));
#26618=CARTESIAN_POINT('Ctrl Pts',(6.29702678978593,8.88310560424431,36.0003444559531));
#26619=CARTESIAN_POINT('Ctrl Pts',(6.33554935823244,8.99919970639965,36.0020990808332));
#26620=CARTESIAN_POINT('Ctrl Pts',(6.37461073779751,9.11691760456761,36.0038782474673));
#26621=CARTESIAN_POINT('Ctrl Pts',(6.41764670411273,9.23449529826853,36.0033337063286));
#26622=CARTESIAN_POINT('Ctrl Pts',(6.46469470269562,9.35137976204491,36.0003295326905));
#26623=CARTESIAN_POINT('Ctrl Pts',(6.49326431830481,9.42235715324882,35.9985052662254));
#26624=CARTESIAN_POINT('Ctrl Pts',(6.52331248769736,9.49307850835852,35.9957744359039));
#26625=CARTESIAN_POINT('Ctrl Pts',(6.55483963837312,9.56341716182466,35.9921106142428));
#26626=CARTESIAN_POINT('Ctrl Pts',(6.6054856677456,9.67641099200306,35.9862249564689));
#26627=CARTESIAN_POINT('Ctrl Pts',(6.65994309733397,9.78839632357628,35.9779303378731));
#26628=CARTESIAN_POINT('Ctrl Pts',(6.71807963141235,9.8988893637436,35.9672031436686));
#26629=CARTESIAN_POINT('Ctrl Pts',(6.77958949265545,10.0157936766126,35.9558535123653));
#26630=CARTESIAN_POINT('Ctrl Pts',(6.84521800543911,10.1310268984939,35.9417805765286));
#26631=CARTESIAN_POINT('Ctrl Pts',(6.91475494575386,10.2440187011872,35.9249878271734));
#26632=CARTESIAN_POINT('Ctrl Pts',(6.98227077550244,10.3537263656185,35.9086831637623));
#26633=CARTESIAN_POINT('Ctrl Pts',(7.0534705942374,10.4613204844052,35.889814696835));
#26634=CARTESIAN_POINT('Ctrl Pts',(7.12811667144906,10.5662898659821,35.8684140213195));
#26635=CARTESIAN_POINT('Ctrl Pts',(7.20611458428071,10.6759726916585,35.8460523904643));
#26636=CARTESIAN_POINT('Ctrl Pts',(7.28787514481612,10.7827889482106,35.8209258990643));
#26637=CARTESIAN_POINT('Ctrl Pts',(7.3730807348754,10.8861779564396,35.7931020365523));
#26638=CARTESIAN_POINT('Ctrl Pts',(7.45828632493467,10.9895669646686,35.7652781740402));
#26639=CARTESIAN_POINT('Ctrl Pts',(7.54693650290243,11.0895280193208,35.7347570496131));
#26640=CARTESIAN_POINT('Ctrl Pts',(7.63867256219533,11.1855339059313,35.7016367919737));
#26641=CARTESIAN_POINT('Ctrl Pts',(7.72657542381267,11.2775281798321,35.6699004666241));
#26642=CARTESIAN_POINT('Ctrl Pts',(7.817297224444,11.3658762863397,35.6357829950211));
#26643=CARTESIAN_POINT('Ctrl Pts',(7.91040854597731,11.4502607243423,35.5994666771117));
#26644=CARTESIAN_POINT('Ctrl Pts',(8.00553850608143,11.5364746034753,35.5623630272337));
#26645=CARTESIAN_POINT('Ctrl Pts',(8.10316223285158,11.6185505432381,35.5229643244588));
#26646=CARTESIAN_POINT('Ctrl Pts',(8.20279923200281,11.6961959778098,35.481487511484));
#26647=CARTESIAN_POINT('Ctrl Pts',(8.29945318522714,11.7715167749545,35.4412524785613));
#26648=CARTESIAN_POINT('Ctrl Pts',(8.39800107480342,11.8426682994013,35.399062228609));
#26649=CARTESIAN_POINT('Ctrl Pts',(8.49799155856761,11.9094303708404,35.355131834794));
#26650=CARTESIAN_POINT('Ctrl Pts',(8.59704122042377,11.9755642703067,35.3116147870833));
#26651=CARTESIAN_POINT('Ctrl Pts',(8.69750597515344,12.0373907339787,35.2663904256451));
#26652=CARTESIAN_POINT('Ctrl Pts',(8.79894221884864,12.0947447723716,35.2196807634251));
#26653=CARTESIAN_POINT('Ctrl Pts',(8.8988601184582,12.151240309288,35.173670272791));
#26654=CARTESIAN_POINT('Ctrl Pts',(8.99972021909529,12.2033962128038,35.1262188376991));
#26655=CARTESIAN_POINT('Ctrl Pts',(9.10110045647863,12.2511046771421,35.0775478545603));
#26656=CARTESIAN_POINT('Ctrl Pts',(9.11421610266926,12.2572767611173,35.071251248722));
#26657=CARTESIAN_POINT('Ctrl Pts',(9.12734046197164,12.2633744796126,35.064934241669));
#26658=CARTESIAN_POINT('Ctrl Pts',(9.14047262843657,12.2693976625559,35.0585973212989));
#26659=CARTESIAN_POINT('Ctrl Pts',(9.24363829396072,12.316715496866,35.0088147809166));
#26660=CARTESIAN_POINT('Ctrl Pts',(9.34726516304456,12.3594653682618,34.9578218063714));
#26661=CARTESIAN_POINT('Ctrl Pts',(9.45089273271621,12.3976812193455,34.9058912848185));
#26662=CARTESIAN_POINT('Ctrl Pts',(9.55303426965392,12.4353490501885,34.8547054536521));
#26663=CARTESIAN_POINT('Ctrl Pts',(9.65517611959064,12.4686120581666,34.80260900324));
#26664=CARTESIAN_POINT('Ctrl Pts',(9.75689503342485,12.4975498540534,34.7498627514186));
#26665=CARTESIAN_POINT('Ctrl Pts',(9.83095240164152,12.5186182760862,34.7114603693449));
#26666=CARTESIAN_POINT('Ctrl Pts',(9.90478593516031,12.5373950091742,34.6727135461419));
#26667=CARTESIAN_POINT('Ctrl Pts',(9.97823993362961,12.5539264020161,34.6337217553221));
#26668=CARTESIAN_POINT('Ctrl Pts',(10.0799380486856,12.576814352656,34.5797370613413));
#26669=CARTESIAN_POINT('Ctrl Pts',(10.1809050381322,12.595396582188,34.5252845278622));
#26670=CARTESIAN_POINT('Ctrl Pts',(10.2807483971162,12.6098896651045,34.4706355317297));
#26671=CARTESIAN_POINT('Ctrl Pts',(10.3796426825865,12.6242449822119,34.4165060084527));
#26672=CARTESIAN_POINT('Ctrl Pts',(10.4774343677974,12.6345887162112,34.3621839124305));
#26673=CARTESIAN_POINT('Ctrl Pts',(10.5737742299969,12.641169267053,34.3079222096205));
#26674=CARTESIAN_POINT('Ctrl Pts',(10.6609849886113,12.6471262491154,34.2588023109854));
#26675=CARTESIAN_POINT('Ctrl Pts',(10.7470063181382,12.65,34.209731852514));
#26676=CARTESIAN_POINT('Ctrl Pts',(10.8316043908595,12.65,34.1608891324555));
#26677=CARTESIAN_POINT('Origin',(10.8316043908595,7.65,34.1608891324555));
#26678=CARTESIAN_POINT('Origin',(2.31648752866394,7.65,19.4122740947459));
#26679=CARTESIAN_POINT('Ctrl Pts',(2.31648752866395,12.65,19.4122740947459));
#26680=CARTESIAN_POINT('Ctrl Pts',(-2.01363949025827,12.65,21.9122740947459));
#26681=CARTESIAN_POINT('Ctrl Pts',(-2.01363949025827,7.65,21.9122740947459));
#26682=CARTESIAN_POINT('Ctrl Pts',(2.158945941114,12.65,19.398011120066));
#26683=CARTESIAN_POINT('Ctrl Pts',(-2.05862391633069,12.5223340542653,21.8343587832445));
#26684=CARTESIAN_POINT('Ctrl Pts',(-2.21006130259589,7.65000000135137,21.5720615360624));
#26685=CARTESIAN_POINT('Ctrl Pts',(1.99474242287254,12.653204019381,19.3831385282839));
#26686=CARTESIAN_POINT('Ctrl Pts',(-2.1174497070286,12.4006679911032,21.732469524956));
#26687=CARTESIAN_POINT('Ctrl Pts',(-2.40496369270825,7.68525114336183,21.2344806938712));
#26688=CARTESIAN_POINT('Ctrl Pts',(1.82293408768446,12.6595351585866,19.3672161093864));
#26689=CARTESIAN_POINT('Ctrl Pts',(-2.18962966210555,12.2921100651332,21.6074501754736));
#26690=CARTESIAN_POINT('Ctrl Pts',(-2.59826221543248,7.75488674445211,20.8996778314848));
#26691=CARTESIAN_POINT('Origin',(1.73186480348973,7.75488674445211,18.3996778314848));
#26692=CARTESIAN_POINT('Ctrl Pts',(1.82293408768446,12.6595351585866,19.3672161093864));
#26693=CARTESIAN_POINT('Ctrl Pts',(-2.18962966210555,12.2921100651332,21.6074501754736));
#26694=CARTESIAN_POINT('Ctrl Pts',(-2.59826221543248,7.75488674445211,20.8996778314848));
#26695=CARTESIAN_POINT('Ctrl Pts',(1.63885776870729,12.666318372986,19.3501567500646));
#26696=CARTESIAN_POINT('Ctrl Pts',(-2.15856705477721,12.1520935820205,21.6023737557688));
#26697=CARTESIAN_POINT('Ctrl Pts',(-2.71413769515256,7.82950008896478,20.6989756132582));
#26698=CARTESIAN_POINT('Ctrl Pts',(1.43007155004091,12.6763099143986,19.3352963986434));
#26699=CARTESIAN_POINT('Ctrl Pts',(-2.14786497084269,12.0132183330853,21.5377143077062));
#26700=CARTESIAN_POINT('Ctrl Pts',(-2.83650075163869,7.93940906195218,20.5121824209172));
#26701=CARTESIAN_POINT('Ctrl Pts',(0.963339160700537,12.7012381622111,19.30453683087));
#26702=CARTESIAN_POINT('Ctrl Pts',(-2.19297758782216,11.7832074074835,21.3189597524121));
#26703=CARTESIAN_POINT('Ctrl Pts',(-3.09238573762713,8.21361978075487,20.1608140239618));
#26704=CARTESIAN_POINT('Ctrl Pts',(0.705363484677257,12.7161912440272,19.288651778162));
#26705=CARTESIAN_POINT('Ctrl Pts',(-2.24613629826497,11.6912659624442,21.1690685793912));
#26706=CARTESIAN_POINT('Ctrl Pts',(-3.22591261316364,8.37810368845214,19.9963051847538));
#26707=CARTESIAN_POINT('Ctrl Pts',(0.140400190055169,12.7502046526726,19.2497063845938));
#26708=CARTESIAN_POINT('Ctrl Pts',(-2.42082465748723,11.5747870675349,20.8220625359603));
#26709=CARTESIAN_POINT('Ctrl Pts',(-3.50309246541194,8.752251175245,19.6864071512402));
#26710=CARTESIAN_POINT('Ctrl Pts',(-0.165902550976841,12.7692327202596,
19.2265953913871));
#26711=CARTESIAN_POINT('Ctrl Pts',(-2.53989492939034,11.5484270002409,20.6273404315831));
#26712=CARTESIAN_POINT('Ctrl Pts',(-3.64629128691028,8.96155992656158,19.5417641964904));
#26713=CARTESIAN_POINT('Ctrl Pts',(-0.806001813909957,12.8095022395594,
19.1684463542416));
#26714=CARTESIAN_POINT('Ctrl Pts',(-2.82783067410163,11.5605687167961,20.2354968998797));
#26715=CARTESIAN_POINT('Ctrl Pts',(-3.93377998354566,9.40452463144772,19.2763433096647));
#26716=CARTESIAN_POINT('Ctrl Pts',(-1.14199205761375,12.8308799157878,19.1332633001334));
#26717=CARTESIAN_POINT('Ctrl Pts',(-2.99594386527674,11.5962530038109,20.0365408492835));
#26718=CARTESIAN_POINT('Ctrl Pts',(-4.07916420286535,9.63967907679387,19.154337615297));
#26719=CARTESIAN_POINT('Ctrl Pts',(-1.84114015329749,12.8755415399104,19.0455933955465));
#26720=CARTESIAN_POINT('Ctrl Pts',(-3.37066091328056,11.7180448914426,19.6515306856625));
#26721=CARTESIAN_POINT('Ctrl Pts',(-4.37345844384653,10.130956935887,18.9279994114957));
#26722=CARTESIAN_POINT('Ctrl Pts',(-2.20430287120771,12.8988286442761,18.9930962044593));
#26723=CARTESIAN_POINT('Ctrl Pts',(-3.57709720780661,11.8029800287245,19.4640891732687));
#26724=CARTESIAN_POINT('Ctrl Pts',(-4.52236818283683,10.3871150892957,18.8236885760162));
#26725=CARTESIAN_POINT('Ctrl Pts',(-2.95205920179125,12.9468769497921,18.8665254363902));
#26726=CARTESIAN_POINT('Ctrl Pts',(-4.01923841720749,12.0098985669601,19.1115051973322));
#26727=CARTESIAN_POINT('Ctrl Pts',(-4.82424696791924,10.9156464454547,18.630388670795));
#26728=CARTESIAN_POINT('Ctrl Pts',(-3.33661790917173,12.9716383743556,18.7923691610298));
#26729=CARTESIAN_POINT('Ctrl Pts',(-4.2557208557653,12.1317581217325,18.9448703376736));
#26730=CARTESIAN_POINT('Ctrl Pts',(-4.97719956846094,11.1880221188625,18.5414763577422));
#26731=CARTESIAN_POINT('Ctrl Pts',(-4.49972223032189,13.0467768755487,18.5361288699168));
#26732=CARTESIAN_POINT('Ctrl Pts',(-4.98545023588316,12.5265039443217,18.4937409410444));
#26733=CARTESIAN_POINT('Ctrl Pts',(-5.43846005488829,12.0145456291375,18.2977545914973));
#26734=CARTESIAN_POINT('Ctrl Pts',(-5.29194977390885,13.0982771986938,18.3187627795489));
#26735=CARTESIAN_POINT('Ctrl Pts',(-5.52173238862912,12.8398642052775,18.2414753432483));
#26736=CARTESIAN_POINT('Ctrl Pts',(-5.75087153299792,12.5811750651829,18.1644043383511));
#26737=CARTESIAN_POINT('Ctrl Pts',(-6.07314264709777,13.15,18.0560083736135));
#26738=CARTESIAN_POINT('Ctrl Pts',(-6.07314264709777,13.15,18.0560083736135));
#26739=CARTESIAN_POINT('Ctrl Pts',(-6.07314264709777,13.15,18.0560083736135));
#26740=CARTESIAN_POINT('Ctrl Pts',(19.3987830406924,7.75488674445212,8.19967783148497));
#26741=CARTESIAN_POINT('Ctrl Pts',(19.8074155940193,12.2921100651332,8.90745017547383));
#26742=CARTESIAN_POINT('Ctrl Pts',(15.8610341074694,12.6595351585866,11.2623152840528));
#26743=CARTESIAN_POINT('Ctrl Pts',(19.2855266632425,7.82781362133611,8.00351203146055));
#26744=CARTESIAN_POINT('Ctrl Pts',(19.7879152801881,12.1550958708994,8.93129057874443));
#26745=CARTESIAN_POINT('Ctrl Pts',(15.9364179871942,12.6661532847409,11.0984582286157));
#26746=CARTESIAN_POINT('Ctrl Pts',(19.1823236395831,7.93905335192905,7.79982027051171));
#26747=CARTESIAN_POINT('Ctrl Pts',(19.7264316747511,12.0132242375897,8.90923757193522));
#26748=CARTESIAN_POINT('Ctrl Pts',(16.0296209501497,12.6762775771014,10.9065165940293));
#26749=CARTESIAN_POINT('Ctrl Pts',(19.0040016931701,8.21703647488254,7.39768013956664));
#26750=CARTESIAN_POINT('Ctrl Pts',(19.557182530546,11.7807433434263,8.75824658918266));
#26751=CARTESIAN_POINT('Ctrl Pts',(16.2390578042154,12.7015487707905,10.4814724604871));
#26752=CARTESIAN_POINT('Ctrl Pts',(18.9284689774622,8.3825852909746,7.19938553412737));
#26753=CARTESIAN_POINT('Ctrl Pts',(19.4533169997301,11.6893488147424,8.6356549012008));
#26754=CARTESIAN_POINT('Ctrl Pts',(16.3548377364231,12.7165986624452,10.2489932522172));
#26755=CARTESIAN_POINT('Ctrl Pts',(18.7997330838058,8.75509815651615,6.80675061892527));
#26756=CARTESIAN_POINT('Ctrl Pts',(19.2413293102956,11.5743897252593,8.31178222410246));
#26757=CARTESIAN_POINT('Ctrl Pts',(16.6023485239282,12.7504634691448,9.74267567033139));
#26758=CARTESIAN_POINT('Ctrl Pts',(18.746488538986,8.96258837046799,6.61206546391529));
#26759=CARTESIAN_POINT('Ctrl Pts',(19.1331742313435,11.5481648613881,8.11318039916058));
#26760=CARTESIAN_POINT('Ctrl Pts',(16.7343513793893,12.7693262151716,9.46825494383473));
#26761=CARTESIAN_POINT('Ctrl Pts',(18.6597959133881,9.40977222762574,6.22704833757024));
#26762=CARTESIAN_POINT('Ctrl Pts',(18.9362340785775,11.5609929861831,7.6634850426214));
#26763=CARTESIAN_POINT('Ctrl Pts',(17.0065026260195,12.809979293746,8.87930623328658));
#26764=CARTESIAN_POINT('Ctrl Pts',(18.6269092451068,9.6461467700861,6.03947028079449));
#26765=CARTESIAN_POINT('Ctrl Pts',(18.8478843674036,11.5974627760309,7.41694458211731));
#26766=CARTESIAN_POINT('Ctrl Pts',(17.1446085817907,12.831467887923,8.56912654441456));
#26767=CARTESIAN_POINT('Ctrl Pts',(18.5540682318161,10.3837101835148,5.48752128769627));
#26768=CARTESIAN_POINT('Ctrl Pts',(18.6326070027182,11.7789057456669,6.6515072612234));
#26769=CARTESIAN_POINT('Ctrl Pts',(17.5550848097915,12.8985191081256,7.59418606796978));
#26770=CARTESIAN_POINT('Ctrl Pts',(18.5395119579207,10.9130303131145,5.13382873159073));
#26771=CARTESIAN_POINT('Ctrl Pts',(18.5435272704706,11.9964940699733,6.08081604217292));
#26772=CARTESIAN_POINT('Ctrl Pts',(17.8232803225471,12.9466391191647,6.8843284908237));
#26773=CARTESIAN_POINT('Ctrl Pts',(18.5654641308157,12.0122001031253,4.4404896187003));
#26774=CARTESIAN_POINT('Ctrl Pts',(18.50877362979,12.5253529301349,4.9317460477106));
#26775=CARTESIAN_POINT('Ctrl Pts',(18.3016406778754,13.046563645948,5.37443005716869));
#26776=CARTESIAN_POINT('Ctrl Pts',(18.6064525652392,12.5827074287898,4.10090346837722));
#26777=CARTESIAN_POINT('Ctrl Pts',(18.5587510299058,12.8406828545658,4.33727184508721));
#26778=CARTESIAN_POINT('Ctrl Pts',(18.5109195335152,13.0984138348512,4.57428419864026));
#26779=CARTESIAN_POINT('Ctrl Pts',(18.6735332660427,13.15,3.76850837361377));
#26780=CARTESIAN_POINT('Ctrl Pts',(18.6735332660427,13.15,3.76850837361377));
#26781=CARTESIAN_POINT('Ctrl Pts',(18.6735332660427,13.15,3.76850837361377));
#26782=CARTESIAN_POINT('Origin',(15.0686560217701,7.75488674445212,10.6996778314849));
#26783=CARTESIAN_POINT('Ctrl Pts',(19.9834057658666,7.65,9.21227409474614));
#26784=CARTESIAN_POINT('Ctrl Pts',(19.9834057658666,12.65,9.21227409474612));
#26785=CARTESIAN_POINT('Ctrl Pts',(15.6532787469444,12.65,11.7122740947461));
#26786=CARTESIAN_POINT('Ctrl Pts',(19.786983953529,7.65000000135137,8.87206153606267));
#26787=CARTESIAN_POINT('Ctrl Pts',(19.9384213397991,12.5223340542634,9.13435878324342));
#26788=CARTESIAN_POINT('Ctrl Pts',(15.7196974423163,12.65,11.5687075904368));
#26789=CARTESIAN_POINT('Ctrl Pts',(19.5920815634165,7.68525114336148,8.53448069387126));
#26790=CARTESIAN_POINT('Ctrl Pts',(19.879595549097,12.4006679911059,9.03246952495355));
#26791=CARTESIAN_POINT('Ctrl Pts',(15.788919159126,12.6532040193819,11.4190668763545));
#26792=CARTESIAN_POINT('Ctrl Pts',(19.3987830406924,7.75488674445212,8.19967783148497));
#26793=CARTESIAN_POINT('Ctrl Pts',(19.8074155940193,12.2921100651331,8.90745017547383));
#26794=CARTESIAN_POINT('Ctrl Pts',(15.8610341074694,12.6595351585866,11.2623152840528));
#26795=CARTESIAN_POINT('Origin',(15.6532787469444,7.65,11.7122740947461));
#26796=CARTESIAN_POINT('Origin',(30.6683956091398,7.65,37.7192193816533));
#26797=CARTESIAN_POINT('Ctrl Pts',(28.0510228507774,7.65,23.1857967818227));
#26798=CARTESIAN_POINT('Ctrl Pts',(28.060568513588,7.7566555034772,23.2023303548025));
#26799=CARTESIAN_POINT('Ctrl Pts',(28.067262554179,7.86490613592002,23.2208400119076));
#26800=CARTESIAN_POINT('Ctrl Pts',(28.0708536646935,7.97437516838686,23.2413929792046));
#26801=CARTESIAN_POINT('Ctrl Pts',(28.0744659811386,8.08449062838318,23.2620673141941));
#26802=CARTESIAN_POINT('Ctrl Pts',(28.0749384532501,8.19583869503577,23.2848092082189));
#26803=CARTESIAN_POINT('Ctrl Pts',(28.0720456380773,8.30800050757001,23.3096622459521));
#26804=CARTESIAN_POINT('Ctrl Pts',(28.0691141798405,8.42166061012386,23.3348472777708));
#26805=CARTESIAN_POINT('Ctrl Pts',(28.0627267344978,8.53615607897753,23.3622002876166));
#26806=CARTESIAN_POINT('Ctrl Pts',(28.0526824883414,8.65101843498394,23.3917403847766));
#26807=CARTESIAN_POINT('Ctrl Pts',(28.0425512526588,8.76687557166174,23.4215363178668));
#26808=CARTESIAN_POINT('Ctrl Pts',(28.0286994489531,8.88310560424122,23.4535573962429));
#26809=CARTESIAN_POINT('Ctrl Pts',(28.0109577144504,8.99919970639603,23.4877962315765));
#26810=CARTESIAN_POINT('Ctrl Pts',(27.9929678281707,9.11691760456367,23.5225139619036));
#26811=CARTESIAN_POINT('Ctrl Pts',(27.9709782585537,9.23449529826427,23.5595119314396));
#26812=CARTESIAN_POINT('Ctrl Pts',(27.9448525685745,9.35137976204033,23.5987546065903));
#26813=CARTESIAN_POINT('Ctrl Pts',(27.9289878996676,9.42235715324562,23.6225844862522));
#26814=CARTESIAN_POINT('Ctrl Pts',(27.9115988465393,9.49307850835669,23.6472415491231));
#26815=CARTESIAN_POINT('Ctrl Pts',(27.8926623085676,9.56341716182418,23.6727129516872));
#26816=CARTESIAN_POINT('Ctrl Pts',(27.8622421647312,9.67641099200259,23.7136308708377));
#26817=CARTESIAN_POINT('Ctrl Pts',(27.8278300995184,9.78839632357584,23.7566450789882));
#26818=CARTESIAN_POINT('Ctrl Pts',(27.7894718097869,9.89888936374319,23.801629197286));
#26819=CARTESIAN_POINT('Ctrl Pts',(27.7488878101332,10.0157936766121,23.8492234840541));
#26820=CARTESIAN_POINT('Ctrl Pts',(27.703886033801,10.1310268984934,23.899022975419));
#26821=CARTESIAN_POINT('Ctrl Pts',(27.6545746161027,10.2440187011867,23.9508473575555));
#26822=CARTESIAN_POINT('Ctrl Pts',(27.6066964485145,10.3537263656175,24.0011654495696));
#26823=CARTESIAN_POINT('Ctrl Pts',(27.5547559674577,10.4613204844038,24.053392067875));
#26824=CARTESIAN_POINT('Ctrl Pts',(27.4988994001976,10.5662898659804,24.1073371292752));
#26825=CARTESIAN_POINT('Ctrl Pts',(27.440534703391,10.6759726916569,24.163704487802));
#26826=CARTESIAN_POINT('Ctrl Pts',(27.3778942432628,10.7827889482093,24.2219479645533));
#26827=CARTESIAN_POINT('Ctrl Pts',(27.3111952764661,10.8861779564386,24.2818262388331));
#26828=CARTESIAN_POINT('Ctrl Pts',(27.2444963096694,10.9895669646679,24.3417045131128));
#26829=CARTESIAN_POINT('Ctrl Pts',(27.1737391515792,11.0895280193203,24.4032172570693));
#26830=CARTESIAN_POINT('Ctrl Pts',(27.0991881374367,11.1855339059311,24.4661028860402));
#26831=CARTESIAN_POINT('Ctrl Pts',(27.0277522426528,11.2775281798315,24.5263608345907));
#26832=CARTESIAN_POINT('Ctrl Pts',(26.9528447452163,11.3658762863386,24.5878694828124));
#26833=CARTESIAN_POINT('Ctrl Pts',(26.8748382305686,11.4502607243407,24.6503480936848));
#26834=CARTESIAN_POINT('Ctrl Pts',(26.7951405471489,11.536474603474,24.7141812308569));
#26835=CARTESIAN_POINT('Ctrl Pts',(26.7122084062844,11.618550543237,24.7790265068645));
#26836=CARTESIAN_POINT('Ctrl Pts',(26.6264699330043,11.6961959778089,24.8445762727988));
#26837=CARTESIAN_POINT('Ctrl Pts',(26.5432983957594,11.7715167749532,24.9081635352054));
#26838=CARTESIAN_POINT('Ctrl Pts',(26.4574866227211,11.8426682993997,24.9724133860912));
#26839=CARTESIAN_POINT('Ctrl Pts',(26.3694465437975,11.9094303708384,25.0370424882597));
#26840=CARTESIAN_POINT('Ctrl Pts',(26.2822348440543,11.9755642703047,25.1010634878078));
#26841=CARTESIAN_POINT('Ctrl Pts',(26.1928370208142,12.0373907339768,25.1654563368694));
#26842=CARTESIAN_POINT('Ctrl Pts',(26.1016671448819,12.0947447723696,25.2299478696638));
#26843=CARTESIAN_POINT('Ctrl Pts',(26.0118619413472,12.1512403092862,25.2934740637014));
#26844=CARTESIAN_POINT('Ctrl Pts',(25.9203377427928,12.2033962128022,25.3570957555355));
#26845=CARTESIAN_POINT('Ctrl Pts',(25.8274973162755,12.2511046771407,25.4205581249819));
#26846=CARTESIAN_POINT('Ctrl Pts',(25.8154864725656,12.2572767611165,25.4287683048515));
#26847=CARTESIAN_POINT('Ctrl Pts',(25.8034536043297,12.2633744796122,25.4369758298899));
#26848=CARTESIAN_POINT('Ctrl Pts',(25.791399587074,12.269397662556,25.4451801594709));
#26849=CARTESIAN_POINT('Ctrl Pts',(25.6967038096742,12.3167154968669,25.509632976423));
#26850=CARTESIAN_POINT('Ctrl Pts',(25.60072916376,12.3594653682634,25.5738799902926));
#26851=CARTESIAN_POINT('Ctrl Pts',(25.5039422280259,12.3976812193475,25.6376588373852));
#26852=CARTESIAN_POINT('Ctrl Pts',(25.4085432294501,12.4353490501916,25.7005230875736));
#26853=CARTESIAN_POINT('Ctrl Pts',(25.3123554549748,12.4686120581704,25.7629322992041));
#26854=CARTESIAN_POINT('Ctrl Pts',(25.215816404023,12.4975498540577,25.8246503367211));
#26855=CARTESIAN_POINT('Ctrl Pts',(25.1455302814777,12.5186182760887,25.8695847078942));
#26856=CARTESIAN_POINT('Ctrl Pts',(25.0750577815132,12.5373950091753,25.9141530119682));
#26857=CARTESIAN_POINT('Ctrl Pts',(25.0045629008943,12.5539264020161,25.9582701452394));
#26858=CARTESIAN_POINT('Ctrl Pts',(24.9069617269622,12.5768143526563,26.0193509494053));
#26859=CARTESIAN_POINT('Ctrl Pts',(24.8093209549444,12.5953965821885,26.0795646604711));
#26860=CARTESIAN_POINT('Ctrl Pts',(24.7120718565095,12.6098896651051,26.1387070476852));
#26861=CARTESIAN_POINT('Ctrl Pts',(24.6157471715197,12.6242449822127,26.1972872495546));
#26862=CARTESIAN_POINT('Ctrl Pts',(24.5198070137702,12.634588716212,26.2548162852166));
#26863=CARTESIAN_POINT('Ctrl Pts',(24.4246450695825,12.6411692670537,26.3111182018749));
#26864=CARTESIAN_POINT('Ctrl Pts',(24.3385006102295,12.6471262491156,26.3620849849988));
#26865=CARTESIAN_POINT('Ctrl Pts',(24.252993681858,12.65,26.4120464123989));
#26866=CARTESIAN_POINT('Ctrl Pts',(24.1683956091399,12.65,26.4608891324556));
#26867=CARTESIAN_POINT('Ctrl Pts',(28.0510228507774,7.65,23.1857967818227));
#26868=CARTESIAN_POINT('Ctrl Pts',(28.0510228507774,7.65,23.1857967818227));
#26869=CARTESIAN_POINT('Ctrl Pts',(28.0510228507774,7.65,23.1857967818227));
#26870=CARTESIAN_POINT('Ctrl Pts',(28.1096109945774,8.30461645762897,23.2872744236054));
#26871=CARTESIAN_POINT('Ctrl Pts',(28.1827326335685,8.23864736688808,23.4139248174707));
#26872=CARTESIAN_POINT('Ctrl Pts',(28.256050107547,8.17355351675034,23.540914407484));
#26873=CARTESIAN_POINT('Ctrl Pts',(28.0554533489513,8.95873944331359,23.4537438809049));
#26874=CARTESIAN_POINT('Ctrl Pts',(28.2260332521862,8.83304537535202,23.6960674267152));
#26875=CARTESIAN_POINT('Ctrl Pts',(28.3482211841544,8.69671236121383,23.9608326462977));
#26876=CARTESIAN_POINT('Ctrl Pts',(27.7298712681797,10.1680948803373,23.8916820224643));
#26877=CARTESIAN_POINT('Ctrl Pts',(28.1174229188319,9.96758997398087,24.3450248584824));
#26878=CARTESIAN_POINT('Ctrl Pts',(28.2931745220997,9.66393871899201,24.8673518783236));
#26879=CARTESIAN_POINT('Ctrl Pts',(27.4585643389691,10.7227336174025,24.1629601490681));
#26880=CARTESIAN_POINT('Ctrl Pts',(27.9614466252574,10.5146815062456,24.7177754547336));
#26881=CARTESIAN_POINT('Ctrl Pts',(28.1459414742105,10.1075313875396,25.3535322712672));
#26882=CARTESIAN_POINT('Ctrl Pts',(26.7398119358942,11.648334194463,24.7692456230013));
#26883=CARTESIAN_POINT('Ctrl Pts',(27.427873623927,11.4817645043907,25.5255530602099));
#26884=CARTESIAN_POINT('Ctrl Pts',(27.634247915884,10.8478143907818,26.3184541844612));
#26885=CARTESIAN_POINT('Ctrl Pts',(26.2926491798939,12.0189319519099,25.1040144904058));
#26886=CARTESIAN_POINT('Ctrl Pts',(27.0436555217853,11.8983870794298,25.9626621322522));
#26887=CARTESIAN_POINT('Ctrl Pts',(27.2699886772591,11.1442135371051,26.7968161560863));
#26888=CARTESIAN_POINT('Ctrl Pts',(25.5407747906579,12.3946305178797,25.6157629939958));
#26889=CARTESIAN_POINT('Ctrl Pts',(26.313365510933,12.3384327759139,26.6116793021193));
#26890=CARTESIAN_POINT('Ctrl Pts',(26.6021588672628,11.4446922420911,27.4541341410199));
#26891=CARTESIAN_POINT('Ctrl Pts',(25.2768095107291,12.4900832460695,25.7878926672769));
#26892=CARTESIAN_POINT('Ctrl Pts',(26.0434829582219,12.4537748504032,26.8270965730057));
#26893=CARTESIAN_POINT('Ctrl Pts',(26.3595465684327,11.5210340617089,27.6632482624575));
#26894=CARTESIAN_POINT('Ctrl Pts',(24.732316291055,12.6177695579628,26.1286476231956));
#26895=CARTESIAN_POINT('Ctrl Pts',(25.4647461978773,12.6099538847864,27.2419325139665));
#26896=CARTESIAN_POINT('Ctrl Pts',(25.8436170520301,11.6231558718974,28.053477003694));
#26897=CARTESIAN_POINT('Ctrl Pts',(24.45180496607,12.65,26.2972626639395));
#26898=CARTESIAN_POINT('Ctrl Pts',(25.1571469337936,12.6499999999603,27.4402179902489));
#26899=CARTESIAN_POINT('Ctrl Pts',(25.5703157464209,11.6489333498045,28.2345801643211));
#26900=CARTESIAN_POINT('Ctrl Pts',(24.1683956091399,12.65,26.4608891324556));
#26901=CARTESIAN_POINT('Ctrl Pts',(24.8396452750671,12.65,27.623527658405));
#26902=CARTESIAN_POINT('Ctrl Pts',(25.2869063894896,11.6489333498058,28.3982066328348));
#26903=CARTESIAN_POINT('Ctrl Pts',(28.0510228507774,7.65,23.1857967818227));
#26904=CARTESIAN_POINT('Ctrl Pts',(28.0844275796731,7.73530164996095,23.243655469483));
#26905=CARTESIAN_POINT('Ctrl Pts',(28.1153375201379,7.82187906280546,23.3041082955208));
#26906=CARTESIAN_POINT('Ctrl Pts',(28.1434170892384,7.90943093574786,23.3670765172883));
#26907=CARTESIAN_POINT('Ctrl Pts',(28.1716624715014,7.99749981281107,23.4304165738212));
#26908=CARTESIAN_POINT('Ctrl Pts',(28.1970437461975,8.08655451224725,23.4963017794788));
#26909=CARTESIAN_POINT('Ctrl Pts',(28.2192417703173,8.1762600347923,23.5646134256722));
#26910=CARTESIAN_POINT('Ctrl Pts',(28.2417363220809,8.26716386972267,23.6338375986463));
#26911=CARTESIAN_POINT('Ctrl Pts',(28.2609617599807,8.35873581948415,23.7055534235978));
#26912=CARTESIAN_POINT('Ctrl Pts',(28.276612470514,8.45060120069979,23.7795984912439));
#26913=CARTESIAN_POINT('Ctrl Pts',(28.292398726102,8.54326219423563,23.8542848360207));
#26914=CARTESIAN_POINT('Ctrl Pts',(28.3045478312839,8.63622142494294,23.9313408096347));
#26915=CARTESIAN_POINT('Ctrl Pts',(28.3127765977397,8.72907194030857,24.0105618721281));
#26916=CARTESIAN_POINT('Ctrl Pts',(28.3211204590875,8.82322114607964,24.0908909913013));
#26917=CARTESIAN_POINT('Ctrl Pts',(28.3254332730565,8.91725821818692,24.1734460255698));
#26918=CARTESIAN_POINT('Ctrl Pts',(28.3254548896342,9.01074085424139,24.2579771641602));
#26919=CARTESIAN_POINT('Ctrl Pts',(28.3254680161717,9.06750762559021,24.3093081922392));
#26920=CARTESIAN_POINT('Ctrl Pts',(28.3238994826617,9.12406962268391,24.3613671988861));
#26921=CARTESIAN_POINT('Ctrl Pts',(28.3206978531259,9.18032554010459,24.4140922623076));
#26922=CARTESIAN_POINT('Ctrl Pts',(28.3155546727227,9.27069649927002,24.4987911663861));
#26923=CARTESIAN_POINT('Ctrl Pts',(28.3061939676307,9.36026087469428,24.5851956030652));
#26924=CARTESIAN_POINT('Ctrl Pts',(28.292553209215,9.44863173534435,24.6729917414403));
#26925=CARTESIAN_POINT('Ctrl Pts',(28.2781209564036,9.54213024643806,24.765882182446));
#26926=CARTESIAN_POINT('Ctrl Pts',(28.2588971002568,9.63429224123548,24.8603303412854));
#26927=CARTESIAN_POINT('Ctrl Pts',(28.234862192439,9.7246615788445,24.9559349227726));
#26928=CARTESIAN_POINT('Ctrl Pts',(28.2115258659209,9.81240430644903,25.0487607304318));
#26929=CARTESIAN_POINT('Ctrl Pts',(28.1836544212169,9.89845664842074,25.1426761425893));
#26930=CARTESIAN_POINT('Ctrl Pts',(28.1512797309364,9.98240976055992,25.2372930079755));
#26931=CARTESIAN_POINT('Ctrl Pts',(28.1174513187174,10.0701326224597,25.3361584580365));
#26932=CARTESIAN_POINT('Ctrl Pts',(28.078705885483,10.1555628405854,25.435789335416));
#26933=CARTESIAN_POINT('Ctrl Pts',(28.0351352627411,10.2382519911876,25.5357270766931));
#26934=CARTESIAN_POINT('Ctrl Pts',(27.9915646399991,10.3209411417899,25.6356648179701));
#26935=CARTESIAN_POINT('Ctrl Pts',(27.9431689853577,10.4008886608162,25.735908822033));
#26936=CARTESIAN_POINT('Ctrl Pts',(27.8900946950455,10.4776728891654,25.8359932278577));
#26937=CARTESIAN_POINT('Ctrl Pts',(27.839238117679,10.5512486831439,25.9318955997605));
#26938=CARTESIAN_POINT('Ctrl Pts',(27.7840942821528,10.6219083210448,26.0276359145545));
#26939=CARTESIAN_POINT('Ctrl Pts',(27.7249647482248,10.6893978697112,26.1228104151272));
#26940=CARTESIAN_POINT('Ctrl Pts',(27.6645532954503,10.7583505810078,26.2200482836633));
#26941=CARTESIAN_POINT('Ctrl Pts',(27.5999817192723,10.8239938235548,26.3166949905633));
#26942=CARTESIAN_POINT('Ctrl Pts',(27.531612697115,10.8860936071087,26.4123295283418));
#26943=CARTESIAN_POINT('Ctrl Pts',(27.4652905845881,10.9463341766357,26.5051008504386));
#26944=CARTESIAN_POINT('Ctrl Pts',(27.395395560976,11.0032402174354,26.5969193200223));
#26945=CARTESIAN_POINT('Ctrl Pts',(27.3222903013768,11.0566356322311,26.687416288063));
#26946=CARTESIAN_POINT('Ctrl Pts',(27.2498728975335,11.1095286434568,26.7770617597724));
#26947=CARTESIAN_POINT('Ctrl Pts',(27.1743057875189,11.1589766249525,26.865410106846));
#26948=CARTESIAN_POINT('Ctrl Pts',(27.0959661336344,11.2048476203275,26.9521242360999));
#26949=CARTESIAN_POINT('Ctrl Pts',(27.0187991035164,11.2500319976655,27.0375403886101));
#26950=CARTESIAN_POINT('Ctrl Pts',(26.9389422930304,11.2917455940572,27.1213705893704));
#26951=CARTESIAN_POINT('Ctrl Pts',(26.8567743528486,11.3299021878793,27.2033182473929));
#26952=CARTESIAN_POINT('Ctrl Pts',(26.8461442176319,11.3348385383688,27.2139198845222));
#26953=CARTESIAN_POINT('Ctrl Pts',(26.8354754221709,11.3397154123387,27.2244900529112));
#26954=CARTESIAN_POINT('Ctrl Pts',(26.8247688039266,11.3445326737677,27.2350281460368));
#26955=CARTESIAN_POINT('Ctrl Pts',(26.7406581280837,11.3823768469003,27.3178148966865));
#26956=CARTESIAN_POINT('Ctrl Pts',(26.6542467205738,11.4165676241853,27.3986259253548));
#26957=CARTESIAN_POINT('Ctrl Pts',(26.5660087531245,11.4471321524631,27.4772120198665));
#26958=CARTESIAN_POINT('Ctrl Pts',(26.4790361295247,11.4772583814579,27.5546711796332));
#26959=CARTESIAN_POINT('Ctrl Pts',(26.3902893616535,11.5038616918416,27.6299685927576));
#26960=CARTESIAN_POINT('Ctrl Pts',(26.3002237580355,11.5270057552498,27.702898969953));
#26961=CARTESIAN_POINT('Ctrl Pts',(26.2346506869213,11.5438559983479,27.7559965856699));
#26962=CARTESIAN_POINT('Ctrl Pts',(26.16837858263,11.5588733791764,27.8078401884681));
#26963=CARTESIAN_POINT('Ctrl Pts',(26.1015818102301,11.5720949668065,27.8583626330729));
#26964=CARTESIAN_POINT('Ctrl Pts',(26.009100720206,11.5904004446306,27.928311682703));
#26965=CARTESIAN_POINT('Ctrl Pts',(25.9156168330012,11.605262264108,27.9957253294626));
#26966=CARTESIAN_POINT('Ctrl Pts',(25.8216098684647,11.6168536386306,28.0604832573104));
#26967=CARTESIAN_POINT('Ctrl Pts',(25.7284964988654,11.6283348298957,28.1246256205907));
#26968=CARTESIAN_POINT('Ctrl Pts',(25.6348702567158,11.6366076104655,28.1861624756317));
#26969=CARTESIAN_POINT('Ctrl Pts',(25.5411803959419,11.6418706473094,28.2450141155512));
#26970=CARTESIAN_POINT('Ctrl Pts',(25.4563685263168,11.6466349621557,28.2982890117977));
#26971=CARTESIAN_POINT('Ctrl Pts',(25.371504462211,11.6489333498058,28.3493639127762));
#26972=CARTESIAN_POINT('Ctrl Pts',(25.2869063894896,11.6489333498058,28.3982066328348));
#26973=CARTESIAN_POINT('Origin',(30.6683956091398,-7.9,37.7192193816533));
#26974=CARTESIAN_POINT('Origin',(30.6683956091398,-7.9,37.7192193816533));
#26975=CARTESIAN_POINT('Origin',(30.6683956091398,-7.90000000000001,37.7192193816533));
#26976=CARTESIAN_POINT('Origin',(30.6683956091398,-7.90000000000001,37.7192193816533));
#26977=CARTESIAN_POINT('Origin',(30.6683956091398,-7.90000000000001,37.7192193816533));
#26978=CARTESIAN_POINT('Origin',(30.6683956091398,-21.9,37.7192193816533));
#26979=CARTESIAN_POINT('Ctrl Pts',(-15.5865359611318,-22.9,11.8009489759233));
#26980=CARTESIAN_POINT('Ctrl Pts',(-15.7517039698567,-22.9,12.7872144213759));
#26981=CARTESIAN_POINT('Ctrl Pts',(-15.7517039698567,-21.9,12.7872144213759));
#26982=CARTESIAN_POINT('Ctrl Pts',(-15.3559607473128,-22.9,11.9647821254064));
#26983=CARTESIAN_POINT('Ctrl Pts',(-15.5607856662629,-22.7827980547214,
12.8191871306933));
#26984=CARTESIAN_POINT('Ctrl Pts',(-15.4355591423194,-21.9000000281286,
12.8401585976865));
#26985=CARTESIAN_POINT('Ctrl Pts',(-15.1190374158585,-22.9205735494498,
12.1462781863217));
#26986=CARTESIAN_POINT('Ctrl Pts',(-15.2973142372118,-22.7172748074572,
12.8709905227205));
#26987=CARTESIAN_POINT('Ctrl Pts',(-15.1328683878844,-21.9617206530121,
12.915148108118));
#26988=CARTESIAN_POINT('Ctrl Pts',(-14.6271245805211,-22.9836857365403,
12.5399038917133));
#26989=CARTESIAN_POINT('Ctrl Pts',(-14.7359632242306,-22.6985884975707,
13.0355614944526));
#26990=CARTESIAN_POINT('Ctrl Pts',(-14.5466360368447,-22.151057204958,13.105466734237));
#26991=CARTESIAN_POINT('Ctrl Pts',(-14.3791131979057,-23.0257436937064,
12.7464145774642));
#26992=CARTESIAN_POINT('Ctrl Pts',(-14.4436326996405,-22.7356048512228,
13.1424140441331));
#26993=CARTESIAN_POINT('Ctrl Pts',(-14.2714100237779,-22.2772310832513,
13.2181656147264));
#26994=CARTESIAN_POINT('Ctrl Pts',(-13.6286677467523,-23.1675945141807,
13.383230113175));
#26995=CARTESIAN_POINT('Ctrl Pts',(-13.6265116615006,-22.9266590509653,
13.5179293418098));
#26996=CARTESIAN_POINT('Ctrl Pts',(-13.4894327977986,-22.7027835382778,
13.6005990193291));
#26997=CARTESIAN_POINT('Ctrl Pts',(-13.1126423384295,-23.2843988132411,
13.8357364471931));
#26998=CARTESIAN_POINT('Ctrl Pts',(-13.0648889625182,-23.1694382547404,
13.877850966168));
#26999=CARTESIAN_POINT('Ctrl Pts',(-13.0193938287046,-23.0534635976961,
13.9179739028129));
#27000=CARTESIAN_POINT('Ctrl Pts',(-12.6003906189451,-23.4,14.2875));
#27001=CARTESIAN_POINT('Ctrl Pts',(-12.6003906189451,-23.4,14.2875));
#27002=CARTESIAN_POINT('Ctrl Pts',(-12.6003906189451,-23.4,14.2875));
#27003=CARTESIAN_POINT('Origin',(-15.5865359611318,-21.9,11.8009489759233));
#27004=CARTESIAN_POINT('Origin',(-16.8005208252602,-21.9,19.05));
#27005=CARTESIAN_POINT('Origin',(-16.8005208252602,-21.9,11.7));
#27006=CARTESIAN_POINT('Origin',(-48.,-21.9,11.7));
#27007=CARTESIAN_POINT('Origin',(-48.,-21.9,11.7));
#27008=CARTESIAN_POINT('Origin',(-48.,-21.9,7.7));
#27009=CARTESIAN_POINT('Origin',(-52.,-21.9,7.7));
#27010=CARTESIAN_POINT('Origin',(-52.,-21.9,12.7));
#27011=CARTESIAN_POINT('Origin',(-52.,-21.9,-7.7));
#27012=CARTESIAN_POINT('Origin',(-48.,-21.9,-7.7));
#27013=CARTESIAN_POINT('Origin',(-48.,-21.9,-11.7));
#27014=CARTESIAN_POINT('Origin',(4.15723558123562E-15,-21.9,-11.7));
#27015=CARTESIAN_POINT('Origin',(-16.8005208252602,-21.9,-11.7));
#27016=CARTESIAN_POINT('Origin',(-16.8005208252602,-21.9,-19.05));
#27017=CARTESIAN_POINT('Origin',(-15.5865359611318,-21.9,-11.8009489759233));
#27018=CARTESIAN_POINT('Ctrl Pts',(-15.7517039698567,-21.9,-12.7872144213759));
#27019=CARTESIAN_POINT('Ctrl Pts',(-15.7517039698567,-22.9,-12.7872144213759));
#27020=CARTESIAN_POINT('Ctrl Pts',(-15.5865359611318,-22.9,-11.8009489759233));
#27021=CARTESIAN_POINT('Ctrl Pts',(-15.4355591423194,-21.9000000281286,
-12.8401585976865));
#27022=CARTESIAN_POINT('Ctrl Pts',(-15.5607856662644,-22.7827980547194,
-12.8191871306931));
#27023=CARTESIAN_POINT('Ctrl Pts',(-15.3559607473148,-22.9,-11.9647821254094));
#27024=CARTESIAN_POINT('Ctrl Pts',(-15.1328683878844,-21.9617206530121,
-12.915148108118));
#27025=CARTESIAN_POINT('Ctrl Pts',(-15.2973142372121,-22.7172748074559,
-12.8709905227205));
#27026=CARTESIAN_POINT('Ctrl Pts',(-15.1190374158585,-22.9205735494498,
-12.1462781863214));
#27027=CARTESIAN_POINT('Ctrl Pts',(-14.5466360368447,-22.151057204958,-13.105466734237));
#27028=CARTESIAN_POINT('Ctrl Pts',(-14.7359632242303,-22.6985884975719,
-13.0355614944526));
#27029=CARTESIAN_POINT('Ctrl Pts',(-14.6271245805211,-22.9836857365402,
-12.5399038917136));
#27030=CARTESIAN_POINT('Ctrl Pts',(-14.2714100237779,-22.2772310832513,
-13.2181656147264));
#27031=CARTESIAN_POINT('Ctrl Pts',(-14.4436326996405,-22.7356048512221,
-13.1424140441331));
#27032=CARTESIAN_POINT('Ctrl Pts',(-14.3791131979061,-23.0257436937059,
-12.7464145774643));
#27033=CARTESIAN_POINT('Ctrl Pts',(-13.4894327977986,-22.7027835382778,
-13.6005990193291));
#27034=CARTESIAN_POINT('Ctrl Pts',(-13.6265116615004,-22.9266590509666,
-13.5179293418098));
#27035=CARTESIAN_POINT('Ctrl Pts',(-13.6286677467514,-23.1675945141816,
-13.3832301131747));
#27036=CARTESIAN_POINT('Ctrl Pts',(-13.0193938287093,-23.0534635977063,
-13.9179739028087));
#27037=CARTESIAN_POINT('Ctrl Pts',(-13.0648889625215,-23.1694382547513,
-13.8778509661652));
#27038=CARTESIAN_POINT('Ctrl Pts',(-13.1126423384301,-23.2843988132432,
-13.8357364471925));
#27039=CARTESIAN_POINT('Ctrl Pts',(-12.6003906189451,-23.4,-14.2875));
#27040=CARTESIAN_POINT('Ctrl Pts',(-12.6003906189451,-23.4,-14.2875));
#27041=CARTESIAN_POINT('Ctrl Pts',(-12.6003906189451,-23.4,-14.2875));
#27042=CARTESIAN_POINT('Ctrl Pts',(18.9499045174787,-21.9,-7.24776858010006));
#27043=CARTESIAN_POINT('Ctrl Pts',(18.9499045174787,-22.9,-7.24776858010006));
#27044=CARTESIAN_POINT('Ctrl Pts',(18.0131895824795,-22.9,-7.59786161137808));
#27045=CARTESIAN_POINT('Ctrl Pts',(18.8376831053774,-21.9000000281286,-6.94750704002252));
#27046=CARTESIAN_POINT('Ctrl Pts',(18.8821345441792,-22.7827980547207,-7.06644212448199));
#27047=CARTESIAN_POINT('Ctrl Pts',(18.0397856450054,-22.9,-7.31626104398644));
#27048=CARTESIAN_POINT('Ctrl Pts',(18.7512805492109,-21.9617206530127,-6.64787440197507));
#27049=CARTESIAN_POINT('Ctrl Pts',(18.7952618831513,-22.7172748074566,-6.81236747773836));
#27050=CARTESIAN_POINT('Ctrl Pts',(18.0785041787165,-22.9205735494498,-7.02033138973984));
#27051=CARTESIAN_POINT('Ctrl Pts',(18.6229851387236,-22.1510572049574,-6.04502298039525));
#27052=CARTESIAN_POINT('Ctrl Pts',(18.6571090189048,-22.6985884975713,-6.24393775419057));
#27053=CARTESIAN_POINT('Ctrl Pts',(18.1734376214998,-22.9836857365402,-6.39750952519446));
#27054=CARTESIAN_POINT('Ctrl Pts',(18.582972225672,-22.2772310832513,-5.75032082105227));
#27055=CARTESIAN_POINT('Ctrl Pts',(18.6034807790932,-22.7356048512228,-5.93734581875364));
#27056=CARTESIAN_POINT('Ctrl Pts',(18.2282754302052,-23.0257436937062,-6.07947002454654));
#27057=CARTESIAN_POINT('Ctrl Pts',(18.5231806563241,-22.7027835382778,-4.88189197587188));
#27058=CARTESIAN_POINT('Ctrl Pts',(18.5201260473201,-22.9266590509653,-5.04194059291939));
#27059=CARTESIAN_POINT('Ctrl Pts',(18.4045511360785,-23.1675945141811,-5.11115743183685));
#27060=CARTESIAN_POINT('Ctrl Pts',(18.5630158834026,-23.0534635976512,-4.31613884609869));
#27061=CARTESIAN_POINT('Ctrl Pts',(18.5510159678978,-23.1694382547042,-4.37560025606624));
#27062=CARTESIAN_POINT('Ctrl Pts',(18.5384204125509,-23.2843988132179,-4.43801315221929));
#27063=CARTESIAN_POINT('Ctrl Pts',(18.6735332660427,-23.4,-3.76850837361349));
#27064=CARTESIAN_POINT('Ctrl Pts',(18.6735332660427,-23.4,-3.76850837361349));
#27065=CARTESIAN_POINT('Ctrl Pts',(18.6735332660427,-23.4,-3.76850837361349));
#27066=CARTESIAN_POINT('Origin',(18.0131895824795,-21.9,-7.59786161137808));
#27067=CARTESIAN_POINT('Origin',(24.8980443547237,-21.9,-5.02467783148466));
#27068=CARTESIAN_POINT('Origin',(18.5327576369081,-21.9,-8.69967783148469));
#27069=CARTESIAN_POINT('Origin',(10.1324972242779,-21.9,5.85000000000005));
#27070=CARTESIAN_POINT('Origin',(34.1324972242781,-21.9,-35.7192193816529));
#27071=CARTESIAN_POINT('Origin',(30.6683956091404,-21.9,-37.7192193816529));
#27072=CARTESIAN_POINT('Origin',(32.6683956091404,-21.9,-41.1833209967907));
#27073=CARTESIAN_POINT('Origin',(15.0014773719379,-21.9,-51.3833209967907));
#27074=CARTESIAN_POINT('Origin',(19.3316043908601,-21.9,-48.8833209967907));
#27075=CARTESIAN_POINT('Origin',(17.33160439086,-21.9,-45.419219381653));
#27076=CARTESIAN_POINT('Origin',(13.8675027757223,-21.9,-47.419219381653));
#27077=CARTESIAN_POINT('Origin',(13.8675027757223,-21.9,-47.419219381653));
#27078=CARTESIAN_POINT('Origin',(-1.73223681164776,-21.9,-20.3996778314848));
#27079=CARTESIAN_POINT('Origin',(-8.09752352946338,-21.9,-24.0746778314848));
#27080=CARTESIAN_POINT('Origin',(-2.42665362134758,-21.9,-19.3988105873015));
#27081=CARTESIAN_POINT('Ctrl Pts',(-2.42665362134758,-22.9,-19.3988105873015));
#27082=CARTESIAN_POINT('Ctrl Pts',(-3.19820054762184,-22.9,-20.0349830014761));
#27083=CARTESIAN_POINT('Ctrl Pts',(-3.19820054762184,-21.9,-20.0349830014761));
#27084=CARTESIAN_POINT('Ctrl Pts',(-2.6838248976923,-22.9,-19.281043169395));
#27085=CARTESIAN_POINT('Ctrl Pts',(-3.32134887791377,-22.7827980547212,
-19.8856292551749));
#27086=CARTESIAN_POINT('Ctrl Pts',(-3.40212396305772,-21.9000000281286,
-19.7876656377092));
#27087=CARTESIAN_POINT('Ctrl Pts',(-2.9594667628583,-22.9205735494497,-19.1666095760619));
#27088=CARTESIAN_POINT('Ctrl Pts',(-3.49794764593905,-22.7172748074552,
-19.6833580004591));
#27089=CARTESIAN_POINT('Ctrl Pts',(-3.61841216132671,-21.9617206530128,
-19.5630225100931));
#27090=CARTESIAN_POINT('Ctrl Pts',(-3.54631304097816,-22.9836857365404,
-18.9374134169076));
#27091=CARTESIAN_POINT('Ctrl Pts',(-3.92114579467461,-22.6985884975725,
-19.2794992486431));
#27092=CARTESIAN_POINT('Ctrl Pts',(-4.07634910187847,-22.1510572049574,
-19.1504897146324));
#27093=CARTESIAN_POINT('Ctrl Pts',(-3.84916223229935,-23.0257436937064,
-18.8258846020106));
#27094=CARTESIAN_POINT('Ctrl Pts',(-4.15984807945244,-22.7356048512215,
-19.0797598628861));
#27095=CARTESIAN_POINT('Ctrl Pts',(-4.31156220189444,-22.2772310832507,
-18.9684864357784));
#27096=CARTESIAN_POINT('Ctrl Pts',(-4.77588338932629,-23.1675945141807,
-18.4943875450126));
#27097=CARTESIAN_POINT('Ctrl Pts',(-4.8936143858196,-22.9266590509677,-18.5598699347309));
#27098=CARTESIAN_POINT('Ctrl Pts',(-5.03374785852442,-22.702783538279,-18.4824909952018));
#27099=CARTESIAN_POINT('Ctrl Pts',(-5.42577807412219,-23.2843988132312,
-18.2737495994153));
#27100=CARTESIAN_POINT('Ctrl Pts',(-5.48612700538341,-23.169438254721,-18.2534512222455));
#27101=CARTESIAN_POINT('Ctrl Pts',(-5.54362205470623,-23.053463597673,-18.2341127489343));
#27102=CARTESIAN_POINT('Ctrl Pts',(-6.07314264709753,-23.4,-18.0560083736136));
#27103=CARTESIAN_POINT('Ctrl Pts',(-6.07314264709753,-23.4,-18.0560083736136));
#27104=CARTESIAN_POINT('Ctrl Pts',(-6.07314264709753,-23.4,-18.0560083736136));
#27105=CARTESIAN_POINT('Ctrl Pts',(-3.19820054762209,-21.9,20.0349830014761));
#27106=CARTESIAN_POINT('Ctrl Pts',(-3.19820054762209,-22.9,20.0349830014761));
#27107=CARTESIAN_POINT('Ctrl Pts',(-2.42665362134782,-22.9,19.3988105873015));
#27108=CARTESIAN_POINT('Ctrl Pts',(-3.40212396305782,-21.9000000281286,
19.7876656377093));
#27109=CARTESIAN_POINT('Ctrl Pts',(-3.32134887791476,-22.7827980547218,
19.8856292551756));
#27110=CARTESIAN_POINT('Ctrl Pts',(-2.68382489769184,-22.9,19.2810431693938));
#27111=CARTESIAN_POINT('Ctrl Pts',(-3.61841216132718,-21.9617206530121,
19.5630225100929));
#27112=CARTESIAN_POINT('Ctrl Pts',(-3.49794764593911,-22.7172748074559,
19.6833580004577));
#27113=CARTESIAN_POINT('Ctrl Pts',(-2.95946676285849,-22.9205735494499,
19.1666095760613));
#27114=CARTESIAN_POINT('Ctrl Pts',(-4.07634910187848,-22.151057204958,19.1504897146326));
#27115=CARTESIAN_POINT('Ctrl Pts',(-3.92114579467499,-22.6985884975719,
19.2794992486443));
#27116=CARTESIAN_POINT('Ctrl Pts',(-3.54631304097847,-22.9836857365401,
18.9374134169081));
#27117=CARTESIAN_POINT('Ctrl Pts',(-4.31156220189439,-22.2772310832513,
18.9684864357786));
#27118=CARTESIAN_POINT('Ctrl Pts',(-4.15984807945252,-22.7356048512228,
19.079759862886));
#27119=CARTESIAN_POINT('Ctrl Pts',(-3.84916223229944,-23.0257436937064,
18.8258846020105));
#27120=CARTESIAN_POINT('Ctrl Pts',(-5.03374785852525,-22.7027835382778,
18.4824909952013));
#27121=CARTESIAN_POINT('Ctrl Pts',(-4.89361438582019,-22.9266590509653,
18.5598699347308));
#27122=CARTESIAN_POINT('Ctrl Pts',(-4.77588338932682,-23.1675945141806,
18.4943875450126));
#27123=CARTESIAN_POINT('Ctrl Pts',(-5.54362205469395,-23.0534635976944,
18.2341127489385));
#27124=CARTESIAN_POINT('Ctrl Pts',(-5.48612700537819,-23.1694382547378,
18.2534512222473));
#27125=CARTESIAN_POINT('Ctrl Pts',(-5.42577807412138,-23.2843988132367,
18.2737495994156));
#27126=CARTESIAN_POINT('Ctrl Pts',(-6.07314264709777,-23.4,18.0560083736135));
#27127=CARTESIAN_POINT('Ctrl Pts',(-6.07314264709777,-23.4,18.0560083736135));
#27128=CARTESIAN_POINT('Ctrl Pts',(-6.07314264709777,-23.4,18.0560083736135));
#27129=CARTESIAN_POINT('Origin',(-2.42665362134782,-21.9,19.3988105873015));
#27130=CARTESIAN_POINT('Origin',(-8.09752352946369,-21.9,24.0746778314847));
#27131=CARTESIAN_POINT('Origin',(-1.73223681164803,-21.9,20.3996778314848));
#27132=CARTESIAN_POINT('Origin',(-10.132497224278,-21.9,5.8499999999999));
#27133=CARTESIAN_POINT('Origin',(36.998522628062,-21.9,38.6833209967911));
#27134=CARTESIAN_POINT('Origin',(32.6683956091398,-21.9,41.1833209967911));
#27135=CARTESIAN_POINT('Origin',(30.6683956091398,-21.9,37.7192193816533));
#27136=CARTESIAN_POINT('Origin',(34.1324972242776,-21.9,35.7192193816534));
#27137=CARTESIAN_POINT('Origin',(34.1324972242776,-21.9,35.7192193816534));
#27138=CARTESIAN_POINT('Origin',(18.5327576369079,-21.9,8.69967783148496));
#27139=CARTESIAN_POINT('Origin',(24.8980443547236,-21.9,5.02467783148503));
#27140=CARTESIAN_POINT('Origin',(18.0131895824794,-21.9,7.59786161137834));
#27141=CARTESIAN_POINT('Ctrl Pts',(18.0131895824794,-22.9,7.59786161137834));
#27142=CARTESIAN_POINT('Ctrl Pts',(18.9499045174786,-22.9,7.24776858010034));
#27143=CARTESIAN_POINT('Ctrl Pts',(18.9499045174786,-21.9,7.24776858010033));
#27144=CARTESIAN_POINT('Ctrl Pts',(18.0397856450098,-22.9,7.31626104398709));
#27145=CARTESIAN_POINT('Ctrl Pts',(18.8821345441806,-22.7827980547183,7.06644212448328));
#27146=CARTESIAN_POINT('Ctrl Pts',(18.8376831053773,-21.9000000281286,6.9475070400228));
#27147=CARTESIAN_POINT('Ctrl Pts',(18.0785041787167,-22.9205735494497,7.02033138974019));
#27148=CARTESIAN_POINT('Ctrl Pts',(18.7952618831505,-22.7172748074566,6.81236747773876));
#27149=CARTESIAN_POINT('Ctrl Pts',(18.7512805492108,-21.9617206530121,6.64787440197535));
#27150=CARTESIAN_POINT('Ctrl Pts',(18.1734376214995,-22.9836857365403,6.39750952519463));
#27151=CARTESIAN_POINT('Ctrl Pts',(18.6571090189054,-22.6985884975713,6.24393775419066));
#27152=CARTESIAN_POINT('Ctrl Pts',(18.6229851387235,-22.151057204958,6.04502298039552));
#27153=CARTESIAN_POINT('Ctrl Pts',(18.2282754302052,-23.0257436937062,6.0794700245468));
#27154=CARTESIAN_POINT('Ctrl Pts',(18.6034807790925,-22.7356048512234,5.93734581875439));
#27155=CARTESIAN_POINT('Ctrl Pts',(18.5829722256719,-22.2772310832513,5.75032082105249));
#27156=CARTESIAN_POINT('Ctrl Pts',(18.4045511360784,-23.1675945141811,5.11115743183711));
#27157=CARTESIAN_POINT('Ctrl Pts',(18.5201260473212,-22.9266590509641,5.04194059291876));
#27158=CARTESIAN_POINT('Ctrl Pts',(18.523180656324,-22.7027835382778,4.88189197587223));
#27159=CARTESIAN_POINT('Ctrl Pts',(18.5384204125495,-23.2843988132564,4.43801315222598));
#27160=CARTESIAN_POINT('Ctrl Pts',(18.5510159678927,-23.1694382547702,4.37560025609122));
#27161=CARTESIAN_POINT('Ctrl Pts',(18.5630158833926,-23.053463597732,4.31613884614811));
#27162=CARTESIAN_POINT('Ctrl Pts',(18.6735332660427,-23.4,3.76850837361377));
#27163=CARTESIAN_POINT('Ctrl Pts',(18.6735332660427,-23.4,3.76850837361377));
#27164=CARTESIAN_POINT('Ctrl Pts',(18.6735332660427,-23.4,3.76850837361377));
#40791=UNCERTAINTY_MEASURE_WITH_UNIT(LENGTH_MEASURE(0.01),#40810,
'DISTANCE_ACCURACY_VALUE',
'Maximum model space distance between geometric entities at asserted c
onnectivities');
#40799=UNCERTAINTY_MEASURE_WITH_UNIT(LENGTH_MEASURE(0.01),#40810,
'DISTANCE_ACCURACY_VALUE',
'Maximum model space distance between geometric entities at asserted c
onnectivities');
#40801=(
GEOMETRIC_REPRESENTATION_CONTEXT(3)
GLOBAL_UNCERTAINTY_ASSIGNED_CONTEXT((#40791))
GLOBAL_UNIT_ASSIGNED_CONTEXT((#40810,#40812,#40813))
REPRESENTATION_CONTEXT('','3D')
);
#40809=(
GEOMETRIC_REPRESENTATION_CONTEXT(3)
GLOBAL_UNCERTAINTY_ASSIGNED_CONTEXT((#40799))
GLOBAL_UNIT_ASSIGNED_CONTEXT((#40810,#40812,#40813))
REPRESENTATION_CONTEXT('','3D')
);
#40810=(
LENGTH_UNIT()
NAMED_UNIT(*)
SI_UNIT(.MILLI.,.METRE.)
);
#40812=(
NAMED_UNIT(*)
PLANE_ANGLE_UNIT()
SI_UNIT($,.RADIAN.)
);
#40813=(
NAMED_UNIT(*)
SI_UNIT($,.STERADIAN.)
SOLID_ANGLE_UNIT()
);
#40815=SHAPE_DEFINITION_REPRESENTATION(#40824,#40857);
#40824=PRODUCT_DEFINITION_SHAPE('',$,#40867);
#40857=SHAPE_REPRESENTATION('',(#6396),#40801);
#40865=PRODUCT_DEFINITION_CONTEXT('part definition',#40894,'design');
#40867=PRODUCT_DEFINITION('Spider Wheel','Spider Wheel',#40876,#40865);
#40876=PRODUCT_DEFINITION_FORMATION('',$,#40897);
#40894=APPLICATION_CONTEXT(
'Core Data for Automotive Mechanical Design Process');
#40895=PRODUCT_CONTEXT('part definition',#40894,'mechanical');
#40897=PRODUCT('Spider Wheel','Spider Wheel',$,(#40895));
#40906=PRESENTATION_STYLE_ASSIGNMENT((#40911));
#40911=SURFACE_STYLE_USAGE(.BOTH.,#40916);
#40916=SURFACE_SIDE_STYLE('',(#40921));
#40921=SURFACE_STYLE_FILL_AREA(#40926);
#40926=FILL_AREA_STYLE('Opaque(227,224,212)',(#40931));
#40931=FILL_AREA_STYLE_COLOUR('Opaque(227,224,212)',#40936);
#40936=COLOUR_RGB('Opaque(227,224,212)',0.890196078431372,0.87843137254902,
0.831372549019608);
ENDSEC;
END-ISO-10303-21;
